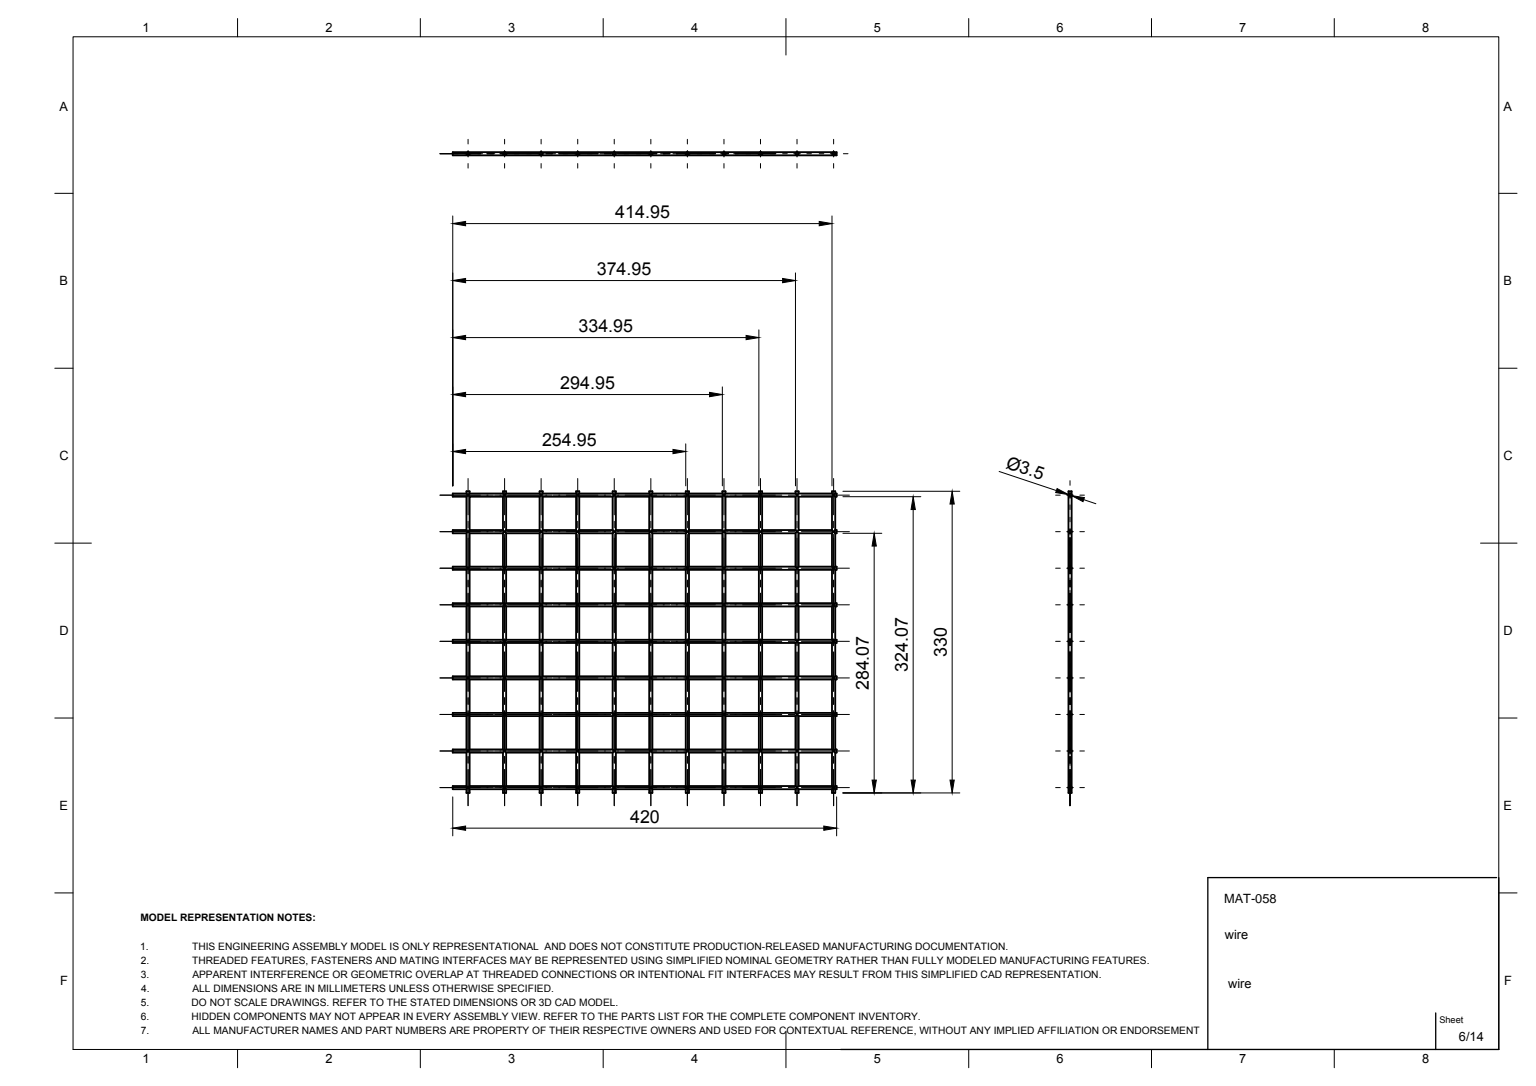
ISO-10303-21;
HEADER;
FILE_DESCRIPTION (('STEP AP214'),
    '1' );
FILE_NAME ('wire.step',
    '2026-10-21T17:54:40',
    ( '' ),
    ( '' ),
    'SwSTEP 2.0',
    'SolidWorks 2026',
    '' );
FILE_SCHEMA (( 'AUTOMOTIVE_DESIGN' ));
ENDSEC;

DATA;
#4=FACE_OUTER_BOUND ( 'NONE', #5138, .T. ) ;
#5=ORIENTED_EDGE ( 'NONE', *, *, #50322, .T. ) ;
#7=ORIENTED_EDGE ( 'NONE', *, *, #34701, .F. ) ;
#9=DIRECTION ( 'NONE',  ( -1.000000000000000000, -0.000000000000000000, -0.000000000000000000 ) ) ;
#11=ORIENTED_EDGE ( 'NONE', *, *, #36636, .F. ) ;
#12=EDGE_CURVE ( 'NONE', #49361, #27194, #1364, .T. ) ;
#14=ORIENTED_EDGE ( 'NONE', *, *, #5906, .T. ) ;
#15=CARTESIAN_POINT ( 'NONE',  ( 71.55402655318505367, 1.025126265847089657, 79.06828755692797017 ) ) ;
#16=DIRECTION ( 'NONE',  ( -1.000000000000000000, -0.000000000000000000, -0.000000000000000000 ) ) ;
#17=ORIENTED_EDGE ( 'NONE', *, *, #15192, .T. ) ;
#21=CARTESIAN_POINT ( 'NONE',  ( 191.5540265531851105, 0.000000000000000000, 162.5682875569279702 ) ) ;
#29=CARTESIAN_POINT ( 'NONE',  ( 155.0540265531850537, 2.143131898507880377E-16, -37.43171244307205825 ) ) ;
#39=CARTESIAN_POINT ( 'NONE',  ( -48.44597344681495343, 0.000000000000000000, 159.0682875569279702 ) ) ;
#41=DIRECTION ( 'NONE',  ( -1.000000000000000000, -0.000000000000000000, -0.000000000000000000 ) ) ;
#47=ADVANCED_FACE ( 'NONE', ( #25459 ), #1863, .T. ) ;
#50=CARTESIAN_POINT ( 'NONE',  ( 112.2789002873379758, -1.749999999999996891, -80.20683870891909351 ) ) ;
#54=CARTESIAN_POINT ( 'NONE',  ( -85.67084718096784002, 1.750000000000010214, -118.1565861772249519 ) ) ;
#60=AXIS2_PLACEMENT_3D ( 'NONE', #7908, #4040, #30745 ) ;
#63=ORIENTED_EDGE ( 'NONE', *, *, #25801, .F. ) ;
#64=CYLINDRICAL_SURFACE ( 'NONE', #8155, 1.750000000000001554 ) ;
#66=ORIENTED_EDGE ( 'NONE', *, *, #13113, .F. ) ;
#78=DIRECTION ( 'NONE',  ( -0.000000000000000000, -0.000000000000000000, -1.000000000000000000 ) ) ;
#81=EDGE_CURVE ( 'NONE', #16655, #7516, #13481, .T. ) ;
#82=ORIENTED_EDGE ( 'NONE', *, *, #7839, .T. ) ;
#85=ORIENTED_EDGE ( 'NONE', *, *, #19964, .F. ) ;
#86=CARTESIAN_POINT ( 'NONE',  ( 71.55402655318505367, 0.000000000000000000, 165.0000000000000000 ) ) ;
#90=CARTESIAN_POINT ( 'NONE',  ( 193.3040265531851105, 1.750000000000010658, 80.81828755692798438 ) ) ;
#95=CARTESIAN_POINT ( 'NONE',  ( 111.5540265531850679, 0.000000000000000000, -77.43171244307204404 ) ) ;
#104=CARTESIAN_POINT ( 'NONE',  ( -164.9459734468149463, 1.025126265847089435, -40.93171244307204404 ) ) ;
#112=ORIENTED_EDGE ( 'NONE', *, *, #36233, .F. ) ;
#113=EDGE_CURVE ( 'NONE', #40036, #44970, #10285, .T. ) ;
#122=( BOUNDED_CURVE ( )  B_SPLINE_CURVE ( 3, ( #11119, #46228, #4929, #44170 ),
 .UNSPECIFIED., .F., .F. ) 
 B_SPLINE_CURVE_WITH_KNOTS ( ( 4, 4 ),
 ( 0.000000000000000000, 1.570796326794896558 ),
 .UNSPECIFIED. ) 
 CURVE ( )  GEOMETRIC_REPRESENTATION_ITEM ( )  RATIONAL_B_SPLINE_CURVE ( ( 1.000000000000000000, 0.8047378541243649375, 0.8047378541243649375, 1.000000000000000000 ) ) 
 REPRESENTATION_ITEM ( '' )  );
#124=DIRECTION ( 'NONE',  ( -0.000000000000000000, -0.000000000000000000, -1.000000000000000000 ) ) ;
#136=CARTESIAN_POINT ( 'NONE',  ( -127.7210997126620242, -1.749999999999996891, 119.7931612910809065 ) ) ;
#139=ORIENTED_EDGE ( 'NONE', *, *, #39135, .F. ) ;
#143=ADVANCED_FACE ( 'NONE', ( #18750 ), #30578, .T. ) ;
#144=FACE_OUTER_BOUND ( 'NONE', #19501, .T. ) ;
#145=ORIENTED_EDGE ( 'NONE', *, *, #17426, .F. ) ;
#147=CARTESIAN_POINT ( 'NONE',  ( -44.94597344681493922, 2.143131898507880377E-16, -37.43171244307200141 ) ) ;
#155=DIRECTION ( 'NONE',  ( 0.000000000000000000, 0.000000000000000000, 1.000000000000000000 ) ) ;
#159=CARTESIAN_POINT ( 'NONE',  ( 73.30402655318508209, 1.750000000000010658, -119.1817124430720440 ) ) ;
#160=ORIENTED_EDGE ( 'NONE', *, *, #20171, .T. ) ;
#161=ORIENTED_EDGE ( 'NONE', *, *, #26521, .T. ) ;
#163=CARTESIAN_POINT ( 'NONE',  ( -124.9459734468149463, 2.143131898507847836E-16, -120.9317124430720156 ) ) ;
#172=EDGE_CURVE ( 'NONE', #7661, #23271, #44918, .T. ) ;
#173=CARTESIAN_POINT ( 'NONE',  ( 113.3040265531850537, 1.749999999999997113, 40.81828755692798438 ) ) ;
#179=ORIENTED_EDGE ( 'NONE', *, *, #14430, .F. ) ;
#182=ADVANCED_FACE ( 'NONE', ( #17198 ), #5386, .T. ) ;
#183=DIRECTION ( 'NONE',  ( -1.000000000000000000, -0.000000000000000000, -0.000000000000000000 ) ) ;
#184=CARTESIAN_POINT ( 'NONE',  ( 115.0540265531850395, 2.143131898507847836E-16, 42.56828755692795596 ) ) ;
#190=CARTESIAN_POINT ( 'NONE',  ( 151.5540265531850537, 1.025126265847089435, 39.06828755692797728 ) ) ;
#191=ORIENTED_EDGE ( 'NONE', *, *, #24035, .F. ) ;
#192=CARTESIAN_POINT ( 'NONE',  ( -88.44597344681497475, 0.000000000000000000, 122.5682875569279986 ) ) ;
#194=ADVANCED_FACE ( 'NONE', ( #21045 ), #12090, .T. ) ;
#199=CYLINDRICAL_SURFACE ( 'NONE', #44476, 1.750000000000015543 ) ;
#201=AXIS2_PLACEMENT_3D ( 'NONE', #39874, #40365, #36024 ) ;
#202=ORIENTED_EDGE ( 'NONE', *, *, #48337, .T. ) ;
#205=ORIENTED_EDGE ( 'NONE', *, *, #34328, .T. ) ;
#206=CARTESIAN_POINT ( 'NONE',  ( -46.69597344681494633, -1.750000000000010214, -39.18171244307202983 ) ) ;
#214=VERTEX_POINT ( 'NONE', #5134 ) ;
#217=DIRECTION ( 'NONE',  ( -1.000000000000000000, -0.000000000000000000, -0.000000000000000000 ) ) ;
#222=EDGE_CURVE ( 'NONE', #31646, #38096, #39265, .T. ) ;
#226=VECTOR ( 'NONE', #47044, 1000.000000000000000 ) ;
#228=ORIENTED_EDGE ( 'NONE', *, *, #24802, .T. ) ;
#229=CARTESIAN_POINT ( 'NONE',  ( -166.6959734468149463, -1.750000000000010658, -79.18171244307201562 ) ) ;
#232=ADVANCED_FACE ( 'NONE', ( #4388 ), #35956, .T. ) ;
#237=AXIS2_PLACEMENT_3D ( 'NONE', #8518, #24169, #12111 ) ;
#242=EDGE_CURVE ( 'NONE', #42713, #16089, #36464, .T. ) ;
#247=EDGE_CURVE ( 'NONE', #43286, #47057, #22018, .T. ) ;
#248=LINE ( 'NONE', #3822, #36404 ) ;
#249=CARTESIAN_POINT ( 'NONE',  ( -128.4459734468149179, 0.000000000000000000, -117.4317124430720725 ) ) ;
#252=CARTESIAN_POINT ( 'NONE',  ( -86.69597344681494633, -1.750000000000009992, 0.8182875569279768335 ) ) ;
#258=CARTESIAN_POINT ( 'NONE',  ( 155.0540265531850537, 2.143131898507880377E-16, 165.0000000000000000 ) ) ;
#259=( BOUNDED_CURVE ( )  B_SPLINE_CURVE ( 3, ( #2249, #37429, #6606, #3247 ),
 .UNSPECIFIED., .F., .F. ) 
 B_SPLINE_CURVE_WITH_KNOTS ( ( 4, 4 ),
 ( 1.570796326794896558, 3.141592653589793116 ),
 .UNSPECIFIED. ) 
 CURVE ( )  GEOMETRIC_REPRESENTATION_ITEM ( )  RATIONAL_B_SPLINE_CURVE ( ( 1.000000000000000000, 0.8047378541243649375, 0.8047378541243649375, 1.000000000000000000 ) ) 
 REPRESENTATION_ITEM ( '' )  );
#266=DIRECTION ( 'NONE',  ( 0.000000000000000000, 0.000000000000000000, 1.000000000000000000 ) ) ;
#267=( BOUNDED_CURVE ( )  B_SPLINE_CURVE ( 3, ( #50247, #49055, #13937, #13448 ),
 .UNSPECIFIED., .F., .F. ) 
 B_SPLINE_CURVE_WITH_KNOTS ( ( 4, 4 ),
 ( 4.712388980384689674, 6.283185307179586232 ),
 .UNSPECIFIED. ) 
 CURVE ( )  GEOMETRIC_REPRESENTATION_ITEM ( )  RATIONAL_B_SPLINE_CURVE ( ( 1.000000000000000000, 0.8047378541243649375, 0.8047378541243649375, 1.000000000000000000 ) ) 
 REPRESENTATION_ITEM ( '' )  );
#268=ORIENTED_EDGE ( 'NONE', *, *, #3344, .T. ) ;
#271=CARTESIAN_POINT ( 'NONE',  ( 71.55402655318506788, 0.000000000000000000, 162.5682875569279702 ) ) ;
#273=VECTOR ( 'NONE', #4541, 1000.000000000000000 ) ;
#275=CARTESIAN_POINT ( 'NONE',  ( -84.94597344681493212, 1.025126265847089879, 122.5682875569280128 ) ) ;
#283=ORIENTED_EDGE ( 'NONE', *, *, #247, .F. ) ;
#288=CARTESIAN_POINT ( 'NONE',  ( -168.4459734468149463, 0.000000000000000000, 2.568287556927978166 ) ) ;
#293=LINE ( 'NONE', #43877, #10669 ) ;
#294=CARTESIAN_POINT ( 'NONE',  ( 74.32915281903215998, -1.750000000000009548, -78.15658617722490931 ) ) ;
#307=CARTESIAN_POINT ( 'NONE',  ( 113.3040265531850537, -1.749999999999997335, -79.18171244307201562 ) ) ;
#309=CARTESIAN_POINT ( 'NONE',  ( 192.2789002873380184, 1.750000000000009548, 39.79316129108089228 ) ) ;
#314=EDGE_CURVE ( 'NONE', #4361, #2042, #6678, .T. ) ;
#317=DIRECTION ( 'NONE',  ( -0.000000000000000000, -0.000000000000000000, -1.000000000000000000 ) ) ;
#320=CYLINDRICAL_SURFACE ( 'NONE', #46063, 1.750000000000015543 ) ;
#322=CARTESIAN_POINT ( 'NONE',  ( -128.4459734468149179, 0.000000000000000000, 165.0000000000000000 ) ) ;
#326=FACE_OUTER_BOUND ( 'NONE', #20541, .T. ) ;
#329=CARTESIAN_POINT ( 'NONE',  ( 191.5540265531850537, -1.025126265847089435, -157.4317124430720582 ) ) ;
#349=EDGE_LOOP ( 'NONE', ( #28250, #8227, #4948, #139, #25034, #3385 ) ) ;
#358=ORIENTED_EDGE ( 'NONE', *, *, #25263, .T. ) ;
#360=DIRECTION ( 'NONE',  ( 0.000000000000000000, 0.000000000000000000, 1.000000000000000000 ) ) ;
#361=CARTESIAN_POINT ( 'NONE',  ( -84.94597344681493212, -1.025126265847088991, 159.0682875569279418 ) ) ;
#367=ORIENTED_EDGE ( 'NONE', *, *, #18075, .F. ) ;
#368=CARTESIAN_POINT ( 'NONE',  ( -126.6959734468149321, -1.749999999999997335, 80.81828755692798438 ) ) ;
#371=VECTOR ( 'NONE', #12956, 1000.000000000000000 ) ;
#374=EDGE_LOOP ( 'NONE', ( #37007, #35684, #23876, #49067, #24411 ) ) ;
#379=FACE_OUTER_BOUND ( 'NONE', #33356, .T. ) ;
#381=AXIS2_PLACEMENT_3D ( 'NONE', #4181, #15227, #23679 ) ;
#382=CARTESIAN_POINT ( 'NONE',  ( 195.0540265531851105, 2.143131898507880377E-16, 79.06828755692797017 ) ) ;
#383=ORIENTED_EDGE ( 'NONE', *, *, #37796, .F. ) ;
#387=VERTEX_POINT ( 'NONE', #1801 ) ;
#394=CARTESIAN_POINT ( 'NONE',  ( 153.3040265531850537, 1.750000000000010658, 80.81828755692798438 ) ) ;
#406=ORIENTED_EDGE ( 'NONE', *, *, #20191, .F. ) ;
#407=DIRECTION ( 'NONE',  ( -0.000000000000000000, -0.000000000000000000, -1.000000000000000000 ) ) ;
#411=ORIENTED_EDGE ( 'NONE', *, *, #49299, .F. ) ;
#413=CARTESIAN_POINT ( 'NONE',  ( -126.6959734468149321, -1.749999999999997113, -39.18171244307202983 ) ) ;
#415=( BOUNDED_CURVE ( )  B_SPLINE_CURVE ( 3, ( #5683, #44416, #25963, #48241 ),
 .UNSPECIFIED., .F., .F. ) 
 B_SPLINE_CURVE_WITH_KNOTS ( ( 4, 4 ),
 ( 4.712388980384689674, 6.283185307179586232 ),
 .UNSPECIFIED. ) 
 CURVE ( )  GEOMETRIC_REPRESENTATION_ITEM ( )  RATIONAL_B_SPLINE_CURVE ( ( 1.000000000000000000, 0.8047378541243649375, 0.8047378541243649375, 1.000000000000000000 ) ) 
 REPRESENTATION_ITEM ( '' )  );
#421=ORIENTED_EDGE ( 'NONE', *, *, #38475, .T. ) ;
#423=CARTESIAN_POINT ( 'NONE',  ( -47.72109971266203132, 1.750000000000010436, 119.7931612910808781 ) ) ;
#425=CYLINDRICAL_SURFACE ( 'NONE', #22465, 1.750000000000001554 ) ;
#429=DIRECTION ( 'NONE',  ( -1.000000000000000000, 0.000000000000000000, 0.000000000000000000 ) ) ;
#431=EDGE_CURVE ( 'NONE', #16089, #12079, #28992, .T. ) ;
#436=AXIS2_PLACEMENT_3D ( 'NONE', #25349, #45321, #26098 ) ;
#440=EDGE_CURVE ( 'NONE', #43432, #19548, #26025, .T. ) ;
#443=VECTOR ( 'NONE', #3485, 1000.000000000000000 ) ;
#447=CARTESIAN_POINT ( 'NONE',  ( 35.05402655318504657, 2.143131898507880377E-16, 42.56828755692798438 ) ) ;
#448=DIRECTION ( 'NONE',  ( 0.000000000000000000, 0.000000000000000000, 1.000000000000000000 ) ) ;
#452=ADVANCED_FACE ( 'NONE', ( #16069 ), #23519, .T. ) ;
#454=ORIENTED_EDGE ( 'NONE', *, *, #15929, .F. ) ;
#458=EDGE_CURVE ( 'NONE', #40596, #15960, #31982, .T. ) ;
#459=EDGE_CURVE ( 'NONE', #16448, #40222, #8626, .T. ) ;
#464=EDGE_CURVE ( 'NONE', #48470, #25557, #25629, .T. ) ;
#466=DIRECTION ( 'NONE',  ( 0.000000000000000000, 0.000000000000000000, 1.000000000000000000 ) ) ;
#467=ORIENTED_EDGE ( 'NONE', *, *, #8643, .T. ) ;
#470=AXIS2_PLACEMENT_3D ( 'NONE', #3136, #22152, #46465 ) ;
#472=CYLINDRICAL_SURFACE ( 'NONE', #11197, 1.750000000000008438 ) ;
#482=EDGE_CURVE ( 'NONE', #50669, #27161, #35845, .T. ) ;
#485=DIRECTION ( 'NONE',  ( -0.000000000000000000, -0.000000000000000000, -1.000000000000000000 ) ) ;
#488=CARTESIAN_POINT ( 'NONE',  ( -87.72109971266203843, -1.750000000000009548, 159.7931612910809065 ) ) ;
#491=AXIS2_PLACEMENT_3D ( 'NONE', #861, #24715, #16507 ) ;
#502=( BOUNDED_CURVE ( )  B_SPLINE_CURVE ( 3, ( #2955, #14255, #29915, #26067 ),
 .UNSPECIFIED., .F., .F. ) 
 B_SPLINE_CURVE_WITH_KNOTS ( ( 4, 4 ),
 ( 1.570796326794896558, 3.141592653589793116 ),
 .UNSPECIFIED. ) 
 CURVE ( )  GEOMETRIC_REPRESENTATION_ITEM ( )  RATIONAL_B_SPLINE_CURVE ( ( 1.000000000000000000, 0.8047378541243649375, 0.8047378541243649375, 1.000000000000000000 ) ) 
 REPRESENTATION_ITEM ( '' )  );
#506=CARTESIAN_POINT ( 'NONE',  ( 193.3040265531851105, 1.750000000000010658, -119.1817124430720440 ) ) ;
#507=CARTESIAN_POINT ( 'NONE',  ( 113.3040265531850537, -1.749999999999996891, 160.8182875569279702 ) ) ;
#510=ORIENTED_EDGE ( 'NONE', *, *, #27958, .F. ) ;
#511=FACE_OUTER_BOUND ( 'NONE', #39266, .T. ) ;
#519=CARTESIAN_POINT ( 'NONE',  ( 191.5540265531851105, 0.000000000000000000, -77.43171244307204404 ) ) ;
#520=CARTESIAN_POINT ( 'NONE',  ( 111.5540265531850537, 1.025126265847081886, -120.9317124430720440 ) ) ;
#523=ORIENTED_EDGE ( 'NONE', *, *, #44396, .T. ) ;
#526=ADVANCED_FACE ( 'NONE', ( #38927 ), #19406, .T. ) ;
#527=ORIENTED_EDGE ( 'NONE', *, *, #43614, .T. ) ;
#531=ORIENTED_EDGE ( 'NONE', *, *, #41855, .T. ) ;
#532=CARTESIAN_POINT ( 'NONE',  ( -126.6959734468149321, 1.749999999999996891, -159.1817124430720298 ) ) ;
#534=EDGE_CURVE ( 'NONE', #28470, #12513, #27359, .T. ) ;
#538=AXIS2_PLACEMENT_3D ( 'NONE', #2831, #26198, #14128 ) ;
#543=CARTESIAN_POINT ( 'NONE',  ( -127.7210997126620242, -1.749999999999996891, -80.20683870891909351 ) ) ;
#544=EDGE_LOOP ( 'NONE', ( #3336, #43444, #1050, #33795, #29407 ) ) ;
#546=FACE_OUTER_BOUND ( 'NONE', #42414, .T. ) ;
#547=ORIENTED_EDGE ( 'NONE', *, *, #1230, .F. ) ;
#548=LINE ( 'NONE', #16187, #556 ) ;
#555=CARTESIAN_POINT ( 'NONE',  ( -206.6959734468149463, 0.000000000000000000, 165.0000000000000000 ) ) ;
#556=VECTOR ( 'NONE', #4868, 1000.000000000000000 ) ;
#559=VERTEX_POINT ( 'NONE', #44993 ) ;
#560=ORIENTED_EDGE ( 'NONE', *, *, #34963, .T. ) ;
#563=( BOUNDED_CURVE ( )  B_SPLINE_CURVE ( 3, ( #5786, #21426, #38810, #49593 ),
 .UNSPECIFIED., .F., .F. ) 
 B_SPLINE_CURVE_WITH_KNOTS ( ( 4, 4 ),
 ( 1.570796326794896558, 3.141592653589793116 ),
 .UNSPECIFIED. ) 
 CURVE ( )  GEOMETRIC_REPRESENTATION_ITEM ( )  RATIONAL_B_SPLINE_CURVE ( ( 1.000000000000000000, 0.8047378541243649375, 0.8047378541243649375, 1.000000000000000000 ) ) 
 REPRESENTATION_ITEM ( '' )  );
#567=DIRECTION ( 'NONE',  ( -1.000000000000000000, -0.000000000000000000, -0.000000000000000000 ) ) ;
#568=( BOUNDED_CURVE ( )  B_SPLINE_CURVE ( 3, ( #26623, #27136, #28083, #11235 ),
 .UNSPECIFIED., .F., .F. ) 
 B_SPLINE_CURVE_WITH_KNOTS ( ( 4, 4 ),
 ( 1.570796326794896558, 3.141592653589793116 ),
 .UNSPECIFIED. ) 
 CURVE ( )  GEOMETRIC_REPRESENTATION_ITEM ( )  RATIONAL_B_SPLINE_CURVE ( ( 1.000000000000000000, 0.8047378541243649375, 0.8047378541243649375, 1.000000000000000000 ) ) 
 REPRESENTATION_ITEM ( '' )  );
#569=CARTESIAN_POINT ( 'NONE',  ( -47.72109971266203132, -1.750000000000009548, 41.84341382277508359 ) ) ;
#571=DIRECTION ( 'NONE',  ( 0.000000000000000000, 0.000000000000000000, 1.000000000000000000 ) ) ;
#573=DIRECTION ( 'NONE',  ( -1.000000000000000000, -0.000000000000000000, -0.000000000000000000 ) ) ;
#575=FACE_OUTER_BOUND ( 'NONE', #37918, .T. ) ;
#577=CARTESIAN_POINT ( 'NONE',  ( -4.945973446814917018, 1.025126265847097429, 42.56828755692800570 ) ) ;
#578=CARTESIAN_POINT ( 'NONE',  ( -4.945973446814903696, 2.143131898507912917E-16, 2.568287556928034121 ) ) ;
#580=ORIENTED_EDGE ( 'NONE', *, *, #21589, .T. ) ;
#581=ADVANCED_FACE ( 'NONE', ( #9872 ), #36344, .T. ) ;
#583=EDGE_CURVE ( 'NONE', #42490, #24640, #48326, .T. ) ;
#585=DIRECTION ( 'NONE',  ( -1.000000000000000000, 0.000000000000000000, 0.000000000000000000 ) ) ;
#587=CARTESIAN_POINT ( 'NONE',  ( -206.6959734468149463, 1.750000000000010214, -39.18171244307202983 ) ) ;
#588=CARTESIAN_POINT ( 'NONE',  ( 32.27890028733795447, -1.750000000000009548, 41.84341382277508359 ) ) ;
#591=ORIENTED_EDGE ( 'NONE', *, *, #21037, .F. ) ;
#595=EDGE_CURVE ( 'NONE', #49549, #4874, #20923, .T. ) ;
#600=FACE_OUTER_BOUND ( 'NONE', #36261, .T. ) ;
#601=ORIENTED_EDGE ( 'NONE', *, *, #3400, .F. ) ;
#602=CARTESIAN_POINT ( 'NONE',  ( 195.0540265531851105, 2.143131898507880377E-16, 79.06828755692797017 ) ) ;
#604=ADVANCED_FACE ( 'NONE', ( #36090 ), #930, .T. ) ;
#610=DIRECTION ( 'NONE',  ( -1.000000000000000000, -0.000000000000000000, -0.000000000000000000 ) ) ;
#611=CARTESIAN_POINT ( 'NONE',  ( -5.670847180967843570, -1.750000000000023315, 121.8434138227750623 ) ) ;
#620=CARTESIAN_POINT ( 'NONE',  ( 34.32915281903212446, 1.750000000000009326, 161.8434138227750907 ) ) ;
#630=FACE_OUTER_BOUND ( 'NONE', #38256, .T. ) ;
#635=ORIENTED_EDGE ( 'NONE', *, *, #15818, .F. ) ;
#638=DIRECTION ( 'NONE',  ( 0.000000000000000000, 0.000000000000000000, -1.000000000000000000 ) ) ;
#641=DIRECTION ( 'NONE',  ( -0.000000000000000000, -0.000000000000000000, -1.000000000000000000 ) ) ;
#645=ORIENTED_EDGE ( 'NONE', *, *, #18172, .T. ) ;
#646=CARTESIAN_POINT ( 'NONE',  ( -124.9459734468149463, 2.143131898507847836E-16, -120.9317124430720156 ) ) ;
#649=DIRECTION ( 'NONE',  ( -0.000000000000000000, -0.000000000000000000, -1.000000000000000000 ) ) ;
#652=ORIENTED_EDGE ( 'NONE', *, *, #762, .F. ) ;
#653=ADVANCED_FACE ( 'NONE', ( #40684 ), #36606, .T. ) ;
#658=ORIENTED_EDGE ( 'NONE', *, *, #1230, .T. ) ;
#662=CIRCLE ( 'NONE', #47316, 1.750000000000001554 ) ;
#663=CARTESIAN_POINT ( 'NONE',  ( -204.9459734468149463, 2.143131898507880377E-16, 2.568287556927978166 ) ) ;
#667=CARTESIAN_POINT ( 'NONE',  ( -126.6959734468149321, 1.749999999999997335, 80.81828755692798438 ) ) ;
#676=CARTESIAN_POINT ( 'NONE',  ( 155.0540265531850537, 1.025126265847089879, 122.5682875569280128 ) ) ;
#683=( BOUNDED_CURVE ( )  B_SPLINE_CURVE ( 3, ( #1713, #9405, #36121, #5040 ),
 .UNSPECIFIED., .F., .F. ) 
 B_SPLINE_CURVE_WITH_KNOTS ( ( 4, 4 ),
 ( 1.570796326794896558, 3.141592653589793116 ),
 .UNSPECIFIED. ) 
 CURVE ( )  GEOMETRIC_REPRESENTATION_ITEM ( )  RATIONAL_B_SPLINE_CURVE ( ( 1.000000000000000000, 0.8047378541243649375, 0.8047378541243649375, 1.000000000000000000 ) ) 
 REPRESENTATION_ITEM ( '' )  );
#687=ORIENTED_EDGE ( 'NONE', *, *, #36269, .F. ) ;
#689=CARTESIAN_POINT ( 'NONE',  ( 154.3291528190321458, -1.750000000000009548, -40.20683870891912193 ) ) ;
#691=CYLINDRICAL_SURFACE ( 'NONE', #41373, 1.750000000000015543 ) ;
#698=CARTESIAN_POINT ( 'NONE',  ( -210.0000000000000568, 0.000000000000000000, -119.1817124430720440 ) ) ;
#700=DIRECTION ( 'NONE',  ( 1.000000000000000000, 0.000000000000000000, 0.000000000000000000 ) ) ;
#703=ADVANCED_FACE ( 'NONE', ( #24523 ), #36856, .T. ) ;
#704=( BOUNDED_CURVE ( )  B_SPLINE_CURVE ( 3, ( #40799, #48942, #14089, #33120 ),
 .UNSPECIFIED., .F., .F. ) 
 B_SPLINE_CURVE_WITH_KNOTS ( ( 4, 4 ),
 ( 0.000000000000000000, 1.570796326794896558 ),
 .UNSPECIFIED. ) 
 CURVE ( )  GEOMETRIC_REPRESENTATION_ITEM ( )  RATIONAL_B_SPLINE_CURVE ( ( 1.000000000000000000, 0.8047378541243649375, 0.8047378541243649375, 1.000000000000000000 ) ) 
 REPRESENTATION_ITEM ( '' )  );
#705=CARTESIAN_POINT ( 'NONE',  ( 75.05402655318509630, 1.025126265847089879, 82.56828755692798438 ) ) ;
#713=CARTESIAN_POINT ( 'NONE',  ( 75.05402655318509630, 1.025126265847089879, 122.5682875569280128 ) ) ;
#714=ORIENTED_EDGE ( 'NONE', *, *, #39946, .T. ) ;
#719=EDGE_CURVE ( 'NONE', #32283, #25110, #43691, .T. ) ;
#725=CARTESIAN_POINT ( 'NONE',  ( 113.3040265531850537, 0.000000000000000000, 165.0000000000000000 ) ) ;
#729=CYLINDRICAL_SURFACE ( 'NONE', #31264, 1.750000000000015543 ) ;
#730=CARTESIAN_POINT ( 'NONE',  ( 152.2789002873379900, 1.750000000000009548, 159.7931612910809065 ) ) ;
#731=CARTESIAN_POINT ( 'NONE',  ( -204.9459734468149463, 2.143131898507880377E-16, -80.93171244307201562 ) ) ;
#734=PLANE ( 'NONE',  #17438 ) ;
#735=EDGE_CURVE ( 'NONE', #23031, #24640, #41747, .T. ) ;
#738=DIRECTION ( 'NONE',  ( -1.000000000000000000, -0.000000000000000000, -0.000000000000000000 ) ) ;
#741=CARTESIAN_POINT ( 'NONE',  ( -204.9459734468149463, 2.143131898507880377E-16, 39.06828755692798438 ) ) ;
#743=ORIENTED_EDGE ( 'NONE', *, *, #50525, .T. ) ;
#746=DIRECTION ( 'NONE',  ( -0.000000000000000000, -0.000000000000000000, -1.000000000000000000 ) ) ;
#748=CARTESIAN_POINT ( 'NONE',  ( 153.3040265531850537, -1.750000000000009992, 160.8182875569279702 ) ) ;
#749=VECTOR ( 'NONE', #19138, 1000.000000000000000 ) ;
#757=CARTESIAN_POINT ( 'NONE',  ( -124.9459734468149463, 2.143131898507847836E-16, -77.43171244307204404 ) ) ;
#758=VECTOR ( 'NONE', #16905, 1000.000000000000000 ) ;
#760=ORIENTED_EDGE ( 'NONE', *, *, #40276, .T. ) ;
#762=EDGE_CURVE ( 'NONE', #38466, #44684, #48892, .T. ) ;
#765=AXIS2_PLACEMENT_3D ( 'NONE', #29029, #12869, #12609 ) ;
#778=EDGE_CURVE ( 'NONE', #19154, #19994, #662, .T. ) ;
#784=DIRECTION ( 'NONE',  ( 1.000000000000000000, 0.000000000000000000, 0.000000000000000000 ) ) ;
#787=AXIS2_PLACEMENT_3D ( 'NONE', #7371, #10699, #11720 ) ;
#793=( BOUNDED_CURVE ( )  B_SPLINE_CURVE ( 3, ( #39098, #35003, #3405, #39345 ),
 .UNSPECIFIED., .F., .F. ) 
 B_SPLINE_CURVE_WITH_KNOTS ( ( 4, 4 ),
 ( 0.000000000000000000, 1.570796326794896558 ),
 .UNSPECIFIED. ) 
 CURVE ( )  GEOMETRIC_REPRESENTATION_ITEM ( )  RATIONAL_B_SPLINE_CURVE ( ( 1.000000000000000000, 0.8047378541243649375, 0.8047378541243649375, 1.000000000000000000 ) ) 
 REPRESENTATION_ITEM ( '' )  );
#796=VECTOR ( 'NONE', #5565, 1000.000000000000000 ) ;
#800=ORIENTED_EDGE ( 'NONE', *, *, #21171, .T. ) ;
#801=ADVANCED_FACE ( 'NONE', ( #14216 ), #41679, .T. ) ;
#807=EDGE_CURVE ( 'NONE', #14566, #8176, #18570, .T. ) ;
#809=DIRECTION ( 'NONE',  ( -1.000000000000000000, 0.000000000000000000, 0.000000000000000000 ) ) ;
#810=CARTESIAN_POINT ( 'NONE',  ( -85.67084718096784002, -1.750000000000010436, -80.20683870891910772 ) ) ;
#815=ADVANCED_FACE ( 'NONE', ( #7814 ), #26795, .T. ) ;
#824=CARTESIAN_POINT ( 'NONE',  ( 195.0540265531851105, 2.143131898507880377E-16, -80.93171244307201562 ) ) ;
#829=VERTEX_POINT ( 'NONE', #368 ) ;
#830=AXIS2_PLACEMENT_3D ( 'NONE', #22262, #22003, #42013 ) ;
#833=EDGE_CURVE ( 'NONE', #38070, #15143, #32836, .T. ) ;
#836=CARTESIAN_POINT ( 'NONE',  ( -208.4459734468148611, 1.025126265847089213, -37.43171244307202272 ) ) ;
#837=CARTESIAN_POINT ( 'NONE',  ( -44.94597344681493922, 2.143131898507880377E-16, 165.0000000000000000 ) ) ;
#840=AXIS2_PLACEMENT_3D ( 'NONE', #7728, #46676, #34680 ) ;
#841=ORIENTED_EDGE ( 'NONE', *, *, #33518, .T. ) ;
#851=LINE ( 'NONE', #19823, #3024 ) ;
#852=EDGE_CURVE ( 'NONE', #6557, #6202, #30915, .T. ) ;
#854=( BOUNDED_CURVE ( )  B_SPLINE_CURVE ( 3, ( #12564, #12315, #543, #19499 ),
 .UNSPECIFIED., .F., .F. ) 
 B_SPLINE_CURVE_WITH_KNOTS ( ( 4, 4 ),
 ( 0.000000000000000000, 1.570796326794896558 ),
 .UNSPECIFIED. ) 
 CURVE ( )  GEOMETRIC_REPRESENTATION_ITEM ( )  RATIONAL_B_SPLINE_CURVE ( ( 1.000000000000000000, 0.8047378541243649375, 0.8047378541243649375, 1.000000000000000000 ) ) 
 REPRESENTATION_ITEM ( '' )  );
#855=CARTESIAN_POINT ( 'NONE',  ( -204.9459734468148895, -1.025126265847089657, 119.0682875569279560 ) ) ;
#858=EDGE_CURVE ( 'NONE', #47433, #8314, #11391, .T. ) ;
#861=CARTESIAN_POINT ( 'NONE',  ( 153.3040265531850537, 0.000000000000000000, 165.0000000000000000 ) ) ;
#862=( BOUNDED_CURVE ( )  B_SPLINE_CURVE ( 3, ( #46764, #38884, #31695, #35808 ),
 .UNSPECIFIED., .F., .F. ) 
 B_SPLINE_CURVE_WITH_KNOTS ( ( 4, 4 ),
 ( 0.000000000000000000, 1.570796326794896780 ),
 .UNSPECIFIED. ) 
 CURVE ( )  GEOMETRIC_REPRESENTATION_ITEM ( )  RATIONAL_B_SPLINE_CURVE ( ( 1.000000000000000000, 0.8047378541243649375, 0.8047378541243649375, 1.000000000000000000 ) ) 
 REPRESENTATION_ITEM ( '' )  );
#864=ORIENTED_EDGE ( 'NONE', *, *, #18638, .T. ) ;
#868=ORIENTED_EDGE ( 'NONE', *, *, #35811, .F. ) ;
#872=CARTESIAN_POINT ( 'NONE',  ( 155.0540265531850537, -1.025126265847088991, -157.4317124430720582 ) ) ;
#886=DIRECTION ( 'NONE',  ( 1.000000000000000000, 0.000000000000000000, -0.000000000000000000 ) ) ;
#903=CARTESIAN_POINT ( 'NONE',  ( 153.3040265531850537, -1.750000000000010658, -119.1817124430720440 ) ) ;
#906=AXIS2_PLACEMENT_3D ( 'NONE', #14046, #29713, #45328 ) ;
#909=CARTESIAN_POINT ( 'NONE',  ( -44.94597344681493922, 2.143131898507880377E-16, 159.0682875569279702 ) ) ;
#910=CARTESIAN_POINT ( 'NONE',  ( 35.05402655318504657, 2.143131898507880377E-16, 42.56828755692798438 ) ) ;
#911=CARTESIAN_POINT ( 'NONE',  ( -204.9459734468148895, 1.025126265847089213, -0.9317124430720324924 ) ) ;
#915=ORIENTED_EDGE ( 'NONE', *, *, #35068, .T. ) ;
#918=CARTESIAN_POINT ( 'NONE',  ( -84.94597344681494633, 2.143131898507880377E-16, -77.43171244307204404 ) ) ;
#920=VERTEX_POINT ( 'NONE', #34765 ) ;
#923=FACE_OUTER_BOUND ( 'NONE', #18696, .T. ) ;
#924=CARTESIAN_POINT ( 'NONE',  ( -204.9459734468149463, 2.143131898507880377E-16, -117.4317124430720725 ) ) ;
#925=ORIENTED_EDGE ( 'NONE', *, *, #735, .T. ) ;
#926=ORIENTED_EDGE ( 'NONE', *, *, #50038, .F. ) ;
#928=CARTESIAN_POINT ( 'NONE',  ( -164.9459734468149463, 1.025126265847089657, -80.93171244307201562 ) ) ;
#930=CYLINDRICAL_SURFACE ( 'NONE', #24074, 1.750000000000015543 ) ;
#931=CARTESIAN_POINT ( 'NONE',  ( -207.7210997126620384, 1.750000000000009548, 121.8434138227750623 ) ) ;
#935=CARTESIAN_POINT ( 'NONE',  ( -84.94597344681494633, 2.143131898507873721E-16, 165.0000000000000000 ) ) ;
#936=VERTEX_POINT ( 'NONE', #12401 ) ;
#939=CARTESIAN_POINT ( 'NONE',  ( 210.0000000000000568, 0.000000000000000000, -79.18171244307201562 ) ) ;
#942=DIRECTION ( 'NONE',  ( -0.000000000000000000, -0.000000000000000000, -1.000000000000000000 ) ) ;
#944=ADVANCED_FACE ( 'NONE', ( #47762 ), #9567, .T. ) ;
#947=LINE ( 'NONE', #16587, #9432 ) ;
#956=CARTESIAN_POINT ( 'NONE',  ( -204.9459734468149463, 2.143131898507880377E-16, -77.43171244307204404 ) ) ;
#960=VERTEX_POINT ( 'NONE', #8817 ) ;
#962=CYLINDRICAL_SURFACE ( 'NONE', #6597, 1.750000000000008438 ) ;
#963=ORIENTED_EDGE ( 'NONE', *, *, #1726, .F. ) ;
#965=CYLINDRICAL_SURFACE ( 'NONE', #36426, 1.750000000000001554 ) ;
#969=CARTESIAN_POINT ( 'NONE',  ( 210.0000000000000568, 2.143131898507881856E-16, 119.0682875569279560 ) ) ;
#972=CARTESIAN_POINT ( 'NONE',  ( -8.445973446814962315, -1.025126265847097207, -157.4317124430720014 ) ) ;
#979=ORIENTED_EDGE ( 'NONE', *, *, #1420, .T. ) ;
#982=CARTESIAN_POINT ( 'NONE',  ( 191.5540265531850537, 1.025126265847089657, -80.93171244307201562 ) ) ;
#985=LINE ( 'NONE', #10188, #43833 ) ;
#986=CYLINDRICAL_SURFACE ( 'NONE', #23136, 1.750000000000008438 ) ;
#991=PLANE ( 'NONE',  #47135 ) ;
#992=FACE_OUTER_BOUND ( 'NONE', #20572, .T. ) ;
#995=( BOUNDED_CURVE ( )  B_SPLINE_CURVE ( 3, ( #20608, #1379, #32169, #1875 ),
 .UNSPECIFIED., .F., .F. ) 
 B_SPLINE_CURVE_WITH_KNOTS ( ( 4, 4 ),
 ( 0.000000000000000000, 1.570796326794896558 ),
 .UNSPECIFIED. ) 
 CURVE ( )  GEOMETRIC_REPRESENTATION_ITEM ( )  RATIONAL_B_SPLINE_CURVE ( ( 1.000000000000000000, 0.8047378541243649375, 0.8047378541243649375, 1.000000000000000000 ) ) 
 REPRESENTATION_ITEM ( '' )  );
#1000=FACE_OUTER_BOUND ( 'NONE', #32780, .T. ) ;
#1001=( BOUNDED_CURVE ( )  B_SPLINE_CURVE ( 3, ( #47575, #25032, #24518, #44247 ),
 .UNSPECIFIED., .F., .F. ) 
 B_SPLINE_CURVE_WITH_KNOTS ( ( 4, 4 ),
 ( 4.712388980384689674, 6.283185307179586232 ),
 .UNSPECIFIED. ) 
 CURVE ( )  GEOMETRIC_REPRESENTATION_ITEM ( )  RATIONAL_B_SPLINE_CURVE ( ( 1.000000000000000000, 0.8047378541243649375, 0.8047378541243649375, 1.000000000000000000 ) ) 
 REPRESENTATION_ITEM ( '' )  );
#1004=CARTESIAN_POINT ( 'NONE',  ( 210.0000000000000568, 0.000000000000000000, 0.8182875569279768335 ) ) ;
#1010=CARTESIAN_POINT ( 'NONE',  ( -210.0000000000000568, 0.000000000000000000, 80.81828755692798438 ) ) ;
#1015=( BOUNDED_CURVE ( )  B_SPLINE_CURVE ( 3, ( #7919, #15095, #7653, #30753 ),
 .UNSPECIFIED., .F., .F. ) 
 B_SPLINE_CURVE_WITH_KNOTS ( ( 4, 4 ),
 ( 4.712388980384689674, 6.283185307179586232 ),
 .UNSPECIFIED. ) 
 CURVE ( )  GEOMETRIC_REPRESENTATION_ITEM ( )  RATIONAL_B_SPLINE_CURVE ( ( 1.000000000000000000, 0.8047378541243649375, 0.8047378541243649375, 1.000000000000000000 ) ) 
 REPRESENTATION_ITEM ( '' )  );
#1017=ORIENTED_EDGE ( 'NONE', *, *, #10506, .T. ) ;
#1021=CARTESIAN_POINT ( 'NONE',  ( 210.0000000000000568, 0.000000000000000000, -79.18171244307201562 ) ) ;
#1022=VERTEX_POINT ( 'NONE', #16761 ) ;
#1023=FACE_OUTER_BOUND ( 'NONE', #10966, .T. ) ;
#1028=ORIENTED_EDGE ( 'NONE', *, *, #35334, .F. ) ;
#1030=ORIENTED_EDGE ( 'NONE', *, *, #46824, .F. ) ;
#1032=CARTESIAN_POINT ( 'NONE',  ( -86.69597344681496054, 0.000000000000000000, 165.0000000000000000 ) ) ;
#1040=CARTESIAN_POINT ( 'NONE',  ( -44.94597344681493922, 1.025126265847089657, 79.06828755692797017 ) ) ;
#1049=VERTEX_POINT ( 'NONE', #48515 ) ;
#1050=ORIENTED_EDGE ( 'NONE', *, *, #34971, .T. ) ;
#1052=CARTESIAN_POINT ( 'NONE',  ( -168.4459734468149747, 0.000000000000000000, 162.5682875569279702 ) ) ;
#1055=CARTESIAN_POINT ( 'NONE',  ( 191.5540265531850537, 1.025126265847089435, 39.06828755692797728 ) ) ;
#1059=CARTESIAN_POINT ( 'NONE',  ( 210.0000000000000568, 2.143131898507881856E-16, 119.0682875569279560 ) ) ;
#1061=VECTOR ( 'NONE', #15986, 1000.000000000000000 ) ;
#1062=CARTESIAN_POINT ( 'NONE',  ( -206.6959734468149463, -1.750000000000009992, 160.8182875569279702 ) ) ;
#1068=CARTESIAN_POINT ( 'NONE',  ( 193.3040265531851105, -1.750000000000010658, 120.8182875569279702 ) ) ;
#1072=DIRECTION ( 'NONE',  ( -0.000000000000000000, -0.000000000000000000, -1.000000000000000000 ) ) ;
#1075=CARTESIAN_POINT ( 'NONE',  ( -205.6708471809678827, 1.750000000000009548, -158.1565861772249377 ) ) ;
#1077=ORIENTED_EDGE ( 'NONE', *, *, #44672, .T. ) ;
#1081=ORIENTED_EDGE ( 'NONE', *, *, #27876, .T. ) ;
#1083=CARTESIAN_POINT ( 'NONE',  ( -5.670847180967843570, 1.750000000000022871, -160.2068387089191219 ) ) ;
#1085=DIRECTION ( 'NONE',  ( -0.000000000000000000, -0.000000000000000000, -1.000000000000000000 ) ) ;
#1086=ORIENTED_EDGE ( 'NONE', *, *, #37198, .T. ) ;
#1092=EDGE_CURVE ( 'NONE', #21408, #45663, #19109, .T. ) ;
#1093=EDGE_CURVE ( 'NONE', #47298, #26902, #31284, .T. ) ;
#1094=EDGE_LOOP ( 'NONE', ( #46101, #20220, #8122, #7542, #28111, #7098 ) ) ;
#1095=CARTESIAN_POINT ( 'NONE',  ( 33.30402655318503946, 0.000000000000000000, 165.0000000000000000 ) ) ;
#1098=( BOUNDED_CURVE ( )  B_SPLINE_CURVE ( 3, ( #43625, #11841, #40298, #12329 ),
 .UNSPECIFIED., .F., .F. ) 
 B_SPLINE_CURVE_WITH_KNOTS ( ( 4, 4 ),
 ( 0.000000000000000000, 1.570796326794896558 ),
 .UNSPECIFIED. ) 
 CURVE ( )  GEOMETRIC_REPRESENTATION_ITEM ( )  RATIONAL_B_SPLINE_CURVE ( ( 1.000000000000000000, 0.8047378541243649375, 0.8047378541243649375, 1.000000000000000000 ) ) 
 REPRESENTATION_ITEM ( '' )  );
#1099=ORIENTED_EDGE ( 'NONE', *, *, #42448, .F. ) ;
#1103=CARTESIAN_POINT ( 'NONE',  ( 111.5540265531850679, 0.000000000000000000, 79.06828755692798438 ) ) ;
#1110=EDGE_LOOP ( 'NONE', ( #43754, #46043, #30091, #454, #22015, #22407 ) ) ;
#1112=CIRCLE ( 'NONE', #1913, 1.749999999999987566 ) ;
#1113=CARTESIAN_POINT ( 'NONE',  ( -6.695973446814940111, -1.750000000000024203, 80.81828755692798438 ) ) ;
#1114=CARTESIAN_POINT ( 'NONE',  ( -6.695973446814940111, -1.750000000000023315, 0.8182875569279768335 ) ) ;
#1120=EDGE_LOOP ( 'NONE', ( #7077, #35444, #31188, #7911, #45465, #8066 ) ) ;
#1125=ADVANCED_FACE ( 'NONE', ( #2606 ), #42111, .T. ) ;
#1126=EDGE_CURVE ( 'NONE', #11740, #19783, #18760, .T. ) ;
#1129=CARTESIAN_POINT ( 'NONE',  ( -168.4459734468149747, 2.143131898507880377E-16, -160.9317124430720298 ) ) ;
#1135=DIRECTION ( 'NONE',  ( -1.000000000000000000, 0.000000000000000000, 0.000000000000000000 ) ) ;
#1139=CARTESIAN_POINT ( 'NONE',  ( 195.0540265531851105, 2.143131898507880377E-16, -40.93171244307202983 ) ) ;
#1141=EDGE_CURVE ( 'NONE', #23855, #44104, #48772, .T. ) ;
#1142=CARTESIAN_POINT ( 'NONE',  ( 210.0000000000000568, 2.143131898507881856E-16, 79.06828755692797017 ) ) ;
#1145=CARTESIAN_POINT ( 'NONE',  ( 111.5540265531850537, -1.025126265847082108, 82.56828755692798438 ) ) ;
#1149=CARTESIAN_POINT ( 'NONE',  ( -88.44597344681497475, 0.000000000000000000, -37.43171244307200141 ) ) ;
#1150=DIRECTION ( 'NONE',  ( 0.000000000000000000, 0.000000000000000000, 1.000000000000000000 ) ) ;
#1157=( BOUNDED_CURVE ( )  B_SPLINE_CURVE ( 3, ( #28676, #45302, #25091, #40741 ),
 .UNSPECIFIED., .F., .F. ) 
 B_SPLINE_CURVE_WITH_KNOTS ( ( 4, 4 ),
 ( 3.141592653589793116, 4.712388980384689674 ),
 .UNSPECIFIED. ) 
 CURVE ( )  GEOMETRIC_REPRESENTATION_ITEM ( )  RATIONAL_B_SPLINE_CURVE ( ( 1.000000000000000000, 0.8047378541243649375, 0.8047378541243649375, 1.000000000000000000 ) ) 
 REPRESENTATION_ITEM ( '' )  );
#1159=EDGE_CURVE ( 'NONE', #9081, #16392, #13856, .T. ) ;
#1160=ORIENTED_EDGE ( 'NONE', *, *, #3882, .F. ) ;
#1165=CARTESIAN_POINT ( 'NONE',  ( -124.9459734468149321, 1.025126265847081442, -160.9317124430720014 ) ) ;
#1167=ORIENTED_EDGE ( 'NONE', *, *, #38891, .F. ) ;
#1168=EDGE_LOOP ( 'NONE', ( #24157, #47816, #45794, #1614, #31460, #48514 ) ) ;
#1169=( BOUNDED_CURVE ( )  B_SPLINE_CURVE ( 3, ( #25913, #29750, #33611, #45623 ),
 .UNSPECIFIED., .F., .F. ) 
 B_SPLINE_CURVE_WITH_KNOTS ( ( 4, 4 ),
 ( 3.141592653589793116, 4.712388980384689674 ),
 .UNSPECIFIED. ) 
 CURVE ( )  GEOMETRIC_REPRESENTATION_ITEM ( )  RATIONAL_B_SPLINE_CURVE ( ( 1.000000000000000000, 0.8047378541243649375, 0.8047378541243649375, 1.000000000000000000 ) ) 
 REPRESENTATION_ITEM ( '' )  );
#1170=EDGE_CURVE ( 'NONE', #15638, #28163, #46956, .T. ) ;
#1173=EDGE_CURVE ( 'NONE', #7223, #5437, #15181, .T. ) ;
#1176=ORIENTED_EDGE ( 'NONE', *, *, #32433, .T. ) ;
#1178=EDGE_CURVE ( 'NONE', #36229, #829, #36440, .T. ) ;
#1179=CARTESIAN_POINT ( 'NONE',  ( 210.0000000000000568, 0.000000000000000000, -39.18171244307202983 ) ) ;
#1184=EDGE_LOOP ( 'NONE', ( #33562, #16368, #48239, #12425, #6053, #20848 ) ) ;
#1188=EDGE_CURVE ( 'NONE', #25957, #49918, #41661, .T. ) ;
#1189=VECTOR ( 'NONE', #4370, 1000.000000000000000 ) ;
#1192=AXIS2_PLACEMENT_3D ( 'NONE', #40576, #16973, #37010 ) ;
#1199=CARTESIAN_POINT ( 'NONE',  ( 193.3040265531851105, -1.750000000000009992, 0.8182875569279768335 ) ) ;
#1208=CARTESIAN_POINT ( 'NONE',  ( 153.3040265531850537, 0.000000000000000000, 165.0000000000000000 ) ) ;
#1212=CYLINDRICAL_SURFACE ( 'NONE', #9348, 1.750000000000001554 ) ;
#1217=EDGE_CURVE ( 'NONE', #29584, #33010, #8647, .T. ) ;
#1219=ORIENTED_EDGE ( 'NONE', *, *, #14868, .T. ) ;
#1221=CARTESIAN_POINT ( 'NONE',  ( -126.6959734468149321, 0.000000000000000000, 165.0000000000000000 ) ) ;
#1222=AXIS2_PLACEMENT_3D ( 'NONE', #1095, #37459, #12621 ) ;
#1224=ORIENTED_EDGE ( 'NONE', *, *, #47145, .F. ) ;
#1228=AXIS2_PLACEMENT_3D ( 'NONE', #19135, #50138, #31468 ) ;
#1230=EDGE_CURVE ( 'NONE', #27492, #45408, #11849, .T. ) ;
#1241=EDGE_CURVE ( 'NONE', #44363, #9118, #17083, .T. ) ;
#1243=EDGE_LOOP ( 'NONE', ( #50125, #24001, #26640, #3951, #38835, #44398 ) ) ;
#1244=FACE_OUTER_BOUND ( 'NONE', #11101, .T. ) ;
#1246=DIRECTION ( 'NONE',  ( -1.000000000000000000, -0.000000000000000000, -0.000000000000000000 ) ) ;
#1253=DIRECTION ( 'NONE',  ( -0.000000000000000000, -0.000000000000000000, -1.000000000000000000 ) ) ;
#1257=CARTESIAN_POINT ( 'NONE',  ( 193.3040265531851105, -1.750000000000009992, 160.8182875569279702 ) ) ;
#1258=ORIENTED_EDGE ( 'NONE', *, *, #41775, .T. ) ;
#1263=VECTOR ( 'NONE', #19839, 1000.000000000000000 ) ;
#1265=EDGE_CURVE ( 'NONE', #1473, #46979, #43333, .T. ) ;
#1267=CARTESIAN_POINT ( 'NONE',  ( -126.6959734468149321, 1.749999999999997335, -79.18171244307201562 ) ) ;
#1269=ORIENTED_EDGE ( 'NONE', *, *, #4630, .T. ) ;
#1276=VECTOR ( 'NONE', #31120, 1000.000000000000000 ) ;
#1279=CARTESIAN_POINT ( 'NONE',  ( 73.30402655318508209, 1.750000000000010658, -79.18171244307201562 ) ) ;
#1286=ORIENTED_EDGE ( 'NONE', *, *, #1126, .T. ) ;
#1291=VECTOR ( 'NONE', #33544, 1000.000000000000000 ) ;
#1295=EDGE_CURVE ( 'NONE', #17662, #44875, #38456, .T. ) ;
#1296=CYLINDRICAL_SURFACE ( 'NONE', #33237, 1.750000000000015543 ) ;
#1298=VECTOR ( 'NONE', #22249, 1000.000000000000000 ) ;
#1299=CARTESIAN_POINT ( 'NONE',  ( 210.0000000000000568, 0.000000000000000000, 80.81828755692798438 ) ) ;
#1302=( BOUNDED_CURVE ( )  B_SPLINE_CURVE ( 3, ( #10478, #2526, #13567, #6129 ),
 .UNSPECIFIED., .F., .F. ) 
 B_SPLINE_CURVE_WITH_KNOTS ( ( 4, 4 ),
 ( 3.141592653589793116, 4.712388980384689674 ),
 .UNSPECIFIED. ) 
 CURVE ( )  GEOMETRIC_REPRESENTATION_ITEM ( )  RATIONAL_B_SPLINE_CURVE ( ( 1.000000000000000000, 0.8047378541243649375, 0.8047378541243649375, 1.000000000000000000 ) ) 
 REPRESENTATION_ITEM ( '' )  );
#1307=( BOUNDED_CURVE ( )  B_SPLINE_CURVE ( 3, ( #25709, #38540, #45167, #41355 ),
 .UNSPECIFIED., .F., .F. ) 
 B_SPLINE_CURVE_WITH_KNOTS ( ( 4, 4 ),
 ( 1.570796326794896558, 3.141592653589793116 ),
 .UNSPECIFIED. ) 
 CURVE ( )  GEOMETRIC_REPRESENTATION_ITEM ( )  RATIONAL_B_SPLINE_CURVE ( ( 1.000000000000000000, 0.8047378541243649375, 0.8047378541243649375, 1.000000000000000000 ) ) 
 REPRESENTATION_ITEM ( '' )  );
#1313=CARTESIAN_POINT ( 'NONE',  ( 114.3291528190321173, -1.749999999999996669, -78.15658617722492352 ) ) ;
#1321=( BOUNDED_CURVE ( )  B_SPLINE_CURVE ( 3, ( #15247, #104, #47003, #15738 ),
 .UNSPECIFIED., .F., .F. ) 
 B_SPLINE_CURVE_WITH_KNOTS ( ( 4, 4 ),
 ( 0.000000000000000000, 1.570796326794896558 ),
 .UNSPECIFIED. ) 
 CURVE ( )  GEOMETRIC_REPRESENTATION_ITEM ( )  RATIONAL_B_SPLINE_CURVE ( ( 1.000000000000000000, 0.8047378541243649375, 0.8047378541243649375, 1.000000000000000000 ) ) 
 REPRESENTATION_ITEM ( '' )  );
#1324=CARTESIAN_POINT ( 'NONE',  ( 192.2789002873380184, 1.750000000000009548, -40.20683870891912193 ) ) ;
#1327=CARTESIAN_POINT ( 'NONE',  ( -44.94597344681493922, -1.025126265847089213, -0.9317124430720324924 ) ) ;
#1328=EDGE_LOOP ( 'NONE', ( #49208, #8539, #2407, #30372, #15839 ) ) ;
#1330=ORIENTED_EDGE ( 'NONE', *, *, #36328, .F. ) ;
#1335=AXIS2_PLACEMENT_3D ( 'NONE', #7844, #641, #27597 ) ;
#1339=CARTESIAN_POINT ( 'NONE',  ( -125.6708471809678542, -1.749999999999996669, -0.2068387089191042749 ) ) ;
#1340=DIRECTION ( 'NONE',  ( -1.000000000000000000, 0.000000000000000000, 0.000000000000000000 ) ) ;
#1343=ORIENTED_EDGE ( 'NONE', *, *, #6034, .T. ) ;
#1350=DIRECTION ( 'NONE',  ( -1.000000000000000000, 0.000000000000000000, 0.000000000000000000 ) ) ;
#1352=ORIENTED_EDGE ( 'NONE', *, *, #24699, .T. ) ;
#1355=CARTESIAN_POINT ( 'NONE',  ( 71.55402655318505367, 1.025126265847089213, -160.9317124430720014 ) ) ;
#1364=( BOUNDED_CURVE ( )  B_SPLINE_CURVE ( 3, ( #17997, #5699, #49762, #14661 ),
 .UNSPECIFIED., .F., .F. ) 
 B_SPLINE_CURVE_WITH_KNOTS ( ( 4, 4 ),
 ( 1.570796326794896558, 3.141592653589793116 ),
 .UNSPECIFIED. ) 
 CURVE ( )  GEOMETRIC_REPRESENTATION_ITEM ( )  RATIONAL_B_SPLINE_CURVE ( ( 1.000000000000000000, 0.8047378541243649375, 0.8047378541243649375, 1.000000000000000000 ) ) 
 REPRESENTATION_ITEM ( '' )  );
#1365=AXIS2_PLACEMENT_3D ( 'NONE', #3048, #30262, #37722 ) ;
#1369=EDGE_CURVE ( 'NONE', #19789, #23031, #22321, .T. ) ;
#1372=FACE_OUTER_BOUND ( 'NONE', #38774, .T. ) ;
#1373=ORIENTED_EDGE ( 'NONE', *, *, #32808, .T. ) ;
#1379=CARTESIAN_POINT ( 'NONE',  ( 151.5540265531850537, -1.025126265847089435, 39.06828755692797728 ) ) ;
#1380=DIRECTION ( 'NONE',  ( -0.000000000000000000, -0.000000000000000000, -1.000000000000000000 ) ) ;
#1383=CARTESIAN_POINT ( 'NONE',  ( -48.44597344681495343, 0.000000000000000000, 79.06828755692797017 ) ) ;
#1385=EDGE_CURVE ( 'NONE', #16019, #47057, #49932, .T. ) ;
#1388=EDGE_CURVE ( 'NONE', #559, #40360, #45760, .T. ) ;
#1392=CARTESIAN_POINT ( 'NONE',  ( 71.55402655318505367, 1.025126265847089657, -80.93171244307201562 ) ) ;
#1393=ORIENTED_EDGE ( 'NONE', *, *, #33518, .F. ) ;
#1395=CARTESIAN_POINT ( 'NONE',  ( 210.0000000000000568, 2.143131898507880377E-16, 159.0682875569279702 ) ) ;
#1396=EDGE_CURVE ( 'NONE', #41719, #15554, #13342, .T. ) ;
#1401=( BOUNDED_CURVE ( )  B_SPLINE_CURVE ( 3, ( #35197, #47685, #294, #11834 ),
 .UNSPECIFIED., .F., .F. ) 
 B_SPLINE_CURVE_WITH_KNOTS ( ( 4, 4 ),
 ( 3.141592653589793116, 4.712388980384689674 ),
 .UNSPECIFIED. ) 
 CURVE ( )  GEOMETRIC_REPRESENTATION_ITEM ( )  RATIONAL_B_SPLINE_CURVE ( ( 1.000000000000000000, 0.8047378541243649375, 0.8047378541243649375, 1.000000000000000000 ) ) 
 REPRESENTATION_ITEM ( '' )  );
#1402=DIRECTION ( 'NONE',  ( 1.000000000000000000, 0.000000000000000000, -0.000000000000000000 ) ) ;
#1403=DIRECTION ( 'NONE',  ( -1.000000000000000000, -0.000000000000000000, -0.000000000000000000 ) ) ;
#1410=EDGE_CURVE ( 'NONE', #28349, #13625, #22863, .T. ) ;
#1416=CARTESIAN_POINT ( 'NONE',  ( -126.6959734468149321, 0.000000000000000000, 165.0000000000000000 ) ) ;
#1418=EDGE_LOOP ( 'NONE', ( #24828, #1884, #25493, #14264, #8599, #47070 ) ) ;
#1419=ORIENTED_EDGE ( 'NONE', *, *, #15155, .F. ) ;
#1420=EDGE_CURVE ( 'NONE', #29366, #26020, #29016, .T. ) ;
#1423=DIRECTION ( 'NONE',  ( -1.000000000000000000, 0.000000000000000000, 0.000000000000000000 ) ) ;
#1427=ORIENTED_EDGE ( 'NONE', *, *, #38703, .F. ) ;
#1430=ORIENTED_EDGE ( 'NONE', *, *, #1388, .F. ) ;
#1431=ORIENTED_EDGE ( 'NONE', *, *, #5538, .T. ) ;
#1434=VERTEX_POINT ( 'NONE', #1052 ) ;
#1436=CARTESIAN_POINT ( 'NONE',  ( -86.69597344681494633, -1.750000000000009992, -159.1817124430720298 ) ) ;
#1437=CARTESIAN_POINT ( 'NONE',  ( 155.0540265531850537, 1.025126265847089435, -157.4317124430720582 ) ) ;
#1439=CARTESIAN_POINT ( 'NONE',  ( -44.94597344681493922, 2.143131898507880377E-16, -120.9317124430720725 ) ) ;
#1444=FACE_OUTER_BOUND ( 'NONE', #28602, .T. ) ;
#1446=EDGE_CURVE ( 'NONE', #7572, #36969, #31859, .T. ) ;
#1448=EDGE_CURVE ( 'NONE', #3971, #2131, #35928, .T. ) ;
#1452=CARTESIAN_POINT ( 'NONE',  ( -165.6708471809677974, 1.750000000000009326, 161.8434138227750907 ) ) ;
#1453=DIRECTION ( 'NONE',  ( -0.000000000000000000, -0.000000000000000000, -1.000000000000000000 ) ) ;
#1455=EDGE_LOOP ( 'NONE', ( #11191, #5724, #8614, #8801, #38223, #46999 ) ) ;
#1458=CYLINDRICAL_SURFACE ( 'NONE', #11513, 1.750000000000001554 ) ;
#1459=ORIENTED_EDGE ( 'NONE', *, *, #28494, .T. ) ;
#1460=DIRECTION ( 'NONE',  ( -0.000000000000000000, -0.000000000000000000, -1.000000000000000000 ) ) ;
#1463=( BOUNDED_CURVE ( )  B_SPLINE_CURVE ( 3, ( #9577, #49023, #10340, #2376 ),
 .UNSPECIFIED., .F., .F. ) 
 B_SPLINE_CURVE_WITH_KNOTS ( ( 4, 4 ),
 ( 3.141592653589793116, 4.712388980384689674 ),
 .UNSPECIFIED. ) 
 CURVE ( )  GEOMETRIC_REPRESENTATION_ITEM ( )  RATIONAL_B_SPLINE_CURVE ( ( 1.000000000000000000, 0.8047378541243649375, 0.8047378541243649375, 1.000000000000000000 ) ) 
 REPRESENTATION_ITEM ( '' )  );
#1464=ORIENTED_EDGE ( 'NONE', *, *, #17426, .T. ) ;
#1466=ORIENTED_EDGE ( 'NONE', *, *, #22101, .T. ) ;
#1468=CARTESIAN_POINT ( 'NONE',  ( -166.6959734468149463, -1.750000000000010658, -79.18171244307201562 ) ) ;
#1470=EDGE_CURVE ( 'NONE', #13625, #28349, #28185, .T. ) ;
#1473=VERTEX_POINT ( 'NONE', #36989 ) ;
#1475=AXIS2_PLACEMENT_3D ( 'NONE', #39373, #4210, #35524 ) ;
#1479=CARTESIAN_POINT ( 'NONE',  ( 154.3291528190321458, 1.750000000000009326, 161.8434138227750907 ) ) ;
#1480=FACE_OUTER_BOUND ( 'NONE', #35023, .T. ) ;
#1482=DIRECTION ( 'NONE',  ( -1.000000000000000000, -0.000000000000000000, -0.000000000000000000 ) ) ;
#1485=ORIENTED_EDGE ( 'NONE', *, *, #21891, .T. ) ;
#1486=CARTESIAN_POINT ( 'NONE',  ( -204.9459734468149463, 2.143131898507880377E-16, 122.5682875569279702 ) ) ;
#1487=EDGE_CURVE ( 'NONE', #11190, #14077, #2552, .T. ) ;
#1495=VECTOR ( 'NONE', #17389, 1000.000000000000000 ) ;
#1498=CARTESIAN_POINT ( 'NONE',  ( 31.55402655318503236, 1.025126265847089213, 42.56828755692799149 ) ) ;
#1499=DIRECTION ( 'NONE',  ( -1.000000000000000000, -0.000000000000000000, -0.000000000000000000 ) ) ;
#1500=CARTESIAN_POINT ( 'NONE',  ( -125.6708471809678542, -1.749999999999997113, 119.7931612910809065 ) ) ;
#1501=CARTESIAN_POINT ( 'NONE',  ( -6.695973446814940111, 0.000000000000000000, 165.0000000000000000 ) ) ;
#1502=EDGE_CURVE ( 'NONE', #35123, #48877, #11637, .T. ) ;
#1512=EDGE_CURVE ( 'NONE', #49857, #7014, #14095, .T. ) ;
#1517=CARTESIAN_POINT ( 'NONE',  ( 152.2789002873379900, 1.750000000000009548, -118.1565861772249519 ) ) ;
#1519=EDGE_CURVE ( 'NONE', #25904, #17310, #3074, .T. ) ;
#1521=CARTESIAN_POINT ( 'NONE',  ( -208.4459734468148611, -1.025126265847089879, 122.5682875569280128 ) ) ;
#1523=ORIENTED_EDGE ( 'NONE', *, *, #41886, .T. ) ;
#1527=CARTESIAN_POINT ( 'NONE',  ( -5.670847180967843570, -1.750000000000023981, -80.20683870891910772 ) ) ;
#1529=DIRECTION ( 'NONE',  ( 0.000000000000000000, 0.000000000000000000, -1.000000000000000000 ) ) ;
#1533=CARTESIAN_POINT ( 'NONE',  ( -166.6959734468149463, -1.750000000000009992, 0.8182875569279768335 ) ) ;
#1536=CARTESIAN_POINT ( 'NONE',  ( -210.0000000000000568, 0.000000000000000000, -79.18171244307201562 ) ) ;
#1537=ORIENTED_EDGE ( 'NONE', *, *, #15885, .T. ) ;
#1542=ORIENTED_EDGE ( 'NONE', *, *, #23285, .F. ) ;
#1546=ORIENTED_EDGE ( 'NONE', *, *, #35417, .T. ) ;
#1547=EDGE_CURVE ( 'NONE', #25771, #44889, #44722, .T. ) ;
#1548=CARTESIAN_POINT ( 'NONE',  ( -128.4459734468149179, 0.000000000000000000, 119.0682875569279986 ) ) ;
#1550=CARTESIAN_POINT ( 'NONE',  ( 193.3040265531851105, 0.000000000000000000, 165.0000000000000000 ) ) ;
#1553=DIRECTION ( 'NONE',  ( -0.000000000000000000, -0.000000000000000000, -1.000000000000000000 ) ) ;
#1558=CARTESIAN_POINT ( 'NONE',  ( 113.3040265531850537, -1.749999999999997335, 120.8182875569279702 ) ) ;
#1565=VECTOR ( 'NONE', #13665, 1000.000000000000000 ) ;
#1566=CARTESIAN_POINT ( 'NONE',  ( 195.0540265531851105, 2.143131898507880377E-16, 42.56828755692798438 ) ) ;
#1570=LINE ( 'NONE', #25167, #3304 ) ;
#1572=EDGE_CURVE ( 'NONE', #24608, #2518, #38179, .T. ) ;
#1574=ORIENTED_EDGE ( 'NONE', *, *, #47710, .F. ) ;
#1576=ORIENTED_EDGE ( 'NONE', *, *, #48562, .F. ) ;
#1581=DIRECTION ( 'NONE',  ( -0.000000000000000000, -0.000000000000000000, -1.000000000000000000 ) ) ;
#1582=CARTESIAN_POINT ( 'NONE',  ( 34.32915281903212446, 1.750000000000010214, 79.79316129108087807 ) ) ;
#1584=CARTESIAN_POINT ( 'NONE',  ( -8.445973446814976526, 0.000000000000000000, -77.43171244307198720 ) ) ;
#1586=CYLINDRICAL_SURFACE ( 'NONE', #35227, 1.750000000000015543 ) ;
#1588=FACE_OUTER_BOUND ( 'NONE', #19756, .T. ) ;
#1590=DIRECTION ( 'NONE',  ( -1.000000000000000000, -0.000000000000000000, -0.000000000000000000 ) ) ;
#1591=EDGE_LOOP ( 'NONE', ( #7982, #46133, #48902, #23547, #10690, #1872 ) ) ;
#1592=ORIENTED_EDGE ( 'NONE', *, *, #5961, .F. ) ;
#1594=( BOUNDED_CURVE ( )  B_SPLINE_CURVE ( 3, ( #48627, #41480, #48878, #13516 ),
 .UNSPECIFIED., .F., .F. ) 
 B_SPLINE_CURVE_WITH_KNOTS ( ( 4, 4 ),
 ( 3.141592653589793116, 4.712388980384689674 ),
 .UNSPECIFIED. ) 
 CURVE ( )  GEOMETRIC_REPRESENTATION_ITEM ( )  RATIONAL_B_SPLINE_CURVE ( ( 1.000000000000000000, 0.8047378541243649375, 0.8047378541243649375, 1.000000000000000000 ) ) 
 REPRESENTATION_ITEM ( '' )  );
#1595=AXIS2_PLACEMENT_3D ( 'NONE', #29390, #45260, #29643 ) ;
#1596=ORIENTED_EDGE ( 'NONE', *, *, #17680, .T. ) ;
#1603=( BOUNDED_CURVE ( )  B_SPLINE_CURVE ( 3, ( #5591, #14040, #45324, #13543 ),
 .UNSPECIFIED., .F., .F. ) 
 B_SPLINE_CURVE_WITH_KNOTS ( ( 4, 4 ),
 ( 4.712388980384689674, 6.283185307179586232 ),
 .UNSPECIFIED. ) 
 CURVE ( )  GEOMETRIC_REPRESENTATION_ITEM ( )  RATIONAL_B_SPLINE_CURVE ( ( 1.000000000000000000, 0.8047378541243649375, 0.8047378541243649375, 1.000000000000000000 ) ) 
 REPRESENTATION_ITEM ( '' )  );
#1607=EDGE_CURVE ( 'NONE', #31600, #29622, #248, .T. ) ;
#1610=AXIS2_PLACEMENT_3D ( 'NONE', #47849, #48853, #16594 ) ;
#1611=CYLINDRICAL_SURFACE ( 'NONE', #46841, 1.750000000000015543 ) ;
#1614=ORIENTED_EDGE ( 'NONE', *, *, #14576, .T. ) ;
#1618=( BOUNDED_CURVE ( )  B_SPLINE_CURVE ( 3, ( #30631, #42408, #38595, #3414 ),
 .UNSPECIFIED., .F., .F. ) 
 B_SPLINE_CURVE_WITH_KNOTS ( ( 4, 4 ),
 ( 3.141592653589793116, 4.712388980384689674 ),
 .UNSPECIFIED. ) 
 CURVE ( )  GEOMETRIC_REPRESENTATION_ITEM ( )  RATIONAL_B_SPLINE_CURVE ( ( 1.000000000000000000, 0.8047378541243649375, 0.8047378541243649375, 1.000000000000000000 ) ) 
 REPRESENTATION_ITEM ( '' )  );
#1620=ORIENTED_EDGE ( 'NONE', *, *, #34416, .F. ) ;
#1625=DIRECTION ( 'NONE',  ( 0.000000000000000000, 0.000000000000000000, 1.000000000000000000 ) ) ;
#1627=CARTESIAN_POINT ( 'NONE',  ( 210.0000000000000568, 0.000000000000000000, -77.43171244307200141 ) ) ;
#1629=ORIENTED_EDGE ( 'NONE', *, *, #19967, .T. ) ;
#1631=CARTESIAN_POINT ( 'NONE',  ( -44.94597344681493922, 2.143131898507880377E-16, 165.0000000000000000 ) ) ;
#1632=DIRECTION ( 'NONE',  ( -0.000000000000000000, -0.000000000000000000, -1.000000000000000000 ) ) ;
#1635=VECTOR ( 'NONE', #46203, 1000.000000000000000 ) ;
#1636=CARTESIAN_POINT ( 'NONE',  ( -46.69597344681494633, 0.000000000000000000, 165.0000000000000000 ) ) ;
#1637=ORIENTED_EDGE ( 'NONE', *, *, #40941, .F. ) ;
#1641=AXIS2_PLACEMENT_3D ( 'NONE', #31335, #27725, #27222 ) ;
#1650=DIRECTION ( 'NONE',  ( 0.000000000000000000, 0.000000000000000000, 1.000000000000000000 ) ) ;
#1651=ORIENTED_EDGE ( 'NONE', *, *, #23469, .T. ) ;
#1652=ORIENTED_EDGE ( 'NONE', *, *, #46034, .F. ) ;
#1656=ORIENTED_EDGE ( 'NONE', *, *, #833, .F. ) ;
#1657=CARTESIAN_POINT ( 'NONE',  ( -86.69597344681496054, 0.000000000000000000, 165.0000000000000000 ) ) ;
#1666=VECTOR ( 'NONE', #34213, 1000.000000000000000 ) ;
#1667=EDGE_CURVE ( 'NONE', #10095, #32209, #7435, .T. ) ;
#1672=CARTESIAN_POINT ( 'NONE',  ( 35.05402655318504657, -1.025126265847089213, -0.9317124430720324924 ) ) ;
#1674=CARTESIAN_POINT ( 'NONE',  ( 210.0000000000000568, 0.000000000000000000, 42.56828755692799149 ) ) ;
#1678=CARTESIAN_POINT ( 'NONE',  ( -128.4459734468149179, 0.000000000000000000, 82.56828755692795596 ) ) ;
#1679=ORIENTED_EDGE ( 'NONE', *, *, #13074, .F. ) ;
#1681=DIRECTION ( 'NONE',  ( -1.000000000000000000, 0.000000000000000000, 0.000000000000000000 ) ) ;
#1682=CARTESIAN_POINT ( 'NONE',  ( -206.6959734468149463, 1.750000000000010214, 40.81828755692798438 ) ) ;
#1684=CARTESIAN_POINT ( 'NONE',  ( 152.2789002873379900, -1.750000000000009548, 1.843413822775065825 ) ) ;
#1687=FACE_OUTER_BOUND ( 'NONE', #16486, .T. ) ;
#1693=CARTESIAN_POINT ( 'NONE',  ( 151.5540265531850537, 0.000000000000000000, 82.56828755692798438 ) ) ;
#1695=CYLINDRICAL_SURFACE ( 'NONE', #26203, 1.750000000000001554 ) ;
#1699=EDGE_LOOP ( 'NONE', ( #15444, #5119, #18178, #21063, #5514, #12297 ) ) ;
#1704=CYLINDRICAL_SURFACE ( 'NONE', #1610, 1.750000000000008438 ) ;
#1706=CARTESIAN_POINT ( 'NONE',  ( 31.55402655318503236, 1.025126265847089435, 39.06828755692797728 ) ) ;
#1713=CARTESIAN_POINT ( 'NONE',  ( -166.6959734468149463, -1.750000000000010658, 120.8182875569279702 ) ) ;
#1714=ORIENTED_EDGE ( 'NONE', *, *, #45469, .F. ) ;
#1715=CYLINDRICAL_SURFACE ( 'NONE', #30337, 1.750000000000001554 ) ;
#1720=EDGE_CURVE ( 'NONE', #12850, #13383, #4738, .T. ) ;
#1726=EDGE_CURVE ( 'NONE', #13717, #19110, #49961, .T. ) ;
#1727=CARTESIAN_POINT ( 'NONE',  ( 115.0540265531850395, 2.143131898507847836E-16, 79.06828755692798438 ) ) ;
#1735=DIRECTION ( 'NONE',  ( -1.000000000000000000, -0.000000000000000000, -0.000000000000000000 ) ) ;
#1736=ORIENTED_EDGE ( 'NONE', *, *, #9293, .T. ) ;
#1738=CARTESIAN_POINT ( 'NONE',  ( -88.44597344681494633, -1.025126265847089657, -120.9317124430720440 ) ) ;
#1739=LINE ( 'NONE', #41487, #7585 ) ;
#1741=CARTESIAN_POINT ( 'NONE',  ( -205.6708471809678827, -1.750000000000010436, -120.2068387089191219 ) ) ;
#1744=DIRECTION ( 'NONE',  ( 0.000000000000000000, 0.000000000000000000, 1.000000000000000000 ) ) ;
#1745=CYLINDRICAL_SURFACE ( 'NONE', #44480, 1.750000000000015543 ) ;
#1754=( BOUNDED_CURVE ( )  B_SPLINE_CURVE ( 3, ( #9067, #31680, #620, #16014 ),
 .UNSPECIFIED., .F., .F. ) 
 B_SPLINE_CURVE_WITH_KNOTS ( ( 4, 4 ),
 ( 3.141592653589793116, 4.712388980384689674 ),
 .UNSPECIFIED. ) 
 CURVE ( )  GEOMETRIC_REPRESENTATION_ITEM ( )  RATIONAL_B_SPLINE_CURVE ( ( 1.000000000000000000, 0.8047378541243649375, 0.8047378541243649375, 1.000000000000000000 ) ) 
 REPRESENTATION_ITEM ( '' )  );
#1763=DIRECTION ( 'NONE',  ( -1.000000000000000000, 0.000000000000000000, 0.000000000000000000 ) ) ;
#1764=EDGE_CURVE ( 'NONE', #43746, #42197, #37215, .T. ) ;
#1765=CARTESIAN_POINT ( 'NONE',  ( -45.67084718096785423, -1.750000000000009548, -40.20683870891912193 ) ) ;
#1767=ORIENTED_EDGE ( 'NONE', *, *, #19317, .F. ) ;
#1768=DIRECTION ( 'NONE',  ( 0.000000000000000000, 0.000000000000000000, 1.000000000000000000 ) ) ;
#1773=DIRECTION ( 'NONE',  ( 0.000000000000000000, 0.000000000000000000, 1.000000000000000000 ) ) ;
#1786=ADVANCED_FACE ( 'NONE', ( #24847 ), #20480, .T. ) ;
#1793=CARTESIAN_POINT ( 'NONE',  ( -46.69597344681494633, 1.750000000000010214, 40.81828755692798438 ) ) ;
#1798=ADVANCED_FACE ( 'NONE', ( #32050 ), #48395, .T. ) ;
#1801=CARTESIAN_POINT ( 'NONE',  ( -6.695973446814940111, -1.750000000000024203, -79.18171244307201562 ) ) ;
#1803=VECTOR ( 'NONE', #28805, 1000.000000000000000 ) ;
#1806=ORIENTED_EDGE ( 'NONE', *, *, #46982, .T. ) ;
#1810=CARTESIAN_POINT ( 'NONE',  ( 210.0000000000000568, 0.000000000000000000, -39.18171244307202983 ) ) ;
#1814=CYLINDRICAL_SURFACE ( 'NONE', #15023, 1.750000000000001554 ) ;
#1816=CARTESIAN_POINT ( 'NONE',  ( 111.5540265531850679, 0.000000000000000000, -80.93171244307201562 ) ) ;
#1819=CYLINDRICAL_SURFACE ( 'NONE', #30724, 1.750000000000015543 ) ;
#1821=ORIENTED_EDGE ( 'NONE', *, *, #4553, .F. ) ;
#1825=ORIENTED_EDGE ( 'NONE', *, *, #41293, .T. ) ;
#1827=PLANE ( 'NONE',  #9378 ) ;
#1835=FACE_OUTER_BOUND ( 'NONE', #10491, .T. ) ;
#1838=VECTOR ( 'NONE', #35519, 1000.000000000000000 ) ;
#1846=EDGE_CURVE ( 'NONE', #34157, #42077, #39752, .T. ) ;
#1849=CYLINDRICAL_SURFACE ( 'NONE', #5146, 1.750000000000001554 ) ;
#1850=EDGE_LOOP ( 'NONE', ( #41128, #43176, #714, #3952, #8728 ) ) ;
#1852=EDGE_CURVE ( 'NONE', #22517, #47093, #8348, .T. ) ;
#1854=ORIENTED_EDGE ( 'NONE', *, *, #32860, .T. ) ;
#1856=CARTESIAN_POINT ( 'NONE',  ( -168.4459734468149463, 0.000000000000000000, 42.56828755692798438 ) ) ;
#1857=EDGE_CURVE ( 'NONE', #12663, #29500, #44070, .T. ) ;
#1859=EDGE_CURVE ( 'NONE', #29900, #14767, #13571, .T. ) ;
#1860=CARTESIAN_POINT ( 'NONE',  ( 75.05402655318509630, 2.143131898507880377E-16, -157.4317124430720014 ) ) ;
#1862=EDGE_LOOP ( 'NONE', ( #10679, #24004, #17988, #47529, #29113, #6209 ) ) ;
#1863=PLANE ( 'NONE',  #11373 ) ;
#1865=EDGE_CURVE ( 'NONE', #12549, #9233, #37577, .T. ) ;
#1868=VECTOR ( 'NONE', #24949, 1000.000000000000000 ) ;
#1869=FACE_OUTER_BOUND ( 'NONE', #41521, .T. ) ;
#1870=ORIENTED_EDGE ( 'NONE', *, *, #39322, .T. ) ;
#1872=ORIENTED_EDGE ( 'NONE', *, *, #3267, .F. ) ;
#1873=CARTESIAN_POINT ( 'NONE',  ( 210.0000000000000568, 0.000000000000000000, 40.81828755692798438 ) ) ;
#1875=CARTESIAN_POINT ( 'NONE',  ( 153.3040265531850537, -1.750000000000010214, 40.81828755692798438 ) ) ;
#1877=CARTESIAN_POINT ( 'NONE',  ( -4.945973446814916130, -1.025126265847097207, -117.4317124430720014 ) ) ;
#1881=DIRECTION ( 'NONE',  ( -1.000000000000000000, -0.000000000000000000, -0.000000000000000000 ) ) ;
#1882=CARTESIAN_POINT ( 'NONE',  ( -44.94597344681493922, 2.143131898507880377E-16, 165.0000000000000000 ) ) ;
#1884=ORIENTED_EDGE ( 'NONE', *, *, #43377, .T. ) ;
#1886=CYLINDRICAL_SURFACE ( 'NONE', #26163, 1.750000000000008438 ) ;
#1890=CARTESIAN_POINT ( 'NONE',  ( 113.3040265531850537, 1.749999999999997335, 120.8182875569279702 ) ) ;
#1893=ORIENTED_EDGE ( 'NONE', *, *, #9050, .T. ) ;
#1894=( BOUNDED_CURVE ( )  B_SPLINE_CURVE ( 3, ( #41568, #34150, #37741, #30036 ),
 .UNSPECIFIED., .F., .F. ) 
 B_SPLINE_CURVE_WITH_KNOTS ( ( 4, 4 ),
 ( 3.141592653589793116, 4.712388980384689674 ),
 .UNSPECIFIED. ) 
 CURVE ( )  GEOMETRIC_REPRESENTATION_ITEM ( )  RATIONAL_B_SPLINE_CURVE ( ( 1.000000000000000000, 0.8047378541243649375, 0.8047378541243649375, 1.000000000000000000 ) ) 
 REPRESENTATION_ITEM ( '' )  );
#1896=DIRECTION ( 'NONE',  ( -1.000000000000000000, -0.000000000000000000, -0.000000000000000000 ) ) ;
#1897=CARTESIAN_POINT ( 'NONE',  ( 191.5540265531851105, 0.000000000000000000, 122.5682875569279702 ) ) ;
#1898=CYLINDRICAL_SURFACE ( 'NONE', #47107, 1.750000000000015543 ) ;
#1899=( BOUNDED_CURVE ( )  B_SPLINE_CURVE ( 3, ( #48724, #49230, #21568, #2085 ),
 .UNSPECIFIED., .F., .F. ) 
 B_SPLINE_CURVE_WITH_KNOTS ( ( 4, 4 ),
 ( 1.570796326794896558, 3.141592653589793116 ),
 .UNSPECIFIED. ) 
 CURVE ( )  GEOMETRIC_REPRESENTATION_ITEM ( )  RATIONAL_B_SPLINE_CURVE ( ( 1.000000000000000000, 0.8047378541243649375, 0.8047378541243649375, 1.000000000000000000 ) ) 
 REPRESENTATION_ITEM ( '' )  );
#1901=ORIENTED_EDGE ( 'NONE', *, *, #25875, .F. ) ;
#1904=VERTEX_POINT ( 'NONE', #5846 ) ;
#1909=AXIS2_PLACEMENT_3D ( 'NONE', #12057, #9, #266 ) ;
#1910=CARTESIAN_POINT ( 'NONE',  ( 195.0540265531851105, 2.143131898507880377E-16, 165.0000000000000000 ) ) ;
#1911=ORIENTED_EDGE ( 'NONE', *, *, #42272, .T. ) ;
#1913=AXIS2_PLACEMENT_3D ( 'NONE', #28622, #40183, #13223 ) ;
#1914=VERTEX_POINT ( 'NONE', #29443 ) ;
#1915=( BOUNDED_CURVE ( )  B_SPLINE_CURVE ( 3, ( #26416, #22314, #37990, #2808 ),
 .UNSPECIFIED., .F., .F. ) 
 B_SPLINE_CURVE_WITH_KNOTS ( ( 4, 4 ),
 ( 4.712388980384689674, 6.283185307179586232 ),
 .UNSPECIFIED. ) 
 CURVE ( )  GEOMETRIC_REPRESENTATION_ITEM ( )  RATIONAL_B_SPLINE_CURVE ( ( 1.000000000000000000, 0.8047378541243649375, 0.8047378541243649375, 1.000000000000000000 ) ) 
 REPRESENTATION_ITEM ( '' )  );
#1919=AXIS2_PLACEMENT_3D ( 'NONE', #37490, #44623, #28758 ) ;
#1921=ORIENTED_EDGE ( 'NONE', *, *, #20459, .T. ) ;
#1924=CARTESIAN_POINT ( 'NONE',  ( 191.5540265531850537, -1.025126265847089213, -0.9317124430720324924 ) ) ;
#1926=ORIENTED_EDGE ( 'NONE', *, *, #34329, .T. ) ;
#1931=DIRECTION ( 'NONE',  ( -1.000000000000000000, 0.000000000000000000, 0.000000000000000000 ) ) ;
#1943=VECTOR ( 'NONE', #24188, 1000.000000000000000 ) ;
#1946=FACE_OUTER_BOUND ( 'NONE', #38863, .T. ) ;
#1947=DIRECTION ( 'NONE',  ( -1.000000000000000000, 0.000000000000000000, 0.000000000000000000 ) ) ;
#1948=AXIS2_PLACEMENT_3D ( 'NONE', #12120, #40325, #32122 ) ;
#1950=ORIENTED_EDGE ( 'NONE', *, *, #18975, .T. ) ;
#1951=CYLINDRICAL_SURFACE ( 'NONE', #46917, 1.750000000000001554 ) ;
#1955=DIRECTION ( 'NONE',  ( -0.000000000000000000, -0.000000000000000000, -1.000000000000000000 ) ) ;
#1962=ORIENTED_EDGE ( 'NONE', *, *, #5488, .T. ) ;
#1967=CARTESIAN_POINT ( 'NONE',  ( 210.0000000000000568, 2.143131898507881116E-16, -40.93171244307203693 ) ) ;
#1973=CARTESIAN_POINT ( 'NONE',  ( 33.30402655318503946, 1.750000000000010658, 120.8182875569279702 ) ) ;
#1977=ORIENTED_EDGE ( 'NONE', *, *, #7701, .T. ) ;
#1980=VECTOR ( 'NONE', #46135, 1000.000000000000000 ) ;
#1984=CARTESIAN_POINT ( 'NONE',  ( 210.0000000000000568, 2.143131898507881856E-16, 79.06828755692797017 ) ) ;
#1992=DIRECTION ( 'NONE',  ( -0.000000000000000000, -0.000000000000000000, -1.000000000000000000 ) ) ;
#1993=FACE_OUTER_BOUND ( 'NONE', #14346, .T. ) ;
#1994=ADVANCED_FACE ( 'NONE', ( #23255 ), #26608, .T. ) ;
#1996=ADVANCED_FACE ( 'NONE', ( #30458 ), #10695, .T. ) ;
#1997=CARTESIAN_POINT ( 'NONE',  ( 112.2789002873379758, 1.749999999999996225, -158.1565861772249377 ) ) ;
#2001=DIRECTION ( 'NONE',  ( -1.000000000000000000, -0.000000000000000000, -0.000000000000000000 ) ) ;
#2002=EDGE_CURVE ( 'NONE', #37195, #28486, #15058, .T. ) ;
#2003=ADVANCED_FACE ( 'NONE', ( #30721 ), #22499, .T. ) ;
#2006=ORIENTED_EDGE ( 'NONE', *, *, #12062, .T. ) ;
#2007=CARTESIAN_POINT ( 'NONE',  ( -86.69597344681494633, 1.750000000000010658, -119.1817124430720440 ) ) ;
#2008=EDGE_CURVE ( 'NONE', #36250, #23942, #18637, .T. ) ;
#2012=CYLINDRICAL_SURFACE ( 'NONE', #25510, 1.750000000000001554 ) ;
#2013=ADVANCED_FACE ( 'NONE', ( #42003 ), #22754, .T. ) ;
#2016=CARTESIAN_POINT ( 'NONE',  ( 151.5540265531850537, 0.000000000000000000, -117.4317124430720725 ) ) ;
#2020=CARTESIAN_POINT ( 'NONE',  ( 75.05402655318509630, 2.143131898507880377E-16, -117.4317124430720156 ) ) ;
#2022=VERTEX_POINT ( 'NONE', #50418 ) ;
#2024=ORIENTED_EDGE ( 'NONE', *, *, #18436, .T. ) ;
#2028=CYLINDRICAL_SURFACE ( 'NONE', #21636, 1.749999999999987566 ) ;
#2030=EDGE_CURVE ( 'NONE', #19110, #1049, #17178, .T. ) ;
#2036=EDGE_CURVE ( 'NONE', #34157, #44875, #35350, .T. ) ;
#2039=VERTEX_POINT ( 'NONE', #35599 ) ;
#2042=VERTEX_POINT ( 'NONE', #31993 ) ;
#2050=FACE_OUTER_BOUND ( 'NONE', #45912, .T. ) ;
#2052=AXIS2_PLACEMENT_3D ( 'NONE', #21375, #33699, #25745 ) ;
#2054=FACE_OUTER_BOUND ( 'NONE', #36715, .T. ) ;
#2055=( BOUNDED_CURVE ( )  B_SPLINE_CURVE ( 3, ( #37071, #21383, #17037, #25753 ),
 .UNSPECIFIED., .F., .F. ) 
 B_SPLINE_CURVE_WITH_KNOTS ( ( 4, 4 ),
 ( 3.141592653589793116, 4.712388980384689674 ),
 .UNSPECIFIED. ) 
 CURVE ( )  GEOMETRIC_REPRESENTATION_ITEM ( )  RATIONAL_B_SPLINE_CURVE ( ( 1.000000000000000000, 0.8047378541243649375, 0.8047378541243649375, 1.000000000000000000 ) ) 
 REPRESENTATION_ITEM ( '' )  );
#2060=CARTESIAN_POINT ( 'NONE',  ( 72.27890028733797578, 1.750000000000009548, -78.15658617722490931 ) ) ;
#2064=FACE_OUTER_BOUND ( 'NONE', #10931, .T. ) ;
#2066=CARTESIAN_POINT ( 'NONE',  ( -8.445973446814964092, 1.025126265847097207, 122.5682875569280128 ) ) ;
#2071=EDGE_CURVE ( 'NONE', #43863, #40138, #23778, .T. ) ;
#2072=ORIENTED_EDGE ( 'NONE', *, *, #5771, .T. ) ;
#2077=CYLINDRICAL_SURFACE ( 'NONE', #20479, 1.750000000000010214 ) ;
#2082=CARTESIAN_POINT ( 'NONE',  ( 210.0000000000000568, 2.143131898507881856E-16, -80.93171244307202983 ) ) ;
#2083=EDGE_CURVE ( 'NONE', #11343, #22517, #18803, .T. ) ;
#2085=CARTESIAN_POINT ( 'NONE',  ( -164.9459734468149747, 0.000000000000000000, 162.5682875569279702 ) ) ;
#2089=ORIENTED_EDGE ( 'NONE', *, *, #43773, .T. ) ;
#2093=CARTESIAN_POINT ( 'NONE',  ( 115.0540265531850395, 1.025126265847081664, -157.4317124430720582 ) ) ;
#2095=CARTESIAN_POINT ( 'NONE',  ( -46.69597344681494633, 0.000000000000000000, 165.0000000000000000 ) ) ;
#2098=CARTESIAN_POINT ( 'NONE',  ( 191.5540265531850537, 1.025126265847089213, 159.0682875569279418 ) ) ;
#2100=ORIENTED_EDGE ( 'NONE', *, *, #4279, .T. ) ;
#2101=EDGE_CURVE ( 'NONE', #9119, #32429, #27886, .T. ) ;
#2102=DIRECTION ( 'NONE',  ( -0.000000000000000000, -0.000000000000000000, -1.000000000000000000 ) ) ;
#2104=ORIENTED_EDGE ( 'NONE', *, *, #2924, .F. ) ;
#2113=ORIENTED_EDGE ( 'NONE', *, *, #11138, .T. ) ;
#2119=DIRECTION ( 'NONE',  ( -1.000000000000000000, 0.000000000000000000, 0.000000000000000000 ) ) ;
#2121=CARTESIAN_POINT ( 'NONE',  ( -46.69597344681494633, 1.750000000000010658, -79.18171244307201562 ) ) ;
#2126=FACE_OUTER_BOUND ( 'NONE', #28340, .T. ) ;
#2129=CARTESIAN_POINT ( 'NONE',  ( -4.945973446814903696, 2.143131898507912917E-16, -117.4317124430720156 ) ) ;
#2130=CARTESIAN_POINT ( 'NONE',  ( -45.67084718096785423, 1.750000000000010214, -120.2068387089191219 ) ) ;
#2131=VERTEX_POINT ( 'NONE', #8637 ) ;
#2140=( BOUNDED_CURVE ( )  B_SPLINE_CURVE ( 3, ( #33015, #47850, #44517, #12741 ),
 .UNSPECIFIED., .F., .F. ) 
 B_SPLINE_CURVE_WITH_KNOTS ( ( 4, 4 ),
 ( 1.570796326794896558, 3.141592653589793116 ),
 .UNSPECIFIED. ) 
 CURVE ( )  GEOMETRIC_REPRESENTATION_ITEM ( )  RATIONAL_B_SPLINE_CURVE ( ( 1.000000000000000000, 0.8047378541243649375, 0.8047378541243649375, 1.000000000000000000 ) ) 
 REPRESENTATION_ITEM ( '' )  );
#2143=CARTESIAN_POINT ( 'NONE',  ( 72.27890028733797578, -1.750000000000010214, -78.15658617722490931 ) ) ;
#2148=ADVANCED_FACE ( 'NONE', ( #22919 ), #46235, .T. ) ;
#2153=AXIS2_PLACEMENT_3D ( 'NONE', #23373, #24400, #27731 ) ;
#2155=CARTESIAN_POINT ( 'NONE',  ( -6.695973446814940111, -1.750000000000023315, 0.8182875569279768335 ) ) ;
#2164=CARTESIAN_POINT ( 'NONE',  ( 155.0540265531850537, 2.143131898507880377E-16, -77.43171244307204404 ) ) ;
#2166=CARTESIAN_POINT ( 'NONE',  ( 34.32915281903212446, -1.750000000000009548, -78.15658617722490931 ) ) ;
#2169=ORIENTED_EDGE ( 'NONE', *, *, #17078, .F. ) ;
#2170=ORIENTED_EDGE ( 'NONE', *, *, #41182, .T. ) ;
#2171=CIRCLE ( 'NONE', #12823, 1.750000000000015543 ) ;
#2174=ORIENTED_EDGE ( 'NONE', *, *, #25665, .F. ) ;
#2177=LINE ( 'NONE', #10380, #18316 ) ;
#2182=DIRECTION ( 'NONE',  ( -1.000000000000000000, -0.000000000000000000, -0.000000000000000000 ) ) ;
#2184=CARTESIAN_POINT ( 'NONE',  ( -48.44597344681496054, -1.025126265847089879, -77.43171244307200141 ) ) ;
#2191=CARTESIAN_POINT ( 'NONE',  ( -204.9459734468149463, 2.143131898507880377E-16, 165.0000000000000000 ) ) ;
#2193=FACE_OUTER_BOUND ( 'NONE', #40521, .T. ) ;
#2195=( BOUNDED_CURVE ( )  B_SPLINE_CURVE ( 3, ( #16084, #47336, #19672, #35358 ),
 .UNSPECIFIED., .F., .F. ) 
 B_SPLINE_CURVE_WITH_KNOTS ( ( 4, 4 ),
 ( 0.000000000000000000, 1.570796326794896558 ),
 .UNSPECIFIED. ) 
 CURVE ( )  GEOMETRIC_REPRESENTATION_ITEM ( )  RATIONAL_B_SPLINE_CURVE ( ( 1.000000000000000000, 0.8047378541243649375, 0.8047378541243649375, 1.000000000000000000 ) ) 
 REPRESENTATION_ITEM ( '' )  );
#2197=CARTESIAN_POINT ( 'NONE',  ( 72.27890028733797578, -1.750000000000010214, 121.8434138227750623 ) ) ;
#2200=( BOUNDED_CURVE ( )  B_SPLINE_CURVE ( 3, ( #18719, #41836, #11041, #45146 ),
 .UNSPECIFIED., .F., .F. ) 
 B_SPLINE_CURVE_WITH_KNOTS ( ( 4, 4 ),
 ( 1.570796326794896558, 3.141592653589793116 ),
 .UNSPECIFIED. ) 
 CURVE ( )  GEOMETRIC_REPRESENTATION_ITEM ( )  RATIONAL_B_SPLINE_CURVE ( ( 1.000000000000000000, 0.8047378541243649375, 0.8047378541243649375, 1.000000000000000000 ) ) 
 REPRESENTATION_ITEM ( '' )  );
#2207=CARTESIAN_POINT ( 'NONE',  ( 210.0000000000000568, 0.000000000000000000, 122.5682875569279844 ) ) ;
#2215=AXIS2_PLACEMENT_3D ( 'NONE', #38167, #22491, #25842 ) ;
#2218=DIRECTION ( 'NONE',  ( 0.000000000000000000, 0.000000000000000000, 1.000000000000000000 ) ) ;
#2222=CARTESIAN_POINT ( 'NONE',  ( 193.3040265531851105, -1.750000000000010658, 120.8182875569279702 ) ) ;
#2230=CARTESIAN_POINT ( 'NONE',  ( 112.2789002873379758, -1.749999999999996669, 159.7931612910809065 ) ) ;
#2232=CARTESIAN_POINT ( 'NONE',  ( -204.9459734468149463, 2.143131898507880377E-16, -160.9317124430720014 ) ) ;
#2235=CARTESIAN_POINT ( 'NONE',  ( 111.5540265531850537, -1.025126265847082108, 42.56828755692797017 ) ) ;
#2242=CARTESIAN_POINT ( 'NONE',  ( -166.6959734468149463, -1.750000000000009992, -159.1817124430720298 ) ) ;
#2246=ORIENTED_EDGE ( 'NONE', *, *, #40382, .T. ) ;
#2247=DIRECTION ( 'NONE',  ( -0.000000000000000000, -0.000000000000000000, -1.000000000000000000 ) ) ;
#2249=CARTESIAN_POINT ( 'NONE',  ( -86.69597344681494633, 1.750000000000009992, -159.1817124430720298 ) ) ;
#2254=DIRECTION ( 'NONE',  ( -1.000000000000000000, -0.000000000000000000, -0.000000000000000000 ) ) ;
#2255=DIRECTION ( 'NONE',  ( -0.000000000000000000, -0.000000000000000000, -1.000000000000000000 ) ) ;
#2258=DIRECTION ( 'NONE',  ( -1.000000000000000000, -0.000000000000000000, -0.000000000000000000 ) ) ;
#2259=VERTEX_POINT ( 'NONE', #19062 ) ;
#2260=FACE_OUTER_BOUND ( 'NONE', #4386, .T. ) ;
#2262=ORIENTED_EDGE ( 'NONE', *, *, #42212, .T. ) ;
#2263=ORIENTED_EDGE ( 'NONE', *, *, #26257, .F. ) ;
#2265=ORIENTED_EDGE ( 'NONE', *, *, #48091, .T. ) ;
#2266=CARTESIAN_POINT ( 'NONE',  ( -128.4459734468149179, 0.000000000000000000, 39.06828755692801280 ) ) ;
#2267=CYLINDRICAL_SURFACE ( 'NONE', #3574, 1.750000000000001554 ) ;
#2271=CARTESIAN_POINT ( 'NONE',  ( -166.6959734468149463, 1.750000000000010658, 80.81828755692798438 ) ) ;
#2273=ORIENTED_EDGE ( 'NONE', *, *, #32773, .F. ) ;
#2280=LINE ( 'NONE', #48431, #50475 ) ;
#2290=CARTESIAN_POINT ( 'NONE',  ( -166.6959734468149463, 0.000000000000000000, 165.0000000000000000 ) ) ;
#2291=CYLINDRICAL_SURFACE ( 'NONE', #32009, 1.750000000000036193 ) ;
#2293=ADVANCED_FACE ( 'NONE', ( #48232 ), #25439, .T. ) ;
#2294=EDGE_CURVE ( 'NONE', #19943, #37516, #21076, .T. ) ;
#2296=DIRECTION ( 'NONE',  ( -1.000000000000000000, -0.000000000000000000, -0.000000000000000000 ) ) ;
#2297=CARTESIAN_POINT ( 'NONE',  ( -164.9459734468149463, 2.143131898507880377E-16, 165.0000000000000000 ) ) ;
#2305=ORIENTED_EDGE ( 'NONE', *, *, #1512, .F. ) ;
#2310=EDGE_CURVE ( 'NONE', #49578, #37522, #40337, .T. ) ;
#2314=LINE ( 'NONE', #17954, #23145 ) ;
#2317=ADVANCED_FACE ( 'NONE', ( #37271 ), #33159, .T. ) ;
#2318=CARTESIAN_POINT ( 'NONE',  ( 210.0000000000000568, 0.000000000000000000, 0.8182875569279768335 ) ) ;
#2320=DIRECTION ( 'NONE',  ( 1.000000000000000000, 0.000000000000000000, 0.000000000000000000 ) ) ;
#2321=EDGE_CURVE ( 'NONE', #13085, #5639, #43096, .T. ) ;
#2326=( BOUNDED_CURVE ( )  B_SPLINE_CURVE ( 3, ( #7322, #10911, #26567, #34798 ),
 .UNSPECIFIED., .F., .F. ) 
 B_SPLINE_CURVE_WITH_KNOTS ( ( 4, 4 ),
 ( 0.000000000000000000, 1.570796326794896558 ),
 .UNSPECIFIED. ) 
 CURVE ( )  GEOMETRIC_REPRESENTATION_ITEM ( )  RATIONAL_B_SPLINE_CURVE ( ( 1.000000000000000000, 0.8047378541243649375, 0.8047378541243649375, 1.000000000000000000 ) ) 
 REPRESENTATION_ITEM ( '' )  );
#2331=CARTESIAN_POINT ( 'NONE',  ( 113.3040265531850537, 1.749999999999996891, -159.1817124430720298 ) ) ;
#2338=ORIENTED_EDGE ( 'NONE', *, *, #25664, .F. ) ;
#2343=( BOUNDED_CURVE ( )  B_SPLINE_CURVE ( 3, ( #23743, #20137, #35827, #12436 ),
 .UNSPECIFIED., .F., .F. ) 
 B_SPLINE_CURVE_WITH_KNOTS ( ( 4, 4 ),
 ( 3.141592653589793116, 4.712388980384689674 ),
 .UNSPECIFIED. ) 
 CURVE ( )  GEOMETRIC_REPRESENTATION_ITEM ( )  RATIONAL_B_SPLINE_CURVE ( ( 1.000000000000000000, 0.8047378541243649375, 0.8047378541243649375, 1.000000000000000000 ) ) 
 REPRESENTATION_ITEM ( '' )  );
#2349=CARTESIAN_POINT ( 'NONE',  ( 155.0540265531850537, 2.143131898507880377E-16, -117.4317124430720725 ) ) ;
#2350=CARTESIAN_POINT ( 'NONE',  ( -127.7210997126620242, -1.749999999999996669, 159.7931612910809065 ) ) ;
#2351=CARTESIAN_POINT ( 'NONE',  ( 73.30402655318508209, -1.750000000000009992, -159.1817124430720298 ) ) ;
#2352=EDGE_CURVE ( 'NONE', #28177, #387, #24089, .T. ) ;
#2353=ADVANCED_FACE ( 'NONE', ( #7465 ), #38275, .T. ) ;
#2354=ORIENTED_EDGE ( 'NONE', *, *, #33928, .T. ) ;
#2358=EDGE_CURVE ( 'NONE', #7036, #16858, #9980, .T. ) ;
#2364=VERTEX_POINT ( 'NONE', #14898 ) ;
#2366=ORIENTED_EDGE ( 'NONE', *, *, #34383, .T. ) ;
#2370=DIRECTION ( 'NONE',  ( -0.000000000000000000, -0.000000000000000000, -1.000000000000000000 ) ) ;
#2376=CARTESIAN_POINT ( 'NONE',  ( 73.30402655318508209, 1.750000000000009992, -159.1817124430720298 ) ) ;
#2382=ORIENTED_EDGE ( 'NONE', *, *, #42487, .T. ) ;
#2391=CARTESIAN_POINT ( 'NONE',  ( 33.30402655318503946, 0.000000000000000000, 165.0000000000000000 ) ) ;
#2394=CARTESIAN_POINT ( 'NONE',  ( -208.4459734468148611, -1.025126265847089435, -40.93171244307204404 ) ) ;
#2398=ORIENTED_EDGE ( 'NONE', *, *, #9205, .F. ) ;
#2402=ORIENTED_EDGE ( 'NONE', *, *, #20620, .T. ) ;
#2406=EDGE_CURVE ( 'NONE', #45654, #13485, #8049, .T. ) ;
#2407=ORIENTED_EDGE ( 'NONE', *, *, #26303, .T. ) ;
#2409=ORIENTED_EDGE ( 'NONE', *, *, #22387, .F. ) ;
#2410=CARTESIAN_POINT ( 'NONE',  ( -46.69597344681494633, 0.000000000000000000, 165.0000000000000000 ) ) ;
#2413=ADVANCED_FACE ( 'NONE', ( #42342 ), #49994, .T. ) ;
#2426=AXIS2_PLACEMENT_3D ( 'NONE', #37433, #21497, #6610 ) ;
#2427=ORIENTED_EDGE ( 'NONE', *, *, #18054, .F. ) ;
#2430=CARTESIAN_POINT ( 'NONE',  ( -166.6959734468149463, -1.750000000000010214, -39.18171244307202983 ) ) ;
#2432=DIRECTION ( 'NONE',  ( -0.000000000000000000, -0.000000000000000000, -1.000000000000000000 ) ) ;
#2433=AXIS2_PLACEMENT_3D ( 'NONE', #14749, #5587, #48149 ) ;
#2434=( BOUNDED_CURVE ( )  B_SPLINE_CURVE ( 3, ( #20078, #46227, #27017, #43177 ),
 .UNSPECIFIED., .F., .F. ) 
 B_SPLINE_CURVE_WITH_KNOTS ( ( 4, 4 ),
 ( 1.570796326794896558, 3.141592653589793116 ),
 .UNSPECIFIED. ) 
 CURVE ( )  GEOMETRIC_REPRESENTATION_ITEM ( )  RATIONAL_B_SPLINE_CURVE ( ( 1.000000000000000000, 0.8047378541243649375, 0.8047378541243649375, 1.000000000000000000 ) ) 
 REPRESENTATION_ITEM ( '' )  );
#2435=DIRECTION ( 'NONE',  ( -1.000000000000000000, -0.000000000000000000, -0.000000000000000000 ) ) ;
#2436=VERTEX_POINT ( 'NONE', #34168 ) ;
#2440=ADVANCED_FACE ( 'NONE', ( #14391 ), #6685, .T. ) ;
#2441=CARTESIAN_POINT ( 'NONE',  ( 72.27890028733797578, 1.750000000000009548, -118.1565861772249519 ) ) ;
#2445=DIRECTION ( 'NONE',  ( -1.000000000000000000, 0.000000000000000000, 0.000000000000000000 ) ) ;
#2446=CARTESIAN_POINT ( 'NONE',  ( 112.2789002873379758, 1.749999999999997113, 119.7931612910809065 ) ) ;
#2454=ORIENTED_EDGE ( 'NONE', *, *, #37265, .T. ) ;
#2456=CARTESIAN_POINT ( 'NONE',  ( 115.0540265531850395, 2.143131898507847836E-16, 165.0000000000000000 ) ) ;
#2459=VECTOR ( 'NONE', #48852, 1000.000000000000000 ) ;
#2465=VECTOR ( 'NONE', #10680, 1000.000000000000000 ) ;
#2466=ORIENTED_EDGE ( 'NONE', *, *, #39946, .F. ) ;
#2471=AXIS2_PLACEMENT_3D ( 'NONE', #7256, #39587, #3909 ) ;
#2474=CARTESIAN_POINT ( 'NONE',  ( 210.0000000000000568, 0.000000000000000000, 0.8182875569279768335 ) ) ;
#2476=CARTESIAN_POINT ( 'NONE',  ( 75.05402655318509630, 2.143131898507880377E-16, 82.56828755692799859 ) ) ;
#2479=ORIENTED_EDGE ( 'NONE', *, *, #42053, .F. ) ;
#2480=CARTESIAN_POINT ( 'NONE',  ( 111.5540265531850679, 0.000000000000000000, -40.93171244307202983 ) ) ;
#2487=( BOUNDED_CURVE ( )  B_SPLINE_CURVE ( 3, ( #46976, #11618, #23920, #38581 ),
 .UNSPECIFIED., .F., .F. ) 
 B_SPLINE_CURVE_WITH_KNOTS ( ( 4, 4 ),
 ( 1.570796326794896558, 3.141592653589793116 ),
 .UNSPECIFIED. ) 
 CURVE ( )  GEOMETRIC_REPRESENTATION_ITEM ( )  RATIONAL_B_SPLINE_CURVE ( ( 1.000000000000000000, 0.8047378541243649375, 0.8047378541243649375, 1.000000000000000000 ) ) 
 REPRESENTATION_ITEM ( '' )  );
#2499=DIRECTION ( 'NONE',  ( -0.000000000000000000, -0.000000000000000000, -1.000000000000000000 ) ) ;
#2505=AXIS2_PLACEMENT_3D ( 'NONE', #5657, #21558, #20802 ) ;
#2508=FACE_OUTER_BOUND ( 'NONE', #19419, .T. ) ;
#2511=CARTESIAN_POINT ( 'NONE',  ( -44.94597344681493922, 2.143131898507880377E-16, -40.93171244307205825 ) ) ;
#2518=VERTEX_POINT ( 'NONE', #8734 ) ;
#2520=CARTESIAN_POINT ( 'NONE',  ( -5.670847180967843570, -1.750000000000023981, -120.2068387089191219 ) ) ;
#2523=FACE_OUTER_BOUND ( 'NONE', #1862, .T. ) ;
#2525=CARTESIAN_POINT ( 'NONE',  ( 73.30402655318508209, -1.750000000000009992, 0.8182875569279768335 ) ) ;
#2526=CARTESIAN_POINT ( 'NONE',  ( 31.55402655318503236, 1.025126265847088991, 2.568287556927986159 ) ) ;
#2530=DIRECTION ( 'NONE',  ( -0.000000000000000000, -0.000000000000000000, -1.000000000000000000 ) ) ;
#2534=CARTESIAN_POINT ( 'NONE',  ( 153.3040265531850537, 1.750000000000010658, -119.1817124430720440 ) ) ;
#2535=EDGE_LOOP ( 'NONE', ( #31786, #44451, #48293, #20274, #5994, #14410 ) ) ;
#2538=CARTESIAN_POINT ( 'NONE',  ( 191.5540265531851105, 0.000000000000000000, 165.0000000000000000 ) ) ;
#2539=CARTESIAN_POINT ( 'NONE',  ( 33.30402655318503946, 0.000000000000000000, 165.0000000000000000 ) ) ;
#2542=DIRECTION ( 'NONE',  ( -0.000000000000000000, -0.000000000000000000, -1.000000000000000000 ) ) ;
#2543=CARTESIAN_POINT ( 'NONE',  ( -86.69597344681494633, -1.750000000000010658, 80.81828755692798438 ) ) ;
#2549=CARTESIAN_POINT ( 'NONE',  ( 210.0000000000000568, 0.000000000000000000, 42.56828755692799149 ) ) ;
#2552=LINE ( 'NONE', #14358, #38851 ) ;
#2556=ORIENTED_EDGE ( 'NONE', *, *, #807, .F. ) ;
#2558=DIRECTION ( 'NONE',  ( 0.000000000000000000, 0.000000000000000000, 1.000000000000000000 ) ) ;
#2559=CARTESIAN_POINT ( 'NONE',  ( -44.94597344681493922, 1.025126265847089435, -157.4317124430720582 ) ) ;
#2563=CARTESIAN_POINT ( 'NONE',  ( -48.44597344681496054, -1.025126265847089879, 122.5682875569280128 ) ) ;
#2564=ORIENTED_EDGE ( 'NONE', *, *, #49638, .F. ) ;
#2569=DIRECTION ( 'NONE',  ( -1.000000000000000000, -0.000000000000000000, -0.000000000000000000 ) ) ;
#2570=AXIS2_PLACEMENT_3D ( 'NONE', #20119, #8583, #24239 ) ;
#2571=EDGE_LOOP ( 'NONE', ( #46749, #13467, #29657, #17898, #34645, #15068 ) ) ;
#2591=CARTESIAN_POINT ( 'NONE',  ( 31.55402655318503236, 0.000000000000000000, -165.0000000000000000 ) ) ;
#2593=CARTESIAN_POINT ( 'NONE',  ( 155.0540265531850537, 2.143131898507880377E-16, 79.06828755692797017 ) ) ;
#2602=EDGE_CURVE ( 'NONE', #3325, #48435, #48297, .T. ) ;
#2606=FACE_OUTER_BOUND ( 'NONE', #42301, .T. ) ;
#2609=DIRECTION ( 'NONE',  ( 0.000000000000000000, 0.000000000000000000, 1.000000000000000000 ) ) ;
#2614=EDGE_CURVE ( 'NONE', #34400, #46777, #40033, .T. ) ;
#2617=( BOUNDED_CURVE ( )  B_SPLINE_CURVE ( 3, ( #23273, #18914, #15346, #27653 ),
 .UNSPECIFIED., .F., .F. ) 
 B_SPLINE_CURVE_WITH_KNOTS ( ( 4, 4 ),
 ( 0.000000000000000000, 1.570796326794896558 ),
 .UNSPECIFIED. ) 
 CURVE ( )  GEOMETRIC_REPRESENTATION_ITEM ( )  RATIONAL_B_SPLINE_CURVE ( ( 1.000000000000000000, 0.8047378541243649375, 0.8047378541243649375, 1.000000000000000000 ) ) 
 REPRESENTATION_ITEM ( '' )  );
#2620=DIRECTION ( 'NONE',  ( 1.000000000000000000, 0.000000000000000000, -0.000000000000000000 ) ) ;
#2622=FACE_OUTER_BOUND ( 'NONE', #44189, .T. ) ;
#2623=( BOUNDED_CURVE ( )  B_SPLINE_CURVE ( 3, ( #29682, #44808, #40985, #26348 ),
 .UNSPECIFIED., .F., .F. ) 
 B_SPLINE_CURVE_WITH_KNOTS ( ( 4, 4 ),
 ( 1.570796326794896558, 3.141592653589793116 ),
 .UNSPECIFIED. ) 
 CURVE ( )  GEOMETRIC_REPRESENTATION_ITEM ( )  RATIONAL_B_SPLINE_CURVE ( ( 1.000000000000000000, 0.8047378541243649375, 0.8047378541243649375, 1.000000000000000000 ) ) 
 REPRESENTATION_ITEM ( '' )  );
#2626=EDGE_CURVE ( 'NONE', #41151, #33474, #47825, .T. ) ;
#2627=DIRECTION ( 'NONE',  ( 0.000000000000000000, 0.000000000000000000, -1.000000000000000000 ) ) ;
#2632=EDGE_CURVE ( 'NONE', #14525, #387, #13267, .T. ) ;
#2641=( BOUNDED_CURVE ( )  B_SPLINE_CURVE ( 3, ( #33806, #3231, #33554, #22245 ),
 .UNSPECIFIED., .F., .F. ) 
 B_SPLINE_CURVE_WITH_KNOTS ( ( 4, 4 ),
 ( 3.141592653589793116, 4.712388980384689674 ),
 .UNSPECIFIED. ) 
 CURVE ( )  GEOMETRIC_REPRESENTATION_ITEM ( )  RATIONAL_B_SPLINE_CURVE ( ( 1.000000000000000000, 0.8047378541243649375, 0.8047378541243649375, 1.000000000000000000 ) ) 
 REPRESENTATION_ITEM ( '' )  );
#2642=ORIENTED_EDGE ( 'NONE', *, *, #28141, .F. ) ;
#2643=ORIENTED_EDGE ( 'NONE', *, *, #15632, .F. ) ;
#2647=EDGE_LOOP ( 'NONE', ( #8365, #19298, #46418, #20713, #36956, #22631 ) ) ;
#2652=FACE_OUTER_BOUND ( 'NONE', #21506, .T. ) ;
#2656=CARTESIAN_POINT ( 'NONE',  ( -166.6959734468149463, 1.750000000000010658, -79.18171244307201562 ) ) ;
#2657=CYLINDRICAL_SURFACE ( 'NONE', #42104, 1.750000000000010214 ) ;
#2659=EDGE_CURVE ( 'NONE', #9213, #50130, #13564, .T. ) ;
#2660=ORIENTED_EDGE ( 'NONE', *, *, #18732, .T. ) ;
#2665=CARTESIAN_POINT ( 'NONE',  ( -46.69597344681494633, -1.750000000000010214, 40.81828755692798438 ) ) ;
#2668=ORIENTED_EDGE ( 'NONE', *, *, #23201, .T. ) ;
#2671=DIRECTION ( 'NONE',  ( -0.000000000000000000, -0.000000000000000000, -1.000000000000000000 ) ) ;
#2673=ORIENTED_EDGE ( 'NONE', *, *, #6086, .T. ) ;
#2676=CARTESIAN_POINT ( 'NONE',  ( -168.4459734468149463, 0.000000000000000000, 165.0000000000000000 ) ) ;
#2678=CARTESIAN_POINT ( 'NONE',  ( -164.9459734468149463, -1.025126265847089657, 79.06828755692797017 ) ) ;
#2679=ORIENTED_EDGE ( 'NONE', *, *, #28748, .T. ) ;
#2686=CYLINDRICAL_SURFACE ( 'NONE', #23111, 1.750000000000008438 ) ;
#2687=CARTESIAN_POINT ( 'NONE',  ( 71.55402655318505367, 0.000000000000000000, 122.5682875569279844 ) ) ;
#2688=ADVANCED_FACE ( 'NONE', ( #5872 ), #6127, .T. ) ;
#2699=ADVANCED_FACE ( 'NONE', ( #44347 ), #2028, .T. ) ;
#2704=EDGE_CURVE ( 'NONE', #4734, #34716, #37453, .T. ) ;
#2708=AXIS2_PLACEMENT_3D ( 'NONE', #11786, #7946, #23582 ) ;
#2712=ORIENTED_EDGE ( 'NONE', *, *, #6473, .F. ) ;
#2715=CARTESIAN_POINT ( 'NONE',  ( -125.6708471809678542, -1.749999999999996669, -160.2068387089191219 ) ) ;
#2716=CARTESIAN_POINT ( 'NONE',  ( 210.0000000000000568, 0.000000000000000000, -159.1817124430720298 ) ) ;
#2722=ORIENTED_EDGE ( 'NONE', *, *, #2924, .T. ) ;
#2724=ORIENTED_EDGE ( 'NONE', *, *, #34275, .F. ) ;
#2725=CARTESIAN_POINT ( 'NONE',  ( 210.0000000000000568, 0.000000000000000000, 122.5682875569279844 ) ) ;
#2726=DIRECTION ( 'NONE',  ( -1.000000000000000000, 0.000000000000000000, 0.000000000000000000 ) ) ;
#2727=LINE ( 'NONE', #2974, #10291 ) ;
#2729=CARTESIAN_POINT ( 'NONE',  ( -208.4459734468149463, 0.000000000000000000, -0.9317124430720247208 ) ) ;
#2732=CYLINDRICAL_SURFACE ( 'NONE', #43327, 1.750000000000001554 ) ;
#2737=AXIS2_PLACEMENT_3D ( 'NONE', #21421, #29632, #11155 ) ;
#2738=CARTESIAN_POINT ( 'NONE',  ( -210.0000000000000568, 0.000000000000000000, 80.81828755692798438 ) ) ;
#2744=CARTESIAN_POINT ( 'NONE',  ( 151.5540265531850537, 0.000000000000000000, 165.0000000000000000 ) ) ;
#2745=DIRECTION ( 'NONE',  ( 0.000000000000000000, 0.000000000000000000, 1.000000000000000000 ) ) ;
#2754=CARTESIAN_POINT ( 'NONE',  ( 32.27890028733795447, 1.750000000000009548, -38.15658617722494483 ) ) ;
#2757=ORIENTED_EDGE ( 'NONE', *, *, #36900, .F. ) ;
#2771=EDGE_CURVE ( 'NONE', #35393, #42459, #37875, .T. ) ;
#2776=AXIS2_PLACEMENT_3D ( 'NONE', #47639, #12527, #28690 ) ;
#2777=DIRECTION ( 'NONE',  ( -1.000000000000000000, -0.000000000000000000, -0.000000000000000000 ) ) ;
#2778=( BOUNDED_CURVE ( )  B_SPLINE_CURVE ( 3, ( #2525, #18166, #49434, #14321 ),
 .UNSPECIFIED., .F., .F. ) 
 B_SPLINE_CURVE_WITH_KNOTS ( ( 4, 4 ),
 ( 4.712388980384689674, 6.283185307179586232 ),
 .UNSPECIFIED. ) 
 CURVE ( )  GEOMETRIC_REPRESENTATION_ITEM ( )  RATIONAL_B_SPLINE_CURVE ( ( 1.000000000000000000, 0.8047378541243649375, 0.8047378541243649375, 1.000000000000000000 ) ) 
 REPRESENTATION_ITEM ( '' )  );
#2781=VERTEX_POINT ( 'NONE', #10722 ) ;
#2782=ORIENTED_EDGE ( 'NONE', *, *, #37767, .T. ) ;
#2786=( BOUNDED_CURVE ( )  B_SPLINE_CURVE ( 3, ( #26945, #47166, #35176, #15144 ),
 .UNSPECIFIED., .F., .F. ) 
 B_SPLINE_CURVE_WITH_KNOTS ( ( 4, 4 ),
 ( 3.141592653589793116, 4.712388980384689674 ),
 .UNSPECIFIED. ) 
 CURVE ( )  GEOMETRIC_REPRESENTATION_ITEM ( )  RATIONAL_B_SPLINE_CURVE ( ( 1.000000000000000000, 0.8047378541243649375, 0.8047378541243649375, 1.000000000000000000 ) ) 
 REPRESENTATION_ITEM ( '' )  );
#2789=ORIENTED_EDGE ( 'NONE', *, *, #5538, .F. ) ;
#2790=CARTESIAN_POINT ( 'NONE',  ( -206.6959734468149463, 1.750000000000009992, 0.8182875569279768335 ) ) ;
#2794=CARTESIAN_POINT ( 'NONE',  ( 151.5540265531850537, -1.025126265847089879, -77.43171244307200141 ) ) ;
#2801=AXIS2_PLACEMENT_3D ( 'NONE', #27850, #12435, #39410 ) ;
#2803=CARTESIAN_POINT ( 'NONE',  ( -44.94597344681493922, 2.143131898507880377E-16, 39.06828755692798438 ) ) ;
#2804=ORIENTED_EDGE ( 'NONE', *, *, #38669, .F. ) ;
#2805=CARTESIAN_POINT ( 'NONE',  ( 210.0000000000000568, 2.143131898507881856E-16, -120.9317124430720582 ) ) ;
#2808=CARTESIAN_POINT ( 'NONE',  ( 71.55402655318506788, 0.000000000000000000, 162.5682875569279702 ) ) ;
#2809=AXIS2_PLACEMENT_3D ( 'NONE', #38403, #11199, #46799 ) ;
#2812=VERTEX_POINT ( 'NONE', #23497 ) ;
#2813=DIRECTION ( 'NONE',  ( -1.000000000000000000, -0.000000000000000000, -0.000000000000000000 ) ) ;
#2815=CARTESIAN_POINT ( 'NONE',  ( -6.695973446814940111, -1.750000000000023759, 40.81828755692798438 ) ) ;
#2816=DIRECTION ( 'NONE',  ( -1.000000000000000000, 0.000000000000000000, 0.000000000000000000 ) ) ;
#2820=VECTOR ( 'NONE', #30331, 1000.000000000000000 ) ;
#2821=CARTESIAN_POINT ( 'NONE',  ( -85.67084718096784002, -1.750000000000009548, -0.2068387089191121020 ) ) ;
#2826=CARTESIAN_POINT ( 'NONE',  ( -88.44597344681497475, 0.000000000000000000, -117.4317124430720156 ) ) ;
#2829=ORIENTED_EDGE ( 'NONE', *, *, #26161, .F. ) ;
#2831=CARTESIAN_POINT ( 'NONE',  ( 210.0000000000000568, 0.000000000000000000, -79.18171244307201562 ) ) ;
#2837=CARTESIAN_POINT ( 'NONE',  ( -44.94597344681493922, -1.025126265847088991, -157.4317124430720582 ) ) ;
#2838=CARTESIAN_POINT ( 'NONE',  ( 155.0540265531850537, 2.143131898507880377E-16, -80.93171244307201562 ) ) ;
#2844=ORIENTED_EDGE ( 'NONE', *, *, #35570, .T. ) ;
#2846=CARTESIAN_POINT ( 'NONE',  ( 115.0540265531850395, 1.025126265847081664, 2.568287556927973281 ) ) ;
#2854=CARTESIAN_POINT ( 'NONE',  ( 114.3291528190321173, 1.749999999999996891, 79.79316129108087807 ) ) ;
#2858=CARTESIAN_POINT ( 'NONE',  ( 210.0000000000000568, 0.000000000000000000, -37.43171244307202272 ) ) ;
#2863=VECTOR ( 'NONE', #30453, 1000.000000000000000 ) ;
#2867=CARTESIAN_POINT ( 'NONE',  ( 115.0540265531850395, 1.025126265847082108, 82.56828755692798438 ) ) ;
#2869=CARTESIAN_POINT ( 'NONE',  ( -166.6959734468149463, 0.000000000000000000, 165.0000000000000000 ) ) ;
#2878=EDGE_CURVE ( 'NONE', #5639, #25771, #10477, .T. ) ;
#2883=ORIENTED_EDGE ( 'NONE', *, *, #47411, .F. ) ;
#2885=CARTESIAN_POINT ( 'NONE',  ( -204.9459734468149463, 2.143131898507880377E-16, 79.06828755692797017 ) ) ;
#2892=ADVANCED_FACE ( 'NONE', ( #33590 ), #6373, .T. ) ;
#2893=AXIS2_PLACEMENT_3D ( 'NONE', #43630, #40305, #24161 ) ;
#2894=EDGE_CURVE ( 'NONE', #47489, #48612, #14926, .T. ) ;
#2896=EDGE_CURVE ( 'NONE', #936, #48865, #18420, .T. ) ;
#2899=EDGE_LOOP ( 'NONE', ( #926, #6392, #23218, #19533, #19849, #34241 ) ) ;
#2902=ORIENTED_EDGE ( 'NONE', *, *, #25498, .T. ) ;
#2904=CARTESIAN_POINT ( 'NONE',  ( -210.0000000000000568, 2.143131898507876926E-16, -80.93171244307202983 ) ) ;
#2905=EDGE_LOOP ( 'NONE', ( #43290, #29468, #50497, #15454, #205 ) ) ;
#2907=EDGE_CURVE ( 'NONE', #36589, #33796, #2778, .T. ) ;
#2915=( BOUNDED_CURVE ( )  B_SPLINE_CURVE ( 3, ( #10716, #2520, #18415, #29980 ),
 .UNSPECIFIED., .F., .F. ) 
 B_SPLINE_CURVE_WITH_KNOTS ( ( 4, 4 ),
 ( 4.712388980384689674, 6.283185307179586232 ),
 .UNSPECIFIED. ) 
 CURVE ( )  GEOMETRIC_REPRESENTATION_ITEM ( )  RATIONAL_B_SPLINE_CURVE ( ( 1.000000000000000000, 0.8047378541243649375, 0.8047378541243649375, 1.000000000000000000 ) ) 
 REPRESENTATION_ITEM ( '' )  );
#2916=EDGE_CURVE ( 'NONE', #31511, #25305, #21824, .T. ) ;
#2917=CARTESIAN_POINT ( 'NONE',  ( 115.0540265531850395, 2.143131898507847836E-16, -37.43171244307205825 ) ) ;
#2918=CARTESIAN_POINT ( 'NONE',  ( 75.05402655318509630, -1.025126265847089435, -117.4317124430720156 ) ) ;
#2920=EDGE_CURVE ( 'NONE', #44875, #17662, #36277, .T. ) ;
#2921=CARTESIAN_POINT ( 'NONE',  ( -166.6959734468149463, -1.750000000000010658, -119.1817124430720440 ) ) ;
#2922=ORIENTED_EDGE ( 'NONE', *, *, #5675, .F. ) ;
#2923=( BOUNDED_CURVE ( )  B_SPLINE_CURVE ( 3, ( #6080, #21726, #2235, #42481 ),
 .UNSPECIFIED., .F., .F. ) 
 B_SPLINE_CURVE_WITH_KNOTS ( ( 4, 4 ),
 ( 1.570796326794896558, 3.141592653589793116 ),
 .UNSPECIFIED. ) 
 CURVE ( )  GEOMETRIC_REPRESENTATION_ITEM ( )  RATIONAL_B_SPLINE_CURVE ( ( 1.000000000000000000, 0.8047378541243649375, 0.8047378541243649375, 1.000000000000000000 ) ) 
 REPRESENTATION_ITEM ( '' )  );
#2924=EDGE_CURVE ( 'NONE', #42077, #42464, #39827, .T. ) ;
#2927=CARTESIAN_POINT ( 'NONE',  ( 72.27890028733797578, 1.750000000000009548, -38.15658617722494483 ) ) ;
#2936=ORIENTED_EDGE ( 'NONE', *, *, #20797, .T. ) ;
#2939=ADVANCED_FACE ( 'NONE', ( #36322 ), #4745, .T. ) ;
#2940=ADVANCED_FACE ( 'NONE', ( #24505 ), #43982, .T. ) ;
#2947=ORIENTED_EDGE ( 'NONE', *, *, #9831, .T. ) ;
#2950=EDGE_CURVE ( 'NONE', #40469, #36951, #13197, .T. ) ;
#2955=CARTESIAN_POINT ( 'NONE',  ( 193.3040265531851105, 1.750000000000010214, -39.18171244307202983 ) ) ;
#2957=EDGE_LOOP ( 'NONE', ( #35682, #1523, #14776, #47922, #39971, #20751 ) ) ;
#2958=ORIENTED_EDGE ( 'NONE', *, *, #2310, .T. ) ;
#2965=VECTOR ( 'NONE', #33104, 1000.000000000000000 ) ;
#2971=ORIENTED_EDGE ( 'NONE', *, *, #30880, .T. ) ;
#2972=CARTESIAN_POINT ( 'NONE',  ( 111.5540265531850537, -1.025126265847081442, 159.0682875569279418 ) ) ;
#2974=CARTESIAN_POINT ( 'NONE',  ( 210.0000000000000568, 2.143131898507881116E-16, 39.06828755692797728 ) ) ;
#2980=EDGE_CURVE ( 'NONE', #2364, #49857, #50235, .T. ) ;
#2982=CARTESIAN_POINT ( 'NONE',  ( -86.69597344681494633, 1.750000000000009992, -159.1817124430720298 ) ) ;
#2983=ADVANCED_FACE ( 'NONE', ( #27852 ), #43485, .T. ) ;
#2985=CARTESIAN_POINT ( 'NONE',  ( 210.0000000000000568, 2.143131898507881856E-16, 119.0682875569279560 ) ) ;
#2991=LINE ( 'NONE', #31482, #32243 ) ;
#2997=VERTEX_POINT ( 'NONE', #10368 ) ;
#3001=ORIENTED_EDGE ( 'NONE', *, *, #9563, .F. ) ;
#3006=ORIENTED_EDGE ( 'NONE', *, *, #34345, .F. ) ;
#3012=VERTEX_POINT ( 'NONE', #13698 ) ;
#3013=ORIENTED_EDGE ( 'NONE', *, *, #1265, .T. ) ;
#3015=ORIENTED_EDGE ( 'NONE', *, *, #25363, .T. ) ;
#3016=CARTESIAN_POINT ( 'NONE',  ( 111.5540265531850679, 0.000000000000000000, -40.93171244307202983 ) ) ;
#3018=( BOUNDED_CURVE ( )  B_SPLINE_CURVE ( 3, ( #36533, #47755, #4204, #4708 ),
 .UNSPECIFIED., .F., .F. ) 
 B_SPLINE_CURVE_WITH_KNOTS ( ( 4, 4 ),
 ( 4.712388980384689674, 6.283185307179586232 ),
 .UNSPECIFIED. ) 
 CURVE ( )  GEOMETRIC_REPRESENTATION_ITEM ( )  RATIONAL_B_SPLINE_CURVE ( ( 1.000000000000000000, 0.8047378541243649375, 0.8047378541243649375, 1.000000000000000000 ) ) 
 REPRESENTATION_ITEM ( '' )  );
#3022=CARTESIAN_POINT ( 'NONE',  ( 195.0540265531851105, 2.143131898507880377E-16, 165.0000000000000000 ) ) ;
#3024=VECTOR ( 'NONE', #43424, 1000.000000000000000 ) ;
#3025=DIRECTION ( 'NONE',  ( 0.000000000000000000, 0.000000000000000000, 1.000000000000000000 ) ) ;
#3035=ORIENTED_EDGE ( 'NONE', *, *, #8382, .F. ) ;
#3036=DIRECTION ( 'NONE',  ( -0.000000000000000000, -0.000000000000000000, -1.000000000000000000 ) ) ;
#3037=FACE_OUTER_BOUND ( 'NONE', #21079, .T. ) ;
#3039=LINE ( 'NONE', #17694, #20841 ) ;
#3045=EDGE_CURVE ( 'NONE', #23318, #42480, #30981, .T. ) ;
#3048=CARTESIAN_POINT ( 'NONE',  ( 73.30402655318508209, 0.000000000000000000, 165.0000000000000000 ) ) ;
#3054=DIRECTION ( 'NONE',  ( -1.000000000000000000, -0.000000000000000000, -0.000000000000000000 ) ) ;
#3058=ORIENTED_EDGE ( 'NONE', *, *, #5388, .F. ) ;
#3059=CARTESIAN_POINT ( 'NONE',  ( -165.6708471809677974, 1.750000000000010214, 119.7931612910808781 ) ) ;
#3061=EDGE_CURVE ( 'NONE', #9299, #5041, #18513, .T. ) ;
#3070=DIRECTION ( 'NONE',  ( -0.000000000000000000, -0.000000000000000000, -1.000000000000000000 ) ) ;
#3071=ORIENTED_EDGE ( 'NONE', *, *, #26122, .T. ) ;
#3072=DIRECTION ( 'NONE',  ( -1.000000000000000000, -0.000000000000000000, -0.000000000000000000 ) ) ;
#3074=( BOUNDED_CURVE ( )  B_SPLINE_CURVE ( 3, ( #13599, #45631, #9744, #34135 ),
 .UNSPECIFIED., .F., .F. ) 
 B_SPLINE_CURVE_WITH_KNOTS ( ( 4, 4 ),
 ( 4.712388980384689674, 6.283185307179586232 ),
 .UNSPECIFIED. ) 
 CURVE ( )  GEOMETRIC_REPRESENTATION_ITEM ( )  RATIONAL_B_SPLINE_CURVE ( ( 1.000000000000000000, 0.8047378541243649375, 0.8047378541243649375, 1.000000000000000000 ) ) 
 REPRESENTATION_ITEM ( '' )  );
#3080=ORIENTED_EDGE ( 'NONE', *, *, #47279, .F. ) ;
#3082=FACE_OUTER_BOUND ( 'NONE', #32907, .T. ) ;
#3084=( BOUNDED_CURVE ( )  B_SPLINE_CURVE ( 3, ( #19137, #27112, #19659, #11455 ),
 .UNSPECIFIED., .F., .F. ) 
 B_SPLINE_CURVE_WITH_KNOTS ( ( 4, 4 ),
 ( 1.570796326794896558, 3.141592653589793116 ),
 .UNSPECIFIED. ) 
 CURVE ( )  GEOMETRIC_REPRESENTATION_ITEM ( )  RATIONAL_B_SPLINE_CURVE ( ( 1.000000000000000000, 0.8047378541243649375, 0.8047378541243649375, 1.000000000000000000 ) ) 
 REPRESENTATION_ITEM ( '' )  );
#3085=EDGE_LOOP ( 'NONE', ( #2922, #23541, #10418, #18159, #25180, #45487 ) ) ;
#3094=CARTESIAN_POINT ( 'NONE',  ( -168.4459734468149463, 0.000000000000000000, 82.56828755692798438 ) ) ;
#3108=ORIENTED_EDGE ( 'NONE', *, *, #35912, .F. ) ;
#3110=EDGE_CURVE ( 'NONE', #15554, #9081, #37082, .T. ) ;
#3111=EDGE_CURVE ( 'NONE', #20412, #42459, #33229, .T. ) ;
#3112=DIRECTION ( 'NONE',  ( -1.000000000000000000, 0.000000000000000000, 0.000000000000000000 ) ) ;
#3114=CARTESIAN_POINT ( 'NONE',  ( 115.0540265531850395, 2.143131898507847836E-16, 79.06828755692798438 ) ) ;
#3120=EDGE_CURVE ( 'NONE', #18505, #50033, #41449, .T. ) ;
#3126=DIRECTION ( 'NONE',  ( -1.000000000000000000, -0.000000000000000000, -0.000000000000000000 ) ) ;
#3132=CARTESIAN_POINT ( 'NONE',  ( -210.0000000000000568, 0.000000000000000000, -39.18171244307202983 ) ) ;
#3135=DIRECTION ( 'NONE',  ( 0.000000000000000000, 0.000000000000000000, 1.000000000000000000 ) ) ;
#3136=CARTESIAN_POINT ( 'NONE',  ( 210.0000000000000568, 0.000000000000000000, 160.8182875569279702 ) ) ;
#3139=CARTESIAN_POINT ( 'NONE',  ( -208.4459734468148611, -1.025126265847089435, 162.5682875569279133 ) ) ;
#3143=EDGE_LOOP ( 'NONE', ( #11241, #17569, #15727, #15784, #45336, #25581 ) ) ;
#3147=LINE ( 'NONE', #46728, #12000 ) ;
#3151=ORIENTED_EDGE ( 'NONE', *, *, #8795, .F. ) ;
#3155=ORIENTED_EDGE ( 'NONE', *, *, #27453, .F. ) ;
#3160=CARTESIAN_POINT ( 'NONE',  ( -167.7210997126620384, 1.750000000000010436, -120.2068387089191219 ) ) ;
#3163=ORIENTED_EDGE ( 'NONE', *, *, #23730, .F. ) ;
#3167=CARTESIAN_POINT ( 'NONE',  ( -208.4459734468149463, 0.000000000000000000, 2.568287556927978166 ) ) ;
#3169=CARTESIAN_POINT ( 'NONE',  ( -88.44597344681494633, 1.025126265847089213, -37.43171244307202272 ) ) ;
#3170=CARTESIAN_POINT ( 'NONE',  ( 71.55402655318505367, 0.000000000000000000, -0.9317124430720524764 ) ) ;
#3178=CIRCLE ( 'NONE', #31046, 1.750000000000001554 ) ;
#3195=ORIENTED_EDGE ( 'NONE', *, *, #14454, .F. ) ;
#3203=ORIENTED_EDGE ( 'NONE', *, *, #39529, .T. ) ;
#3205=ORIENTED_EDGE ( 'NONE', *, *, #50496, .T. ) ;
#3210=( BOUNDED_CURVE ( )  B_SPLINE_CURVE ( 3, ( #8952, #28706, #47906, #40510 ),
 .UNSPECIFIED., .F., .F. ) 
 B_SPLINE_CURVE_WITH_KNOTS ( ( 4, 4 ),
 ( 4.712388980384689674, 6.283185307179586232 ),
 .UNSPECIFIED. ) 
 CURVE ( )  GEOMETRIC_REPRESENTATION_ITEM ( )  RATIONAL_B_SPLINE_CURVE ( ( 1.000000000000000000, 0.8047378541243649375, 0.8047378541243649375, 1.000000000000000000 ) ) 
 REPRESENTATION_ITEM ( '' )  );
#3212=CIRCLE ( 'NONE', #2433, 1.750000000000001554 ) ;
#3214=CARTESIAN_POINT ( 'NONE',  ( 75.05402655318509630, 2.143131898507880377E-16, -40.93171244307205825 ) ) ;
#3215=VERTEX_POINT ( 'NONE', #15470 ) ;
#3217=DIRECTION ( 'NONE',  ( 0.000000000000000000, 0.000000000000000000, -1.000000000000000000 ) ) ;
#3220=( BOUNDED_CURVE ( )  B_SPLINE_CURVE ( 3, ( #11599, #27249, #42874, #7238 ),
 .UNSPECIFIED., .F., .F. ) 
 B_SPLINE_CURVE_WITH_KNOTS ( ( 4, 4 ),
 ( 4.712388980384689674, 6.283185307179586232 ),
 .UNSPECIFIED. ) 
 CURVE ( )  GEOMETRIC_REPRESENTATION_ITEM ( )  RATIONAL_B_SPLINE_CURVE ( ( 1.000000000000000000, 0.8047378541243649375, 0.8047378541243649375, 1.000000000000000000 ) ) 
 REPRESENTATION_ITEM ( '' )  );
#3222=CARTESIAN_POINT ( 'NONE',  ( 115.0540265531850395, 1.025126265847082108, -37.43171244307203693 ) ) ;
#3223=ORIENTED_EDGE ( 'NONE', *, *, #41886, .F. ) ;
#3224=ORIENTED_EDGE ( 'NONE', *, *, #3704, .F. ) ;
#3225=CARTESIAN_POINT ( 'NONE',  ( 191.5540265531850537, 1.025126265847089657, 119.0682875569279560 ) ) ;
#3226=FACE_OUTER_BOUND ( 'NONE', #27179, .T. ) ;
#3228=CYLINDRICAL_SURFACE ( 'NONE', #4739, 1.750000000000015543 ) ;
#3231=CARTESIAN_POINT ( 'NONE',  ( -44.94597344681493922, -1.025126265847088991, 159.0682875569279418 ) ) ;
#3237=( BOUNDED_CURVE ( )  B_SPLINE_CURVE ( 3, ( #23946, #43940, #39608, #32410 ),
 .UNSPECIFIED., .F., .F. ) 
 B_SPLINE_CURVE_WITH_KNOTS ( ( 4, 4 ),
 ( 3.141592653589793116, 4.712388980384689674 ),
 .UNSPECIFIED. ) 
 CURVE ( )  GEOMETRIC_REPRESENTATION_ITEM ( )  RATIONAL_B_SPLINE_CURVE ( ( 1.000000000000000000, 0.8047378541243649375, 0.8047378541243649375, 1.000000000000000000 ) ) 
 REPRESENTATION_ITEM ( '' )  );
#3245=DIRECTION ( 'NONE',  ( -1.000000000000000000, 0.000000000000000000, 0.000000000000000000 ) ) ;
#3247=CARTESIAN_POINT ( 'NONE',  ( -84.94597344681494633, 2.143131898507880377E-16, -157.4317124430720582 ) ) ;
#3249=CARTESIAN_POINT ( 'NONE',  ( -206.6959734468149463, 0.000000000000000000, 165.0000000000000000 ) ) ;
#3260=ADVANCED_FACE ( 'NONE', ( #18549 ), #7267, .T. ) ;
#3264=DIRECTION ( 'NONE',  ( -0.000000000000000000, -0.000000000000000000, -1.000000000000000000 ) ) ;
#3266=EDGE_CURVE ( 'NONE', #14624, #46895, #27063, .T. ) ;
#3267=EDGE_CURVE ( 'NONE', #12079, #14709, #30671, .T. ) ;
#3273=ADVANCED_FACE ( 'NONE', ( #27019 ), #3666, .T. ) ;
#3274=CARTESIAN_POINT ( 'NONE',  ( 73.30402655318508209, -1.750000000000010658, 80.81828755692798438 ) ) ;
#3276=CARTESIAN_POINT ( 'NONE',  ( 74.32915281903215998, 1.750000000000009548, 159.7931612910809065 ) ) ;
#3277=FACE_OUTER_BOUND ( 'NONE', #48315, .T. ) ;
#3278=CARTESIAN_POINT ( 'NONE',  ( -8.445973446814964092, 1.025126265847097429, 119.0682875569279133 ) ) ;
#3288=AXIS2_PLACEMENT_3D ( 'NONE', #19939, #8158, #39211 ) ;
#3289=ADVANCED_FACE ( 'NONE', ( #50573 ), #16493, .T. ) ;
#3293=VECTOR ( 'NONE', #13618, 1000.000000000000000 ) ;
#3294=ADVANCED_FACE ( 'NONE', ( #4692 ), #32393, .T. ) ;
#3295=CARTESIAN_POINT ( 'NONE',  ( 32.27890028733795447, -1.750000000000010214, -80.20683870891910772 ) ) ;
#3296=CARTESIAN_POINT ( 'NONE',  ( -86.69597344681494633, -1.750000000000010658, 80.81828755692798438 ) ) ;
#3299=CYLINDRICAL_SURFACE ( 'NONE', #39700, 1.750000000000001554 ) ;
#3300=CARTESIAN_POINT ( 'NONE',  ( -124.9459734468149463, 2.143131898507847836E-16, 79.06828755692798438 ) ) ;
#3303=CARTESIAN_POINT ( 'NONE',  ( -126.6959734468149321, 0.000000000000000000, 165.0000000000000000 ) ) ;
#3304=VECTOR ( 'NONE', #28764, 1000.000000000000000 ) ;
#3305=ORIENTED_EDGE ( 'NONE', *, *, #13985, .T. ) ;
#3310=ORIENTED_EDGE ( 'NONE', *, *, #28398, .T. ) ;
#3311=CARTESIAN_POINT ( 'NONE',  ( -7.721099712662037540, 1.750000000000023315, 121.8434138227750623 ) ) ;
#3313=DIRECTION ( 'NONE',  ( 1.000000000000000000, 0.000000000000000000, 0.000000000000000000 ) ) ;
#3321=ORIENTED_EDGE ( 'NONE', *, *, #10741, .F. ) ;
#3324=ORIENTED_EDGE ( 'NONE', *, *, #40374, .F. ) ;
#3325=VERTEX_POINT ( 'NONE', #28541 ) ;
#3328=ADVANCED_FACE ( 'NONE', ( #600 ), #8042, .F. ) ;
#3335=CARTESIAN_POINT ( 'NONE',  ( -45.67084718096785423, 1.750000000000009548, 1.843413822775065825 ) ) ;
#3336=ORIENTED_EDGE ( 'NONE', *, *, #17142, .F. ) ;
#3340=ORIENTED_EDGE ( 'NONE', *, *, #13714, .F. ) ;
#3341=CARTESIAN_POINT ( 'NONE',  ( -87.72109971266203843, -1.750000000000009548, 161.8434138227750907 ) ) ;
#3344=EDGE_CURVE ( 'NONE', #34855, #45594, #22413, .T. ) ;
#3347=CARTESIAN_POINT ( 'NONE',  ( 73.30402655318508209, 0.000000000000000000, 165.0000000000000000 ) ) ;
#3352=EDGE_LOOP ( 'NONE', ( #11966, #12871, #41989, #33452, #15521, #7643 ) ) ;
#3354=CARTESIAN_POINT ( 'NONE',  ( 153.3040265531850537, 0.000000000000000000, 165.0000000000000000 ) ) ;
#3365=CARTESIAN_POINT ( 'NONE',  ( 115.0540265531850395, 2.143131898507847836E-16, 122.5682875569279560 ) ) ;
#3371=CARTESIAN_POINT ( 'NONE',  ( -46.69597344681494633, 1.750000000000010658, -79.18171244307201562 ) ) ;
#3382=LINE ( 'NONE', #11348, #13475 ) ;
#3383=( BOUNDED_CURVE ( )  B_SPLINE_CURVE ( 3, ( #12038, #22625, #6717, #49769 ),
 .UNSPECIFIED., .F., .F. ) 
 B_SPLINE_CURVE_WITH_KNOTS ( ( 4, 4 ),
 ( 1.570796326794896558, 3.141592653589793116 ),
 .UNSPECIFIED. ) 
 CURVE ( )  GEOMETRIC_REPRESENTATION_ITEM ( )  RATIONAL_B_SPLINE_CURVE ( ( 1.000000000000000000, 0.8047378541243649375, 0.8047378541243649375, 1.000000000000000000 ) ) 
 REPRESENTATION_ITEM ( '' )  );
#3384=CARTESIAN_POINT ( 'NONE',  ( -46.69597344681494633, 1.750000000000009992, 160.8182875569279702 ) ) ;
#3385=ORIENTED_EDGE ( 'NONE', *, *, #3061, .T. ) ;
#3386=EDGE_CURVE ( 'NONE', #37650, #42224, #20834, .T. ) ;
#3387=FACE_OUTER_BOUND ( 'NONE', #9694, .T. ) ;
#3390=ORIENTED_EDGE ( 'NONE', *, *, #43963, .F. ) ;
#3391=CARTESIAN_POINT ( 'NONE',  ( 194.3291528190321742, -1.750000000000009326, 159.7931612910809065 ) ) ;
#3393=FACE_OUTER_BOUND ( 'NONE', #43556, .T. ) ;
#3397=ORIENTED_EDGE ( 'NONE', *, *, #26556, .F. ) ;
#3400=EDGE_CURVE ( 'NONE', #12850, #18090, #27783, .T. ) ;
#3401=ADVANCED_FACE ( 'NONE', ( #31656 ), #47243, .T. ) ;
#3403=ORIENTED_EDGE ( 'NONE', *, *, #36200, .T. ) ;
#3405=CARTESIAN_POINT ( 'NONE',  ( 194.3291528190321742, 1.750000000000010214, -120.2068387089191219 ) ) ;
#3406=CARTESIAN_POINT ( 'NONE',  ( -84.94597344681493212, 1.025126265847089657, -120.9317124430720440 ) ) ;
#3407=CARTESIAN_POINT ( 'NONE',  ( 35.05402655318504657, 1.025126265847089435, 39.06828755692797728 ) ) ;
#3410=EDGE_CURVE ( 'NONE', #47482, #16170, #16889, .T. ) ;
#3411=ORIENTED_EDGE ( 'NONE', *, *, #1446, .F. ) ;
#3414=CARTESIAN_POINT ( 'NONE',  ( 193.3040265531851105, -1.750000000000010658, 80.81828755692798438 ) ) ;
#3417=ORIENTED_EDGE ( 'NONE', *, *, #44305, .F. ) ;
#3423=CARTESIAN_POINT ( 'NONE',  ( 195.0540265531851105, 1.025126265847089435, 39.06828755692797728 ) ) ;
#3425=CARTESIAN_POINT ( 'NONE',  ( -6.695973446814940111, 1.750000000000023315, -159.1817124430720298 ) ) ;
#3430=FACE_OUTER_BOUND ( 'NONE', #20895, .T. ) ;
#3434=EDGE_CURVE ( 'NONE', #27788, #18915, #36228, .T. ) ;
#3436=CARTESIAN_POINT ( 'NONE',  ( 72.27890028733797578, -1.750000000000010214, -118.1565861772249519 ) ) ;
#3437=FACE_OUTER_BOUND ( 'NONE', #5296, .T. ) ;
#3443=ORIENTED_EDGE ( 'NONE', *, *, #1572, .T. ) ;
#3447=DIRECTION ( 'NONE',  ( -0.000000000000000000, -0.000000000000000000, -1.000000000000000000 ) ) ;
#3450=AXIS2_PLACEMENT_3D ( 'NONE', #20387, #43735, #48303 ) ;
#3455=ORIENTED_EDGE ( 'NONE', *, *, #583, .F. ) ;
#3456=EDGE_LOOP ( 'NONE', ( #18971, #34663, #41921, #30952, #6831 ) ) ;
#3458=CARTESIAN_POINT ( 'NONE',  ( -125.6708471809678542, -1.749999999999996225, -158.1565861772249377 ) ) ;
#3459=LINE ( 'NONE', #30426, #41439 ) ;
#3460=AXIS2_PLACEMENT_3D ( 'NONE', #21411, #21668, #25271 ) ;
#3461=ORIENTED_EDGE ( 'NONE', *, *, #26682, .F. ) ;
#3466=AXIS2_PLACEMENT_3D ( 'NONE', #31875, #4666, #47967 ) ;
#3469=ORIENTED_EDGE ( 'NONE', *, *, #35637, .F. ) ;
#3471=VECTOR ( 'NONE', #22284, 1000.000000000000000 ) ;
#3472=CARTESIAN_POINT ( 'NONE',  ( 155.0540265531850537, 2.143131898507880377E-16, 42.56828755692798438 ) ) ;
#3476=ORIENTED_EDGE ( 'NONE', *, *, #18614, .T. ) ;
#3477=ORIENTED_EDGE ( 'NONE', *, *, #34297, .F. ) ;
#3483=CYLINDRICAL_SURFACE ( 'NONE', #20815, 1.750000000000015543 ) ;
#3485=DIRECTION ( 'NONE',  ( -1.000000000000000000, -0.000000000000000000, -0.000000000000000000 ) ) ;
#3486=CARTESIAN_POINT ( 'NONE',  ( 191.5540265531850537, -1.025126265847089213, -160.9317124430720014 ) ) ;
#3488=CYLINDRICAL_SURFACE ( 'NONE', #46067, 1.750000000000010214 ) ;
#3489=CARTESIAN_POINT ( 'NONE',  ( 151.5540265531850537, -1.025126265847089657, -37.43171244307202272 ) ) ;
#3492=CARTESIAN_POINT ( 'NONE',  ( -124.9459734468149321, 1.025126265847081886, -120.9317124430720440 ) ) ;
#3493=ORIENTED_EDGE ( 'NONE', *, *, #41058, .F. ) ;
#3503=ORIENTED_EDGE ( 'NONE', *, *, #39131, .T. ) ;
#3513=ORIENTED_EDGE ( 'NONE', *, *, #2083, .F. ) ;
#3514=CARTESIAN_POINT ( 'NONE',  ( 210.0000000000000568, 0.000000000000000000, -117.4317124430720298 ) ) ;
#3515=( BOUNDED_CURVE ( )  B_SPLINE_CURVE ( 3, ( #39533, #4371, #3341, #35694 ),
 .UNSPECIFIED., .F., .F. ) 
 B_SPLINE_CURVE_WITH_KNOTS ( ( 4, 4 ),
 ( 0.000000000000000000, 1.570796326794896558 ),
 .UNSPECIFIED. ) 
 CURVE ( )  GEOMETRIC_REPRESENTATION_ITEM ( )  RATIONAL_B_SPLINE_CURVE ( ( 1.000000000000000000, 0.8047378541243649375, 0.8047378541243649375, 1.000000000000000000 ) ) 
 REPRESENTATION_ITEM ( '' )  );
#3518=FACE_OUTER_BOUND ( 'NONE', #45969, .T. ) ;
#3521=( BOUNDED_CURVE ( )  B_SPLINE_CURVE ( 3, ( #42759, #49673, #26109, #26627 ),
 .UNSPECIFIED., .F., .F. ) 
 B_SPLINE_CURVE_WITH_KNOTS ( ( 4, 4 ),
 ( 3.141592653589793116, 4.712388980384689674 ),
 .UNSPECIFIED. ) 
 CURVE ( )  GEOMETRIC_REPRESENTATION_ITEM ( )  RATIONAL_B_SPLINE_CURVE ( ( 1.000000000000000000, 0.8047378541243649375, 0.8047378541243649375, 1.000000000000000000 ) ) 
 REPRESENTATION_ITEM ( '' )  );
#3524=CARTESIAN_POINT ( 'NONE',  ( 193.3040265531851105, -1.750000000000010658, -79.18171244307201562 ) ) ;
#3530=DIRECTION ( 'NONE',  ( -1.000000000000000000, -0.000000000000000000, -0.000000000000000000 ) ) ;
#3533=ORIENTED_EDGE ( 'NONE', *, *, #48129, .F. ) ;
#3535=VECTOR ( 'NONE', #183, 1000.000000000000000 ) ;
#3538=( BOUNDED_CURVE ( )  B_SPLINE_CURVE ( 3, ( #19582, #31148, #31407, #7805 ),
 .UNSPECIFIED., .F., .F. ) 
 B_SPLINE_CURVE_WITH_KNOTS ( ( 4, 4 ),
 ( 0.000000000000000000, 1.570796326794896558 ),
 .UNSPECIFIED. ) 
 CURVE ( )  GEOMETRIC_REPRESENTATION_ITEM ( )  RATIONAL_B_SPLINE_CURVE ( ( 1.000000000000000000, 0.8047378541243649375, 0.8047378541243649375, 1.000000000000000000 ) ) 
 REPRESENTATION_ITEM ( '' )  );
#3539=CARTESIAN_POINT ( 'NONE',  ( 155.0540265531850537, 2.143131898507880377E-16, 2.568287556927978166 ) ) ;
#3540=ORIENTED_EDGE ( 'NONE', *, *, #31994, .T. ) ;
#3546=CARTESIAN_POINT ( 'NONE',  ( -48.44597344681495343, 0.000000000000000000, 42.56828755692798438 ) ) ;
#3548=CARTESIAN_POINT ( 'NONE',  ( 115.0540265531850395, 2.143131898507847836E-16, 165.0000000000000000 ) ) ;
#3549=CARTESIAN_POINT ( 'NONE',  ( -6.695973446814940111, 0.000000000000000000, 165.0000000000000000 ) ) ;
#3552=LINE ( 'NONE', #2549, #4333 ) ;
#3555=ORIENTED_EDGE ( 'NONE', *, *, #23846, .F. ) ;
#3557=CARTESIAN_POINT ( 'NONE',  ( -124.9459734468149321, 1.025126265847082108, 42.56828755692797017 ) ) ;
#3558=EDGE_CURVE ( 'NONE', #9513, #48877, #13873, .T. ) ;
#3560=AXIS2_PLACEMENT_3D ( 'NONE', #19131, #50398, #50133 ) ;
#3564=ADVANCED_FACE ( 'NONE', ( #32910 ), #1849, .T. ) ;
#3566=CARTESIAN_POINT ( 'NONE',  ( -6.695973446814940111, 0.000000000000000000, 165.0000000000000000 ) ) ;
#3571=ORIENTED_EDGE ( 'NONE', *, *, #46563, .T. ) ;
#3574=AXIS2_PLACEMENT_3D ( 'NONE', #44094, #9714, #41025 ) ;
#3575=ORIENTED_EDGE ( 'NONE', *, *, #33987, .T. ) ;
#3579=VERTEX_POINT ( 'NONE', #19246 ) ;
#3580=CARTESIAN_POINT ( 'NONE',  ( 195.0540265531851105, 2.143131898507880377E-16, 165.0000000000000000 ) ) ;
#3583=VECTOR ( 'NONE', #39264, 1000.000000000000000 ) ;
#3584=VECTOR ( 'NONE', #7170, 1000.000000000000000 ) ;
#3589=CYLINDRICAL_SURFACE ( 'NONE', #14230, 1.750000000000008438 ) ;
#3593=ADVANCED_FACE ( 'NONE', ( #38284 ), #14649, .T. ) ;
#3594=CARTESIAN_POINT ( 'NONE',  ( 210.0000000000000568, 0.000000000000000000, -119.1817124430720440 ) ) ;
#3596=ORIENTED_EDGE ( 'NONE', *, *, #40000, .F. ) ;
#3600=AXIS2_PLACEMENT_3D ( 'NONE', #9631, #36347, #24788 ) ;
#3601=ORIENTED_EDGE ( 'NONE', *, *, #19583, .F. ) ;
#3602=CARTESIAN_POINT ( 'NONE',  ( -165.6708471809677974, 1.750000000000009548, -38.15658617722494483 ) ) ;
#3604=ORIENTED_EDGE ( 'NONE', *, *, #46511, .T. ) ;
#3618=CARTESIAN_POINT ( 'NONE',  ( 113.3040265531850537, -1.749999999999996891, 0.8182875569279768335 ) ) ;
#3625=CARTESIAN_POINT ( 'NONE',  ( 33.30402655318503946, -1.750000000000010214, 40.81828755692798438 ) ) ;
#3631=CARTESIAN_POINT ( 'NONE',  ( 33.30402655318503946, 1.750000000000010214, -39.18171244307202983 ) ) ;
#3632=ORIENTED_EDGE ( 'NONE', *, *, #6372, .T. ) ;
#3635=EDGE_CURVE ( 'NONE', #21418, #28177, #4441, .T. ) ;
#3637=DIRECTION ( 'NONE',  ( -0.000000000000000000, -0.000000000000000000, -1.000000000000000000 ) ) ;
#3638=DIRECTION ( 'NONE',  ( -0.000000000000000000, -0.000000000000000000, -1.000000000000000000 ) ) ;
#3643=VERTEX_POINT ( 'NONE', #11055 ) ;
#3647=DIRECTION ( 'NONE',  ( -1.000000000000000000, 0.000000000000000000, 0.000000000000000000 ) ) ;
#3649=CARTESIAN_POINT ( 'NONE',  ( 114.3291528190321173, 1.749999999999996669, -0.2068387089191042749 ) ) ;
#3651=DIRECTION ( 'NONE',  ( -1.000000000000000000, -0.000000000000000000, -0.000000000000000000 ) ) ;
#3656=VECTOR ( 'NONE', #11629, 1000.000000000000000 ) ;
#3657=LINE ( 'NONE', #27273, #9833 ) ;
#3661=VECTOR ( 'NONE', #29191, 1000.000000000000000 ) ;
#3665=CARTESIAN_POINT ( 'NONE',  ( -85.67084718096784002, 1.750000000000010214, -120.2068387089191219 ) ) ;
#3666=CYLINDRICAL_SURFACE ( 'NONE', #23948, 1.750000000000010214 ) ;
#3667=ORIENTED_EDGE ( 'NONE', *, *, #20668, .T. ) ;
#3670=EDGE_CURVE ( 'NONE', #47848, #29172, #854, .T. ) ;
#3671=DIRECTION ( 'NONE',  ( 0.000000000000000000, 0.000000000000000000, 1.000000000000000000 ) ) ;
#3672=CARTESIAN_POINT ( 'NONE',  ( -84.94597344681494633, 2.143131898507880377E-16, 79.06828755692797017 ) ) ;
#3678=FACE_OUTER_BOUND ( 'NONE', #38951, .T. ) ;
#3682=ORIENTED_EDGE ( 'NONE', *, *, #40758, .T. ) ;
#3685=CARTESIAN_POINT ( 'NONE',  ( -164.9459734468149463, 2.143131898507880377E-16, 42.56828755692798438 ) ) ;
#3686=EDGE_LOOP ( 'NONE', ( #31338, #48065, #22159, #18658, #11705, #26828 ) ) ;
#3689=CARTESIAN_POINT ( 'NONE',  ( -84.94597344681493212, -1.025126265847089657, 119.0682875569279560 ) ) ;
#3697=CARTESIAN_POINT ( 'NONE',  ( 153.3040265531850537, 1.750000000000009992, -159.1817124430720298 ) ) ;
#3698=CARTESIAN_POINT ( 'NONE',  ( -86.69597344681494633, -1.750000000000010658, -79.18171244307201562 ) ) ;
#3699=( BOUNDED_CURVE ( )  B_SPLINE_CURVE ( 3, ( #37582, #49057, #40664, #36831 ),
 .UNSPECIFIED., .F., .F. ) 
 B_SPLINE_CURVE_WITH_KNOTS ( ( 4, 4 ),
 ( 4.712388980384689674, 6.283185307179586232 ),
 .UNSPECIFIED. ) 
 CURVE ( )  GEOMETRIC_REPRESENTATION_ITEM ( )  RATIONAL_B_SPLINE_CURVE ( ( 1.000000000000000000, 0.8047378541243649375, 0.8047378541243649375, 1.000000000000000000 ) ) 
 REPRESENTATION_ITEM ( '' )  );
#3701=DIRECTION ( 'NONE',  ( 1.000000000000000000, 0.000000000000000000, -0.000000000000000000 ) ) ;
#3704=EDGE_CURVE ( 'NONE', #40138, #34589, #22121, .T. ) ;
#3710=ADVANCED_FACE ( 'NONE', ( #31593 ), #47674, .T. ) ;
#3724=ORIENTED_EDGE ( 'NONE', *, *, #40212, .F. ) ;
#3726=DIRECTION ( 'NONE',  ( -1.000000000000000000, -0.000000000000000000, -0.000000000000000000 ) ) ;
#3727=DIRECTION ( 'NONE',  ( -0.000000000000000000, -0.000000000000000000, -1.000000000000000000 ) ) ;
#3736=LINE ( 'NONE', #46036, #47958 ) ;
#3744=FACE_OUTER_BOUND ( 'NONE', #19132, .T. ) ;
#3747=ORIENTED_EDGE ( 'NONE', *, *, #48586, .F. ) ;
#3748=ORIENTED_EDGE ( 'NONE', *, *, #9507, .F. ) ;
#3752=AXIS2_PLACEMENT_3D ( 'NONE', #18603, #34279, #3981 ) ;
#3755=CARTESIAN_POINT ( 'NONE',  ( -210.0000000000000568, 0.000000000000000000, -159.1817124430720298 ) ) ;
#3756=CARTESIAN_POINT ( 'NONE',  ( -167.7210997126620384, -1.750000000000010214, 81.84341382277507648 ) ) ;
#3759=LINE ( 'NONE', #47071, #12747 ) ;
#3764=DIRECTION ( 'NONE',  ( -1.000000000000000000, 0.000000000000000000, 0.000000000000000000 ) ) ;
#3765=EDGE_CURVE ( 'NONE', #9029, #24426, #18751, .T. ) ;
#3769=EDGE_CURVE ( 'NONE', #34589, #47864, #20467, .T. ) ;
#3775=CARTESIAN_POINT ( 'NONE',  ( -4.945973446814917018, -1.025126265847096763, 159.0682875569279418 ) ) ;
#3777=( BOUNDED_CURVE ( )  B_SPLINE_CURVE ( 3, ( #10523, #6424, #34159, #6670 ),
 .UNSPECIFIED., .F., .F. ) 
 B_SPLINE_CURVE_WITH_KNOTS ( ( 4, 4 ),
 ( 0.000000000000000000, 1.570796326794896558 ),
 .UNSPECIFIED. ) 
 CURVE ( )  GEOMETRIC_REPRESENTATION_ITEM ( )  RATIONAL_B_SPLINE_CURVE ( ( 1.000000000000000000, 0.8047378541243649375, 0.8047378541243649375, 1.000000000000000000 ) ) 
 REPRESENTATION_ITEM ( '' )  );
#3779=CARTESIAN_POINT ( 'NONE',  ( -44.94597344681493922, 2.143131898507880377E-16, 119.0682875569279702 ) ) ;
#3782=LINE ( 'NONE', #15587, #43815 ) ;
#3787=CARTESIAN_POINT ( 'NONE',  ( 195.0540265531851105, 2.143131898507880377E-16, 122.5682875569279702 ) ) ;
#3793=CARTESIAN_POINT ( 'NONE',  ( -8.445973446814914354, 2.143131898507880377E-16, -160.9317124430720298 ) ) ;
#3794=VERTEX_POINT ( 'NONE', #47429 ) ;
#3797=CARTESIAN_POINT ( 'NONE',  ( -6.695973446814940111, 1.750000000000024203, 120.8182875569279702 ) ) ;
#3799=AXIS2_PLACEMENT_3D ( 'NONE', #2716, #49862, #33290 ) ;
#3810=AXIS2_PLACEMENT_3D ( 'NONE', #5177, #32388, #4924 ) ;
#3814=CYLINDRICAL_SURFACE ( 'NONE', #23539, 1.749999999999973799 ) ;
#3815=CARTESIAN_POINT ( 'NONE',  ( 151.5540265531850537, 0.000000000000000000, -77.43171244307204404 ) ) ;
#3822=CARTESIAN_POINT ( 'NONE',  ( 210.0000000000000568, 2.143131898507881856E-16, 119.0682875569279560 ) ) ;
#3824=AXIS2_PLACEMENT_3D ( 'NONE', #35385, #15605, #19446 ) ;
#3825=CARTESIAN_POINT ( 'NONE',  ( 113.3040265531850537, 1.749999999999996891, 0.8182875569279768335 ) ) ;
#3826=CARTESIAN_POINT ( 'NONE',  ( -87.72109971266203843, -1.750000000000009548, -0.2068387089191121020 ) ) ;
#3831=CARTESIAN_POINT ( 'NONE',  ( -124.9459734468149605, 0.000000000000000000, 162.5682875569279702 ) ) ;
#3833=( BOUNDED_CURVE ( )  B_SPLINE_CURVE ( 3, ( #14959, #23667, #23425, #34732 ),
 .UNSPECIFIED., .F., .F. ) 
 B_SPLINE_CURVE_WITH_KNOTS ( ( 4, 4 ),
 ( 0.000000000000000000, 1.570796326794896780 ),
 .UNSPECIFIED. ) 
 CURVE ( )  GEOMETRIC_REPRESENTATION_ITEM ( )  RATIONAL_B_SPLINE_CURVE ( ( 1.000000000000000000, 0.8047378541243649375, 0.8047378541243649375, 1.000000000000000000 ) ) 
 REPRESENTATION_ITEM ( '' )  );
#3836=ORIENTED_EDGE ( 'NONE', *, *, #42791, .F. ) ;
#3842=( BOUNDED_CURVE ( )  B_SPLINE_CURVE ( 3, ( #18011, #29571, #2130, #29829 ),
 .UNSPECIFIED., .F., .F. ) 
 B_SPLINE_CURVE_WITH_KNOTS ( ( 4, 4 ),
 ( 0.000000000000000000, 1.570796326794896558 ),
 .UNSPECIFIED. ) 
 CURVE ( )  GEOMETRIC_REPRESENTATION_ITEM ( )  RATIONAL_B_SPLINE_CURVE ( ( 1.000000000000000000, 0.8047378541243649375, 0.8047378541243649375, 1.000000000000000000 ) ) 
 REPRESENTATION_ITEM ( '' )  );
#3843=ORIENTED_EDGE ( 'NONE', *, *, #5961, .T. ) ;
#3844=DIRECTION ( 'NONE',  ( -1.000000000000000000, 0.000000000000000000, 0.000000000000000000 ) ) ;
#3845=ORIENTED_EDGE ( 'NONE', *, *, #39163, .T. ) ;
#3848=ORIENTED_EDGE ( 'NONE', *, *, #25155, .F. ) ;
#3849=FACE_OUTER_BOUND ( 'NONE', #16334, .T. ) ;
#3862=LINE ( 'NONE', #7980, #39047 ) ;
#3864=ORIENTED_EDGE ( 'NONE', *, *, #28961, .F. ) ;
#3866=CARTESIAN_POINT ( 'NONE',  ( 210.0000000000000568, 2.143131898507881856E-16, 79.06828755692797017 ) ) ;
#3876=EDGE_LOOP ( 'NONE', ( #20562, #30762, #43189, #31382, #33457, #22011 ) ) ;
#3878=VERTEX_POINT ( 'NONE', #37218 ) ;
#3882=EDGE_CURVE ( 'NONE', #34400, #47251, #17126, .T. ) ;
#3885=CARTESIAN_POINT ( 'NONE',  ( 155.0540265531850537, 2.143131898507880377E-16, -120.9317124430720156 ) ) ;
#3887=CARTESIAN_POINT ( 'NONE',  ( -166.6959734468149463, 1.750000000000009992, 0.8182875569279768335 ) ) ;
#3890=CARTESIAN_POINT ( 'NONE',  ( -164.9459734468149463, 1.025126265847089435, 159.0682875569279418 ) ) ;
#3896=ORIENTED_EDGE ( 'NONE', *, *, #28398, .F. ) ;
#3899=ORIENTED_EDGE ( 'NONE', *, *, #28728, .F. ) ;
#3906=ORIENTED_EDGE ( 'NONE', *, *, #35697, .F. ) ;
#3909=DIRECTION ( 'NONE',  ( 0.000000000000000000, 0.000000000000000000, 1.000000000000000000 ) ) ;
#3912=ORIENTED_EDGE ( 'NONE', *, *, #48957, .T. ) ;
#3915=CARTESIAN_POINT ( 'NONE',  ( 210.0000000000000568, 0.000000000000000000, -79.18171244307201562 ) ) ;
#3922=CARTESIAN_POINT ( 'NONE',  ( 151.5540265531850537, 0.000000000000000000, 165.0000000000000000 ) ) ;
#3923=CARTESIAN_POINT ( 'NONE',  ( 34.32915281903212446, 1.750000000000009548, 39.79316129108089228 ) ) ;
#3924=ORIENTED_EDGE ( 'NONE', *, *, #37456, .T. ) ;
#3925=DIRECTION ( 'NONE',  ( -0.000000000000000000, -0.000000000000000000, -1.000000000000000000 ) ) ;
#3930=CARTESIAN_POINT ( 'NONE',  ( -126.6959734468149321, 0.000000000000000000, 165.0000000000000000 ) ) ;
#3933=AXIS2_PLACEMENT_3D ( 'NONE', #38935, #27118, #7620 ) ;
#3935=ORIENTED_EDGE ( 'NONE', *, *, #16714, .T. ) ;
#3937=CARTESIAN_POINT ( 'NONE',  ( -48.44597344681495343, 0.000000000000000000, 165.0000000000000000 ) ) ;
#3945=CARTESIAN_POINT ( 'NONE',  ( 75.05402655318509630, 2.143131898507880377E-16, 165.0000000000000000 ) ) ;
#3948=ADVANCED_FACE ( 'NONE', ( #28979 ), #44594, .T. ) ;
#3950=CYLINDRICAL_SURFACE ( 'NONE', #50286, 1.750000000000008438 ) ;
#3951=ORIENTED_EDGE ( 'NONE', *, *, #17445, .F. ) ;
#3952=ORIENTED_EDGE ( 'NONE', *, *, #48838, .T. ) ;
#3956=DIRECTION ( 'NONE',  ( 0.000000000000000000, 0.000000000000000000, 1.000000000000000000 ) ) ;
#3966=EDGE_CURVE ( 'NONE', #46337, #15022, #22288, .T. ) ;
#3971=VERTEX_POINT ( 'NONE', #34604 ) ;
#3974=( BOUNDED_CURVE ( )  B_SPLINE_CURVE ( 3, ( #31860, #30848, #39059, #23638 ),
 .UNSPECIFIED., .F., .F. ) 
 B_SPLINE_CURVE_WITH_KNOTS ( ( 4, 4 ),
 ( 4.712388980384689674, 6.283185307179586232 ),
 .UNSPECIFIED. ) 
 CURVE ( )  GEOMETRIC_REPRESENTATION_ITEM ( )  RATIONAL_B_SPLINE_CURVE ( ( 1.000000000000000000, 0.8047378541243649375, 0.8047378541243649375, 1.000000000000000000 ) ) 
 REPRESENTATION_ITEM ( '' )  );
#3977=ORIENTED_EDGE ( 'NONE', *, *, #44635, .T. ) ;
#3978=ORIENTED_EDGE ( 'NONE', *, *, #29078, .F. ) ;
#3981=DIRECTION ( 'NONE',  ( -1.000000000000000000, 0.000000000000000000, 0.000000000000000000 ) ) ;
#3983=ORIENTED_EDGE ( 'NONE', *, *, #21589, .F. ) ;
#3985=VERTEX_POINT ( 'NONE', #30000 ) ;
#3993=CARTESIAN_POINT ( 'NONE',  ( 33.30402655318503946, -1.750000000000010658, 80.81828755692798438 ) ) ;
#3997=DIRECTION ( 'NONE',  ( 0.000000000000000000, 0.000000000000000000, 1.000000000000000000 ) ) ;
#3999=EDGE_CURVE ( 'NONE', #45654, #40426, #19184, .T. ) ;
#4000=( BOUNDED_CURVE ( )  B_SPLINE_CURVE ( 3, ( #39859, #12622, #36258, #24450 ),
 .UNSPECIFIED., .F., .F. ) 
 B_SPLINE_CURVE_WITH_KNOTS ( ( 4, 4 ),
 ( 1.570796326794896558, 3.141592653589793116 ),
 .UNSPECIFIED. ) 
 CURVE ( )  GEOMETRIC_REPRESENTATION_ITEM ( )  RATIONAL_B_SPLINE_CURVE ( ( 1.000000000000000000, 0.8047378541243649375, 0.8047378541243649375, 1.000000000000000000 ) ) 
 REPRESENTATION_ITEM ( '' )  );
#4001=CARTESIAN_POINT ( 'NONE',  ( 112.2789002873379758, -1.749999999999996669, -0.2068387089191042749 ) ) ;
#4008=CARTESIAN_POINT ( 'NONE',  ( 210.0000000000000568, 2.143131898507881116E-16, -40.93171244307203693 ) ) ;
#4011=VECTOR ( 'NONE', #27751, 1000.000000000000000 ) ;
#4012=CARTESIAN_POINT ( 'NONE',  ( -86.69597344681496054, 0.000000000000000000, 165.0000000000000000 ) ) ;
#4017=LINE ( 'NONE', #19413, #46952 ) ;
#4031=ORIENTED_EDGE ( 'NONE', *, *, #39464, .F. ) ;
#4036=CARTESIAN_POINT ( 'NONE',  ( 195.0540265531851105, 1.025126265847089879, -117.4317124430720156 ) ) ;
#4038=ORIENTED_EDGE ( 'NONE', *, *, #49620, .T. ) ;
#4040=DIRECTION ( 'NONE',  ( -1.000000000000000000, -0.000000000000000000, -0.000000000000000000 ) ) ;
#4049=VECTOR ( 'NONE', #32562, 1000.000000000000000 ) ;
#4052=CARTESIAN_POINT ( 'NONE',  ( 73.30402655318508209, 1.750000000000010658, 120.8182875569279702 ) ) ;
#4058=VERTEX_POINT ( 'NONE', #2534 ) ;
#4059=DIRECTION ( 'NONE',  ( -1.000000000000000000, 0.000000000000000000, 0.000000000000000000 ) ) ;
#4068=ORIENTED_EDGE ( 'NONE', *, *, #9441, .T. ) ;
#4076=FACE_OUTER_BOUND ( 'NONE', #31892, .T. ) ;
#4079=CARTESIAN_POINT ( 'NONE',  ( 35.05402655318504657, 2.143131898507880377E-16, 119.0682875569279702 ) ) ;
#4083=VECTOR ( 'NONE', #46518, 1000.000000000000000 ) ;
#4084=( BOUNDED_CURVE ( )  B_SPLINE_CURVE ( 3, ( #29993, #38216, #10989, #45608 ),
 .UNSPECIFIED., .F., .F. ) 
 B_SPLINE_CURVE_WITH_KNOTS ( ( 4, 4 ),
 ( 3.141592653589793116, 4.712388980384689674 ),
 .UNSPECIFIED. ) 
 CURVE ( )  GEOMETRIC_REPRESENTATION_ITEM ( )  RATIONAL_B_SPLINE_CURVE ( ( 1.000000000000000000, 0.8047378541243649375, 0.8047378541243649375, 1.000000000000000000 ) ) 
 REPRESENTATION_ITEM ( '' )  );
#4087=ORIENTED_EDGE ( 'NONE', *, *, #15514, .T. ) ;
#4097=DIRECTION ( 'NONE',  ( 1.000000000000000000, 0.000000000000000000, 0.000000000000000000 ) ) ;
#4102=CARTESIAN_POINT ( 'NONE',  ( -48.44597344681495343, 0.000000000000000000, 165.0000000000000000 ) ) ;
#4108=DIRECTION ( 'NONE',  ( -0.000000000000000000, -0.000000000000000000, -1.000000000000000000 ) ) ;
#4111=CARTESIAN_POINT ( 'NONE',  ( -4.945973446814917018, 1.025126265847097429, -37.43171244307200851 ) ) ;
#4117=CARTESIAN_POINT ( 'NONE',  ( -210.0000000000000568, 0.000000000000000000, 162.5682875569279702 ) ) ;
#4119=VECTOR ( 'NONE', #6423, 1000.000000000000000 ) ;
#4122=AXIS2_PLACEMENT_3D ( 'NONE', #13723, #20925, #48072 ) ;
#4125=ORIENTED_EDGE ( 'NONE', *, *, #14574, .F. ) ;
#4126=CARTESIAN_POINT ( 'NONE',  ( -88.44597344681494633, 1.025126265847089213, -0.9317124430720324924 ) ) ;
#4131=ORIENTED_EDGE ( 'NONE', *, *, #9276, .F. ) ;
#4134=DIRECTION ( 'NONE',  ( 1.000000000000000000, 0.000000000000000000, 0.000000000000000000 ) ) ;
#4138=CARTESIAN_POINT ( 'NONE',  ( -85.67084718096784002, 1.750000000000009548, -160.2068387089191219 ) ) ;
#4144=( BOUNDED_CURVE ( )  B_SPLINE_CURVE ( 3, ( #21576, #10292, #37269, #41335 ),
 .UNSPECIFIED., .F., .F. ) 
 B_SPLINE_CURVE_WITH_KNOTS ( ( 4, 4 ),
 ( 1.570796326794896558, 3.141592653589793116 ),
 .UNSPECIFIED. ) 
 CURVE ( )  GEOMETRIC_REPRESENTATION_ITEM ( )  RATIONAL_B_SPLINE_CURVE ( ( 1.000000000000000000, 0.8047378541243649375, 0.8047378541243649375, 1.000000000000000000 ) ) 
 REPRESENTATION_ITEM ( '' )  );
#4148=CARTESIAN_POINT ( 'NONE',  ( -86.69597344681494633, 1.750000000000010658, -119.1817124430720440 ) ) ;
#4149=ORIENTED_EDGE ( 'NONE', *, *, #50255, .T. ) ;
#4151=( BOUNDED_CURVE ( )  B_SPLINE_CURVE ( 3, ( #39901, #7638, #15584, #46583 ),
 .UNSPECIFIED., .F., .F. ) 
 B_SPLINE_CURVE_WITH_KNOTS ( ( 4, 4 ),
 ( 4.712388980384689674, 6.283185307179586232 ),
 .UNSPECIFIED. ) 
 CURVE ( )  GEOMETRIC_REPRESENTATION_ITEM ( )  RATIONAL_B_SPLINE_CURVE ( ( 1.000000000000000000, 0.8047378541243649375, 0.8047378541243649375, 1.000000000000000000 ) ) 
 REPRESENTATION_ITEM ( '' )  );
#4155=AXIS2_PLACEMENT_3D ( 'NONE', #17900, #17664, #48915 ) ;
#4156=ORIENTED_EDGE ( 'NONE', *, *, #13284, .F. ) ;
#4157=VECTOR ( 'NONE', #45461, 1000.000000000000000 ) ;
#4158=CARTESIAN_POINT ( 'NONE',  ( 155.0540265531850537, 2.143131898507880377E-16, 159.0682875569279702 ) ) ;
#4162=CARTESIAN_POINT ( 'NONE',  ( -44.94597344681493922, 2.143131898507880377E-16, 165.0000000000000000 ) ) ;
#4166=CARTESIAN_POINT ( 'NONE',  ( 75.05402655318509630, 2.143131898507880377E-16, 42.56828755692799859 ) ) ;
#4175=CYLINDRICAL_SURFACE ( 'NONE', #39814, 1.750000000000001554 ) ;
#4176=EDGE_LOOP ( 'NONE', ( #8785, #33695, #17889, #30160, #42386, #35308 ) ) ;
#4177=ORIENTED_EDGE ( 'NONE', *, *, #34369, .F. ) ;
#4178=CARTESIAN_POINT ( 'NONE',  ( 111.5540265531850537, -1.025126265847082108, -117.4317124430720440 ) ) ;
#4181=CARTESIAN_POINT ( 'NONE',  ( -86.69597344681496054, 0.000000000000000000, 165.0000000000000000 ) ) ;
#4185=CARTESIAN_POINT ( 'NONE',  ( 195.0540265531851105, 1.025126265847089657, 79.06828755692797017 ) ) ;
#4195=ORIENTED_EDGE ( 'NONE', *, *, #29985, .F. ) ;
#4200=LINE ( 'NONE', #3937, #14220 ) ;
#4204=CARTESIAN_POINT ( 'NONE',  ( 191.5540265531850537, 1.025126265847089213, -0.9317124430720324924 ) ) ;
#4210=DIRECTION ( 'NONE',  ( -0.000000000000000000, -0.000000000000000000, -1.000000000000000000 ) ) ;
#4212=CARTESIAN_POINT ( 'NONE',  ( -168.4459734468149463, 0.000000000000000000, -117.4317124430720725 ) ) ;
#4215=ORIENTED_EDGE ( 'NONE', *, *, #39352, .T. ) ;
#4219=FACE_OUTER_BOUND ( 'NONE', #26773, .T. ) ;
#4220=EDGE_CURVE ( 'NONE', #2364, #50479, #6082, .T. ) ;
#4221=ADVANCED_FACE ( 'NONE', ( #27663 ), #23292, .T. ) ;
#4230=CARTESIAN_POINT ( 'NONE',  ( -165.6708471809677974, 1.750000000000009548, -158.1565861772249377 ) ) ;
#4238=EDGE_LOOP ( 'NONE', ( #17859, #49257, #27859, #523, #20517, #8561 ) ) ;
#4240=CARTESIAN_POINT ( 'NONE',  ( 153.3040265531850537, 0.000000000000000000, 165.0000000000000000 ) ) ;
#4248=DIRECTION ( 'NONE',  ( 0.000000000000000000, 0.000000000000000000, 1.000000000000000000 ) ) ;
#4249=ORIENTED_EDGE ( 'NONE', *, *, #27985, .F. ) ;
#4250=ORIENTED_EDGE ( 'NONE', *, *, #13132, .F. ) ;
#4251=ORIENTED_EDGE ( 'NONE', *, *, #40268, .F. ) ;
#4252=EDGE_CURVE ( 'NONE', #34485, #38451, #34569, .T. ) ;
#4253=ORIENTED_EDGE ( 'NONE', *, *, #26768, .T. ) ;
#4258=LINE ( 'NONE', #31728, #46709 ) ;
#4261=FACE_OUTER_BOUND ( 'NONE', #9905, .T. ) ;
#4267=ORIENTED_EDGE ( 'NONE', *, *, #38433, .T. ) ;
#4271=VECTOR ( 'NONE', #567, 1000.000000000000000 ) ;
#4272=EDGE_CURVE ( 'NONE', #27650, #39465, #17370, .T. ) ;
#4279=EDGE_CURVE ( 'NONE', #17107, #19110, #46657, .T. ) ;
#4280=EDGE_CURVE ( 'NONE', #23932, #38451, #17620, .T. ) ;
#4286=ADVANCED_FACE ( 'NONE', ( #45046 ), #48875, .T. ) ;
#4287=( BOUNDED_CURVE ( )  B_SPLINE_CURVE ( 3, ( #46835, #31496, #30991, #11729 ),
 .UNSPECIFIED., .F., .F. ) 
 B_SPLINE_CURVE_WITH_KNOTS ( ( 4, 4 ),
 ( 0.000000000000000000, 1.570796326794896780 ),
 .UNSPECIFIED. ) 
 CURVE ( )  GEOMETRIC_REPRESENTATION_ITEM ( )  RATIONAL_B_SPLINE_CURVE ( ( 1.000000000000000000, 0.8047378541243649375, 0.8047378541243649375, 1.000000000000000000 ) ) 
 REPRESENTATION_ITEM ( '' )  );
#4288=ORIENTED_EDGE ( 'NONE', *, *, #778, .F. ) ;
#4289=CARTESIAN_POINT ( 'NONE',  ( 153.3040265531850537, 0.000000000000000000, 165.0000000000000000 ) ) ;
#4291=ORIENTED_EDGE ( 'NONE', *, *, #40242, .T. ) ;
#4293=CARTESIAN_POINT ( 'NONE',  ( 210.0000000000000568, 0.000000000000000000, -157.4317124430720298 ) ) ;
#4294=( BOUNDED_CURVE ( )  B_SPLINE_CURVE ( 3, ( #13777, #40240, #48391, #28937 ),
 .UNSPECIFIED., .F., .F. ) 
 B_SPLINE_CURVE_WITH_KNOTS ( ( 4, 4 ),
 ( 1.570796326794896558, 3.141592653589793116 ),
 .UNSPECIFIED. ) 
 CURVE ( )  GEOMETRIC_REPRESENTATION_ITEM ( )  RATIONAL_B_SPLINE_CURVE ( ( 1.000000000000000000, 0.8047378541243649375, 0.8047378541243649375, 1.000000000000000000 ) ) 
 REPRESENTATION_ITEM ( '' )  );
#4295=AXIS2_PLACEMENT_3D ( 'NONE', #31411, #34496, #46745 ) ;
#4296=ORIENTED_EDGE ( 'NONE', *, *, #23738, .F. ) ;
#4297=CARTESIAN_POINT ( 'NONE',  ( -164.9459734468149463, -1.025126265847089435, -40.93171244307204404 ) ) ;
#4299=ORIENTED_EDGE ( 'NONE', *, *, #6752, .F. ) ;
#4302=CARTESIAN_POINT ( 'NONE',  ( 113.3040265531850537, 0.000000000000000000, 165.0000000000000000 ) ) ;
#4308=( BOUNDED_CURVE ( )  B_SPLINE_CURVE ( 3, ( #44547, #5577, #21232, #17383 ),
 .UNSPECIFIED., .F., .F. ) 
 B_SPLINE_CURVE_WITH_KNOTS ( ( 4, 4 ),
 ( 1.570796326794896558, 3.141592653589793116 ),
 .UNSPECIFIED. ) 
 CURVE ( )  GEOMETRIC_REPRESENTATION_ITEM ( )  RATIONAL_B_SPLINE_CURVE ( ( 1.000000000000000000, 0.8047378541243649375, 0.8047378541243649375, 1.000000000000000000 ) ) 
 REPRESENTATION_ITEM ( '' )  );
#4316=CARTESIAN_POINT ( 'NONE',  ( 210.0000000000000568, 2.143131898507881116E-16, 39.06828755692797728 ) ) ;
#4318=ORIENTED_EDGE ( 'NONE', *, *, #1857, .T. ) ;
#4321=LINE ( 'NONE', #7154, #18025 ) ;
#4322=VECTOR ( 'NONE', #22280, 1000.000000000000000 ) ;
#4324=ORIENTED_EDGE ( 'NONE', *, *, #13583, .F. ) ;
#4327=FACE_OUTER_BOUND ( 'NONE', #11889, .T. ) ;
#4333=VECTOR ( 'NONE', #6399, 1000.000000000000000 ) ;
#4334=CARTESIAN_POINT ( 'NONE',  ( -4.945973446814917018, 1.025126265847096985, -0.9317124430720461481 ) ) ;
#4339=CARTESIAN_POINT ( 'NONE',  ( -124.9459734468149463, 2.143131898507847836E-16, 42.56828755692795596 ) ) ;
#4342=CARTESIAN_POINT ( 'NONE',  ( -205.6708471809678827, -1.750000000000009548, 39.79316129108089228 ) ) ;
#4343=CARTESIAN_POINT ( 'NONE',  ( 153.3040265531850537, 1.750000000000010658, 120.8182875569279702 ) ) ;
#4358=CARTESIAN_POINT ( 'NONE',  ( 75.05402655318509630, 2.143131898507880377E-16, -40.93171244307205825 ) ) ;
#4360=EDGE_CURVE ( 'NONE', #36853, #40426, #11940, .T. ) ;
#4361=VERTEX_POINT ( 'NONE', #26338 ) ;
#4365=CYLINDRICAL_SURFACE ( 'NONE', #11434, 1.750000000000008438 ) ;
#4366=CARTESIAN_POINT ( 'NONE',  ( -84.94597344681494633, 2.143131898507880377E-16, 122.5682875569279702 ) ) ;
#4367=ORIENTED_EDGE ( 'NONE', *, *, #12538, .F. ) ;
#4368=DIRECTION ( 'NONE',  ( 0.000000000000000000, 0.000000000000000000, 1.000000000000000000 ) ) ;
#4369=CARTESIAN_POINT ( 'NONE',  ( -5.670847180967843570, 1.750000000000023315, -38.15658617722493062 ) ) ;
#4370=DIRECTION ( 'NONE',  ( -1.000000000000000000, -0.000000000000000000, -0.000000000000000000 ) ) ;
#4371=CARTESIAN_POINT ( 'NONE',  ( -88.44597344681494633, -1.025126265847089213, 162.5682875569279133 ) ) ;
#4386=EDGE_LOOP ( 'NONE', ( #15931, #16609, #44113, #2724, #14117 ) ) ;
#4387=( BOUNDED_CURVE ( )  B_SPLINE_CURVE ( 3, ( #45771, #6555, #25809, #21695 ),
 .UNSPECIFIED., .F., .F. ) 
 B_SPLINE_CURVE_WITH_KNOTS ( ( 4, 4 ),
 ( 4.712388980384689674, 6.283185307179586232 ),
 .UNSPECIFIED. ) 
 CURVE ( )  GEOMETRIC_REPRESENTATION_ITEM ( )  RATIONAL_B_SPLINE_CURVE ( ( 1.000000000000000000, 0.8047378541243649375, 0.8047378541243649375, 1.000000000000000000 ) ) 
 REPRESENTATION_ITEM ( '' )  );
#4388=FACE_OUTER_BOUND ( 'NONE', #1120, .T. ) ;
#4401=AXIS2_PLACEMENT_3D ( 'NONE', #11536, #38995, #14870 ) ;
#4403=CARTESIAN_POINT ( 'NONE',  ( -166.6959734468149463, 1.750000000000009992, 160.8182875569279702 ) ) ;
#4408=CARTESIAN_POINT ( 'NONE',  ( 191.5540265531851105, 0.000000000000000000, 119.0682875569279702 ) ) ;
#4411=ORIENTED_EDGE ( 'NONE', *, *, #29292, .T. ) ;
#4415=CARTESIAN_POINT ( 'NONE',  ( 31.55402655318503236, 0.000000000000000000, 165.0000000000000000 ) ) ;
#4416=CARTESIAN_POINT ( 'NONE',  ( -4.945973446814917018, -1.025126265847096763, -157.4317124430720014 ) ) ;
#4419=LINE ( 'NONE', #43404, #4847 ) ;
#4423=CARTESIAN_POINT ( 'NONE',  ( -4.945973446814903696, 2.143131898507912917E-16, -160.9317124430720582 ) ) ;
#4424=CARTESIAN_POINT ( 'NONE',  ( 210.0000000000000568, 0.000000000000000000, -117.4317124430720298 ) ) ;
#4428=CARTESIAN_POINT ( 'NONE',  ( 155.0540265531850537, 1.025126265847089435, -40.93171244307204404 ) ) ;
#4429=ORIENTED_EDGE ( 'NONE', *, *, #28643, .T. ) ;
#4430=CARTESIAN_POINT ( 'NONE',  ( 193.3040265531851105, 1.750000000000010658, -79.18171244307201562 ) ) ;
#4432=AXIS2_PLACEMENT_3D ( 'NONE', #2095, #16985, #13124 ) ;
#4441=( BOUNDED_CURVE ( )  B_SPLINE_CURVE ( 3, ( #14906, #38777, #45917, #33911 ),
 .UNSPECIFIED., .F., .F. ) 
 B_SPLINE_CURVE_WITH_KNOTS ( ( 4, 4 ),
 ( 4.712388980384689674, 6.283185307179586232 ),
 .UNSPECIFIED. ) 
 CURVE ( )  GEOMETRIC_REPRESENTATION_ITEM ( )  RATIONAL_B_SPLINE_CURVE ( ( 1.000000000000000000, 0.8047378541243649375, 0.8047378541243649375, 1.000000000000000000 ) ) 
 REPRESENTATION_ITEM ( '' )  );
#4446=VERTEX_POINT ( 'NONE', #10929 ) ;
#4449=( BOUNDED_CURVE ( )  B_SPLINE_CURVE ( 3, ( #49921, #38208, #6880, #2266 ),
 .UNSPECIFIED., .F., .F. ) 
 B_SPLINE_CURVE_WITH_KNOTS ( ( 4, 4 ),
 ( 4.712388980384689674, 6.283185307179586232 ),
 .UNSPECIFIED. ) 
 CURVE ( )  GEOMETRIC_REPRESENTATION_ITEM ( )  RATIONAL_B_SPLINE_CURVE ( ( 1.000000000000000000, 0.8047378541243649375, 0.8047378541243649375, 1.000000000000000000 ) ) 
 REPRESENTATION_ITEM ( '' )  );
#4456=CARTESIAN_POINT ( 'NONE',  ( -8.445973446814964092, 1.025126265847097207, -117.4317124430720014 ) ) ;
#4462=VERTEX_POINT ( 'NONE', #30698 ) ;
#4464=CARTESIAN_POINT ( 'NONE',  ( 153.3040265531850537, 0.000000000000000000, 165.0000000000000000 ) ) ;
#4467=CARTESIAN_POINT ( 'NONE',  ( -84.94597344681494633, 2.143131898507880377E-16, -117.4317124430720725 ) ) ;
#4468=ORIENTED_EDGE ( 'NONE', *, *, #31539, .T. ) ;
#4471=CARTESIAN_POINT ( 'NONE',  ( -168.4459734468149463, 0.000000000000000000, 119.0682875569279702 ) ) ;
#4480=ORIENTED_EDGE ( 'NONE', *, *, #45948, .F. ) ;
#4486=VERTEX_POINT ( 'NONE', #8611 ) ;
#4492=CARTESIAN_POINT ( 'NONE',  ( 111.5540265531850537, -1.025126265847081886, -120.9317124430720440 ) ) ;
#4496=ORIENTED_EDGE ( 'NONE', *, *, #7218, .F. ) ;
#4498=EDGE_CURVE ( 'NONE', #4914, #35123, #27673, .T. ) ;
#4501=ORIENTED_EDGE ( 'NONE', *, *, #7966, .F. ) ;
#4502=EDGE_CURVE ( 'NONE', #26902, #39708, #9681, .T. ) ;
#4504=VECTOR ( 'NONE', #50122, 1000.000000000000000 ) ;
#4505=ORIENTED_EDGE ( 'NONE', *, *, #18934, .T. ) ;
#4510=CARTESIAN_POINT ( 'NONE',  ( -210.0000000000000568, 0.000000000000000000, 42.56828755692799149 ) ) ;
#4512=ORIENTED_EDGE ( 'NONE', *, *, #15506, .T. ) ;
#4522=CARTESIAN_POINT ( 'NONE',  ( 191.5540265531851105, 0.000000000000000000, -120.9317124430720156 ) ) ;
#4531=ADVANCED_FACE ( 'NONE', ( #39165 ), #15798, .T. ) ;
#4537=CARTESIAN_POINT ( 'NONE',  ( 195.0540265531851105, -1.025126265847089435, 162.5682875569279133 ) ) ;
#4540=CARTESIAN_POINT ( 'NONE',  ( 155.0540265531850537, -1.025126265847089435, -40.93171244307204404 ) ) ;
#4541=DIRECTION ( 'NONE',  ( -0.000000000000000000, -0.000000000000000000, -1.000000000000000000 ) ) ;
#4546=ORIENTED_EDGE ( 'NONE', *, *, #21898, .T. ) ;
#4547=AXIS2_PLACEMENT_3D ( 'NONE', #42677, #42422, #34242 ) ;
#4549=CARTESIAN_POINT ( 'NONE',  ( -7.721099712662037540, 1.750000000000023981, 79.79316129108087807 ) ) ;
#4553=EDGE_CURVE ( 'NONE', #9206, #40841, #39922, .T. ) ;
#4557=ORIENTED_EDGE ( 'NONE', *, *, #39805, .T. ) ;
#4558=CYLINDRICAL_SURFACE ( 'NONE', #31592, 1.750000000000015543 ) ;
#4562=ORIENTED_EDGE ( 'NONE', *, *, #29967, .T. ) ;
#4574=CARTESIAN_POINT ( 'NONE',  ( 35.05402655318504657, 2.143131898507880377E-16, 119.0682875569279702 ) ) ;
#4575=ORIENTED_EDGE ( 'NONE', *, *, #34002, .T. ) ;
#4576=CARTESIAN_POINT ( 'NONE',  ( -45.67084718096785423, -1.750000000000009548, 121.8434138227750623 ) ) ;
#4584=CARTESIAN_POINT ( 'NONE',  ( -84.94597344681493212, -1.025126265847089435, 39.06828755692797728 ) ) ;
#4592=( BOUNDED_CURVE ( )  B_SPLINE_CURVE ( 3, ( #3296, #44920, #11007, #7163 ),
 .UNSPECIFIED., .F., .F. ) 
 B_SPLINE_CURVE_WITH_KNOTS ( ( 4, 4 ),
 ( 1.570796326794896558, 3.141592653589793116 ),
 .UNSPECIFIED. ) 
 CURVE ( )  GEOMETRIC_REPRESENTATION_ITEM ( )  RATIONAL_B_SPLINE_CURVE ( ( 1.000000000000000000, 0.8047378541243649375, 0.8047378541243649375, 1.000000000000000000 ) ) 
 REPRESENTATION_ITEM ( '' )  );
#4595=CARTESIAN_POINT ( 'NONE',  ( 151.5540265531850537, 0.000000000000000000, 119.0682875569279702 ) ) ;
#4598=( BOUNDED_CURVE ( )  B_SPLINE_CURVE ( 3, ( #5970, #18013, #37310, #29077 ),
 .UNSPECIFIED., .F., .F. ) 
 B_SPLINE_CURVE_WITH_KNOTS ( ( 4, 4 ),
 ( 4.712388980384689674, 6.283185307179586232 ),
 .UNSPECIFIED. ) 
 CURVE ( )  GEOMETRIC_REPRESENTATION_ITEM ( )  RATIONAL_B_SPLINE_CURVE ( ( 1.000000000000000000, 0.8047378541243649375, 0.8047378541243649375, 1.000000000000000000 ) ) 
 REPRESENTATION_ITEM ( '' )  );
#4607=AXIS2_PLACEMENT_3D ( 'NONE', #14913, #45676, #34685 ) ;
#4611=EDGE_CURVE ( 'NONE', #11124, #41652, #20908, .T. ) ;
#4613=( BOUNDED_CURVE ( )  B_SPLINE_CURVE ( 3, ( #48134, #37168, #47888, #32552 ),
 .UNSPECIFIED., .F., .F. ) 
 B_SPLINE_CURVE_WITH_KNOTS ( ( 4, 4 ),
 ( 1.570796326794896558, 3.141592653589793116 ),
 .UNSPECIFIED. ) 
 CURVE ( )  GEOMETRIC_REPRESENTATION_ITEM ( )  RATIONAL_B_SPLINE_CURVE ( ( 1.000000000000000000, 0.8047378541243649375, 0.8047378541243649375, 1.000000000000000000 ) ) 
 REPRESENTATION_ITEM ( '' )  );
#4615=FACE_OUTER_BOUND ( 'NONE', #17247, .T. ) ;
#4616=EDGE_LOOP ( 'NONE', ( #23040, #33537, #3836, #29847, #40588, #31326 ) ) ;
#4618=CARTESIAN_POINT ( 'NONE',  ( -206.6959734468149463, 1.750000000000010658, 120.8182875569279702 ) ) ;
#4625=ORIENTED_EDGE ( 'NONE', *, *, #39462, .T. ) ;
#4627=CARTESIAN_POINT ( 'NONE',  ( -84.94597344681494633, 2.143131898507880377E-16, -117.4317124430720725 ) ) ;
#4628=EDGE_CURVE ( 'NONE', #6245, #49119, #32621, .T. ) ;
#4629=VERTEX_POINT ( 'NONE', #44485 ) ;
#4630=EDGE_CURVE ( 'NONE', #45663, #44427, #43389, .T. ) ;
#4637=VERTEX_POINT ( 'NONE', #6213 ) ;
#4638=CARTESIAN_POINT ( 'NONE',  ( -45.67084718096785423, 1.750000000000010214, 79.79316129108087807 ) ) ;
#4640=CARTESIAN_POINT ( 'NONE',  ( 71.55402655318505367, 1.025126265847089213, 159.0682875569279418 ) ) ;
#4646=CARTESIAN_POINT ( 'NONE',  ( -45.67084718096785423, 1.750000000000010214, 119.7931612910808781 ) ) ;
#4652=ORIENTED_EDGE ( 'NONE', *, *, #34626, .F. ) ;
#4658=CARTESIAN_POINT ( 'NONE',  ( 210.0000000000000568, 0.000000000000000000, -119.1817124430720440 ) ) ;
#4659=ORIENTED_EDGE ( 'NONE', *, *, #4896, .F. ) ;
#4665=ORIENTED_EDGE ( 'NONE', *, *, #2071, .F. ) ;
#4666=DIRECTION ( 'NONE',  ( -0.000000000000000000, -0.000000000000000000, -1.000000000000000000 ) ) ;
#4669=ORIENTED_EDGE ( 'NONE', *, *, #3120, .T. ) ;
#4677=AXIS2_PLACEMENT_3D ( 'NONE', #39477, #43554, #27409 ) ;
#4678=CARTESIAN_POINT ( 'NONE',  ( 210.0000000000000568, 0.000000000000000000, 162.5682875569279702 ) ) ;
#4681=FACE_OUTER_BOUND ( 'NONE', #374, .T. ) ;
#4683=FACE_OUTER_BOUND ( 'NONE', #36084, .T. ) ;
#4688=EDGE_LOOP ( 'NONE', ( #31087, #510, #30808, #41552, #18648 ) ) ;
#4690=LINE ( 'NONE', #20581, #6917 ) ;
#4692=FACE_OUTER_BOUND ( 'NONE', #35270, .T. ) ;
#4693=( BOUNDED_CURVE ( )  B_SPLINE_CURVE ( 3, ( #49650, #49400, #34067, #14541 ),
 .UNSPECIFIED., .F., .F. ) 
 B_SPLINE_CURVE_WITH_KNOTS ( ( 4, 4 ),
 ( 0.000000000000000000, 1.570796326794896558 ),
 .UNSPECIFIED. ) 
 CURVE ( )  GEOMETRIC_REPRESENTATION_ITEM ( )  RATIONAL_B_SPLINE_CURVE ( ( 1.000000000000000000, 0.8047378541243649375, 0.8047378541243649375, 1.000000000000000000 ) ) 
 REPRESENTATION_ITEM ( '' )  );
#4696=FACE_OUTER_BOUND ( 'NONE', #34839, .T. ) ;
#4698=EDGE_CURVE ( 'NONE', #22032, #7355, #20172, .T. ) ;
#4701=ORIENTED_EDGE ( 'NONE', *, *, #19984, .T. ) ;
#4706=CARTESIAN_POINT ( 'NONE',  ( -8.445973446814976526, 0.000000000000000000, 82.56828755692801280 ) ) ;
#4707=ORIENTED_EDGE ( 'NONE', *, *, #3110, .F. ) ;
#4708=CARTESIAN_POINT ( 'NONE',  ( 191.5540265531851105, 0.000000000000000000, -0.9317124430720247208 ) ) ;
#4714=CARTESIAN_POINT ( 'NONE',  ( -8.445973446814976526, 0.000000000000000000, -117.4317124430720156 ) ) ;
#4715=DIRECTION ( 'NONE',  ( -0.000000000000000000, -0.000000000000000000, -1.000000000000000000 ) ) ;
#4716=AXIS2_PLACEMENT_3D ( 'NONE', #19387, #50389, #27611 ) ;
#4727=CARTESIAN_POINT ( 'NONE',  ( -208.4459734468149463, 0.000000000000000000, -117.4317124430720725 ) ) ;
#4734=VERTEX_POINT ( 'NONE', #39 ) ;
#4738=( BOUNDED_CURVE ( )  B_SPLINE_CURVE ( 3, ( #19204, #23319, #43070, #6915 ),
 .UNSPECIFIED., .F., .F. ) 
 B_SPLINE_CURVE_WITH_KNOTS ( ( 4, 4 ),
 ( 3.141592653589793116, 4.712388980384689674 ),
 .UNSPECIFIED. ) 
 CURVE ( )  GEOMETRIC_REPRESENTATION_ITEM ( )  RATIONAL_B_SPLINE_CURVE ( ( 1.000000000000000000, 0.8047378541243649375, 0.8047378541243649375, 1.000000000000000000 ) ) 
 REPRESENTATION_ITEM ( '' )  );
#4739=AXIS2_PLACEMENT_3D ( 'NONE', #47067, #15047, #11972 ) ;
#4744=CARTESIAN_POINT ( 'NONE',  ( 192.2789002873380184, -1.750000000000010214, -78.15658617722490931 ) ) ;
#4745=CYLINDRICAL_SURFACE ( 'NONE', #3450, 1.750000000000001554 ) ;
#4747=ORIENTED_EDGE ( 'NONE', *, *, #2101, .F. ) ;
#4749=( BOUNDED_CURVE ( )  B_SPLINE_CURVE ( 3, ( #9787, #33173, #25707, #48753 ),
 .UNSPECIFIED., .F., .F. ) 
 B_SPLINE_CURVE_WITH_KNOTS ( ( 4, 4 ),
 ( 4.712388980384689674, 6.283185307179586232 ),
 .UNSPECIFIED. ) 
 CURVE ( )  GEOMETRIC_REPRESENTATION_ITEM ( )  RATIONAL_B_SPLINE_CURVE ( ( 1.000000000000000000, 0.8047378541243649375, 0.8047378541243649375, 1.000000000000000000 ) ) 
 REPRESENTATION_ITEM ( '' )  );
#4753=ORIENTED_EDGE ( 'NONE', *, *, #43004, .T. ) ;
#4756=DIRECTION ( 'NONE',  ( 0.000000000000000000, 0.000000000000000000, 1.000000000000000000 ) ) ;
#4761=CARTESIAN_POINT ( 'NONE',  ( -124.9459734468149321, 1.025126265847081886, 79.06828755692797017 ) ) ;
#4764=CARTESIAN_POINT ( 'NONE',  ( -84.94597344681493212, -1.025126265847089213, -160.9317124430720014 ) ) ;
#4771=VECTOR ( 'NONE', #14422, 1000.000000000000000 ) ;
#4777=CARTESIAN_POINT ( 'NONE',  ( 155.0540265531850537, 2.143131898507880377E-16, 42.56828755692798438 ) ) ;
#4778=VERTEX_POINT ( 'NONE', #15671 ) ;
#4781=ORIENTED_EDGE ( 'NONE', *, *, #20610, .T. ) ;
#4790=VERTEX_POINT ( 'NONE', #31079 ) ;
#4797=CIRCLE ( 'NONE', #38417, 1.750000000000015543 ) ;
#4800=CARTESIAN_POINT ( 'NONE',  ( 75.05402655318509630, 2.143131898507880377E-16, 122.5682875569279844 ) ) ;
#4802=VERTEX_POINT ( 'NONE', #42603 ) ;
#4803=VERTEX_POINT ( 'NONE', #7484 ) ;
#4804=CARTESIAN_POINT ( 'NONE',  ( -86.69597344681494633, 1.750000000000010658, 80.81828755692798438 ) ) ;
#4805=EDGE_CURVE ( 'NONE', #46904, #16166, #23114, .T. ) ;
#4807=ORIENTED_EDGE ( 'NONE', *, *, #8704, .T. ) ;
#4809=DIRECTION ( 'NONE',  ( 1.000000000000000000, 0.000000000000000000, 0.000000000000000000 ) ) ;
#4812=CARTESIAN_POINT ( 'NONE',  ( -124.9459734468149463, 2.143131898507847836E-16, 82.56828755692797017 ) ) ;
#4813=CARTESIAN_POINT ( 'NONE',  ( 34.32915281903212446, 1.750000000000009548, -160.2068387089191219 ) ) ;
#4815=DIRECTION ( 'NONE',  ( -0.000000000000000000, -0.000000000000000000, -1.000000000000000000 ) ) ;
#4817=CARTESIAN_POINT ( 'NONE',  ( 33.30402655318503946, -1.750000000000010658, 80.81828755692798438 ) ) ;
#4822=DIRECTION ( 'NONE',  ( -1.000000000000000000, -0.000000000000000000, -0.000000000000000000 ) ) ;
#4825=EDGE_CURVE ( 'NONE', #15344, #37516, #44243, .T. ) ;
#4834=DIRECTION ( 'NONE',  ( 1.000000000000000000, 0.000000000000000000, 0.000000000000000000 ) ) ;
#4836=ORIENTED_EDGE ( 'NONE', *, *, #41224, .T. ) ;
#4837=EDGE_CURVE ( 'NONE', #30887, #12850, #27733, .T. ) ;
#4845=VERTEX_POINT ( 'NONE', #15935 ) ;
#4847=VECTOR ( 'NONE', #50043, 1000.000000000000000 ) ;
#4855=CARTESIAN_POINT ( 'NONE',  ( 111.5540265531850679, 0.000000000000000000, -37.43171244307205825 ) ) ;
#4862=FACE_OUTER_BOUND ( 'NONE', #30834, .T. ) ;
#4863=ORIENTED_EDGE ( 'NONE', *, *, #49340, .F. ) ;
#4864=CARTESIAN_POINT ( 'NONE',  ( 210.0000000000000568, 0.000000000000000000, -77.43171244307200141 ) ) ;
#4868=DIRECTION ( 'NONE',  ( -0.000000000000000000, -0.000000000000000000, -1.000000000000000000 ) ) ;
#4872=( BOUNDED_CURVE ( )  B_SPLINE_CURVE ( 3, ( #602, #4185, #43667, #90 ),
 .UNSPECIFIED., .F., .F. ) 
 B_SPLINE_CURVE_WITH_KNOTS ( ( 4, 4 ),
 ( 0.000000000000000000, 1.570796326794896558 ),
 .UNSPECIFIED. ) 
 CURVE ( )  GEOMETRIC_REPRESENTATION_ITEM ( )  RATIONAL_B_SPLINE_CURVE ( ( 1.000000000000000000, 0.8047378541243649375, 0.8047378541243649375, 1.000000000000000000 ) ) 
 REPRESENTATION_ITEM ( '' )  );
#4874=VERTEX_POINT ( 'NONE', #43619 ) ;
#4875=DIRECTION ( 'NONE',  ( 1.000000000000000000, 0.000000000000000000, 0.000000000000000000 ) ) ;
#4877=EDGE_CURVE ( 'NONE', #47806, #36821, #293, .T. ) ;
#4889=DIRECTION ( 'NONE',  ( 1.000000000000000000, 0.000000000000000000, 0.000000000000000000 ) ) ;
#4892=( BOUNDED_CURVE ( )  B_SPLINE_CURVE ( 3, ( #12322, #1040, #4638, #20281 ),
 .UNSPECIFIED., .F., .F. ) 
 B_SPLINE_CURVE_WITH_KNOTS ( ( 4, 4 ),
 ( 0.000000000000000000, 1.570796326794896558 ),
 .UNSPECIFIED. ) 
 CURVE ( )  GEOMETRIC_REPRESENTATION_ITEM ( )  RATIONAL_B_SPLINE_CURVE ( ( 1.000000000000000000, 0.8047378541243649375, 0.8047378541243649375, 1.000000000000000000 ) ) 
 REPRESENTATION_ITEM ( '' )  );
#4893=CARTESIAN_POINT ( 'NONE',  ( -204.9459734468148895, -1.025126265847088991, 162.5682875569279133 ) ) ;
#4895=CARTESIAN_POINT ( 'NONE',  ( 155.0540265531850537, 2.143131898507880377E-16, -80.93171244307201562 ) ) ;
#4896=EDGE_CURVE ( 'NONE', #49775, #46959, #16678, .T. ) ;
#4897=VERTEX_POINT ( 'NONE', #31604 ) ;
#4899=ORIENTED_EDGE ( 'NONE', *, *, #42974, .T. ) ;
#4902=CARTESIAN_POINT ( 'NONE',  ( 155.0540265531850537, 1.025126265847089657, 119.0682875569279560 ) ) ;
#4904=EDGE_CURVE ( 'NONE', #13485, #19656, #34263, .T. ) ;
#4905=CARTESIAN_POINT ( 'NONE',  ( -84.94597344681493212, 1.025126265847089657, -80.93171244307201562 ) ) ;
#4908=EDGE_LOOP ( 'NONE', ( #17498, #20340, #44801, #29110, #43346 ) ) ;
#4909=EDGE_CURVE ( 'NONE', #17018, #42553, #6381, .T. ) ;
#4914=VERTEX_POINT ( 'NONE', #7990 ) ;
#4915=CARTESIAN_POINT ( 'NONE',  ( -164.9459734468149463, 2.143131898507880377E-16, 39.06828755692798438 ) ) ;
#4918=CARTESIAN_POINT ( 'NONE',  ( -205.6708471809678827, -1.750000000000009548, -0.2068387089191121020 ) ) ;
#4924=DIRECTION ( 'NONE',  ( 0.000000000000000000, 0.000000000000000000, 1.000000000000000000 ) ) ;
#4925=VECTOR ( 'NONE', #26702, 1000.000000000000000 ) ;
#4929=CARTESIAN_POINT ( 'NONE',  ( 192.2789002873380184, -1.750000000000009548, 39.79316129108089228 ) ) ;
#4933=CARTESIAN_POINT ( 'NONE',  ( -48.44597344681492501, 2.143131898507880377E-16, -160.9317124430720298 ) ) ;
#4934=LINE ( 'NONE', #31908, #11163 ) ;
#4937=ORIENTED_EDGE ( 'NONE', *, *, #13729, .F. ) ;
#4940=LINE ( 'NONE', #47751, #16498 ) ;
#4944=CARTESIAN_POINT ( 'NONE',  ( -8.445973446814976526, 0.000000000000000000, -0.9317124430720524764 ) ) ;
#4945=ORIENTED_EDGE ( 'NONE', *, *, #1846, .T. ) ;
#4946=CARTESIAN_POINT ( 'NONE',  ( 210.0000000000000568, 2.143131898507881856E-16, -80.93171244307202983 ) ) ;
#4948=ORIENTED_EDGE ( 'NONE', *, *, #44613, .F. ) ;
#4949=( NAMED_UNIT ( * ) PLANE_ANGLE_UNIT ( ) SI_UNIT ( $, .RADIAN. ) );
#4951=PLANE ( 'NONE',  #21111 ) ;
#4952=CARTESIAN_POINT ( 'NONE',  ( -46.69597344681494633, 1.750000000000010658, -119.1817124430720440 ) ) ;
#4967=ADVANCED_FACE ( 'NONE', ( #9486 ), #25396, .T. ) ;
#4975=ADVANCED_FACE ( 'NONE', ( #21536 ), #2291, .T. ) ;
#4977=CARTESIAN_POINT ( 'NONE',  ( 33.30402655318503946, -1.750000000000010658, -119.1817124430720440 ) ) ;
#4981=EDGE_CURVE ( 'NONE', #38568, #20319, #25728, .T. ) ;
#4982=ORIENTED_EDGE ( 'NONE', *, *, #1720, .T. ) ;
#4985=FACE_OUTER_BOUND ( 'NONE', #42044, .T. ) ;
#4988=EDGE_LOOP ( 'NONE', ( #48397, #20655, #17417, #2673, #10655 ) ) ;
#4990=CARTESIAN_POINT ( 'NONE',  ( -48.44597344681495343, 0.000000000000000000, -37.43171244307200141 ) ) ;
#4991=DIRECTION ( 'NONE',  ( 0.000000000000000000, 0.000000000000000000, 1.000000000000000000 ) ) ;
#4993=DIRECTION ( 'NONE',  ( -0.000000000000000000, -0.000000000000000000, -1.000000000000000000 ) ) ;
#4995=ORIENTED_EDGE ( 'NONE', *, *, #34184, .F. ) ;
#4999=CARTESIAN_POINT ( 'NONE',  ( 71.55402655318505367, -1.025126265847089657, 42.56828755692799149 ) ) ;
#5001=ORIENTED_EDGE ( 'NONE', *, *, #4502, .T. ) ;
#5009=CYLINDRICAL_SURFACE ( 'NONE', #29890, 1.750000000000015543 ) ;
#5012=DIRECTION ( 'NONE',  ( -0.000000000000000000, -0.000000000000000000, -1.000000000000000000 ) ) ;
#5015=CARTESIAN_POINT ( 'NONE',  ( -206.6959734468149463, 1.750000000000010214, -39.18171244307202983 ) ) ;
#5016=ORIENTED_EDGE ( 'NONE', *, *, #42212, .F. ) ;
#5017=LINE ( 'NONE', #17077, #20143 ) ;
#5020=CARTESIAN_POINT ( 'NONE',  ( 155.0540265531850537, 2.143131898507880377E-16, 165.0000000000000000 ) ) ;
#5023=CARTESIAN_POINT ( 'NONE',  ( -207.7210997126620384, -1.750000000000010214, 119.7931612910808781 ) ) ;
#5030=CARTESIAN_POINT ( 'NONE',  ( -84.94597344681494633, 2.143131898507880377E-16, -120.9317124430720156 ) ) ;
#5033=CARTESIAN_POINT ( 'NONE',  ( -205.6708471809678827, -1.750000000000009548, -78.15658617722490931 ) ) ;
#5034=( BOUNDED_CURVE ( )  B_SPLINE_CURVE ( 3, ( #31983, #43756, #931, #12714 ),
 .UNSPECIFIED., .F., .F. ) 
 B_SPLINE_CURVE_WITH_KNOTS ( ( 4, 4 ),
 ( 3.141592653589793116, 4.712388980384689674 ),
 .UNSPECIFIED. ) 
 CURVE ( )  GEOMETRIC_REPRESENTATION_ITEM ( )  RATIONAL_B_SPLINE_CURVE ( ( 1.000000000000000000, 0.8047378541243649375, 0.8047378541243649375, 1.000000000000000000 ) ) 
 REPRESENTATION_ITEM ( '' )  );
#5040=CARTESIAN_POINT ( 'NONE',  ( -168.4459734468149463, 0.000000000000000000, 122.5682875569279702 ) ) ;
#5041=VERTEX_POINT ( 'NONE', #14340 ) ;
#5043=CARTESIAN_POINT ( 'NONE',  ( 210.0000000000000568, 2.143131898507881116E-16, -40.93171244307203693 ) ) ;
#5047=CARTESIAN_POINT ( 'NONE',  ( 210.0000000000000568, 0.000000000000000000, 160.8182875569279702 ) ) ;
#5063=CARTESIAN_POINT ( 'NONE',  ( 35.05402655318504657, 1.025126265847089879, -77.43171244307200141 ) ) ;
#5067=CARTESIAN_POINT ( 'NONE',  ( -206.6959734468149463, -1.750000000000010658, -119.1817124430720440 ) ) ;
#5076=CARTESIAN_POINT ( 'NONE',  ( 210.0000000000000568, 0.000000000000000000, -37.43171244307202272 ) ) ;
#5079=FACE_OUTER_BOUND ( 'NONE', #46048, .T. ) ;
#5081=CARTESIAN_POINT ( 'NONE',  ( 194.3291528190321742, 1.750000000000009548, -0.2068387089191121020 ) ) ;
#5088=CARTESIAN_POINT ( 'NONE',  ( -44.94597344681493922, 2.143131898507880377E-16, -117.4317124430720156 ) ) ;
#5092=ORIENTED_EDGE ( 'NONE', *, *, #50468, .F. ) ;
#5097=EDGE_CURVE ( 'NONE', #39980, #23318, #32938, .T. ) ;
#5101=FACE_OUTER_BOUND ( 'NONE', #6898, .T. ) ;
#5106=EDGE_CURVE ( 'NONE', #32944, #4897, #39522, .T. ) ;
#5114=VERTEX_POINT ( 'NONE', #24581 ) ;
#5115=CARTESIAN_POINT ( 'NONE',  ( 210.0000000000000568, 0.000000000000000000, 162.5682875569279702 ) ) ;
#5119=ORIENTED_EDGE ( 'NONE', *, *, #5771, .F. ) ;
#5124=ORIENTED_EDGE ( 'NONE', *, *, #1720, .F. ) ;
#5129=CARTESIAN_POINT ( 'NONE',  ( 195.0540265531851105, 2.143131898507880377E-16, 159.0682875569279702 ) ) ;
#5134=CARTESIAN_POINT ( 'NONE',  ( -206.6959734468149463, -1.750000000000009992, -159.1817124430720298 ) ) ;
#5138=EDGE_LOOP ( 'NONE', ( #9903, #6864 ) ) ;
#5139=ORIENTED_EDGE ( 'NONE', *, *, #11088, .T. ) ;
#5143=CARTESIAN_POINT ( 'NONE',  ( -168.4459734468149463, 0.000000000000000000, -80.93171244307201562 ) ) ;
#5146=AXIS2_PLACEMENT_3D ( 'NONE', #33166, #13637, #6696 ) ;
#5147=CARTESIAN_POINT ( 'NONE',  ( -48.44597344681495343, 0.000000000000000000, 42.56828755692798438 ) ) ;
#5157=CYLINDRICAL_SURFACE ( 'NONE', #35274, 1.750000000000001554 ) ;
#5158=EDGE_CURVE ( 'NONE', #30382, #48120, #37725, .T. ) ;
#5160=FACE_OUTER_BOUND ( 'NONE', #46527, .T. ) ;
#5163=DIRECTION ( 'NONE',  ( -1.000000000000000000, -0.000000000000000000, -0.000000000000000000 ) ) ;
#5164=ORIENTED_EDGE ( 'NONE', *, *, #36112, .T. ) ;
#5173=CARTESIAN_POINT ( 'NONE',  ( -128.4459734468149463, 1.025126265847081664, -117.4317124430720440 ) ) ;
#5174=DIRECTION ( 'NONE',  ( -1.000000000000000000, 0.000000000000000000, 0.000000000000000000 ) ) ;
#5176=EDGE_LOOP ( 'NONE', ( #23301, #12458, #37630, #48825, #24406, #11538 ) ) ;
#5177=CARTESIAN_POINT ( 'NONE',  ( 210.0000000000000568, 0.000000000000000000, -39.18171244307202983 ) ) ;
#5178=ADVANCED_FACE ( 'NONE', ( #35652 ), #39232, .T. ) ;
#5180=VERTEX_POINT ( 'NONE', #43307 ) ;
#5187=( BOUNDED_CURVE ( )  B_SPLINE_CURVE ( 3, ( #11474, #3775, #7633, #19424 ),
 .UNSPECIFIED., .F., .F. ) 
 B_SPLINE_CURVE_WITH_KNOTS ( ( 4, 4 ),
 ( 3.141592653589793116, 4.712388980384689674 ),
 .UNSPECIFIED. ) 
 CURVE ( )  GEOMETRIC_REPRESENTATION_ITEM ( )  RATIONAL_B_SPLINE_CURVE ( ( 1.000000000000000000, 0.8047378541243649375, 0.8047378541243649375, 1.000000000000000000 ) ) 
 REPRESENTATION_ITEM ( '' )  );
#5191=CARTESIAN_POINT ( 'NONE',  ( 210.0000000000000568, 0.000000000000000000, 0.8182875569279768335 ) ) ;
#5194=EDGE_CURVE ( 'NONE', #15554, #17436, #25419, .T. ) ;
#5200=CARTESIAN_POINT ( 'NONE',  ( 191.5540265531851105, 0.000000000000000000, 165.0000000000000000 ) ) ;
#5201=ADVANCED_FACE ( 'NONE', ( #20464 ), #986, .T. ) ;
#5205=( BOUNDED_CURVE ( )  B_SPLINE_CURVE ( 3, ( #30857, #12342, #24168, #7756 ),
 .UNSPECIFIED., .F., .T. ) 
 B_SPLINE_CURVE_WITH_KNOTS ( ( 4, 4 ),
 ( 0.000000000000000000, 1.570796326794896558 ),
 .UNSPECIFIED. ) 
 CURVE ( )  GEOMETRIC_REPRESENTATION_ITEM ( )  RATIONAL_B_SPLINE_CURVE ( ( 1.000000000000000000, 0.8047378541243649375, 0.8047378541243649375, 1.000000000000000000 ) ) 
 REPRESENTATION_ITEM ( '' )  );
#5207=ORIENTED_EDGE ( 'NONE', *, *, #46093, .T. ) ;
#5209=CARTESIAN_POINT ( 'NONE',  ( -8.445973446814976526, 0.000000000000000000, 165.0000000000000000 ) ) ;
#5223=ORIENTED_EDGE ( 'NONE', *, *, #18836, .F. ) ;
#5224=EDGE_CURVE ( 'NONE', #43947, #44210, #1157, .T. ) ;
#5226=ORIENTED_EDGE ( 'NONE', *, *, #41644, .T. ) ;
#5230=ORIENTED_EDGE ( 'NONE', *, *, #2406, .T. ) ;
#5231=ORIENTED_EDGE ( 'NONE', *, *, #20245, .F. ) ;
#5238=ORIENTED_EDGE ( 'NONE', *, *, #40359, .F. ) ;
#5243=EDGE_LOOP ( 'NONE', ( #4659, #1921, #31577, #49527, #10802, #20257 ) ) ;
#5244=ORIENTED_EDGE ( 'NONE', *, *, #13930, .T. ) ;
#5247=CARTESIAN_POINT ( 'NONE',  ( 191.5540265531851105, 0.000000000000000000, -77.43171244307204404 ) ) ;
#5253=EDGE_CURVE ( 'NONE', #9269, #16197, #41143, .T. ) ;
#5264=EDGE_CURVE ( 'NONE', #39465, #8778, #21489, .T. ) ;
#5266=CARTESIAN_POINT ( 'NONE',  ( -127.7210997126620242, 1.749999999999996669, 81.84341382277506227 ) ) ;
#5267=EDGE_LOOP ( 'NONE', ( #16213, #13340, #29410, #39219, #28843, #6897 ) ) ;
#5271=CARTESIAN_POINT ( 'NONE',  ( 210.0000000000000568, 2.143131898507881116E-16, 39.06828755692797728 ) ) ;
#5273=CARTESIAN_POINT ( 'NONE',  ( 210.0000000000000568, 0.000000000000000000, -159.1817124430720298 ) ) ;
#5274=ORIENTED_EDGE ( 'NONE', *, *, #32620, .F. ) ;
#5279=CARTESIAN_POINT ( 'NONE',  ( 153.3040265531850537, 1.750000000000010658, 120.8182875569279702 ) ) ;
#5283=DIRECTION ( 'NONE',  ( 1.000000000000000000, 0.000000000000000000, 0.000000000000000000 ) ) ;
#5284=CARTESIAN_POINT ( 'NONE',  ( -8.445973446814976526, 0.000000000000000000, -117.4317124430720156 ) ) ;
#5285=CARTESIAN_POINT ( 'NONE',  ( -46.69597344681494633, -1.750000000000010658, 80.81828755692798438 ) ) ;
#5296=EDGE_LOOP ( 'NONE', ( #35875, #32658, #39711, #202, #25420, #36700 ) ) ;
#5298=EDGE_CURVE ( 'NONE', #32944, #4845, #46364, .T. ) ;
#5299=CARTESIAN_POINT ( 'NONE',  ( 32.27890028733795447, -1.750000000000010214, -120.2068387089191219 ) ) ;
#5306=CARTESIAN_POINT ( 'NONE',  ( 74.32915281903215998, 1.750000000000010214, 81.84341382277507648 ) ) ;
#5312=EDGE_LOOP ( 'NONE', ( #20604, #5207, #2100, #13380, #30065, #50084 ) ) ;
#5313=CARTESIAN_POINT ( 'NONE',  ( -124.9459734468149463, 2.143131898507847836E-16, -157.4317124430720582 ) ) ;
#5314=EDGE_CURVE ( 'NONE', #17018, #6332, #1739, .T. ) ;
#5318=ORIENTED_EDGE ( 'NONE', *, *, #14260, .T. ) ;
#5322=EDGE_CURVE ( 'NONE', #22009, #36281, #11331, .T. ) ;
#5323=DIRECTION ( 'NONE',  ( 0.000000000000000000, 0.000000000000000000, 1.000000000000000000 ) ) ;
#5328=CARTESIAN_POINT ( 'NONE',  ( -124.9459734468149321, 1.025126265847082108, 82.56828755692798438 ) ) ;
#5335=FACE_OUTER_BOUND ( 'NONE', #9411, .T. ) ;
#5341=LINE ( 'NONE', #5076, #50699 ) ;
#5342=( BOUNDED_CURVE ( )  B_SPLINE_CURVE ( 3, ( #2921, #30140, #45503, #34505 ),
 .UNSPECIFIED., .F., .F. ) 
 B_SPLINE_CURVE_WITH_KNOTS ( ( 4, 4 ),
 ( 4.712388980384689674, 6.283185307179586232 ),
 .UNSPECIFIED. ) 
 CURVE ( )  GEOMETRIC_REPRESENTATION_ITEM ( )  RATIONAL_B_SPLINE_CURVE ( ( 1.000000000000000000, 0.8047378541243649375, 0.8047378541243649375, 1.000000000000000000 ) ) 
 REPRESENTATION_ITEM ( '' )  );
#5344=CARTESIAN_POINT ( 'NONE',  ( -128.4459734468149179, 0.000000000000000000, 165.0000000000000000 ) ) ;
#5355=ORIENTED_EDGE ( 'NONE', *, *, #10249, .T. ) ;
#5356=ORIENTED_EDGE ( 'NONE', *, *, #1852, .T. ) ;
#5358=AXIS2_PLACEMENT_3D ( 'NONE', #34993, #19305, #23154 ) ;
#5360=CARTESIAN_POINT ( 'NONE',  ( -167.7210997126620384, -1.750000000000009548, 39.79316129108089228 ) ) ;
#5362=ORIENTED_EDGE ( 'NONE', *, *, #34367, .F. ) ;
#5365=CARTESIAN_POINT ( 'NONE',  ( -48.44597344681495343, 0.000000000000000000, 165.0000000000000000 ) ) ;
#5369=CARTESIAN_POINT ( 'NONE',  ( -206.6959734468149463, 0.000000000000000000, 165.0000000000000000 ) ) ;
#5371=ORIENTED_EDGE ( 'NONE', *, *, #16278, .F. ) ;
#5380=EDGE_LOOP ( 'NONE', ( #10022, #34348, #22990, #49445, #2829 ) ) ;
#5383=CARTESIAN_POINT ( 'NONE',  ( -164.9459734468149463, 2.143131898507880377E-16, 165.0000000000000000 ) ) ;
#5384=CARTESIAN_POINT ( 'NONE',  ( -208.4459734468148611, -1.025126265847089435, -157.4317124430720582 ) ) ;
#5386=CYLINDRICAL_SURFACE ( 'NONE', #16329, 1.750000000000008438 ) ;
#5387=CARTESIAN_POINT ( 'NONE',  ( 210.0000000000000568, 2.143131898507881856E-16, -120.9317124430720582 ) ) ;
#5388=EDGE_CURVE ( 'NONE', #4058, #47505, #16583, .T. ) ;
#5393=CARTESIAN_POINT ( 'NONE',  ( -6.695973446814940111, 1.750000000000023759, -39.18171244307202983 ) ) ;
#5397=AXIS2_PLACEMENT_3D ( 'NONE', #34541, #50123, #30691 ) ;
#5399=VERTEX_POINT ( 'NONE', #42482 ) ;
#5402=CARTESIAN_POINT ( 'NONE',  ( 210.0000000000000568, 0.000000000000000000, 120.8182875569279702 ) ) ;
#5404=AXIS2_PLACEMENT_3D ( 'NONE', #17365, #48617, #32777 ) ;
#5411=DIRECTION ( 'NONE',  ( -1.000000000000000000, -0.000000000000000000, -0.000000000000000000 ) ) ;
#5412=FACE_OUTER_BOUND ( 'NONE', #25586, .T. ) ;
#5415=ORIENTED_EDGE ( 'NONE', *, *, #10741, .T. ) ;
#5420=LINE ( 'NONE', #9770, #30303 ) ;
#5422=( BOUNDED_CURVE ( )  B_SPLINE_CURVE ( 3, ( #30650, #49079, #41429, #45742 ),
 .UNSPECIFIED., .F., .F. ) 
 B_SPLINE_CURVE_WITH_KNOTS ( ( 4, 4 ),
 ( 4.712388980384689674, 6.283185307179586232 ),
 .UNSPECIFIED. ) 
 CURVE ( )  GEOMETRIC_REPRESENTATION_ITEM ( )  RATIONAL_B_SPLINE_CURVE ( ( 1.000000000000000000, 0.8047378541243649375, 0.8047378541243649375, 1.000000000000000000 ) ) 
 REPRESENTATION_ITEM ( '' )  );
#5423=DIRECTION ( 'NONE',  ( -0.000000000000000000, -0.000000000000000000, -1.000000000000000000 ) ) ;
#5427=ORIENTED_EDGE ( 'NONE', *, *, #7999, .F. ) ;
#5437=VERTEX_POINT ( 'NONE', #21985 ) ;
#5439=DIRECTION ( 'NONE',  ( -0.000000000000000000, -0.000000000000000000, -1.000000000000000000 ) ) ;
#5440=CIRCLE ( 'NONE', #12012, 1.750000000000001554 ) ;
#5446=ORIENTED_EDGE ( 'NONE', *, *, #18323, .T. ) ;
#5447=CARTESIAN_POINT ( 'NONE',  ( -167.7210997126620384, -1.750000000000010214, -118.1565861772249519 ) ) ;
#5458=( NAMED_UNIT ( * ) SI_UNIT ( $, .STERADIAN. ) SOLID_ANGLE_UNIT ( ) );
#5462=FACE_OUTER_BOUND ( 'NONE', #38966, .T. ) ;
#5463=CARTESIAN_POINT ( 'NONE',  ( -46.69597344681494633, -1.750000000000010658, 120.8182875569279702 ) ) ;
#5472=ORIENTED_EDGE ( 'NONE', *, *, #46969, .F. ) ;
#5473=CARTESIAN_POINT ( 'NONE',  ( 193.3040265531851105, 1.750000000000009992, 0.8182875569279768335 ) ) ;
#5475=ADVANCED_FACE ( 'NONE', ( #3226 ), #34556, .T. ) ;
#5478=ORIENTED_EDGE ( 'NONE', *, *, #458, .F. ) ;
#5479=( BOUNDED_CURVE ( )  B_SPLINE_CURVE ( 3, ( #21753, #10208, #25860, #14550 ),
 .UNSPECIFIED., .F., .F. ) 
 B_SPLINE_CURVE_WITH_KNOTS ( ( 4, 4 ),
 ( 0.000000000000000000, 1.570796326794896558 ),
 .UNSPECIFIED. ) 
 CURVE ( )  GEOMETRIC_REPRESENTATION_ITEM ( )  RATIONAL_B_SPLINE_CURVE ( ( 1.000000000000000000, 0.8047378541243649375, 0.8047378541243649375, 1.000000000000000000 ) ) 
 REPRESENTATION_ITEM ( '' )  );
#5484=FACE_OUTER_BOUND ( 'NONE', #40392, .T. ) ;
#5487=( BOUNDED_CURVE ( )  B_SPLINE_CURVE ( 3, ( #19024, #26989, #15198, #46450 ),
 .UNSPECIFIED., .F., .F. ) 
 B_SPLINE_CURVE_WITH_KNOTS ( ( 4, 4 ),
 ( 3.141592653589793116, 4.712388980384689674 ),
 .UNSPECIFIED. ) 
 CURVE ( )  GEOMETRIC_REPRESENTATION_ITEM ( )  RATIONAL_B_SPLINE_CURVE ( ( 1.000000000000000000, 0.8047378541243649375, 0.8047378541243649375, 1.000000000000000000 ) ) 
 REPRESENTATION_ITEM ( '' )  );
#5488=EDGE_CURVE ( 'NONE', #12229, #25250, #9088, .T. ) ;
#5497=FACE_OUTER_BOUND ( 'NONE', #47328, .T. ) ;
#5498=CARTESIAN_POINT ( 'NONE',  ( -168.4459734468149747, 1.025126265847089213, 159.0682875569279418 ) ) ;
#5499=CARTESIAN_POINT ( 'NONE',  ( 33.30402655318503946, 1.750000000000009992, 160.8182875569279702 ) ) ;
#5500=ORIENTED_EDGE ( 'NONE', *, *, #25818, .F. ) ;
#5503=( BOUNDED_CURVE ( )  B_SPLINE_CURVE ( 3, ( #29115, #37087, #41154, #14199 ),
 .UNSPECIFIED., .F., .F. ) 
 B_SPLINE_CURVE_WITH_KNOTS ( ( 4, 4 ),
 ( 0.000000000000000000, 1.570796326794896558 ),
 .UNSPECIFIED. ) 
 CURVE ( )  GEOMETRIC_REPRESENTATION_ITEM ( )  RATIONAL_B_SPLINE_CURVE ( ( 1.000000000000000000, 0.8047378541243649375, 0.8047378541243649375, 1.000000000000000000 ) ) 
 REPRESENTATION_ITEM ( '' )  );
#5504=EDGE_CURVE ( 'NONE', #960, #14675, #33665, .T. ) ;
#5510=ORIENTED_EDGE ( 'NONE', *, *, #12538, .T. ) ;
#5511=VERTEX_POINT ( 'NONE', #19901 ) ;
#5513=CYLINDRICAL_SURFACE ( 'NONE', #28990, 1.750000000000015543 ) ;
#5514=ORIENTED_EDGE ( 'NONE', *, *, #10198, .F. ) ;
#5517=CARTESIAN_POINT ( 'NONE',  ( 210.0000000000000568, 0.000000000000000000, -37.43171244307202272 ) ) ;
#5518=ORIENTED_EDGE ( 'NONE', *, *, #49972, .T. ) ;
#5519=CARTESIAN_POINT ( 'NONE',  ( 152.2789002873379900, -1.750000000000010214, 121.8434138227750623 ) ) ;
#5521=CARTESIAN_POINT ( 'NONE',  ( -86.69597344681494633, -1.750000000000009992, -159.1817124430720298 ) ) ;
#5523=CARTESIAN_POINT ( 'NONE',  ( -206.6959734468149463, 0.000000000000000000, 165.0000000000000000 ) ) ;
#5525=EDGE_CURVE ( 'NONE', #33474, #21965, #27625, .T. ) ;
#5535=CYLINDRICAL_SURFACE ( 'NONE', #1595, 1.750000000000015543 ) ;
#5536=ORIENTED_EDGE ( 'NONE', *, *, #35030, .T. ) ;
#5538=EDGE_CURVE ( 'NONE', #16170, #28550, #19862, .T. ) ;
#5542=FACE_OUTER_BOUND ( 'NONE', #18492, .T. ) ;
#5544=CARTESIAN_POINT ( 'NONE',  ( -44.94597344681493922, 2.143131898507880377E-16, -37.43171244307200141 ) ) ;
#5548=EDGE_LOOP ( 'NONE', ( #25671, #32865, #14516, #34864, #2466 ) ) ;
#5551=CARTESIAN_POINT ( 'NONE',  ( -168.4459734468149747, -1.025126265847089657, -80.93171244307201562 ) ) ;
#5552=EDGE_CURVE ( 'NONE', #40604, #15344, #41165, .T. ) ;
#5554=CARTESIAN_POINT ( 'NONE',  ( -164.9459734468149463, 2.143131898507880377E-16, -160.9317124430720014 ) ) ;
#5560=CYLINDRICAL_SURFACE ( 'NONE', #36501, 1.750000000000010214 ) ;
#5563=ORIENTED_EDGE ( 'NONE', *, *, #43099, .T. ) ;
#5565=DIRECTION ( 'NONE',  ( -0.000000000000000000, -0.000000000000000000, -1.000000000000000000 ) ) ;
#5566=ORIENTED_EDGE ( 'NONE', *, *, #5552, .F. ) ;
#5570=CARTESIAN_POINT ( 'NONE',  ( 192.2789002873380184, 1.750000000000010436, -80.20683870891910772 ) ) ;
#5572=CARTESIAN_POINT ( 'NONE',  ( 34.32915281903212446, 1.750000000000010214, -78.15658617722490931 ) ) ;
#5577=CARTESIAN_POINT ( 'NONE',  ( -205.6708471809678827, 1.750000000000009548, 41.84341382277508359 ) ) ;
#5578=CARTESIAN_POINT ( 'NONE',  ( -47.72109971266203132, -1.750000000000009548, 161.8434138227750907 ) ) ;
#5579=CARTESIAN_POINT ( 'NONE',  ( -88.44597344681497475, 0.000000000000000000, -117.4317124430720156 ) ) ;
#5582=EDGE_CURVE ( 'NONE', #20412, #14675, #30074, .T. ) ;
#5587=DIRECTION ( 'NONE',  ( 1.000000000000000000, 0.000000000000000000, 0.000000000000000000 ) ) ;
#5589=CARTESIAN_POINT ( 'NONE',  ( 155.0540265531850537, 2.143131898507880377E-16, -80.93171244307201562 ) ) ;
#5591=CARTESIAN_POINT ( 'NONE',  ( 33.30402655318503946, 1.750000000000010658, -79.18171244307201562 ) ) ;
#5592=ADVANCED_FACE ( 'NONE', ( #13466 ), #37099, .T. ) ;
#5593=ADVANCED_FACE ( 'NONE', ( #36603 ), #9623, .T. ) ;
#5597=CYLINDRICAL_SURFACE ( 'NONE', #11020, 1.749999999999973799 ) ;
#5598=DIRECTION ( 'NONE',  ( 0.000000000000000000, 0.000000000000000000, 1.000000000000000000 ) ) ;
#5607=AXIS2_PLACEMENT_3D ( 'NONE', #5782, #45751, #6539 ) ;
#5608=ORIENTED_EDGE ( 'NONE', *, *, #18881, .F. ) ;
#5615=DIRECTION ( 'NONE',  ( -1.000000000000000000, 0.000000000000000000, 0.000000000000000000 ) ) ;
#5620=ORIENTED_EDGE ( 'NONE', *, *, #45836, .F. ) ;
#5625=ORIENTED_EDGE ( 'NONE', *, *, #24370, .T. ) ;
#5626=LINE ( 'NONE', #4864, #13876 ) ;
#5627=CARTESIAN_POINT ( 'NONE',  ( -48.44597344681495343, 0.000000000000000000, 39.06828755692798438 ) ) ;
#5630=DIRECTION ( 'NONE',  ( -0.000000000000000000, -0.000000000000000000, -1.000000000000000000 ) ) ;
#5631=CARTESIAN_POINT ( 'NONE',  ( -84.94597344681493212, -1.025126265847089657, 79.06828755692797017 ) ) ;
#5632=CARTESIAN_POINT ( 'NONE',  ( -207.7210997126620384, -1.750000000000009548, -158.1565861772249377 ) ) ;
#5633=ORIENTED_EDGE ( 'NONE', *, *, #24333, .T. ) ;
#5637=( BOUNDED_CURVE ( )  B_SPLINE_CURVE ( 3, ( #10303, #29296, #16991, #48986 ),
 .UNSPECIFIED., .F., .F. ) 
 B_SPLINE_CURVE_WITH_KNOTS ( ( 4, 4 ),
 ( 3.141592653589793116, 4.712388980384689674 ),
 .UNSPECIFIED. ) 
 CURVE ( )  GEOMETRIC_REPRESENTATION_ITEM ( )  RATIONAL_B_SPLINE_CURVE ( ( 1.000000000000000000, 0.8047378541243649375, 0.8047378541243649375, 1.000000000000000000 ) ) 
 REPRESENTATION_ITEM ( '' )  );
#5639=VERTEX_POINT ( 'NONE', #33743 ) ;
#5644=DIRECTION ( 'NONE',  ( 0.000000000000000000, 0.000000000000000000, -1.000000000000000000 ) ) ;
#5646=VECTOR ( 'NONE', #746, 1000.000000000000000 ) ;
#5649=ORIENTED_EDGE ( 'NONE', *, *, #41016, .T. ) ;
#5652=FACE_OUTER_BOUND ( 'NONE', #23410, .T. ) ;
#5656=VECTOR ( 'NONE', #47947, 1000.000000000000000 ) ;
#5657=CARTESIAN_POINT ( 'NONE',  ( 210.0000000000000568, 0.000000000000000000, -119.1817124430720440 ) ) ;
#5661=ORIENTED_EDGE ( 'NONE', *, *, #2704, .T. ) ;
#5664=EDGE_LOOP ( 'NONE', ( #283, #37998, #29739, #28090, #37122, #49497 ) ) ;
#5665=LINE ( 'NONE', #36752, #3293 ) ;
#5666=CARTESIAN_POINT ( 'NONE',  ( -207.7210997126620384, -1.750000000000009548, -160.2068387089191219 ) ) ;
#5668=ORIENTED_EDGE ( 'NONE', *, *, #31852, .F. ) ;
#5675=EDGE_CURVE ( 'NONE', #37518, #33796, #18310, .T. ) ;
#5683=CARTESIAN_POINT ( 'NONE',  ( -126.6959734468149321, -1.749999999999997335, -79.18171244307201562 ) ) ;
#5684=CARTESIAN_POINT ( 'NONE',  ( 32.27890028733795447, 1.750000000000009326, -158.1565861772249377 ) ) ;
#5685=EDGE_LOOP ( 'NONE', ( #1427, #28695, #32580, #5124, #31405, #18798 ) ) ;
#5686=DIRECTION ( 'NONE',  ( -1.000000000000000000, -0.000000000000000000, -0.000000000000000000 ) ) ;
#5689=DIRECTION ( 'NONE',  ( 0.000000000000000000, 0.000000000000000000, 1.000000000000000000 ) ) ;
#5694=AXIS2_PLACEMENT_3D ( 'NONE', #42204, #6045, #30413 ) ;
#5696=ORIENTED_EDGE ( 'NONE', *, *, #25363, .F. ) ;
#5699=CARTESIAN_POINT ( 'NONE',  ( -85.67084718096784002, 1.750000000000010214, 81.84341382277507648 ) ) ;
#5706=VERTEX_POINT ( 'NONE', #14212 ) ;
#5711=CARTESIAN_POINT ( 'NONE',  ( 210.0000000000000568, 0.000000000000000000, 120.8182875569279702 ) ) ;
#5712=DIRECTION ( 'NONE',  ( -1.000000000000000000, -0.000000000000000000, -0.000000000000000000 ) ) ;
#5722=( BOUNDED_CURVE ( )  B_SPLINE_CURVE ( 3, ( #27703, #46902, #7704, #19746 ),
 .UNSPECIFIED., .F., .F. ) 
 B_SPLINE_CURVE_WITH_KNOTS ( ( 4, 4 ),
 ( 1.570796326794896558, 3.141592653589793116 ),
 .UNSPECIFIED. ) 
 CURVE ( )  GEOMETRIC_REPRESENTATION_ITEM ( )  RATIONAL_B_SPLINE_CURVE ( ( 1.000000000000000000, 0.8047378541243649375, 0.8047378541243649375, 1.000000000000000000 ) ) 
 REPRESENTATION_ITEM ( '' )  );
#5724=ORIENTED_EDGE ( 'NONE', *, *, #28511, .T. ) ;
#5726=LINE ( 'NONE', #44455, #7380 ) ;
#5727=CARTESIAN_POINT ( 'NONE',  ( 115.0540265531850395, 2.143131898507847836E-16, 122.5682875569279560 ) ) ;
#5730=AXIS2_PLACEMENT_3D ( 'NONE', #36247, #24940, #9282 ) ;
#5733=DIRECTION ( 'NONE',  ( -1.000000000000000000, -0.000000000000000000, -0.000000000000000000 ) ) ;
#5735=ADVANCED_FACE ( 'NONE', ( #45497 ), #10385, .T. ) ;
#5736=EDGE_LOOP ( 'NONE', ( #48782, #6809, #5608, #21655, #28005, #8658 ) ) ;
#5739=ADVANCED_FACE ( 'NONE', ( #43387 ), #320, .T. ) ;
#5742=ORIENTED_EDGE ( 'NONE', *, *, #2036, .T. ) ;
#5743=VERTEX_POINT ( 'NONE', #8774 ) ;
#5745=DIRECTION ( 'NONE',  ( -0.000000000000000000, -0.000000000000000000, -1.000000000000000000 ) ) ;
#5748=ORIENTED_EDGE ( 'NONE', *, *, #35417, .F. ) ;
#5749=ORIENTED_EDGE ( 'NONE', *, *, #16083, .F. ) ;
#5756=AXIS2_PLACEMENT_3D ( 'NONE', #23139, #20060, #27260 ) ;
#5758=ORIENTED_EDGE ( 'NONE', *, *, #26959, .T. ) ;
#5761=AXIS2_PLACEMENT_3D ( 'NONE', #39042, #4134, #8494 ) ;
#5763=VERTEX_POINT ( 'NONE', #43638 ) ;
#5764=ADVANCED_FACE ( 'NONE', ( #31873 ), #20303, .T. ) ;
#5768=DIRECTION ( 'NONE',  ( -1.000000000000000000, 0.000000000000000000, 0.000000000000000000 ) ) ;
#5769=VERTEX_POINT ( 'NONE', #31100 ) ;
#5770=CARTESIAN_POINT ( 'NONE',  ( 153.3040265531850537, 1.750000000000009992, 160.8182875569279702 ) ) ;
#5771=EDGE_CURVE ( 'NONE', #16293, #6202, #9386, .T. ) ;
#5777=VERTEX_POINT ( 'NONE', #28264 ) ;
#5779=CYLINDRICAL_SURFACE ( 'NONE', #43067, 1.750000000000001554 ) ;
#5780=ADVANCED_FACE ( 'NONE', ( #20052 ), #19794, .T. ) ;
#5782=CARTESIAN_POINT ( 'NONE',  ( 210.0000000000000568, 0.000000000000000000, 40.81828755692798438 ) ) ;
#5783=CARTESIAN_POINT ( 'NONE',  ( -6.695973446814940111, -1.750000000000023315, 0.8182875569279768335 ) ) ;
#5784=( BOUNDED_CURVE ( )  B_SPLINE_CURVE ( 3, ( #35862, #16337, #32005, #47598 ),
 .UNSPECIFIED., .F., .F. ) 
 B_SPLINE_CURVE_WITH_KNOTS ( ( 4, 4 ),
 ( 0.000000000000000000, 1.570796326794896558 ),
 .UNSPECIFIED. ) 
 CURVE ( )  GEOMETRIC_REPRESENTATION_ITEM ( )  RATIONAL_B_SPLINE_CURVE ( ( 1.000000000000000000, 0.8047378541243649375, 0.8047378541243649375, 1.000000000000000000 ) ) 
 REPRESENTATION_ITEM ( '' )  );
#5786=CARTESIAN_POINT ( 'NONE',  ( 193.3040265531851105, -1.750000000000010658, -119.1817124430720440 ) ) ;
#5787=MANIFOLD_SOLID_BREP ( 'Boss-Extrude2', #44141 ) ;
#5789=DIRECTION ( 'NONE',  ( 0.000000000000000000, 0.000000000000000000, 1.000000000000000000 ) ) ;
#5790=( BOUNDED_CURVE ( )  B_SPLINE_CURVE ( 3, ( #31643, #836, #31383, #587 ),
 .UNSPECIFIED., .F., .F. ) 
 B_SPLINE_CURVE_WITH_KNOTS ( ( 4, 4 ),
 ( 3.141592653589793116, 4.712388980384689674 ),
 .UNSPECIFIED. ) 
 CURVE ( )  GEOMETRIC_REPRESENTATION_ITEM ( )  RATIONAL_B_SPLINE_CURVE ( ( 1.000000000000000000, 0.8047378541243649375, 0.8047378541243649375, 1.000000000000000000 ) ) 
 REPRESENTATION_ITEM ( '' )  );
#5800=CARTESIAN_POINT ( 'NONE',  ( 75.05402655318509630, 2.143131898507880377E-16, -80.93171244307204404 ) ) ;
#5804=CARTESIAN_POINT ( 'NONE',  ( -207.7210997126620384, -1.750000000000009548, 1.843413822775065825 ) ) ;
#5810=DIRECTION ( 'NONE',  ( -1.000000000000000000, -0.000000000000000000, -0.000000000000000000 ) ) ;
#5818=ORIENTED_EDGE ( 'NONE', *, *, #7121, .F. ) ;
#5819=CARTESIAN_POINT ( 'NONE',  ( -86.69597344681496054, 0.000000000000000000, 165.0000000000000000 ) ) ;
#5821=CARTESIAN_POINT ( 'NONE',  ( -86.69597344681494633, -1.750000000000010658, -79.18171244307201562 ) ) ;
#5823=EDGE_CURVE ( 'NONE', #47489, #24452, #41065, .T. ) ;
#5825=ORIENTED_EDGE ( 'NONE', *, *, #25519, .T. ) ;
#5826=FACE_OUTER_BOUND ( 'NONE', #30998, .T. ) ;
#5827=CARTESIAN_POINT ( 'NONE',  ( 191.5540265531851105, 0.000000000000000000, -80.93171244307201562 ) ) ;
#5828=ORIENTED_EDGE ( 'NONE', *, *, #45645, .T. ) ;
#5831=CARTESIAN_POINT ( 'NONE',  ( -6.695973446814940111, 1.750000000000024203, -119.1817124430720440 ) ) ;
#5833=CARTESIAN_POINT ( 'NONE',  ( 210.0000000000000568, 0.000000000000000000, 0.8182875569279768335 ) ) ;
#5834=CARTESIAN_POINT ( 'NONE',  ( 73.30402655318508209, 1.750000000000010214, 40.81828755692798438 ) ) ;
#5835=EDGE_CURVE ( 'NONE', #48110, #16730, #32858, .T. ) ;
#5838=EDGE_CURVE ( 'NONE', #19943, #41219, #1570, .T. ) ;
#5846=CARTESIAN_POINT ( 'NONE',  ( -208.4459734468149463, 0.000000000000000000, 122.5682875569279702 ) ) ;
#5849=CARTESIAN_POINT ( 'NONE',  ( -128.4459734468149179, 0.000000000000000000, -37.43171244307205825 ) ) ;
#5851=CARTESIAN_POINT ( 'NONE',  ( 210.0000000000000568, 0.000000000000000000, -159.1817124430720298 ) ) ;
#5853=FACE_OUTER_BOUND ( 'NONE', #32483, .T. ) ;
#5858=CARTESIAN_POINT ( 'NONE',  ( -48.44597344681495343, 0.000000000000000000, 119.0682875569279702 ) ) ;
#5859=CARTESIAN_POINT ( 'NONE',  ( 192.2789002873380184, 1.750000000000009548, 121.8434138227750623 ) ) ;
#5863=ORIENTED_EDGE ( 'NONE', *, *, #16654, .T. ) ;
#5864=ORIENTED_EDGE ( 'NONE', *, *, #24684, .T. ) ;
#5866=ORIENTED_EDGE ( 'NONE', *, *, #26236, .T. ) ;
#5867=DIRECTION ( 'NONE',  ( -1.000000000000000000, -0.000000000000000000, -0.000000000000000000 ) ) ;
#5869=VERTEX_POINT ( 'NONE', #33384 ) ;
#5872=FACE_OUTER_BOUND ( 'NONE', #3456, .T. ) ;
#5873=AXIS2_PLACEMENT_3D ( 'NONE', #44458, #28577, #9338 ) ;
#5875=ORIENTED_EDGE ( 'NONE', *, *, #33151, .F. ) ;
#5877=ORIENTED_EDGE ( 'NONE', *, *, #39352, .F. ) ;
#5878=CARTESIAN_POINT ( 'NONE',  ( -8.445973446814962315, -1.025126265847097207, 2.568287556927999926 ) ) ;
#5880=ORIENTED_EDGE ( 'NONE', *, *, #18054, .T. ) ;
#5881=ORIENTED_EDGE ( 'NONE', *, *, #29143, .F. ) ;
#5882=ORIENTED_EDGE ( 'NONE', *, *, #30777, .T. ) ;
#5884=CARTESIAN_POINT ( 'NONE',  ( -47.72109971266203132, 1.750000000000009548, 39.79316129108089228 ) ) ;
#5890=CARTESIAN_POINT ( 'NONE',  ( -4.945973446814916130, 1.025126265847097651, 82.56828755692798438 ) ) ;
#5891=EDGE_CURVE ( 'NONE', #4629, #3971, #17901, .T. ) ;
#5895=EDGE_CURVE ( 'NONE', #21583, #13512, #28423, .T. ) ;
#5906=EDGE_CURVE ( 'NONE', #4790, #28808, #40554, .T. ) ;
#5909=CARTESIAN_POINT ( 'NONE',  ( 191.5540265531851105, 0.000000000000000000, -40.93171244307202983 ) ) ;
#5910=VERTEX_POINT ( 'NONE', #33884 ) ;
#5911=CARTESIAN_POINT ( 'NONE',  ( -166.6959734468149463, 1.750000000000009992, 0.8182875569279768335 ) ) ;
#5919=( BOUNDED_CURVE ( )  B_SPLINE_CURVE ( 3, ( #12475, #19926, #4537, #16088 ),
 .UNSPECIFIED., .F., .F. ) 
 B_SPLINE_CURVE_WITH_KNOTS ( ( 4, 4 ),
 ( 1.570796326794896558, 3.141592653589793116 ),
 .UNSPECIFIED. ) 
 CURVE ( )  GEOMETRIC_REPRESENTATION_ITEM ( )  RATIONAL_B_SPLINE_CURVE ( ( 1.000000000000000000, 0.8047378541243649375, 0.8047378541243649375, 1.000000000000000000 ) ) 
 REPRESENTATION_ITEM ( '' )  );
#5920=CARTESIAN_POINT ( 'NONE',  ( 35.05402655318504657, 2.143131898507880377E-16, 39.06828755692798438 ) ) ;
#5923=CYLINDRICAL_SURFACE ( 'NONE', #18290, 1.750000000000008438 ) ;
#5925=CARTESIAN_POINT ( 'NONE',  ( 115.0540265531850395, 2.143131898507847836E-16, 42.56828755692795596 ) ) ;
#5928=CARTESIAN_POINT ( 'NONE',  ( 113.3040265531850537, 0.000000000000000000, 165.0000000000000000 ) ) ;
#5929=ORIENTED_EDGE ( 'NONE', *, *, #40910, .F. ) ;
#5930=ORIENTED_EDGE ( 'NONE', *, *, #28345, .T. ) ;
#5932=VECTOR ( 'NONE', #41070, 1000.000000000000000 ) ;
#5933=EDGE_CURVE ( 'NONE', #11195, #4845, #41817, .T. ) ;
#5934=ORIENTED_EDGE ( 'NONE', *, *, #8795, .T. ) ;
#5941=( BOUNDED_CURVE ( )  B_SPLINE_CURVE ( 3, ( #663, #32719, #44743, #36845 ),
 .UNSPECIFIED., .F., .F. ) 
 B_SPLINE_CURVE_WITH_KNOTS ( ( 4, 4 ),
 ( 3.141592653589793116, 4.712388980384689674 ),
 .UNSPECIFIED. ) 
 CURVE ( )  GEOMETRIC_REPRESENTATION_ITEM ( )  RATIONAL_B_SPLINE_CURVE ( ( 1.000000000000000000, 0.8047378541243649375, 0.8047378541243649375, 1.000000000000000000 ) ) 
 REPRESENTATION_ITEM ( '' )  );
#5944=CARTESIAN_POINT ( 'NONE',  ( 194.3291528190321742, 1.750000000000010214, -78.15658617722490931 ) ) ;
#5945=CARTESIAN_POINT ( 'NONE',  ( -126.6959734468149321, 1.749999999999997113, -39.18171244307202983 ) ) ;
#5947=CARTESIAN_POINT ( 'NONE',  ( 115.0540265531850395, 2.143131898507847836E-16, 39.06828755692798438 ) ) ;
#5955=AXIS2_PLACEMENT_3D ( 'NONE', #12138, #21083, #14132 ) ;
#5956=DIRECTION ( 'NONE',  ( -1.000000000000000000, -0.000000000000000000, -0.000000000000000000 ) ) ;
#5957=ORIENTED_EDGE ( 'NONE', *, *, #37256, .T. ) ;
#5961=EDGE_CURVE ( 'NONE', #18600, #42641, #7446, .T. ) ;
#5962=DIRECTION ( 'NONE',  ( 0.000000000000000000, 0.000000000000000000, 1.000000000000000000 ) ) ;
#5964=CYLINDRICAL_SURFACE ( 'NONE', #46278, 1.750000000000008438 ) ;
#5970=CARTESIAN_POINT ( 'NONE',  ( 193.3040265531851105, -1.750000000000010214, -39.18171244307202983 ) ) ;
#5971=AXIS2_PLACEMENT_3D ( 'NONE', #41236, #13024, #20732 ) ;
#5983=CARTESIAN_POINT ( 'NONE',  ( 111.5540265531850679, 0.000000000000000000, 165.0000000000000000 ) ) ;
#5987=CARTESIAN_POINT ( 'NONE',  ( 75.05402655318509630, 2.143131898507880377E-16, -77.43171244307198720 ) ) ;
#5989=ORIENTED_EDGE ( 'NONE', *, *, #41771, .T. ) ;
#5991=DIRECTION ( 'NONE',  ( -1.000000000000000000, 0.000000000000000000, 0.000000000000000000 ) ) ;
#5992=CARTESIAN_POINT ( 'NONE',  ( -124.9459734468149463, 2.143131898507847836E-16, -37.43171244307205825 ) ) ;
#5994=ORIENTED_EDGE ( 'NONE', *, *, #31272, .F. ) ;
#5995=ORIENTED_EDGE ( 'NONE', *, *, #18018, .T. ) ;
#5996=CARTESIAN_POINT ( 'NONE',  ( 154.3291528190321458, 1.750000000000010214, -78.15658617722490931 ) ) ;
#5997=CARTESIAN_POINT ( 'NONE',  ( -85.67084718096784002, 1.750000000000010214, -78.15658617722490931 ) ) ;
#5998=CARTESIAN_POINT ( 'NONE',  ( -206.6959734468149463, 1.750000000000010658, 80.81828755692798438 ) ) ;
#5999=CARTESIAN_POINT ( 'NONE',  ( -84.94597344681493212, -1.025126265847089213, 42.56828755692799149 ) ) ;
#6001=VECTOR ( 'NONE', #46006, 1000.000000000000000 ) ;
#6009=DIRECTION ( 'NONE',  ( 0.000000000000000000, 0.000000000000000000, 1.000000000000000000 ) ) ;
#6010=CARTESIAN_POINT ( 'NONE',  ( -207.7210997126620384, 1.750000000000009326, -158.1565861772249377 ) ) ;
#6012=ORIENTED_EDGE ( 'NONE', *, *, #8932, .T. ) ;
#6013=CARTESIAN_POINT ( 'NONE',  ( -126.6959734468149321, 1.749999999999997113, 40.81828755692798438 ) ) ;
#6017=CARTESIAN_POINT ( 'NONE',  ( 193.3040265531851105, 0.000000000000000000, 165.0000000000000000 ) ) ;
#6021=( BOUNDED_CURVE ( )  B_SPLINE_CURVE ( 3, ( #14558, #22513, #2754, #21763 ),
 .UNSPECIFIED., .F., .F. ) 
 B_SPLINE_CURVE_WITH_KNOTS ( ( 4, 4 ),
 ( 3.141592653589793116, 4.712388980384689674 ),
 .UNSPECIFIED. ) 
 CURVE ( )  GEOMETRIC_REPRESENTATION_ITEM ( )  RATIONAL_B_SPLINE_CURVE ( ( 1.000000000000000000, 0.8047378541243649375, 0.8047378541243649375, 1.000000000000000000 ) ) 
 REPRESENTATION_ITEM ( '' )  );
#6033=CIRCLE ( 'NONE', #11801, 1.750000000000009992 ) ;
#6034=EDGE_CURVE ( 'NONE', #28309, #39980, #1894, .T. ) ;
#6036=EDGE_CURVE ( 'NONE', #10604, #36951, #45755, .T. ) ;
#6040=EDGE_CURVE ( 'NONE', #26888, #1022, #38745, .T. ) ;
#6043=CARTESIAN_POINT ( 'NONE',  ( 33.30402655318503946, 1.750000000000010658, 120.8182875569279702 ) ) ;
#6045=DIRECTION ( 'NONE',  ( -0.000000000000000000, -0.000000000000000000, -1.000000000000000000 ) ) ;
#6052=EDGE_CURVE ( 'NONE', #22572, #46647, #23849, .T. ) ;
#6053=ORIENTED_EDGE ( 'NONE', *, *, #39805, .F. ) ;
#6057=EDGE_CURVE ( 'NONE', #13717, #40787, #8453, .T. ) ;
#6060=ORIENTED_EDGE ( 'NONE', *, *, #4498, .F. ) ;
#6061=DIRECTION ( 'NONE',  ( -1.000000000000000000, -0.000000000000000000, -0.000000000000000000 ) ) ;
#6063=ORIENTED_EDGE ( 'NONE', *, *, #14408, .F. ) ;
#6064=VERTEX_POINT ( 'NONE', #12050 ) ;
#6066=CARTESIAN_POINT ( 'NONE',  ( -124.9459734468149463, 2.143131898507847836E-16, -160.9317124430720014 ) ) ;
#6067=FACE_OUTER_BOUND ( 'NONE', #28869, .T. ) ;
#6072=ORIENTED_EDGE ( 'NONE', *, *, #47432, .F. ) ;
#6074=VECTOR ( 'NONE', #18713, 1000.000000000000000 ) ;
#6080=CARTESIAN_POINT ( 'NONE',  ( 113.3040265531850537, -1.749999999999997113, 40.81828755692798438 ) ) ;
#6082=( BOUNDED_CURVE ( )  B_SPLINE_CURVE ( 3, ( #16615, #31527, #713, #4800 ),
 .UNSPECIFIED., .F., .F. ) 
 B_SPLINE_CURVE_WITH_KNOTS ( ( 4, 4 ),
 ( 1.570796326794896558, 3.141592653589793116 ),
 .UNSPECIFIED. ) 
 CURVE ( )  GEOMETRIC_REPRESENTATION_ITEM ( )  RATIONAL_B_SPLINE_CURVE ( ( 1.000000000000000000, 0.8047378541243649375, 0.8047378541243649375, 1.000000000000000000 ) ) 
 REPRESENTATION_ITEM ( '' )  );
#6086=EDGE_CURVE ( 'NONE', #4778, #37949, #47697, .T. ) ;
#6087=CARTESIAN_POINT ( 'NONE',  ( -204.9459734468148895, -1.025126265847089657, -120.9317124430720440 ) ) ;
#6091=( BOUNDED_CURVE ( )  B_SPLINE_CURVE ( 3, ( #26181, #41825, #18712, #6669 ),
 .UNSPECIFIED., .F., .F. ) 
 B_SPLINE_CURVE_WITH_KNOTS ( ( 4, 4 ),
 ( 3.141592653589793116, 4.712388980384689674 ),
 .UNSPECIFIED. ) 
 CURVE ( )  GEOMETRIC_REPRESENTATION_ITEM ( )  RATIONAL_B_SPLINE_CURVE ( ( 1.000000000000000000, 0.8047378541243649375, 0.8047378541243649375, 1.000000000000000000 ) ) 
 REPRESENTATION_ITEM ( '' )  );
#6094=EDGE_CURVE ( 'NONE', #28572, #33964, #35338, .T. ) ;
#6095=CARTESIAN_POINT ( 'NONE',  ( 210.0000000000000568, 0.000000000000000000, -157.4317124430720298 ) ) ;
#6099=EDGE_LOOP ( 'NONE', ( #43587, #31846, #9985, #46890, #4156, #9861 ) ) ;
#6103=CARTESIAN_POINT ( 'NONE',  ( 155.0540265531850537, 2.143131898507880377E-16, -40.93171244307202983 ) ) ;
#6106=EDGE_CURVE ( 'NONE', #17197, #14015, #20743, .T. ) ;
#6107=ORIENTED_EDGE ( 'NONE', *, *, #222, .F. ) ;
#6108=CARTESIAN_POINT ( 'NONE',  ( -5.670847180967843570, -1.750000000000022427, -158.1565861772249093 ) ) ;
#6109=CYLINDRICAL_SURFACE ( 'NONE', #906, 1.749999999999987566 ) ;
#6110=CARTESIAN_POINT ( 'NONE',  ( -206.6959734468149463, 1.750000000000009992, -159.1817124430720298 ) ) ;
#6111=CARTESIAN_POINT ( 'NONE',  ( 191.5540265531851105, 0.000000000000000000, 122.5682875569279702 ) ) ;
#6117=VECTOR ( 'NONE', #24580, 1000.000000000000000 ) ;
#6123=CARTESIAN_POINT ( 'NONE',  ( 75.05402655318509630, 2.143131898507880377E-16, -80.93171244307204404 ) ) ;
#6125=CARTESIAN_POINT ( 'NONE',  ( 155.0540265531850537, 2.143131898507880377E-16, 79.06828755692797017 ) ) ;
#6127=CYLINDRICAL_SURFACE ( 'NONE', #8544, 1.750000000000008438 ) ;
#6129=CARTESIAN_POINT ( 'NONE',  ( 33.30402655318503946, 1.750000000000009992, 0.8182875569279768335 ) ) ;
#6131=CARTESIAN_POINT ( 'NONE',  ( 210.0000000000000568, 2.143131898507880377E-16, 159.0682875569279702 ) ) ;
#6134=VECTOR ( 'NONE', #42620, 1000.000000000000000 ) ;
#6136=DIRECTION ( 'NONE',  ( -1.000000000000000000, -0.000000000000000000, -0.000000000000000000 ) ) ;
#6137=DIRECTION ( 'NONE',  ( 0.000000000000000000, 0.000000000000000000, -1.000000000000000000 ) ) ;
#6139=VECTOR ( 'NONE', #37000, 1000.000000000000000 ) ;
#6141=ORIENTED_EDGE ( 'NONE', *, *, #21807, .T. ) ;
#6142=CARTESIAN_POINT ( 'NONE',  ( -4.945973446814903696, 2.143131898507912917E-16, -157.4317124430720014 ) ) ;
#6144=VERTEX_POINT ( 'NONE', #32568 ) ;
#6145=CARTESIAN_POINT ( 'NONE',  ( -208.4459734468149463, 0.000000000000000000, 165.0000000000000000 ) ) ;
#6148=CARTESIAN_POINT ( 'NONE',  ( 210.0000000000000568, 0.000000000000000000, -119.1817124430720440 ) ) ;
#6150=ORIENTED_EDGE ( 'NONE', *, *, #28338, .T. ) ;
#6159=CARTESIAN_POINT ( 'NONE',  ( 193.3040265531851105, -1.750000000000010214, -39.18171244307202983 ) ) ;
#6165=ADVANCED_FACE ( 'NONE', ( #21246 ), #13036, .T. ) ;
#6168=CARTESIAN_POINT ( 'NONE',  ( -128.4459734468149179, 0.000000000000000000, 122.5682875569279418 ) ) ;
#6170=ORIENTED_EDGE ( 'NONE', *, *, #1388, .T. ) ;
#6177=ORIENTED_EDGE ( 'NONE', *, *, #14200, .T. ) ;
#6188=CARTESIAN_POINT ( 'NONE',  ( 195.0540265531851105, 2.143131898507880377E-16, 162.5682875569279702 ) ) ;
#6189=DIRECTION ( 'NONE',  ( -0.000000000000000000, -0.000000000000000000, -1.000000000000000000 ) ) ;
#6192=CARTESIAN_POINT ( 'NONE',  ( -126.6959734468149321, 1.749999999999997335, -119.1817124430720440 ) ) ;
#6198=CARTESIAN_POINT ( 'NONE',  ( 193.3040265531851105, 1.750000000000009992, 160.8182875569279702 ) ) ;
#6200=EDGE_CURVE ( 'NONE', #48473, #20980, #14617, .T. ) ;
#6202=VERTEX_POINT ( 'NONE', #5589 ) ;
#6208=CARTESIAN_POINT ( 'NONE',  ( 72.27890028733797578, 1.750000000000009548, -160.2068387089191219 ) ) ;
#6209=ORIENTED_EDGE ( 'NONE', *, *, #24456, .T. ) ;
#6212=FACE_OUTER_BOUND ( 'NONE', #36170, .T. ) ;
#6213=CARTESIAN_POINT ( 'NONE',  ( 195.0540265531851105, 2.143131898507880377E-16, 119.0682875569279702 ) ) ;
#6214=CARTESIAN_POINT ( 'NONE',  ( 113.3040265531850537, 0.000000000000000000, 165.0000000000000000 ) ) ;
#6220=CARTESIAN_POINT ( 'NONE',  ( -46.69597344681494633, -1.750000000000010214, 40.81828755692798438 ) ) ;
#6221=CARTESIAN_POINT ( 'NONE',  ( 113.3040265531850537, 0.000000000000000000, 165.0000000000000000 ) ) ;
#6224=ORIENTED_EDGE ( 'NONE', *, *, #40094, .T. ) ;
#6229=LINE ( 'NONE', #44438, #23600 ) ;
#6231=CARTESIAN_POINT ( 'NONE',  ( 210.0000000000000568, 0.000000000000000000, -39.18171244307202983 ) ) ;
#6234=CARTESIAN_POINT ( 'NONE',  ( -84.94597344681494633, 2.143131898507880377E-16, -157.4317124430720582 ) ) ;
#6235=ORIENTED_EDGE ( 'NONE', *, *, #45914, .F. ) ;
#6240=AXIS2_PLACEMENT_3D ( 'NONE', #44222, #29351, #5991 ) ;
#6241=( BOUNDED_CURVE ( )  B_SPLINE_CURVE ( 3, ( #29321, #25218, #44933, #40865 ),
 .UNSPECIFIED., .F., .F. ) 
 B_SPLINE_CURVE_WITH_KNOTS ( ( 4, 4 ),
 ( 4.712388980384689674, 6.283185307179586232 ),
 .UNSPECIFIED. ) 
 CURVE ( )  GEOMETRIC_REPRESENTATION_ITEM ( )  RATIONAL_B_SPLINE_CURVE ( ( 1.000000000000000000, 0.8047378541243649375, 0.8047378541243649375, 1.000000000000000000 ) ) 
 REPRESENTATION_ITEM ( '' )  );
#6242=CARTESIAN_POINT ( 'NONE',  ( -126.6959734468149321, -1.749999999999996891, 0.8182875569279768335 ) ) ;
#6245=VERTEX_POINT ( 'NONE', #30728 ) ;
#6247=( BOUNDED_CURVE ( )  B_SPLINE_CURVE ( 3, ( #32417, #48013, #12898, #34624 ),
 .UNSPECIFIED., .F., .F. ) 
 B_SPLINE_CURVE_WITH_KNOTS ( ( 4, 4 ),
 ( 4.712388980384689674, 6.283185307179586232 ),
 .UNSPECIFIED. ) 
 CURVE ( )  GEOMETRIC_REPRESENTATION_ITEM ( )  RATIONAL_B_SPLINE_CURVE ( ( 1.000000000000000000, 0.8047378541243649375, 0.8047378541243649375, 1.000000000000000000 ) ) 
 REPRESENTATION_ITEM ( '' )  );
#6252=EDGE_CURVE ( 'NONE', #14684, #45429, #21210, .T. ) ;
#6256=CARTESIAN_POINT ( 'NONE',  ( -207.7210997126620384, -1.750000000000009548, 41.84341382277508359 ) ) ;
#6259=( BOUNDED_CURVE ( )  B_SPLINE_CURVE ( 3, ( #21479, #24587, #41233, #13022 ),
 .UNSPECIFIED., .F., .F. ) 
 B_SPLINE_CURVE_WITH_KNOTS ( ( 4, 4 ),
 ( 0.000000000000000000, 1.570796326794896780 ),
 .UNSPECIFIED. ) 
 CURVE ( )  GEOMETRIC_REPRESENTATION_ITEM ( )  RATIONAL_B_SPLINE_CURVE ( ( 1.000000000000000000, 0.8047378541243649375, 0.8047378541243649375, 1.000000000000000000 ) ) 
 REPRESENTATION_ITEM ( '' )  );
#6266=AXIS2_PLACEMENT_3D ( 'NONE', #36389, #28170, #43800 ) ;
#6272=CARTESIAN_POINT ( 'NONE',  ( -86.69597344681494633, -1.750000000000010214, 40.81828755692798438 ) ) ;
#6279=DIRECTION ( 'NONE',  ( -0.000000000000000000, -0.000000000000000000, -1.000000000000000000 ) ) ;
#6282=ORIENTED_EDGE ( 'NONE', *, *, #41178, .T. ) ;
#6287=ORIENTED_EDGE ( 'NONE', *, *, #9924, .F. ) ;
#6288=LINE ( 'NONE', #41164, #8621 ) ;
#6293=LINE ( 'NONE', #40927, #15373 ) ;
#6297=CARTESIAN_POINT ( 'NONE',  ( -207.7210997126620384, -1.750000000000010214, -80.20683870891910772 ) ) ;
#6298=CARTESIAN_POINT ( 'NONE',  ( 153.3040265531850537, -1.750000000000009992, 160.8182875569279702 ) ) ;
#6303=CARTESIAN_POINT ( 'NONE',  ( 193.3040265531851105, 0.000000000000000000, 165.0000000000000000 ) ) ;
#6319=VECTOR ( 'NONE', #44811, 1000.000000000000000 ) ;
#6322=CYLINDRICAL_SURFACE ( 'NONE', #20833, 1.750000000000001554 ) ;
#6324=EDGE_LOOP ( 'NONE', ( #40781, #39962, #3977, #41126, #30715 ) ) ;
#6326=ORIENTED_EDGE ( 'NONE', *, *, #41178, .F. ) ;
#6328=CARTESIAN_POINT ( 'NONE',  ( -126.6959734468149321, -1.749999999999996891, -159.1817124430720298 ) ) ;
#6329=DIRECTION ( 'NONE',  ( -0.000000000000000000, -0.000000000000000000, -1.000000000000000000 ) ) ;
#6331=CARTESIAN_POINT ( 'NONE',  ( -6.695973446814940111, 1.750000000000023315, -159.1817124430720298 ) ) ;
#6332=VERTEX_POINT ( 'NONE', #30206 ) ;
#6333=( BOUNDED_CURVE ( )  B_SPLINE_CURVE ( 3, ( #23324, #49964, #46120, #38494 ),
 .UNSPECIFIED., .F., .F. ) 
 B_SPLINE_CURVE_WITH_KNOTS ( ( 4, 4 ),
 ( 0.000000000000000000, 1.570796326794896558 ),
 .UNSPECIFIED. ) 
 CURVE ( )  GEOMETRIC_REPRESENTATION_ITEM ( )  RATIONAL_B_SPLINE_CURVE ( ( 1.000000000000000000, 0.8047378541243649375, 0.8047378541243649375, 1.000000000000000000 ) ) 
 REPRESENTATION_ITEM ( '' )  );
#6338=ORIENTED_EDGE ( 'NONE', *, *, #3266, .T. ) ;
#6341=CARTESIAN_POINT ( 'NONE',  ( 210.0000000000000568, 0.000000000000000000, 40.81828755692798438 ) ) ;
#6342=CARTESIAN_POINT ( 'NONE',  ( -87.72109971266203843, 1.750000000000009326, -158.1565861772249377 ) ) ;
#6343=DIRECTION ( 'NONE',  ( -1.000000000000000000, -0.000000000000000000, -0.000000000000000000 ) ) ;
#6344=CARTESIAN_POINT ( 'NONE',  ( 111.5540265531850679, 0.000000000000000000, -165.0000000000000000 ) ) ;
#6345=CARTESIAN_POINT ( 'NONE',  ( -166.6959734468149463, -1.750000000000010214, -39.18171244307202983 ) ) ;
#6348=CARTESIAN_POINT ( 'NONE',  ( -5.670847180967843570, 1.750000000000022871, 1.843413822775074040 ) ) ;
#6350=CARTESIAN_POINT ( 'NONE',  ( 113.3040265531850537, -1.749999999999996891, 160.8182875569279702 ) ) ;
#6355=EDGE_LOOP ( 'NONE', ( #39831, #22422, #27160, #1592, #50379, #22645 ) ) ;
#6358=CARTESIAN_POINT ( 'NONE',  ( 112.2789002873379758, 1.749999999999996669, 161.8434138227750907 ) ) ;
#6361=CARTESIAN_POINT ( 'NONE',  ( 191.5540265531850537, 1.025126265847089435, 122.5682875569280128 ) ) ;
#6367=EDGE_CURVE ( 'NONE', #44970, #37221, #259, .T. ) ;
#6372=EDGE_CURVE ( 'NONE', #42683, #19177, #49157, .T. ) ;
#6373=CYLINDRICAL_SURFACE ( 'NONE', #50106, 1.750000000000008438 ) ;
#6375=VERTEX_POINT ( 'NONE', #25608 ) ;
#6381=( BOUNDED_CURVE ( )  B_SPLINE_CURVE ( 3, ( #12085, #44117, #23883, #24649 ),
 .UNSPECIFIED., .F., .F. ) 
 B_SPLINE_CURVE_WITH_KNOTS ( ( 4, 4 ),
 ( 3.141592653589793116, 4.712388980384689674 ),
 .UNSPECIFIED. ) 
 CURVE ( )  GEOMETRIC_REPRESENTATION_ITEM ( )  RATIONAL_B_SPLINE_CURVE ( ( 1.000000000000000000, 0.8047378541243649375, 0.8047378541243649375, 1.000000000000000000 ) ) 
 REPRESENTATION_ITEM ( '' )  );
#6390=( BOUNDED_CURVE ( )  B_SPLINE_CURVE ( 3, ( #36694, #32828, #520, #43593 ),
 .UNSPECIFIED., .F., .F. ) 
 B_SPLINE_CURVE_WITH_KNOTS ( ( 4, 4 ),
 ( 4.712388980384689674, 6.283185307179586232 ),
 .UNSPECIFIED. ) 
 CURVE ( )  GEOMETRIC_REPRESENTATION_ITEM ( )  RATIONAL_B_SPLINE_CURVE ( ( 1.000000000000000000, 0.8047378541243649375, 0.8047378541243649375, 1.000000000000000000 ) ) 
 REPRESENTATION_ITEM ( '' )  );
#6391=DIRECTION ( 'NONE',  ( -0.000000000000000000, -0.000000000000000000, -1.000000000000000000 ) ) ;
#6392=ORIENTED_EDGE ( 'NONE', *, *, #762, .T. ) ;
#6393=CARTESIAN_POINT ( 'NONE',  ( 75.05402655318509630, 2.143131898507880377E-16, 122.5682875569279844 ) ) ;
#6396=ORIENTED_EDGE ( 'NONE', *, *, #41535, .T. ) ;
#6399=DIRECTION ( 'NONE',  ( -1.000000000000000000, -0.000000000000000000, -0.000000000000000000 ) ) ;
#6401=EDGE_CURVE ( 'NONE', #22572, #4058, #5479, .T. ) ;
#6410=EDGE_CURVE ( 'NONE', #26079, #14709, #31736, .T. ) ;
#6412=CARTESIAN_POINT ( 'NONE',  ( -205.6708471809678827, 1.750000000000010214, 81.84341382277507648 ) ) ;
#6414=CARTESIAN_POINT ( 'NONE',  ( 113.3040265531850537, 0.000000000000000000, 165.0000000000000000 ) ) ;
#6417=ORIENTED_EDGE ( 'NONE', *, *, #16790, .T. ) ;
#6421=DIRECTION ( 'NONE',  ( -0.000000000000000000, -0.000000000000000000, -1.000000000000000000 ) ) ;
#6423=DIRECTION ( 'NONE',  ( -1.000000000000000000, -0.000000000000000000, -0.000000000000000000 ) ) ;
#6424=CARTESIAN_POINT ( 'NONE',  ( 35.05402655318504657, 1.025126265847089657, -80.93171244307201562 ) ) ;
#6427=ORIENTED_EDGE ( 'NONE', *, *, #30634, .F. ) ;
#6434=CARTESIAN_POINT ( 'NONE',  ( -7.721099712662037540, 1.750000000000023315, 41.84341382277508359 ) ) ;
#6439=CARTESIAN_POINT ( 'NONE',  ( 192.2789002873380184, 1.750000000000009548, 159.7931612910809065 ) ) ;
#6441=ORIENTED_EDGE ( 'NONE', *, *, #47534, .F. ) ;
#6446=CARTESIAN_POINT ( 'NONE',  ( 210.0000000000000568, 0.000000000000000000, 82.56828755692799859 ) ) ;
#6450=DIRECTION ( 'NONE',  ( -1.000000000000000000, -0.000000000000000000, -0.000000000000000000 ) ) ;
#6459=ORIENTED_EDGE ( 'NONE', *, *, #46034, .T. ) ;
#6470=CARTESIAN_POINT ( 'NONE',  ( 73.30402655318508209, 0.000000000000000000, 165.0000000000000000 ) ) ;
#6472=CARTESIAN_POINT ( 'NONE',  ( -7.721099712662037540, -1.750000000000023315, 39.79316129108089228 ) ) ;
#6473=EDGE_CURVE ( 'NONE', #29314, #11997, #2195, .T. ) ;
#6475=CARTESIAN_POINT ( 'NONE',  ( -210.0000000000000568, 0.000000000000000000, 82.56828755692799859 ) ) ;
#6480=FACE_OUTER_BOUND ( 'NONE', #49849, .T. ) ;
#6483=CARTESIAN_POINT ( 'NONE',  ( 210.0000000000000568, 2.143131898507881116E-16, -40.93171244307203693 ) ) ;
#6485=DIRECTION ( 'NONE',  ( 1.000000000000000000, 0.000000000000000000, 0.000000000000000000 ) ) ;
#6490=DIRECTION ( 'NONE',  ( -1.000000000000000000, 0.000000000000000000, 0.000000000000000000 ) ) ;
#6492=CARTESIAN_POINT ( 'NONE',  ( -46.69597344681494633, 1.750000000000010214, 40.81828755692798438 ) ) ;
#6495=CYLINDRICAL_SURFACE ( 'NONE', #470, 1.750000000000001554 ) ;
#6500=CIRCLE ( 'NONE', #38504, 1.750000000000015543 ) ;
#6501=ORIENTED_EDGE ( 'NONE', *, *, #39050, .T. ) ;
#6526=( BOUNDED_CURVE ( )  B_SPLINE_CURVE ( 3, ( #24299, #12966, #31996, #40187 ),
 .UNSPECIFIED., .F., .F. ) 
 B_SPLINE_CURVE_WITH_KNOTS ( ( 4, 4 ),
 ( 4.712388980384689674, 6.283185307179586232 ),
 .UNSPECIFIED. ) 
 CURVE ( )  GEOMETRIC_REPRESENTATION_ITEM ( )  RATIONAL_B_SPLINE_CURVE ( ( 1.000000000000000000, 0.8047378541243649375, 0.8047378541243649375, 1.000000000000000000 ) ) 
 REPRESENTATION_ITEM ( '' )  );
#6529=EDGE_CURVE ( 'NONE', #6375, #36250, #12673, .T. ) ;
#6536=( BOUNDED_CURVE ( )  B_SPLINE_CURVE ( 3, ( #31078, #4640, #35953, #11319 ),
 .UNSPECIFIED., .F., .F. ) 
 B_SPLINE_CURVE_WITH_KNOTS ( ( 4, 4 ),
 ( 0.000000000000000000, 1.570796326794896558 ),
 .UNSPECIFIED. ) 
 CURVE ( )  GEOMETRIC_REPRESENTATION_ITEM ( )  RATIONAL_B_SPLINE_CURVE ( ( 1.000000000000000000, 0.8047378541243649375, 0.8047378541243649375, 1.000000000000000000 ) ) 
 REPRESENTATION_ITEM ( '' )  );
#6537=CARTESIAN_POINT ( 'NONE',  ( 75.05402655318509630, 2.143131898507880377E-16, 165.0000000000000000 ) ) ;
#6539=DIRECTION ( 'NONE',  ( 0.000000000000000000, 0.000000000000000000, 1.000000000000000000 ) ) ;
#6540=LINE ( 'NONE', #30925, #19199 ) ;
#6542=EDGE_CURVE ( 'NONE', #38070, #5777, #44130, .T. ) ;
#6549=( BOUNDED_CURVE ( )  B_SPLINE_CURVE ( 3, ( #45233, #1924, #10116, #41671 ),
 .UNSPECIFIED., .F., .F. ) 
 B_SPLINE_CURVE_WITH_KNOTS ( ( 4, 4 ),
 ( 0.000000000000000000, 1.570796326794896780 ),
 .UNSPECIFIED. ) 
 CURVE ( )  GEOMETRIC_REPRESENTATION_ITEM ( )  RATIONAL_B_SPLINE_CURVE ( ( 1.000000000000000000, 0.8047378541243649375, 0.8047378541243649375, 1.000000000000000000 ) ) 
 REPRESENTATION_ITEM ( '' )  );
#6555=CARTESIAN_POINT ( 'NONE',  ( -205.6708471809678827, -1.750000000000009548, -160.2068387089191219 ) ) ;
#6557=VERTEX_POINT ( 'NONE', #28892 ) ;
#6561=CARTESIAN_POINT ( 'NONE',  ( -44.94597344681493922, 2.143131898507880377E-16, 165.0000000000000000 ) ) ;
#6565=CARTESIAN_POINT ( 'NONE',  ( -44.94597344681497475, 0.000000000000000000, 162.5682875569279702 ) ) ;
#6566=CARTESIAN_POINT ( 'NONE',  ( -206.6959734468149463, 1.750000000000010658, -119.1817124430720440 ) ) ;
#6573=CARTESIAN_POINT ( 'NONE',  ( -205.6708471809678827, 1.750000000000009548, -38.15658617722494483 ) ) ;
#6574=CARTESIAN_POINT ( 'NONE',  ( -88.44597344681497475, 0.000000000000000000, 2.568287556928006143 ) ) ;
#6580=CARTESIAN_POINT ( 'NONE',  ( -48.44597344681496054, -1.025126265847089879, -117.4317124430720156 ) ) ;
#6587=DIRECTION ( 'NONE',  ( -0.000000000000000000, -0.000000000000000000, -1.000000000000000000 ) ) ;
#6597=AXIS2_PLACEMENT_3D ( 'NONE', #32525, #48106, #16346 ) ;
#6598=CARTESIAN_POINT ( 'NONE',  ( 111.5540265531850679, 0.000000000000000000, -157.4317124430720582 ) ) ;
#6599=AXIS2_PLACEMENT_3D ( 'NONE', #29273, #1072, #25424 ) ;
#6600=DIRECTION ( 'NONE',  ( -1.000000000000000000, 0.000000000000000000, 0.000000000000000000 ) ) ;
#6603=DIRECTION ( 'NONE',  ( -0.000000000000000000, -0.000000000000000000, -1.000000000000000000 ) ) ;
#6606=CARTESIAN_POINT ( 'NONE',  ( -84.94597344681493212, 1.025126265847089435, -157.4317124430720582 ) ) ;
#6608=CARTESIAN_POINT ( 'NONE',  ( 111.5540265531850679, 0.000000000000000000, -77.43171244307204404 ) ) ;
#6610=DIRECTION ( 'NONE',  ( -1.000000000000000000, 0.000000000000000000, 0.000000000000000000 ) ) ;
#6611=ORIENTED_EDGE ( 'NONE', *, *, #44325, .F. ) ;
#6612=CARTESIAN_POINT ( 'NONE',  ( 111.5540265531850537, 1.025126265847081442, 162.5682875569279133 ) ) ;
#6614=DIRECTION ( 'NONE',  ( -0.000000000000000000, -0.000000000000000000, -1.000000000000000000 ) ) ;
#6615=CARTESIAN_POINT ( 'NONE',  ( -44.94597344681493922, -1.025126265847089435, -40.93171244307204404 ) ) ;
#6617=DIRECTION ( 'NONE',  ( -0.000000000000000000, -0.000000000000000000, -1.000000000000000000 ) ) ;
#6624=( BOUNDED_CURVE ( )  B_SPLINE_CURVE ( 3, ( #23376, #16190, #19774, #35454 ),
 .UNSPECIFIED., .F., .F. ) 
 B_SPLINE_CURVE_WITH_KNOTS ( ( 4, 4 ),
 ( 0.000000000000000000, 1.570796326794896558 ),
 .UNSPECIFIED. ) 
 CURVE ( )  GEOMETRIC_REPRESENTATION_ITEM ( )  RATIONAL_B_SPLINE_CURVE ( ( 1.000000000000000000, 0.8047378541243649375, 0.8047378541243649375, 1.000000000000000000 ) ) 
 REPRESENTATION_ITEM ( '' )  );
#6628=CYLINDRICAL_SURFACE ( 'NONE', #13662, 1.750000000000008438 ) ;
#6630=CARTESIAN_POINT ( 'NONE',  ( -44.94597344681493922, 2.143131898507880377E-16, -37.43171244307200141 ) ) ;
#6637=CARTESIAN_POINT ( 'NONE',  ( 210.0000000000000568, 0.000000000000000000, -79.18171244307201562 ) ) ;
#6645=ORIENTED_EDGE ( 'NONE', *, *, #42734, .F. ) ;
#6655=DIRECTION ( 'NONE',  ( -0.000000000000000000, -0.000000000000000000, -1.000000000000000000 ) ) ;
#6658=EDGE_CURVE ( 'NONE', #21408, #36017, #8882, .T. ) ;
#6665=CARTESIAN_POINT ( 'NONE',  ( 33.30402655318503946, -1.750000000000010658, 80.81828755692798438 ) ) ;
#6669=CARTESIAN_POINT ( 'NONE',  ( -86.69597344681494633, -1.750000000000010214, -39.18171244307202983 ) ) ;
#6670=CARTESIAN_POINT ( 'NONE',  ( 33.30402655318503946, 1.750000000000010658, -79.18171244307201562 ) ) ;
#6671=ADVANCED_FACE ( 'NONE', ( #32747 ), #48340, .T. ) ;
#6672=EDGE_CURVE ( 'NONE', #37522, #42553, #32026, .T. ) ;
#6678=( BOUNDED_CURVE ( )  B_SPLINE_CURVE ( 3, ( #22047, #13827, #37721, #9738 ),
 .UNSPECIFIED., .F., .F. ) 
 B_SPLINE_CURVE_WITH_KNOTS ( ( 4, 4 ),
 ( 0.000000000000000000, 1.570796326794896780 ),
 .UNSPECIFIED. ) 
 CURVE ( )  GEOMETRIC_REPRESENTATION_ITEM ( )  RATIONAL_B_SPLINE_CURVE ( ( 1.000000000000000000, 0.8047378541243649375, 0.8047378541243649375, 1.000000000000000000 ) ) 
 REPRESENTATION_ITEM ( '' )  );
#6681=DIRECTION ( 'NONE',  ( -1.000000000000000000, -0.000000000000000000, -0.000000000000000000 ) ) ;
#6685=CYLINDRICAL_SURFACE ( 'NONE', #29004, 1.750000000000015543 ) ;
#6686=( BOUNDED_CURVE ( )  B_SPLINE_CURVE ( 3, ( #12270, #20988, #39741, #13268 ),
 .UNSPECIFIED., .F., .F. ) 
 B_SPLINE_CURVE_WITH_KNOTS ( ( 4, 4 ),
 ( 1.570796326794896558, 3.141592653589793116 ),
 .UNSPECIFIED. ) 
 CURVE ( )  GEOMETRIC_REPRESENTATION_ITEM ( )  RATIONAL_B_SPLINE_CURVE ( ( 1.000000000000000000, 0.8047378541243649375, 0.8047378541243649375, 1.000000000000000000 ) ) 
 REPRESENTATION_ITEM ( '' )  );
#6694=EDGE_LOOP ( 'NONE', ( #26065, #24713, #33988, #48027, #47760, #3493 ) ) ;
#6696=DIRECTION ( 'NONE',  ( -1.000000000000000000, 0.000000000000000000, 0.000000000000000000 ) ) ;
#6699=AXIS2_PLACEMENT_3D ( 'NONE', #1550, #8992, #21801 ) ;
#6706=CARTESIAN_POINT ( 'NONE',  ( -87.72109971266203843, 1.750000000000009548, 39.79316129108089228 ) ) ;
#6714=ORIENTED_EDGE ( 'NONE', *, *, #47843, .T. ) ;
#6716=CARTESIAN_POINT ( 'NONE',  ( 75.05402655318509630, 1.025126265847089657, -120.9317124430720440 ) ) ;
#6717=CARTESIAN_POINT ( 'NONE',  ( -44.94597344681493922, -1.025126265847089435, 162.5682875569279133 ) ) ;
#6721=DIRECTION ( 'NONE',  ( 0.000000000000000000, 0.000000000000000000, 1.000000000000000000 ) ) ;
#6723=LINE ( 'NONE', #2858, #14130 ) ;
#6727=LINE ( 'NONE', #49777, #20408 ) ;
#6734=EDGE_LOOP ( 'NONE', ( #635, #47451, #7310, #5661, #30992, #14840 ) ) ;
#6738=CARTESIAN_POINT ( 'NONE',  ( -207.7210997126620384, -1.750000000000010214, -78.15658617722490931 ) ) ;
#6739=VERTEX_POINT ( 'NONE', #10644 ) ;
#6741=AXIS2_PLACEMENT_3D ( 'NONE', #13315, #21274, #17177 ) ;
#6746=DIRECTION ( 'NONE',  ( -1.000000000000000000, -0.000000000000000000, -0.000000000000000000 ) ) ;
#6752=EDGE_CURVE ( 'NONE', #24640, #14882, #22699, .T. ) ;
#6753=EDGE_CURVE ( 'NONE', #5437, #36214, #23162, .T. ) ;
#6770=MECHANICAL_DESIGN_GEOMETRIC_PRESENTATION_REPRESENTATION('',(#28896),#45071);
#6771=VERTEX_POINT ( 'NONE', #14235 ) ;
#6773=AXIS2_PLACEMENT_3D ( 'NONE', #44817, #1499, #49146 ) ;
#6779=CARTESIAN_POINT ( 'NONE',  ( 35.05402655318504657, 2.143131898507880377E-16, 165.0000000000000000 ) ) ;
#6781=ORIENTED_EDGE ( 'NONE', *, *, #44542, .F. ) ;
#6783=DIRECTION ( 'NONE',  ( -1.000000000000000000, 0.000000000000000000, 0.000000000000000000 ) ) ;
#6787=CARTESIAN_POINT ( 'NONE',  ( 210.0000000000000568, 2.143131898507881856E-16, 79.06828755692797017 ) ) ;
#6794=DIRECTION ( 'NONE',  ( 1.000000000000000000, 0.000000000000000000, 0.000000000000000000 ) ) ;
#6795=FACE_OUTER_BOUND ( 'NONE', #16561, .T. ) ;
#6796=CYLINDRICAL_SURFACE ( 'NONE', #35174, 1.750000000000001554 ) ;
#6797=CARTESIAN_POINT ( 'NONE',  ( -86.69597344681494633, -1.750000000000009992, -159.1817124430720298 ) ) ;
#6807=CARTESIAN_POINT ( 'NONE',  ( -8.445973446814976526, 0.000000000000000000, -40.93171244307205825 ) ) ;
#6808=AXIS2_PLACEMENT_3D ( 'NONE', #38107, #41685, #30144 ) ;
#6809=ORIENTED_EDGE ( 'NONE', *, *, #40032, .T. ) ;
#6814=ADVANCED_FACE ( 'NONE', ( #15515 ), #34789, .T. ) ;
#6816=ORIENTED_EDGE ( 'NONE', *, *, #22360, .T. ) ;
#6820=LINE ( 'NONE', #18852, #7874 ) ;
#6823=ORIENTED_EDGE ( 'NONE', *, *, #31272, .T. ) ;
#6827=LINE ( 'NONE', #42977, #36570 ) ;
#6830=( BOUNDED_CURVE ( )  B_SPLINE_CURVE ( 3, ( #39925, #27865, #32221, #31973 ),
 .UNSPECIFIED., .F., .F. ) 
 B_SPLINE_CURVE_WITH_KNOTS ( ( 4, 4 ),
 ( 0.000000000000000000, 1.570796326794896558 ),
 .UNSPECIFIED. ) 
 CURVE ( )  GEOMETRIC_REPRESENTATION_ITEM ( )  RATIONAL_B_SPLINE_CURVE ( ( 1.000000000000000000, 0.8047378541243649375, 0.8047378541243649375, 1.000000000000000000 ) ) 
 REPRESENTATION_ITEM ( '' )  );
#6831=ORIENTED_EDGE ( 'NONE', *, *, #26303, .F. ) ;
#6832=CARTESIAN_POINT ( 'NONE',  ( -207.7210997126620384, -1.750000000000010214, 81.84341382277507648 ) ) ;
#6833=CARTESIAN_POINT ( 'NONE',  ( -204.9459734468148895, 1.025126265847089435, 2.568287556927986159 ) ) ;
#6834=CARTESIAN_POINT ( 'NONE',  ( -47.72109971266203132, -1.750000000000010214, -118.1565861772249519 ) ) ;
#6837=CARTESIAN_POINT ( 'NONE',  ( -8.445973446814976526, 0.000000000000000000, 39.06828755692792754 ) ) ;
#6838=( BOUNDED_CURVE ( )  B_SPLINE_CURVE ( 3, ( #4627, #47176, #8482, #27470 ),
 .UNSPECIFIED., .F., .F. ) 
 B_SPLINE_CURVE_WITH_KNOTS ( ( 4, 4 ),
 ( 3.141592653589793116, 4.712388980384689674 ),
 .UNSPECIFIED. ) 
 CURVE ( )  GEOMETRIC_REPRESENTATION_ITEM ( )  RATIONAL_B_SPLINE_CURVE ( ( 1.000000000000000000, 0.8047378541243649375, 0.8047378541243649375, 1.000000000000000000 ) ) 
 REPRESENTATION_ITEM ( '' )  );
#6841=CARTESIAN_POINT ( 'NONE',  ( -48.44597344681496054, 1.025126265847089435, -40.93171244307204404 ) ) ;
#6842=VERTEX_POINT ( 'NONE', #7570 ) ;
#6844=DIRECTION ( 'NONE',  ( -1.000000000000000000, -0.000000000000000000, -0.000000000000000000 ) ) ;
#6847=LINE ( 'NONE', #10943, #749 ) ;
#6848=AXIS2_PLACEMENT_3D ( 'NONE', #12713, #12953, #24784 ) ;
#6850=DIRECTION ( 'NONE',  ( -1.000000000000000000, -0.000000000000000000, -0.000000000000000000 ) ) ;
#6854=( BOUNDED_CURVE ( )  B_SPLINE_CURVE ( 3, ( #45923, #10804, #6962, #46430 ),
 .UNSPECIFIED., .F., .F. ) 
 B_SPLINE_CURVE_WITH_KNOTS ( ( 4, 4 ),
 ( 3.141592653589793116, 4.712388980384689674 ),
 .UNSPECIFIED. ) 
 CURVE ( )  GEOMETRIC_REPRESENTATION_ITEM ( )  RATIONAL_B_SPLINE_CURVE ( ( 1.000000000000000000, 0.8047378541243649375, 0.8047378541243649375, 1.000000000000000000 ) ) 
 REPRESENTATION_ITEM ( '' )  );
#6859=ORIENTED_EDGE ( 'NONE', *, *, #46926, .T. ) ;
#6864=ORIENTED_EDGE ( 'NONE', *, *, #14260, .F. ) ;
#6865=CARTESIAN_POINT ( 'NONE',  ( 195.0540265531851105, 2.143131898507880377E-16, 82.56828755692798438 ) ) ;
#6868=ORIENTED_EDGE ( 'NONE', *, *, #46653, .T. ) ;
#6869=CARTESIAN_POINT ( 'NONE',  ( -48.44597344681496054, -1.025126265847089435, 39.06828755692797728 ) ) ;
#6870=CARTESIAN_POINT ( 'NONE',  ( -164.9459734468149463, 2.143131898507880377E-16, 79.06828755692797017 ) ) ;
#6872=CARTESIAN_POINT ( 'NONE',  ( -87.72109971266203843, 1.750000000000009548, 41.84341382277508359 ) ) ;
#6874=DIRECTION ( 'NONE',  ( 0.000000000000000000, 0.000000000000000000, 1.000000000000000000 ) ) ;
#6880=CARTESIAN_POINT ( 'NONE',  ( -128.4459734468149463, 1.025126265847081886, 39.06828755692799149 ) ) ;
#6890=EDGE_CURVE ( 'NONE', #47659, #12079, #23481, .T. ) ;
#6891=ADVANCED_FACE ( 'NONE', ( #8083 ), #42444, .T. ) ;
#6896=ORIENTED_EDGE ( 'NONE', *, *, #24569, .F. ) ;
#6897=ORIENTED_EDGE ( 'NONE', *, *, #39672, .F. ) ;
#6898=EDGE_LOOP ( 'NONE', ( #33958, #7577, #23608, #21034, #41757 ) ) ;
#6904=CARTESIAN_POINT ( 'NONE',  ( 74.32915281903215998, -1.750000000000009548, 121.8434138227750623 ) ) ;
#6906=CARTESIAN_POINT ( 'NONE',  ( -88.44597344681497475, 0.000000000000000000, 119.0682875569279418 ) ) ;
#6910=CARTESIAN_POINT ( 'NONE',  ( 71.55402655318505367, -1.025126265847089879, 82.56828755692798438 ) ) ;
#6911=DIRECTION ( 'NONE',  ( -0.000000000000000000, -0.000000000000000000, -1.000000000000000000 ) ) ;
#6915=CARTESIAN_POINT ( 'NONE',  ( -6.695973446814940111, 1.750000000000024203, 80.81828755692798438 ) ) ;
#6917=VECTOR ( 'NONE', #25895, 1000.000000000000000 ) ;
#6919=DIRECTION ( 'NONE',  ( 0.000000000000000000, 0.000000000000000000, 1.000000000000000000 ) ) ;
#6920=EDGE_LOOP ( 'NONE', ( #13462, #46064, #40915, #35482, #37027, #868 ) ) ;
#6926=VECTOR ( 'NONE', #45420, 1000.000000000000000 ) ;
#6930=CARTESIAN_POINT ( 'NONE',  ( 153.3040265531850537, 0.000000000000000000, 165.0000000000000000 ) ) ;
#6935=CARTESIAN_POINT ( 'NONE',  ( -206.6959734468149463, 0.000000000000000000, 165.0000000000000000 ) ) ;
#6938=AXIS2_PLACEMENT_3D ( 'NONE', #5273, #47827, #21172 ) ;
#6943=VECTOR ( 'NONE', #26486, 1000.000000000000000 ) ;
#6947=CARTESIAN_POINT ( 'NONE',  ( -47.72109971266203132, -1.750000000000010214, -80.20683870891910772 ) ) ;
#6949=ORIENTED_EDGE ( 'NONE', *, *, #34297, .T. ) ;
#6959=FACE_OUTER_BOUND ( 'NONE', #21472, .T. ) ;
#6961=AXIS2_PLACEMENT_3D ( 'NONE', #14530, #6844, #17871 ) ;
#6962=CARTESIAN_POINT ( 'NONE',  ( 34.32915281903212446, -1.750000000000009326, -158.1565861772249377 ) ) ;
#6966=ORIENTED_EDGE ( 'NONE', *, *, #43237, .F. ) ;
#6983=CARTESIAN_POINT ( 'NONE',  ( -164.9459734468149463, 2.143131898507880377E-16, 2.568287556927978166 ) ) ;
#6992=VERTEX_POINT ( 'NONE', #28834 ) ;
#6993=DIRECTION ( 'NONE',  ( -1.000000000000000000, -0.000000000000000000, -0.000000000000000000 ) ) ;
#6995=( BOUNDED_CURVE ( )  B_SPLINE_CURVE ( 3, ( #36146, #32042, #5328, #4812 ),
 .UNSPECIFIED., .F., .F. ) 
 B_SPLINE_CURVE_WITH_KNOTS ( ( 4, 4 ),
 ( 1.570796326794896558, 3.141592653589793116 ),
 .UNSPECIFIED. ) 
 CURVE ( )  GEOMETRIC_REPRESENTATION_ITEM ( )  RATIONAL_B_SPLINE_CURVE ( ( 1.000000000000000000, 0.8047378541243649375, 0.8047378541243649375, 1.000000000000000000 ) ) 
 REPRESENTATION_ITEM ( '' )  );
#6997=CARTESIAN_POINT ( 'NONE',  ( 192.2789002873380184, -1.750000000000009548, -158.1565861772249377 ) ) ;
#7001=ORIENTED_EDGE ( 'NONE', *, *, #26488, .T. ) ;
#7004=CARTESIAN_POINT ( 'NONE',  ( -128.4459734468149463, -1.025126265847081664, 2.568287556927973281 ) ) ;
#7011=EDGE_CURVE ( 'NONE', #38516, #12576, #35810, .T. ) ;
#7012=VERTEX_POINT ( 'NONE', #40141 ) ;
#7013=EDGE_CURVE ( 'NONE', #10841, #48741, #23901, .T. ) ;
#7014=VERTEX_POINT ( 'NONE', #32957 ) ;
#7015=CARTESIAN_POINT ( 'NONE',  ( -4.945973446814903696, 2.143131898507912917E-16, -157.4317124430720014 ) ) ;
#7021=EDGE_CURVE ( 'NONE', #3215, #33964, #44425, .T. ) ;
#7033=ORIENTED_EDGE ( 'NONE', *, *, #8020, .T. ) ;
#7035=DIRECTION ( 'NONE',  ( -0.000000000000000000, -0.000000000000000000, -1.000000000000000000 ) ) ;
#7036=VERTEX_POINT ( 'NONE', #36047 ) ;
#7039=AXIS2_PLACEMENT_3D ( 'NONE', #2738, #38174, #34065 ) ;
#7041=CYLINDRICAL_SURFACE ( 'NONE', #48743, 1.750000000000015543 ) ;
#7045=CARTESIAN_POINT ( 'NONE',  ( 113.3040265531850537, -1.749999999999997113, -39.18171244307202983 ) ) ;
#7048=DIRECTION ( 'NONE',  ( -0.000000000000000000, -0.000000000000000000, -1.000000000000000000 ) ) ;
#7050=CARTESIAN_POINT ( 'NONE',  ( 155.0540265531850537, 2.143131898507880377E-16, 119.0682875569279702 ) ) ;
#7057=EDGE_CURVE ( 'NONE', #36214, #38997, #14314, .T. ) ;
#7064=ORIENTED_EDGE ( 'NONE', *, *, #11770, .T. ) ;
#7066=DIRECTION ( 'NONE',  ( 0.000000000000000000, 0.000000000000000000, 1.000000000000000000 ) ) ;
#7071=EDGE_LOOP ( 'NONE', ( #32883, #14586, #31441, #8056, #17554 ) ) ;
#7072=EDGE_CURVE ( 'NONE', #10836, #29314, #38926, .T. ) ;
#7074=CIRCLE ( 'NONE', #46377, 1.750000000000001554 ) ;
#7076=EDGE_CURVE ( 'NONE', #46979, #1473, #50064, .T. ) ;
#7077=ORIENTED_EDGE ( 'NONE', *, *, #18745, .F. ) ;
#7079=VERTEX_POINT ( 'NONE', #4727 ) ;
#7080=CARTESIAN_POINT ( 'NONE',  ( -84.94597344681497475, 0.000000000000000000, 162.5682875569279702 ) ) ;
#7081=FACE_OUTER_BOUND ( 'NONE', #49441, .T. ) ;
#7082=ORIENTED_EDGE ( 'NONE', *, *, #46969, .T. ) ;
#7086=CARTESIAN_POINT ( 'NONE',  ( -8.445973446814964092, -1.025126265847097651, 122.5682875569280128 ) ) ;
#7089=DIRECTION ( 'NONE',  ( -0.000000000000000000, -0.000000000000000000, -1.000000000000000000 ) ) ;
#7090=VECTOR ( 'NONE', #19056, 1000.000000000000000 ) ;
#7097=CARTESIAN_POINT ( 'NONE',  ( -46.69597344681494633, 1.750000000000010214, -39.18171244307202983 ) ) ;
#7098=ORIENTED_EDGE ( 'NONE', *, *, #45095, .F. ) ;
#7100=CARTESIAN_POINT ( 'NONE',  ( 74.32915281903215998, 1.750000000000009548, -160.2068387089191219 ) ) ;
#7101=CARTESIAN_POINT ( 'NONE',  ( 153.3040265531850537, 1.750000000000010658, -119.1817124430720440 ) ) ;
#7105=EDGE_CURVE ( 'NONE', #23986, #41219, #12962, .T. ) ;
#7106=LINE ( 'NONE', #2985, #15070 ) ;
#7107=VERTEX_POINT ( 'NONE', #33701 ) ;
#7110=CARTESIAN_POINT ( 'NONE',  ( -124.9459734468149463, 2.143131898507847836E-16, -37.43171244307205825 ) ) ;
#7118=CYLINDRICAL_SURFACE ( 'NONE', #25047, 1.750000000000001554 ) ;
#7120=ADVANCED_FACE ( 'NONE', ( #45456 ), #10350, .T. ) ;
#7121=EDGE_CURVE ( 'NONE', #4802, #24870, #29612, .T. ) ;
#7123=CARTESIAN_POINT ( 'NONE',  ( 210.0000000000000568, 0.000000000000000000, 120.8182875569279702 ) ) ;
#7125=CARTESIAN_POINT ( 'NONE',  ( -4.945973446814903696, 2.143131898507912917E-16, -77.43171244307198720 ) ) ;
#7127=CARTESIAN_POINT ( 'NONE',  ( 111.5540265531850537, 0.000000000000000000, 162.5682875569279702 ) ) ;
#7137=( BOUNDED_CURVE ( )  B_SPLINE_CURVE ( 3, ( #32252, #33014, #44271, #12978 ),
 .UNSPECIFIED., .F., .F. ) 
 B_SPLINE_CURVE_WITH_KNOTS ( ( 4, 4 ),
 ( 3.141592653589793116, 4.712388980384689674 ),
 .UNSPECIFIED. ) 
 CURVE ( )  GEOMETRIC_REPRESENTATION_ITEM ( )  RATIONAL_B_SPLINE_CURVE ( ( 1.000000000000000000, 0.8047378541243649375, 0.8047378541243649375, 1.000000000000000000 ) ) 
 REPRESENTATION_ITEM ( '' )  );
#7141=LINE ( 'NONE', #15087, #36015 ) ;
#7142=( BOUNDED_CURVE ( )  B_SPLINE_CURVE ( 3, ( #34653, #46655, #30804, #26184 ),
 .UNSPECIFIED., .F., .F. ) 
 B_SPLINE_CURVE_WITH_KNOTS ( ( 4, 4 ),
 ( 1.570796326794896558, 3.141592653589793116 ),
 .UNSPECIFIED. ) 
 CURVE ( )  GEOMETRIC_REPRESENTATION_ITEM ( )  RATIONAL_B_SPLINE_CURVE ( ( 1.000000000000000000, 0.8047378541243649375, 0.8047378541243649375, 1.000000000000000000 ) ) 
 REPRESENTATION_ITEM ( '' )  );
#7151=EDGE_LOOP ( 'NONE', ( #4995, #47656, #11427, #25624, #20511, #3983 ) ) ;
#7154=CARTESIAN_POINT ( 'NONE',  ( 210.0000000000000568, 2.143131898507880377E-16, 159.0682875569279702 ) ) ;
#7155=( BOUNDED_CURVE ( )  B_SPLINE_CURVE ( 3, ( #24230, #39891, #23200, #16269 ),
 .UNSPECIFIED., .F., .F. ) 
 B_SPLINE_CURVE_WITH_KNOTS ( ( 4, 4 ),
 ( 0.000000000000000000, 1.570796326794896558 ),
 .UNSPECIFIED. ) 
 CURVE ( )  GEOMETRIC_REPRESENTATION_ITEM ( )  RATIONAL_B_SPLINE_CURVE ( ( 1.000000000000000000, 0.8047378541243649375, 0.8047378541243649375, 1.000000000000000000 ) ) 
 REPRESENTATION_ITEM ( '' )  );
#7159=CYLINDRICAL_SURFACE ( 'NONE', #24996, 1.749999999999987566 ) ;
#7160=CARTESIAN_POINT ( 'NONE',  ( 113.3040265531850537, 1.749999999999997335, 80.81828755692798438 ) ) ;
#7162=CYLINDRICAL_SURFACE ( 'NONE', #26825, 1.749999999999987566 ) ;
#7163=CARTESIAN_POINT ( 'NONE',  ( -88.44597344681497475, 0.000000000000000000, 82.56828755692801280 ) ) ;
#7165=CARTESIAN_POINT ( 'NONE',  ( 33.30402655318503946, -1.750000000000010214, -39.18171244307202983 ) ) ;
#7166=CARTESIAN_POINT ( 'NONE',  ( -206.6959734468149463, 0.000000000000000000, 165.0000000000000000 ) ) ;
#7169=VERTEX_POINT ( 'NONE', #5983 ) ;
#7170=DIRECTION ( 'NONE',  ( -0.000000000000000000, -0.000000000000000000, -1.000000000000000000 ) ) ;
#7174=CARTESIAN_POINT ( 'NONE',  ( 112.2789002873379758, 1.749999999999996225, 1.843413822775058497 ) ) ;
#7177=DIRECTION ( 'NONE',  ( -1.000000000000000000, -0.000000000000000000, -0.000000000000000000 ) ) ;
#7181=CARTESIAN_POINT ( 'NONE',  ( -128.4459734468149463, 1.025126265847081664, 122.5682875569279702 ) ) ;
#7184=EDGE_CURVE ( 'NONE', #36250, #43432, #35481, .T. ) ;
#7185=ORIENTED_EDGE ( 'NONE', *, *, #31190, .T. ) ;
#7188=CARTESIAN_POINT ( 'NONE',  ( 71.55402655318505367, 0.000000000000000000, 42.56828755692799859 ) ) ;
#7189=ORIENTED_EDGE ( 'NONE', *, *, #13566, .T. ) ;
#7192=CARTESIAN_POINT ( 'NONE',  ( 210.0000000000000568, 0.000000000000000000, -119.1817124430720440 ) ) ;
#7193=ORIENTED_EDGE ( 'NONE', *, *, #49595, .F. ) ;
#7201=CARTESIAN_POINT ( 'NONE',  ( 210.0000000000000568, 2.143131898507881856E-16, 79.06828755692797017 ) ) ;
#7203=CARTESIAN_POINT ( 'NONE',  ( -46.69597344681494633, 1.750000000000009992, 0.8182875569279768335 ) ) ;
#7206=CYLINDRICAL_SURFACE ( 'NONE', #49611, 1.750000000000001554 ) ;
#7213=CARTESIAN_POINT ( 'NONE',  ( 210.0000000000000568, 0.000000000000000000, 120.8182875569279702 ) ) ;
#7214=EDGE_CURVE ( 'NONE', #47457, #48103, #7745, .T. ) ;
#7218=EDGE_CURVE ( 'NONE', #10836, #2436, #10717, .T. ) ;
#7220=CARTESIAN_POINT ( 'NONE',  ( -128.4459734468149179, 0.000000000000000000, -77.43171244307204404 ) ) ;
#7223=VERTEX_POINT ( 'NONE', #23415 ) ;
#7225=CARTESIAN_POINT ( 'NONE',  ( 113.3040265531850537, 1.749999999999996891, 0.8182875569279768335 ) ) ;
#7238=CARTESIAN_POINT ( 'NONE',  ( 195.0540265531851105, 2.143131898507880377E-16, 119.0682875569279702 ) ) ;
#7245=ORIENTED_EDGE ( 'NONE', *, *, #13949, .F. ) ;
#7246=ADVANCED_FACE ( 'NONE', ( #19296 ), #35226, .T. ) ;
#7247=LINE ( 'NONE', #14168, #1635 ) ;
#7252=DIRECTION ( 'NONE',  ( 0.000000000000000000, 0.000000000000000000, 1.000000000000000000 ) ) ;
#7255=CARTESIAN_POINT ( 'NONE',  ( 193.3040265531851105, -1.750000000000009992, 160.8182875569279702 ) ) ;
#7256=CARTESIAN_POINT ( 'NONE',  ( 210.0000000000000568, 0.000000000000000000, -39.18171244307202983 ) ) ;
#7261=CARTESIAN_POINT ( 'NONE',  ( 113.3040265531850537, -1.749999999999997335, -79.18171244307201562 ) ) ;
#7265=CARTESIAN_POINT ( 'NONE',  ( 75.05402655318509630, 1.025126265847089213, -0.9317124430720324924 ) ) ;
#7267=CYLINDRICAL_SURFACE ( 'NONE', #19020, 1.750000000000001554 ) ;
#7270=EDGE_LOOP ( 'NONE', ( #25862, #6224, #367, #44266, #66, #9102 ) ) ;
#7277=VERTEX_POINT ( 'NONE', #11612 ) ;
#7278=ORIENTED_EDGE ( 'NONE', *, *, #8105, .F. ) ;
#7281=DIRECTION ( 'NONE',  ( -0.000000000000000000, -0.000000000000000000, -1.000000000000000000 ) ) ;
#7287=CARTESIAN_POINT ( 'NONE',  ( -206.6959734468149463, 1.750000000000009992, 0.8182875569279768335 ) ) ;
#7290=CARTESIAN_POINT ( 'NONE',  ( 210.0000000000000568, 0.000000000000000000, 160.8182875569279702 ) ) ;
#7291=CARTESIAN_POINT ( 'NONE',  ( 210.0000000000000568, 2.143131898507881116E-16, -40.93171244307203693 ) ) ;
#7292=ORIENTED_EDGE ( 'NONE', *, *, #22439, .T. ) ;
#7295=( BOUNDED_CURVE ( )  B_SPLINE_CURVE ( 3, ( #6111, #6361, #5859, #44831 ),
 .UNSPECIFIED., .F., .F. ) 
 B_SPLINE_CURVE_WITH_KNOTS ( ( 4, 4 ),
 ( 3.141592653589793116, 4.712388980384689674 ),
 .UNSPECIFIED. ) 
 CURVE ( )  GEOMETRIC_REPRESENTATION_ITEM ( )  RATIONAL_B_SPLINE_CURVE ( ( 1.000000000000000000, 0.8047378541243649375, 0.8047378541243649375, 1.000000000000000000 ) ) 
 REPRESENTATION_ITEM ( '' )  );
#7299=AXIS2_PLACEMENT_3D ( 'NONE', #39823, #317, #20301 ) ;
#7304=ORIENTED_EDGE ( 'NONE', *, *, #23469, .F. ) ;
#7310=ORIENTED_EDGE ( 'NONE', *, *, #44305, .T. ) ;
#7312=FACE_OUTER_BOUND ( 'NONE', #1243, .T. ) ;
#7315=CARTESIAN_POINT ( 'NONE',  ( 73.30402655318508209, 1.750000000000010658, -119.1817124430720440 ) ) ;
#7317=ADVANCED_FACE ( 'NONE', ( #18777 ), #31376, .T. ) ;
#7318=VERTEX_POINT ( 'NONE', #46967 ) ;
#7322=CARTESIAN_POINT ( 'NONE',  ( 71.55402655318505367, 0.000000000000000000, 119.0682875569279560 ) ) ;
#7326=CARTESIAN_POINT ( 'NONE',  ( -46.69597344681494633, 1.750000000000010214, -39.18171244307202983 ) ) ;
#7331=ORIENTED_EDGE ( 'NONE', *, *, #22390, .F. ) ;
#7332=EDGE_CURVE ( 'NONE', #24760, #36401, #15981, .T. ) ;
#7337=CARTESIAN_POINT ( 'NONE',  ( -86.69597344681494633, 1.750000000000009992, 160.8182875569279702 ) ) ;
#7352=ADVANCED_FACE ( 'NONE', ( #8527 ), #48906, .T. ) ;
#7353=CARTESIAN_POINT ( 'NONE',  ( 210.0000000000000568, 0.000000000000000000, 160.8182875569279702 ) ) ;
#7355=VERTEX_POINT ( 'NONE', #13790 ) ;
#7357=FACE_OUTER_BOUND ( 'NONE', #24249, .T. ) ;
#7358=CARTESIAN_POINT ( 'NONE',  ( -44.94597344681493922, 2.143131898507880377E-16, 2.568287556927978166 ) ) ;
#7361=LINE ( 'NONE', #49885, #2863 ) ;
#7363=CARTESIAN_POINT ( 'NONE',  ( -48.44597344681495343, 0.000000000000000000, -117.4317124430720156 ) ) ;
#7364=CARTESIAN_POINT ( 'NONE',  ( 153.3040265531850537, -1.750000000000010214, -39.18171244307202983 ) ) ;
#7365=ADVANCED_FACE ( 'NONE', ( #12606 ), #20312, .T. ) ;
#7371=CARTESIAN_POINT ( 'NONE',  ( 210.0000000000000568, 0.000000000000000000, 80.81828755692798438 ) ) ;
#7377=EDGE_CURVE ( 'NONE', #49500, #8521, #47392, .T. ) ;
#7379=ORIENTED_EDGE ( 'NONE', *, *, #28643, .F. ) ;
#7380=VECTOR ( 'NONE', #9335, 1000.000000000000000 ) ;
#7382=( BOUNDED_CURVE ( )  B_SPLINE_CURVE ( 3, ( #11813, #20510, #8471, #28223 ),
 .UNSPECIFIED., .F., .F. ) 
 B_SPLINE_CURVE_WITH_KNOTS ( ( 4, 4 ),
 ( 1.570796326794896558, 3.141592653589793116 ),
 .UNSPECIFIED. ) 
 CURVE ( )  GEOMETRIC_REPRESENTATION_ITEM ( )  RATIONAL_B_SPLINE_CURVE ( ( 1.000000000000000000, 0.8047378541243649375, 0.8047378541243649375, 1.000000000000000000 ) ) 
 REPRESENTATION_ITEM ( '' )  );
#7383=ORIENTED_EDGE ( 'NONE', *, *, #7105, .F. ) ;
#7386=CARTESIAN_POINT ( 'NONE',  ( 75.05402655318509630, -1.025126265847089657, -80.93171244307201562 ) ) ;
#7390=VERTEX_POINT ( 'NONE', #28526 ) ;
#7393=ORIENTED_EDGE ( 'NONE', *, *, #81, .T. ) ;
#7394=ADVANCED_FACE ( 'NONE', ( #47224 ), #2012, .T. ) ;
#7398=DIRECTION ( 'NONE',  ( -1.000000000000000000, -0.000000000000000000, -0.000000000000000000 ) ) ;
#7399=CYLINDRICAL_SURFACE ( 'NONE', #40479, 1.750000000000015543 ) ;
#7404=CARTESIAN_POINT ( 'NONE',  ( -166.6959734468149463, 0.000000000000000000, -165.0000000000000000 ) ) ;
#7406=CARTESIAN_POINT ( 'NONE',  ( -208.4459734468148611, -1.025126265847089657, 79.06828755692797017 ) ) ;
#7408=ORIENTED_EDGE ( 'NONE', *, *, #20678, .F. ) ;
#7413=ORIENTED_EDGE ( 'NONE', *, *, #14574, .T. ) ;
#7415=CARTESIAN_POINT ( 'NONE',  ( 210.0000000000000568, 0.000000000000000000, 160.8182875569279702 ) ) ;
#7416=EDGE_CURVE ( 'NONE', #44023, #41284, #24823, .T. ) ;
#7420=EDGE_CURVE ( 'NONE', #11639, #29172, #17616, .T. ) ;
#7426=FACE_OUTER_BOUND ( 'NONE', #17430, .T. ) ;
#7427=CARTESIAN_POINT ( 'NONE',  ( 75.05402655318509630, 2.143131898507880377E-16, 122.5682875569279844 ) ) ;
#7433=VECTOR ( 'NONE', #47147, 1000.000000000000000 ) ;
#7435=LINE ( 'NONE', #11781, #10147 ) ;
#7444=CYLINDRICAL_SURFACE ( 'NONE', #35689, 1.750000000000015543 ) ;
#7446=( BOUNDED_CURVE ( )  B_SPLINE_CURVE ( 3, ( #17950, #23072, #26681, #46128 ),
 .UNSPECIFIED., .F., .F. ) 
 B_SPLINE_CURVE_WITH_KNOTS ( ( 4, 4 ),
 ( 3.141592653589793116, 4.712388980384689674 ),
 .UNSPECIFIED. ) 
 CURVE ( )  GEOMETRIC_REPRESENTATION_ITEM ( )  RATIONAL_B_SPLINE_CURVE ( ( 1.000000000000000000, 0.8047378541243649375, 0.8047378541243649375, 1.000000000000000000 ) ) 
 REPRESENTATION_ITEM ( '' )  );
#7448=CARTESIAN_POINT ( 'NONE',  ( 35.05402655318504657, 2.143131898507880377E-16, 82.56828755692798438 ) ) ;
#7449=EDGE_LOOP ( 'NONE', ( #34439, #14565, #48935, #2902, #28578, #41636 ) ) ;
#7454=EDGE_CURVE ( 'NONE', #40358, #34395, #42190, .T. ) ;
#7455=( BOUNDED_CURVE ( )  B_SPLINE_CURVE ( 3, ( #10515, #45888, #8951, #12291 ),
 .UNSPECIFIED., .F., .F. ) 
 B_SPLINE_CURVE_WITH_KNOTS ( ( 4, 4 ),
 ( 0.000000000000000000, 1.570796326794896558 ),
 .UNSPECIFIED. ) 
 CURVE ( )  GEOMETRIC_REPRESENTATION_ITEM ( )  RATIONAL_B_SPLINE_CURVE ( ( 1.000000000000000000, 0.8047378541243649375, 0.8047378541243649375, 1.000000000000000000 ) ) 
 REPRESENTATION_ITEM ( '' )  );
#7456=VERTEX_POINT ( 'NONE', #2511 ) ;
#7458=AXIS2_PLACEMENT_3D ( 'NONE', #2391, #34215, #18035 ) ;
#7460=CARTESIAN_POINT ( 'NONE',  ( -84.94597344681494633, 2.143131898507880377E-16, -37.43171244307205825 ) ) ;
#7465=FACE_OUTER_BOUND ( 'NONE', #29065, .T. ) ;
#7469=DIRECTION ( 'NONE',  ( 0.000000000000000000, 0.000000000000000000, 1.000000000000000000 ) ) ;
#7472=ORIENTED_EDGE ( 'NONE', *, *, #49872, .F. ) ;
#7476=ORIENTED_EDGE ( 'NONE', *, *, #45645, .F. ) ;
#7480=ORIENTED_EDGE ( 'NONE', *, *, #22248, .F. ) ;
#7484=CARTESIAN_POINT ( 'NONE',  ( 73.30402655318508209, 1.750000000000010214, 40.81828755692798438 ) ) ;
#7486=CARTESIAN_POINT ( 'NONE',  ( -88.44597344681497475, 0.000000000000000000, 39.06828755692795596 ) ) ;
#7487=ORIENTED_EDGE ( 'NONE', *, *, #42143, .F. ) ;
#7488=DIRECTION ( 'NONE',  ( -0.000000000000000000, -0.000000000000000000, -1.000000000000000000 ) ) ;
#7489=EDGE_CURVE ( 'NONE', #13763, #33331, #11602, .T. ) ;
#7495=CARTESIAN_POINT ( 'NONE',  ( -206.6959734468149463, 1.750000000000010658, -79.18171244307201562 ) ) ;
#7498=DIRECTION ( 'NONE',  ( -1.000000000000000000, 0.000000000000000000, 0.000000000000000000 ) ) ;
#7500=CARTESIAN_POINT ( 'NONE',  ( 153.3040265531850537, 1.750000000000010214, 40.81828755692798438 ) ) ;
#7510=DIRECTION ( 'NONE',  ( -1.000000000000000000, -0.000000000000000000, -0.000000000000000000 ) ) ;
#7513=EDGE_CURVE ( 'NONE', #26878, #24770, #26461, .T. ) ;
#7516=VERTEX_POINT ( 'NONE', #30734 ) ;
#7517=CARTESIAN_POINT ( 'NONE',  ( -7.721099712662037540, 1.750000000000023315, -0.2068387089191201234 ) ) ;
#7521=AXIS2_PLACEMENT_3D ( 'NONE', #25832, #18119, #49130 ) ;
#7522=VECTOR ( 'NONE', #23770, 1000.000000000000000 ) ;
#7530=CARTESIAN_POINT ( 'NONE',  ( 191.5540265531851105, 2.143131898507880377E-16, -160.9317124430720298 ) ) ;
#7531=CYLINDRICAL_SURFACE ( 'NONE', #14443, 1.750000000000010214 ) ;
#7533=ORIENTED_EDGE ( 'NONE', *, *, #7701, .F. ) ;
#7536=DIRECTION ( 'NONE',  ( -1.000000000000000000, -0.000000000000000000, -0.000000000000000000 ) ) ;
#7542=ORIENTED_EDGE ( 'NONE', *, *, #44762, .F. ) ;
#7548=CARTESIAN_POINT ( 'NONE',  ( -87.72109971266203843, -1.750000000000009548, 39.79316129108089228 ) ) ;
#7551=ORIENTED_EDGE ( 'NONE', *, *, #47222, .F. ) ;
#7555=DIRECTION ( 'NONE',  ( -1.000000000000000000, -0.000000000000000000, -0.000000000000000000 ) ) ;
#7568=ORIENTED_EDGE ( 'NONE', *, *, #242, .F. ) ;
#7570=CARTESIAN_POINT ( 'NONE',  ( 151.5540265531850537, 0.000000000000000000, 79.06828755692797017 ) ) ;
#7572=VERTEX_POINT ( 'NONE', #23010 ) ;
#7574=CARTESIAN_POINT ( 'NONE',  ( -168.4459734468149747, 1.025126265847089435, 39.06828755692797728 ) ) ;
#7576=ORIENTED_EDGE ( 'NONE', *, *, #23378, .F. ) ;
#7577=ORIENTED_EDGE ( 'NONE', *, *, #4272, .T. ) ;
#7578=DIRECTION ( 'NONE',  ( -0.000000000000000000, -0.000000000000000000, -1.000000000000000000 ) ) ;
#7580=( BOUNDED_CURVE ( )  B_SPLINE_CURVE ( 3, ( #48295, #20380, #12429, #27845 ),
 .UNSPECIFIED., .F., .F. ) 
 B_SPLINE_CURVE_WITH_KNOTS ( ( 4, 4 ),
 ( 3.141592653589793116, 4.712388980384689674 ),
 .UNSPECIFIED. ) 
 CURVE ( )  GEOMETRIC_REPRESENTATION_ITEM ( )  RATIONAL_B_SPLINE_CURVE ( ( 1.000000000000000000, 0.8047378541243649375, 0.8047378541243649375, 1.000000000000000000 ) ) 
 REPRESENTATION_ITEM ( '' )  );
#7583=DIRECTION ( 'NONE',  ( -1.000000000000000000, -0.000000000000000000, -0.000000000000000000 ) ) ;
#7584=CARTESIAN_POINT ( 'NONE',  ( 71.55402655318505367, 0.000000000000000000, 165.0000000000000000 ) ) ;
#7585=VECTOR ( 'NONE', #17378, 1000.000000000000000 ) ;
#7586=ORIENTED_EDGE ( 'NONE', *, *, #40930, .T. ) ;
#7589=EDGE_LOOP ( 'NONE', ( #35675, #43028, #12282, #4807, #19537, #17621 ) ) ;
#7591=CARTESIAN_POINT ( 'NONE',  ( 193.3040265531851105, -1.750000000000010214, -39.18171244307202983 ) ) ;
#7599=ORIENTED_EDGE ( 'NONE', *, *, #16419, .T. ) ;
#7600=DIRECTION ( 'NONE',  ( -1.000000000000000000, 0.000000000000000000, 0.000000000000000000 ) ) ;
#7603=( BOUNDED_CURVE ( )  B_SPLINE_CURVE ( 3, ( #13939, #25253, #40906, #21394 ),
 .UNSPECIFIED., .F., .F. ) 
 B_SPLINE_CURVE_WITH_KNOTS ( ( 4, 4 ),
 ( 1.570796326794896558, 3.141592653589793116 ),
 .UNSPECIFIED. ) 
 CURVE ( )  GEOMETRIC_REPRESENTATION_ITEM ( )  RATIONAL_B_SPLINE_CURVE ( ( 1.000000000000000000, 0.8047378541243649375, 0.8047378541243649375, 1.000000000000000000 ) ) 
 REPRESENTATION_ITEM ( '' )  );
#7604=CARTESIAN_POINT ( 'NONE',  ( 111.5540265531850679, 0.000000000000000000, -0.9317124430719969652 ) ) ;
#7606=EDGE_LOOP ( 'NONE', ( #21266, #28265, #39229, #26984, #16343, #32088 ) ) ;
#7607=ORIENTED_EDGE ( 'NONE', *, *, #2310, .F. ) ;
#7609=CARTESIAN_POINT ( 'NONE',  ( -125.6708471809678542, 1.749999999999996891, 79.79316129108087807 ) ) ;
#7615=EDGE_LOOP ( 'NONE', ( #45956, #38588, #4468, #14310, #14728, #16993 ) ) ;
#7617=LINE ( 'NONE', #30977, #31635 ) ;
#7620=DIRECTION ( 'NONE',  ( 0.000000000000000000, 0.000000000000000000, 1.000000000000000000 ) ) ;
#7621=EDGE_CURVE ( 'NONE', #20141, #17107, #42483, .T. ) ;
#7627=EDGE_CURVE ( 'NONE', #20559, #38882, #36990, .T. ) ;
#7633=CARTESIAN_POINT ( 'NONE',  ( -5.670847180967843570, -1.750000000000022427, 159.7931612910808781 ) ) ;
#7634=AXIS2_PLACEMENT_3D ( 'NONE', #36741, #48208, #6919 ) ;
#7635=CARTESIAN_POINT ( 'NONE',  ( 33.30402655318503946, 0.000000000000000000, -165.0000000000000000 ) ) ;
#7638=CARTESIAN_POINT ( 'NONE',  ( 72.27890028733797578, 1.750000000000009548, 39.79316129108089228 ) ) ;
#7640=FACE_OUTER_BOUND ( 'NONE', #24597, .T. ) ;
#7641=ORIENTED_EDGE ( 'NONE', *, *, #14848, .T. ) ;
#7643=ORIENTED_EDGE ( 'NONE', *, *, #29939, .T. ) ;
#7651=ORIENTED_EDGE ( 'NONE', *, *, #33145, .T. ) ;
#7653=CARTESIAN_POINT ( 'NONE',  ( 115.0540265531850395, -1.025126265847081886, -120.9317124430720440 ) ) ;
#7661=VERTEX_POINT ( 'NONE', #3779 ) ;
#7674=AXIS2_PLACEMENT_3D ( 'NONE', #1636, #18021, #33694 ) ;
#7675=LINE ( 'NONE', #26909, #44648 ) ;
#7680=ORIENTED_EDGE ( 'NONE', *, *, #1448, .F. ) ;
#7682=CARTESIAN_POINT ( 'NONE',  ( -125.6708471809678542, 1.749999999999996669, 41.84341382277508359 ) ) ;
#7684=( BOUNDED_CURVE ( )  B_SPLINE_CURVE ( 3, ( #32319, #12805, #16919, #32576 ),
 .UNSPECIFIED., .F., .F. ) 
 B_SPLINE_CURVE_WITH_KNOTS ( ( 4, 4 ),
 ( 4.712388980384689674, 6.283185307179586232 ),
 .UNSPECIFIED. ) 
 CURVE ( )  GEOMETRIC_REPRESENTATION_ITEM ( )  RATIONAL_B_SPLINE_CURVE ( ( 1.000000000000000000, 0.8047378541243649375, 0.8047378541243649375, 1.000000000000000000 ) ) 
 REPRESENTATION_ITEM ( '' )  );
#7686=DIRECTION ( 'NONE',  ( -1.000000000000000000, 0.000000000000000000, 0.000000000000000000 ) ) ;
#7688=DIRECTION ( 'NONE',  ( -1.000000000000000000, 0.000000000000000000, 0.000000000000000000 ) ) ;
#7691=EDGE_CURVE ( 'NONE', #28486, #33010, #18205, .T. ) ;
#7700=ORIENTED_EDGE ( 'NONE', *, *, #32054, .T. ) ;
#7701=EDGE_CURVE ( 'NONE', #4897, #43762, #5784, .T. ) ;
#7704=CARTESIAN_POINT ( 'NONE',  ( 195.0540265531851105, 1.025126265847089879, 122.5682875569280128 ) ) ;
#7714=ORIENTED_EDGE ( 'NONE', *, *, #13596, .T. ) ;
#7724=ADVANCED_FACE ( 'NONE', ( #5542 ), #32518, .T. ) ;
#7725=CARTESIAN_POINT ( 'NONE',  ( 210.0000000000000568, 0.000000000000000000, -159.1817124430720298 ) ) ;
#7728=CARTESIAN_POINT ( 'NONE',  ( -206.6959734468149463, 0.000000000000000000, -165.0000000000000000 ) ) ;
#7729=DIRECTION ( 'NONE',  ( -1.000000000000000000, 0.000000000000000000, 0.000000000000000000 ) ) ;
#7736=AXIS2_PLACEMENT_3D ( 'NONE', #34861, #31008, #11494 ) ;
#7739=VECTOR ( 'NONE', #22143, 1000.000000000000000 ) ;
#7744=CARTESIAN_POINT ( 'NONE',  ( 32.27890028733795447, 1.750000000000010436, -120.2068387089191219 ) ) ;
#7745=( BOUNDED_CURVE ( )  B_SPLINE_CURVE ( 3, ( #42640, #11098, #3649, #23142 ),
 .UNSPECIFIED., .F., .F. ) 
 B_SPLINE_CURVE_WITH_KNOTS ( ( 4, 4 ),
 ( 0.000000000000000000, 1.570796326794896780 ),
 .UNSPECIFIED. ) 
 CURVE ( )  GEOMETRIC_REPRESENTATION_ITEM ( )  RATIONAL_B_SPLINE_CURVE ( ( 1.000000000000000000, 0.8047378541243649375, 0.8047378541243649375, 1.000000000000000000 ) ) 
 REPRESENTATION_ITEM ( '' )  );
#7752=CARTESIAN_POINT ( 'NONE',  ( -47.72109971266203132, 1.750000000000009548, -78.15658617722490931 ) ) ;
#7753=( BOUNDED_CURVE ( )  B_SPLINE_CURVE ( 3, ( #19538, #35223, #577, #16216 ),
 .UNSPECIFIED., .F., .F. ) 
 B_SPLINE_CURVE_WITH_KNOTS ( ( 4, 4 ),
 ( 1.570796326794896558, 3.141592653589793116 ),
 .UNSPECIFIED. ) 
 CURVE ( )  GEOMETRIC_REPRESENTATION_ITEM ( )  RATIONAL_B_SPLINE_CURVE ( ( 1.000000000000000000, 0.8047378541243649375, 0.8047378541243649375, 1.000000000000000000 ) ) 
 REPRESENTATION_ITEM ( '' )  );
#7756=CARTESIAN_POINT ( 'NONE',  ( 113.3040265531850537, 1.749999999999997113, -39.18171244307202983 ) ) ;
#7757=( LENGTH_UNIT ( ) NAMED_UNIT ( * ) SI_UNIT ( .MILLI., .METRE. ) );
#7762=ADVANCED_FACE ( 'NONE', ( #36366 ), #29396, .T. ) ;
#7763=VERTEX_POINT ( 'NONE', #13234 ) ;
#7764=CARTESIAN_POINT ( 'NONE',  ( 73.30402655318508209, -1.750000000000009992, 160.8182875569279702 ) ) ;
#7767=ORIENTED_EDGE ( 'NONE', *, *, #47179, .T. ) ;
#7774=ADVANCED_FACE ( 'NONE', ( #45017 ), #1704, .T. ) ;
#7776=CARTESIAN_POINT ( 'NONE',  ( -208.4459734468149463, 0.000000000000000000, 39.06828755692798438 ) ) ;
#7778=VERTEX_POINT ( 'NONE', #9897 ) ;
#7782=CYLINDRICAL_SURFACE ( 'NONE', #2471, 1.750000000000008438 ) ;
#7784=ADVANCED_FACE ( 'NONE', ( #17597 ), #17344, .T. ) ;
#7785=ORIENTED_EDGE ( 'NONE', *, *, #16846, .T. ) ;
#7789=EDGE_LOOP ( 'NONE', ( #28828, #46978, #40860, #45894, #4480, #44245 ) ) ;
#7795=EDGE_LOOP ( 'NONE', ( #1160, #48452, #44718, #2006, #6896 ) ) ;
#7802=ORIENTED_EDGE ( 'NONE', *, *, #1385, .T. ) ;
#7805=CARTESIAN_POINT ( 'NONE',  ( 193.3040265531851105, -1.750000000000009992, 160.8182875569279702 ) ) ;
#7807=VERTEX_POINT ( 'NONE', #5030 ) ;
#7810=EDGE_CURVE ( 'NONE', #48234, #4486, #7137, .T. ) ;
#7812=VERTEX_POINT ( 'NONE', #21438 ) ;
#7813=DIRECTION ( 'NONE',  ( 0.000000000000000000, 0.000000000000000000, 1.000000000000000000 ) ) ;
#7814=FACE_OUTER_BOUND ( 'NONE', #22893, .T. ) ;
#7821=DIRECTION ( 'NONE',  ( -0.000000000000000000, -0.000000000000000000, -1.000000000000000000 ) ) ;
#7823=DIRECTION ( 'NONE',  ( -1.000000000000000000, -0.000000000000000000, -0.000000000000000000 ) ) ;
#7825=ADVANCED_FACE ( 'NONE', ( #20948 ), #25057, .T. ) ;
#7827=ADVANCED_FACE ( 'NONE', ( #20427 ), #13741, .T. ) ;
#7832=EDGE_CURVE ( 'NONE', #25636, #33167, #6500, .T. ) ;
#7836=CARTESIAN_POINT ( 'NONE',  ( 115.0540265531850395, -1.025126265847081442, -160.9317124430720014 ) ) ;
#7837=VECTOR ( 'NONE', #38188, 1000.000000000000000 ) ;
#7839=EDGE_CURVE ( 'NONE', #39727, #19789, #22454, .T. ) ;
#7844=CARTESIAN_POINT ( 'NONE',  ( 193.3040265531851105, 0.000000000000000000, 165.0000000000000000 ) ) ;
#7848=ORIENTED_EDGE ( 'NONE', *, *, #15588, .T. ) ;
#7849=CARTESIAN_POINT ( 'NONE',  ( -45.67084718096785423, 1.750000000000009548, -38.15658617722494483 ) ) ;
#7851=DIRECTION ( 'NONE',  ( -1.000000000000000000, -0.000000000000000000, -0.000000000000000000 ) ) ;
#7856=EDGE_LOOP ( 'NONE', ( #44937, #7082, #31814, #26393, #39662, #17897 ) ) ;
#7857=ORIENTED_EDGE ( 'NONE', *, *, #39672, .T. ) ;
#7867=LINE ( 'NONE', #26842, #12318 ) ;
#7869=VERTEX_POINT ( 'NONE', #49604 ) ;
#7873=ORIENTED_EDGE ( 'NONE', *, *, #13659, .F. ) ;
#7874=VECTOR ( 'NONE', #46285, 1000.000000000000000 ) ;
#7875=DIRECTION ( 'NONE',  ( -1.000000000000000000, -0.000000000000000000, -0.000000000000000000 ) ) ;
#7893=( BOUNDED_CURVE ( )  B_SPLINE_CURVE ( 3, ( #31641, #12125, #27770, #35993 ),
 .UNSPECIFIED., .F., .F. ) 
 B_SPLINE_CURVE_WITH_KNOTS ( ( 4, 4 ),
 ( 3.141592653589793116, 4.712388980384689674 ),
 .UNSPECIFIED. ) 
 CURVE ( )  GEOMETRIC_REPRESENTATION_ITEM ( )  RATIONAL_B_SPLINE_CURVE ( ( 1.000000000000000000, 0.8047378541243649375, 0.8047378541243649375, 1.000000000000000000 ) ) 
 REPRESENTATION_ITEM ( '' )  );
#7898=CARTESIAN_POINT ( 'NONE',  ( 33.30402655318503946, -1.750000000000010214, 40.81828755692798438 ) ) ;
#7902=( BOUNDED_CURVE ( )  B_SPLINE_CURVE ( 3, ( #9074, #13167, #20615, #12165 ),
 .UNSPECIFIED., .F., .F. ) 
 B_SPLINE_CURVE_WITH_KNOTS ( ( 4, 4 ),
 ( 4.712388980384689674, 6.283185307179586232 ),
 .UNSPECIFIED. ) 
 CURVE ( )  GEOMETRIC_REPRESENTATION_ITEM ( )  RATIONAL_B_SPLINE_CURVE ( ( 1.000000000000000000, 0.8047378541243649375, 0.8047378541243649375, 1.000000000000000000 ) ) 
 REPRESENTATION_ITEM ( '' )  );
#7908=CARTESIAN_POINT ( 'NONE',  ( 210.0000000000000568, 0.000000000000000000, 160.8182875569279702 ) ) ;
#7911=ORIENTED_EDGE ( 'NONE', *, *, #33741, .T. ) ;
#7915=( BOUNDED_CURVE ( )  B_SPLINE_CURVE ( 3, ( #26402, #41554, #14601, #3300 ),
 .UNSPECIFIED., .F., .F. ) 
 B_SPLINE_CURVE_WITH_KNOTS ( ( 4, 4 ),
 ( 4.712388980384689674, 6.283185307179586232 ),
 .UNSPECIFIED. ) 
 CURVE ( )  GEOMETRIC_REPRESENTATION_ITEM ( )  RATIONAL_B_SPLINE_CURVE ( ( 1.000000000000000000, 0.8047378541243649375, 0.8047378541243649375, 1.000000000000000000 ) ) 
 REPRESENTATION_ITEM ( '' )  );
#7918=CARTESIAN_POINT ( 'NONE',  ( -206.6959734468149463, 1.750000000000010658, 120.8182875569279702 ) ) ;
#7919=CARTESIAN_POINT ( 'NONE',  ( 113.3040265531850537, -1.749999999999997335, -119.1817124430720440 ) ) ;
#7929=CARTESIAN_POINT ( 'NONE',  ( 115.0540265531850395, 2.143131898507842906E-16, 165.0000000000000000 ) ) ;
#7933=CARTESIAN_POINT ( 'NONE',  ( -164.9459734468149463, 2.143131898507880377E-16, -77.43171244307204404 ) ) ;
#7942=CARTESIAN_POINT ( 'NONE',  ( -204.9459734468148895, -1.025126265847089435, -117.4317124430720156 ) ) ;
#7944=VECTOR ( 'NONE', #7089, 1000.000000000000000 ) ;
#7946=DIRECTION ( 'NONE',  ( 1.000000000000000000, 0.000000000000000000, 0.000000000000000000 ) ) ;
#7947=ORIENTED_EDGE ( 'NONE', *, *, #7832, .T. ) ;
#7949=CARTESIAN_POINT ( 'NONE',  ( 115.0540265531850395, -1.025126265847081219, 159.0682875569279418 ) ) ;
#7950=CARTESIAN_POINT ( 'NONE',  ( 71.55402655318505367, 0.000000000000000000, 159.0682875569279702 ) ) ;
#7953=DIRECTION ( 'NONE',  ( -0.000000000000000000, -0.000000000000000000, -1.000000000000000000 ) ) ;
#7963=ORIENTED_EDGE ( 'NONE', *, *, #30073, .T. ) ;
#7964=ADVANCED_FACE ( 'NONE', ( #22705 ), #25808, .T. ) ;
#7966=EDGE_CURVE ( 'NONE', #34589, #41828, #25124, .T. ) ;
#7969=CARTESIAN_POINT ( 'NONE',  ( -206.6959734468149463, 1.750000000000010214, 40.81828755692798438 ) ) ;
#7972=CARTESIAN_POINT ( 'NONE',  ( 115.0540265531850395, 2.143131898507847836E-16, -77.43171244307204404 ) ) ;
#7977=DIRECTION ( 'NONE',  ( -1.000000000000000000, -0.000000000000000000, -0.000000000000000000 ) ) ;
#7978=ORIENTED_EDGE ( 'NONE', *, *, #534, .F. ) ;
#7980=CARTESIAN_POINT ( 'NONE',  ( 210.0000000000000568, 0.000000000000000000, 162.5682875569279702 ) ) ;
#7982=ORIENTED_EDGE ( 'NONE', *, *, #45528, .F. ) ;
#7987=EDGE_CURVE ( 'NONE', #37507, #23383, #12372, .T. ) ;
#7990=CARTESIAN_POINT ( 'NONE',  ( 111.5540265531850679, 0.000000000000000000, -117.4317124430720725 ) ) ;
#7993=EDGE_CURVE ( 'NONE', #40596, #27788, #49341, .T. ) ;
#7994=ORIENTED_EDGE ( 'NONE', *, *, #48677, .T. ) ;
#7995=( BOUNDED_CURVE ( )  B_SPLINE_CURVE ( 3, ( #47585, #27883, #43512, #4522 ),
 .UNSPECIFIED., .F., .F. ) 
 B_SPLINE_CURVE_WITH_KNOTS ( ( 4, 4 ),
 ( 4.712388980384689674, 6.283185307179586232 ),
 .UNSPECIFIED. ) 
 CURVE ( )  GEOMETRIC_REPRESENTATION_ITEM ( )  RATIONAL_B_SPLINE_CURVE ( ( 1.000000000000000000, 0.8047378541243649375, 0.8047378541243649375, 1.000000000000000000 ) ) 
 REPRESENTATION_ITEM ( '' )  );
#7999=EDGE_CURVE ( 'NONE', #48485, #48152, #37290, .T. ) ;
#8000=DIRECTION ( 'NONE',  ( -0.000000000000000000, -0.000000000000000000, -1.000000000000000000 ) ) ;
#8006=CARTESIAN_POINT ( 'NONE',  ( 191.5540265531851105, 0.000000000000000000, 39.06828755692798438 ) ) ;
#8007=CARTESIAN_POINT ( 'NONE',  ( -204.9459734468148895, -1.025126265847088991, -157.4317124430720582 ) ) ;
#8010=CARTESIAN_POINT ( 'NONE',  ( -48.44597344681495343, 0.000000000000000000, -77.43171244307198720 ) ) ;
#8012=FACE_OUTER_BOUND ( 'NONE', #29019, .T. ) ;
#8017=CARTESIAN_POINT ( 'NONE',  ( 210.0000000000000568, 2.143131898507880377E-16, -160.9317124430720298 ) ) ;
#8018=CIRCLE ( 'NONE', #48092, 1.750000000000015543 ) ;
#8020=EDGE_CURVE ( 'NONE', #39370, #47399, #16281, .T. ) ;
#8021=DIRECTION ( 'NONE',  ( -1.000000000000000000, 0.000000000000000000, 0.000000000000000000 ) ) ;
#8022=ORIENTED_EDGE ( 'NONE', *, *, #36864, .F. ) ;
#8034=VECTOR ( 'NONE', #50342, 1000.000000000000000 ) ;
#8035=ORIENTED_EDGE ( 'NONE', *, *, #13046, .T. ) ;
#8042=PLANE ( 'NONE',  #14972 ) ;
#8044=EDGE_LOOP ( 'NONE', ( #49176, #49626, #22471, #10972, #32273, #48504 ) ) ;
#8045=CARTESIAN_POINT ( 'NONE',  ( -48.44597344681495343, 0.000000000000000000, 165.0000000000000000 ) ) ;
#8046=ORIENTED_EDGE ( 'NONE', *, *, #23529, .F. ) ;
#8049=( BOUNDED_CURVE ( )  B_SPLINE_CURVE ( 3, ( #46417, #33904, #6947, #18985 ),
 .UNSPECIFIED., .F., .F. ) 
 B_SPLINE_CURVE_WITH_KNOTS ( ( 4, 4 ),
 ( 0.000000000000000000, 1.570796326794896558 ),
 .UNSPECIFIED. ) 
 CURVE ( )  GEOMETRIC_REPRESENTATION_ITEM ( )  RATIONAL_B_SPLINE_CURVE ( ( 1.000000000000000000, 0.8047378541243649375, 0.8047378541243649375, 1.000000000000000000 ) ) 
 REPRESENTATION_ITEM ( '' )  );
#8053=ORIENTED_EDGE ( 'NONE', *, *, #1852, .F. ) ;
#8056=ORIENTED_EDGE ( 'NONE', *, *, #40839, .T. ) ;
#8057=LINE ( 'NONE', #16001, #38629 ) ;
#8058=( BOUNDED_CURVE ( )  B_SPLINE_CURVE ( 3, ( #2815, #10026, #33890, #14885 ),
 .UNSPECIFIED., .F., .F. ) 
 B_SPLINE_CURVE_WITH_KNOTS ( ( 4, 4 ),
 ( 1.570796326794896558, 3.141592653589793116 ),
 .UNSPECIFIED. ) 
 CURVE ( )  GEOMETRIC_REPRESENTATION_ITEM ( )  RATIONAL_B_SPLINE_CURVE ( ( 1.000000000000000000, 0.8047378541243649375, 0.8047378541243649375, 1.000000000000000000 ) ) 
 REPRESENTATION_ITEM ( '' )  );
#8062=CARTESIAN_POINT ( 'NONE',  ( 115.0540265531850679, 0.000000000000000000, 162.5682875569279702 ) ) ;
#8066=ORIENTED_EDGE ( 'NONE', *, *, #1572, .F. ) ;
#8070=LINE ( 'NONE', #23708, #17639 ) ;
#8075=DIRECTION ( 'NONE',  ( -0.000000000000000000, -0.000000000000000000, -1.000000000000000000 ) ) ;
#8078=CARTESIAN_POINT ( 'NONE',  ( 114.3291528190321173, -1.749999999999996669, 41.84341382277508359 ) ) ;
#8083=FACE_OUTER_BOUND ( 'NONE', #49608, .T. ) ;
#8084=EDGE_LOOP ( 'NONE', ( #47393, #9425, #35742, #33035, #8592 ) ) ;
#8085=AXIS2_PLACEMENT_3D ( 'NONE', #29140, #26299, #33502 ) ;
#8091=ORIENTED_EDGE ( 'NONE', *, *, #26570, .F. ) ;
#8096=CARTESIAN_POINT ( 'NONE',  ( 210.0000000000000568, 0.000000000000000000, 122.5682875569279844 ) ) ;
#8097=FACE_OUTER_BOUND ( 'NONE', #37955, .T. ) ;
#8103=CARTESIAN_POINT ( 'NONE',  ( -6.695973446814940111, -1.750000000000023759, 40.81828755692798438 ) ) ;
#8105=EDGE_CURVE ( 'NONE', #47659, #26079, #19557, .T. ) ;
#8108=CARTESIAN_POINT ( 'NONE',  ( 31.55402655318503236, 0.000000000000000000, 165.0000000000000000 ) ) ;
#8111=VERTEX_POINT ( 'NONE', #1897 ) ;
#8112=DIRECTION ( 'NONE',  ( -0.000000000000000000, -0.000000000000000000, -1.000000000000000000 ) ) ;
#8113=CARTESIAN_POINT ( 'NONE',  ( -6.695973446814940111, 0.000000000000000000, 165.0000000000000000 ) ) ;
#8119=CARTESIAN_POINT ( 'NONE',  ( 193.3040265531851105, 1.750000000000010658, 120.8182875569279702 ) ) ;
#8120=CARTESIAN_POINT ( 'NONE',  ( -165.6708471809677974, 1.750000000000010214, -80.20683870891910772 ) ) ;
#8122=ORIENTED_EDGE ( 'NONE', *, *, #22908, .F. ) ;
#8126=DIRECTION ( 'NONE',  ( 1.000000000000000000, 0.000000000000000000, 0.000000000000000000 ) ) ;
#8127=VECTOR ( 'NONE', #27437, 1000.000000000000000 ) ;
#8132=CARTESIAN_POINT ( 'NONE',  ( 191.5540265531851105, 2.143131898507880377E-16, -160.9317124430720298 ) ) ;
#8133=CARTESIAN_POINT ( 'NONE',  ( -47.72109971266203132, 1.750000000000010436, -80.20683870891910772 ) ) ;
#8135=FACE_OUTER_BOUND ( 'NONE', #29371, .T. ) ;
#8139=LINE ( 'NONE', #44261, #14689 ) ;
#8140=CARTESIAN_POINT ( 'NONE',  ( 113.3040265531850537, 1.749999999999997113, 40.81828755692798438 ) ) ;
#8144=ORIENTED_EDGE ( 'NONE', *, *, #852, .F. ) ;
#8145=CARTESIAN_POINT ( 'NONE',  ( -84.94597344681493212, -1.025126265847089435, -77.43171244307200141 ) ) ;
#8146=CARTESIAN_POINT ( 'NONE',  ( -208.4459734468149463, 0.000000000000000000, 162.5682875569279702 ) ) ;
#8147=CARTESIAN_POINT ( 'NONE',  ( -84.94597344681493212, -1.025126265847089435, 82.56828755692798438 ) ) ;
#8153=ADVANCED_FACE ( 'NONE', ( #13436 ), #36571, .F. ) ;
#8155=AXIS2_PLACEMENT_3D ( 'NONE', #8265, #35740, #27761 ) ;
#8157=ORIENTED_EDGE ( 'NONE', *, *, #46351, .F. ) ;
#8158=DIRECTION ( 'NONE',  ( -0.000000000000000000, -0.000000000000000000, -1.000000000000000000 ) ) ;
#8161=CIRCLE ( 'NONE', #31085, 1.749999999999987566 ) ;
#8162=LINE ( 'NONE', #46602, #40702 ) ;
#8176=VERTEX_POINT ( 'NONE', #1149 ) ;
#8181=CARTESIAN_POINT ( 'NONE',  ( 210.0000000000000568, 0.000000000000000000, -79.18171244307201562 ) ) ;
#8182=CARTESIAN_POINT ( 'NONE',  ( 153.3040265531850537, -1.750000000000010658, 120.8182875569279702 ) ) ;
#8183=CARTESIAN_POINT ( 'NONE',  ( -208.4459734468149463, 0.000000000000000000, 39.06828755692798438 ) ) ;
#8184=CARTESIAN_POINT ( 'NONE',  ( -86.69597344681494633, -1.750000000000009992, 160.8182875569279702 ) ) ;
#8185=EDGE_CURVE ( 'NONE', #10383, #26504, #17036, .T. ) ;
#8191=DIRECTION ( 'NONE',  ( -1.000000000000000000, -0.000000000000000000, -0.000000000000000000 ) ) ;
#8192=( BOUNDED_CURVE ( )  B_SPLINE_CURVE ( 3, ( #38602, #30904, #42415, #34757 ),
 .UNSPECIFIED., .F., .F. ) 
 B_SPLINE_CURVE_WITH_KNOTS ( ( 4, 4 ),
 ( 4.712388980384689674, 6.283185307179586232 ),
 .UNSPECIFIED. ) 
 CURVE ( )  GEOMETRIC_REPRESENTATION_ITEM ( )  RATIONAL_B_SPLINE_CURVE ( ( 1.000000000000000000, 0.8047378541243649375, 0.8047378541243649375, 1.000000000000000000 ) ) 
 REPRESENTATION_ITEM ( '' )  );
#8193=CARTESIAN_POINT ( 'NONE',  ( 153.3040265531850537, 1.750000000000009992, 0.8182875569279768335 ) ) ;
#8194=AXIS2_PLACEMENT_3D ( 'NONE', #2869, #49030, #33947 ) ;
#8200=( BOUNDED_CURVE ( )  B_SPLINE_CURVE ( 3, ( #40921, #10120, #9868, #6013 ),
 .UNSPECIFIED., .F., .F. ) 
 B_SPLINE_CURVE_WITH_KNOTS ( ( 4, 4 ),
 ( 0.000000000000000000, 1.570796326794896558 ),
 .UNSPECIFIED. ) 
 CURVE ( )  GEOMETRIC_REPRESENTATION_ITEM ( )  RATIONAL_B_SPLINE_CURVE ( ( 1.000000000000000000, 0.8047378541243649375, 0.8047378541243649375, 1.000000000000000000 ) ) 
 REPRESENTATION_ITEM ( '' )  );
#8205=ORIENTED_EDGE ( 'NONE', *, *, #8923, .F. ) ;
#8211=CARTESIAN_POINT ( 'NONE',  ( 115.0540265531850395, 2.143131898507847836E-16, -0.9317124430719969652 ) ) ;
#8212=( BOUNDED_CURVE ( )  B_SPLINE_CURVE ( 3, ( #24221, #16261, #28563, #24474 ),
 .UNSPECIFIED., .F., .F. ) 
 B_SPLINE_CURVE_WITH_KNOTS ( ( 4, 4 ),
 ( 3.141592653589793116, 4.712388980384689674 ),
 .UNSPECIFIED. ) 
 CURVE ( )  GEOMETRIC_REPRESENTATION_ITEM ( )  RATIONAL_B_SPLINE_CURVE ( ( 1.000000000000000000, 0.8047378541243649375, 0.8047378541243649375, 1.000000000000000000 ) ) 
 REPRESENTATION_ITEM ( '' )  );
#8216=ADVANCED_FACE ( 'NONE', ( #5484 ), #34217, .T. ) ;
#8218=CARTESIAN_POINT ( 'NONE',  ( -164.9459734468149463, 2.143131898507880377E-16, 159.0682875569279702 ) ) ;
#8224=AXIS2_PLACEMENT_3D ( 'NONE', #33779, #18351, #41716 ) ;
#8225=LINE ( 'NONE', #39785, #29672 ) ;
#8227=ORIENTED_EDGE ( 'NONE', *, *, #28048, .T. ) ;
#8234=AXIS2_PLACEMENT_3D ( 'NONE', #29245, #25150, #48690 ) ;
#8241=VERTEX_POINT ( 'NONE', #22394 ) ;
#8246=ORIENTED_EDGE ( 'NONE', *, *, #19219, .T. ) ;
#8251=CARTESIAN_POINT ( 'NONE',  ( 154.3291528190321458, -1.750000000000010436, -120.2068387089191219 ) ) ;
#8256=CARTESIAN_POINT ( 'NONE',  ( 31.55402655318503236, 0.000000000000000000, 82.56828755692798438 ) ) ;
#8257=DIRECTION ( 'NONE',  ( -1.000000000000000000, -0.000000000000000000, -0.000000000000000000 ) ) ;
#8263=CARTESIAN_POINT ( 'NONE',  ( -45.67084718096785423, -1.750000000000009548, -0.2068387089191121020 ) ) ;
#8264=ORIENTED_EDGE ( 'NONE', *, *, #27156, .T. ) ;
#8265=CARTESIAN_POINT ( 'NONE',  ( -206.6959734468149463, 0.000000000000000000, 165.0000000000000000 ) ) ;
#8272=CARTESIAN_POINT ( 'NONE',  ( -6.695973446814940111, -1.750000000000023315, -159.1817124430720298 ) ) ;
#8277=CYLINDRICAL_SURFACE ( 'NONE', #26978, 1.750000000000001554 ) ;
#8279=ORIENTED_EDGE ( 'NONE', *, *, #17961, .F. ) ;
#8283=FACE_OUTER_BOUND ( 'NONE', #47795, .T. ) ;
#8286=ORIENTED_EDGE ( 'NONE', *, *, #35125, .T. ) ;
#8287=CARTESIAN_POINT ( 'NONE',  ( 195.0540265531851105, 2.143131898507880377E-16, 165.0000000000000000 ) ) ;
#8289=CARTESIAN_POINT ( 'NONE',  ( -46.69597344681494633, -1.750000000000010658, -79.18171244307201562 ) ) ;
#8290=CARTESIAN_POINT ( 'NONE',  ( 155.0540265531850537, -1.025126265847089435, 82.56828755692798438 ) ) ;
#8292=( BOUNDED_CURVE ( )  B_SPLINE_CURVE ( 3, ( #42673, #27033, #7548, #23185 ),
 .UNSPECIFIED., .F., .F. ) 
 B_SPLINE_CURVE_WITH_KNOTS ( ( 4, 4 ),
 ( 0.000000000000000000, 1.570796326794896558 ),
 .UNSPECIFIED. ) 
 CURVE ( )  GEOMETRIC_REPRESENTATION_ITEM ( )  RATIONAL_B_SPLINE_CURVE ( ( 1.000000000000000000, 0.8047378541243649375, 0.8047378541243649375, 1.000000000000000000 ) ) 
 REPRESENTATION_ITEM ( '' )  );
#8297=ADVANCED_FACE ( 'NONE', ( #45711 ), #29591, .T. ) ;
#8298=CARTESIAN_POINT ( 'NONE',  ( 153.3040265531850537, -1.750000000000010214, -39.18171244307202983 ) ) ;
#8307=CARTESIAN_POINT ( 'NONE',  ( 210.0000000000000568, 0.000000000000000000, 120.8182875569279702 ) ) ;
#8312=CARTESIAN_POINT ( 'NONE',  ( -166.6959734468149463, -1.750000000000010214, -39.18171244307202983 ) ) ;
#8314=VERTEX_POINT ( 'NONE', #5987 ) ;
#8323=ORIENTED_EDGE ( 'NONE', *, *, #34328, .F. ) ;
#8325=CARTESIAN_POINT ( 'NONE',  ( -47.72109971266203132, -1.750000000000009548, 1.843413822775065825 ) ) ;
#8327=DIRECTION ( 'NONE',  ( -1.000000000000000000, 0.000000000000000000, 0.000000000000000000 ) ) ;
#8328=ADVANCED_FACE ( 'NONE', ( #26760 ), #15976, .T. ) ;
#8329=DIRECTION ( 'NONE',  ( 1.000000000000000000, 0.000000000000000000, 0.000000000000000000 ) ) ;
#8330=ORIENTED_EDGE ( 'NONE', *, *, #35477, .T. ) ;
#8334=EDGE_CURVE ( 'NONE', #32609, #43847, #2487, .T. ) ;
#8337=EDGE_CURVE ( 'NONE', #36323, #9039, #3657, .T. ) ;
#8341=ADVANCED_FACE ( 'NONE', ( #11355 ), #7782, .T. ) ;
#8345=CYLINDRICAL_SURFACE ( 'NONE', #1335, 1.750000000000001554 ) ;
#8348=( BOUNDED_CURVE ( )  B_SPLINE_CURVE ( 3, ( #8940, #6348, #21237, #9692 ),
 .UNSPECIFIED., .F., .F. ) 
 B_SPLINE_CURVE_WITH_KNOTS ( ( 4, 4 ),
 ( 1.570796326794896558, 3.141592653589793116 ),
 .UNSPECIFIED. ) 
 CURVE ( )  GEOMETRIC_REPRESENTATION_ITEM ( )  RATIONAL_B_SPLINE_CURVE ( ( 1.000000000000000000, 0.8047378541243649375, 0.8047378541243649375, 1.000000000000000000 ) ) 
 REPRESENTATION_ITEM ( '' )  );
#8350=ORIENTED_EDGE ( 'NONE', *, *, #43073, .T. ) ;
#8357=ORIENTED_EDGE ( 'NONE', *, *, #4279, .F. ) ;
#8360=( BOUNDED_CURVE ( )  B_SPLINE_CURVE ( 3, ( #24421, #4893, #20556, #1062 ),
 .UNSPECIFIED., .F., .F. ) 
 B_SPLINE_CURVE_WITH_KNOTS ( ( 4, 4 ),
 ( 3.141592653589793116, 4.712388980384689674 ),
 .UNSPECIFIED. ) 
 CURVE ( )  GEOMETRIC_REPRESENTATION_ITEM ( )  RATIONAL_B_SPLINE_CURVE ( ( 1.000000000000000000, 0.8047378541243649375, 0.8047378541243649375, 1.000000000000000000 ) ) 
 REPRESENTATION_ITEM ( '' )  );
#8363=EDGE_CURVE ( 'NONE', #41009, #38609, #3833, .T. ) ;
#8364=CARTESIAN_POINT ( 'NONE',  ( 72.27890028733797578, 1.750000000000010436, -120.2068387089191219 ) ) ;
#8365=ORIENTED_EDGE ( 'NONE', *, *, #7332, .T. ) ;
#8366=ORIENTED_EDGE ( 'NONE', *, *, #10815, .T. ) ;
#8369=AXIS2_PLACEMENT_3D ( 'NONE', #6214, #5439, #21093 ) ;
#8370=CARTESIAN_POINT ( 'NONE',  ( 210.0000000000000568, 0.000000000000000000, 80.81828755692798438 ) ) ;
#8371=ORIENTED_EDGE ( 'NONE', *, *, #20884, .F. ) ;
#8375=CARTESIAN_POINT ( 'NONE',  ( 34.32915281903212446, 1.750000000000009548, -158.1565861772249377 ) ) ;
#8376=ORIENTED_EDGE ( 'NONE', *, *, #14890, .F. ) ;
#8378=CARTESIAN_POINT ( 'NONE',  ( 151.5540265531850537, 1.025126265847089435, 122.5682875569280128 ) ) ;
#8382=EDGE_CURVE ( 'NONE', #2039, #16293, #33963, .T. ) ;
#8390=VERTEX_POINT ( 'NONE', #22900 ) ;
#8392=EDGE_CURVE ( 'NONE', #48110, #9081, #39090, .T. ) ;
#8394=CARTESIAN_POINT ( 'NONE',  ( -86.69597344681494633, 1.750000000000009992, 160.8182875569279702 ) ) ;
#8403=CARTESIAN_POINT ( 'NONE',  ( -126.6959734468149321, -1.749999999999997113, -39.18171244307202983 ) ) ;
#8409=CARTESIAN_POINT ( 'NONE',  ( 73.30402655318508209, -1.750000000000009992, -159.1817124430720298 ) ) ;
#8410=EDGE_CURVE ( 'NONE', #37272, #36401, #12129, .T. ) ;
#8411=EDGE_LOOP ( 'NONE', ( #32390, #1352, #5238, #6441, #29699, #9781 ) ) ;
#8423=FACE_OUTER_BOUND ( 'NONE', #49059, .T. ) ;
#8432=CARTESIAN_POINT ( 'NONE',  ( 210.0000000000000568, 0.000000000000000000, 40.81828755692798438 ) ) ;
#8433=DIRECTION ( 'NONE',  ( 0.000000000000000000, 0.000000000000000000, 1.000000000000000000 ) ) ;
#8441=LINE ( 'NONE', #35902, #38224 ) ;
#8443=CARTESIAN_POINT ( 'NONE',  ( 210.0000000000000568, 2.143131898507881856E-16, -80.93171244307202983 ) ) ;
#8452=DIRECTION ( 'NONE',  ( -1.000000000000000000, -0.000000000000000000, -0.000000000000000000 ) ) ;
#8453=LINE ( 'NONE', #28201, #34461 ) ;
#8454=ORIENTED_EDGE ( 'NONE', *, *, #12863, .T. ) ;
#8456=ADVANCED_FACE ( 'NONE', ( #1588 ), #17235, .T. ) ;
#8458=VECTOR ( 'NONE', #2296, 1000.000000000000000 ) ;
#8459=LINE ( 'NONE', #48404, #28649 ) ;
#8465=CARTESIAN_POINT ( 'NONE',  ( -88.44597344681497475, 0.000000000000000000, 165.0000000000000000 ) ) ;
#8467=EDGE_CURVE ( 'NONE', #37272, #21250, #8535, .T. ) ;
#8469=VERTEX_POINT ( 'NONE', #32900 ) ;
#8471=CARTESIAN_POINT ( 'NONE',  ( -4.945973446814917018, -1.025126265847097207, 162.5682875569279986 ) ) ;
#8473=EDGE_LOOP ( 'NONE', ( #2104, #35133, #16095, #20960, #8205 ) ) ;
#8482=CARTESIAN_POINT ( 'NONE',  ( -85.67084718096784002, -1.750000000000009548, -118.1565861772249519 ) ) ;
#8484=CIRCLE ( 'NONE', #2708, 1.750000000000001554 ) ;
#8485=PLANE ( 'NONE',  #14444 ) ;
#8494=DIRECTION ( 'NONE',  ( 0.000000000000000000, 0.000000000000000000, -1.000000000000000000 ) ) ;
#8495=( BOUNDED_CURVE ( )  B_SPLINE_CURVE ( 3, ( #10371, #49309, #14193, #26021 ),
 .UNSPECIFIED., .F., .F. ) 
 B_SPLINE_CURVE_WITH_KNOTS ( ( 4, 4 ),
 ( 3.141592653589793116, 4.712388980384689674 ),
 .UNSPECIFIED. ) 
 CURVE ( )  GEOMETRIC_REPRESENTATION_ITEM ( )  RATIONAL_B_SPLINE_CURVE ( ( 1.000000000000000000, 0.8047378541243649375, 0.8047378541243649375, 1.000000000000000000 ) ) 
 REPRESENTATION_ITEM ( '' )  );
#8497=AXIS2_PLACEMENT_3D ( 'NONE', #30640, #42671, #27800 ) ;
#8501=( BOUNDED_CURVE ( )  B_SPLINE_CURVE ( 3, ( #3887, #34202, #49776, #6983 ),
 .UNSPECIFIED., .F., .F. ) 
 B_SPLINE_CURVE_WITH_KNOTS ( ( 4, 4 ),
 ( 1.570796326794896558, 3.141592653589793116 ),
 .UNSPECIFIED. ) 
 CURVE ( )  GEOMETRIC_REPRESENTATION_ITEM ( )  RATIONAL_B_SPLINE_CURVE ( ( 1.000000000000000000, 0.8047378541243649375, 0.8047378541243649375, 1.000000000000000000 ) ) 
 REPRESENTATION_ITEM ( '' )  );
#8508=CARTESIAN_POINT ( 'NONE',  ( 193.3040265531851105, -1.750000000000010658, -119.1817124430720440 ) ) ;
#8515=( BOUNDED_CURVE ( )  B_SPLINE_CURVE ( 3, ( #49278, #38561, #41381, #41881 ),
 .UNSPECIFIED., .F., .F. ) 
 B_SPLINE_CURVE_WITH_KNOTS ( ( 4, 4 ),
 ( 1.570796326794896558, 3.141592653589793116 ),
 .UNSPECIFIED. ) 
 CURVE ( )  GEOMETRIC_REPRESENTATION_ITEM ( )  RATIONAL_B_SPLINE_CURVE ( ( 1.000000000000000000, 0.8047378541243649375, 0.8047378541243649375, 1.000000000000000000 ) ) 
 REPRESENTATION_ITEM ( '' )  );
#8518=CARTESIAN_POINT ( 'NONE',  ( -6.695973446814940111, 0.000000000000000000, 165.0000000000000000 ) ) ;
#8521=VERTEX_POINT ( 'NONE', #24689 ) ;
#8526=CARTESIAN_POINT ( 'NONE',  ( 210.0000000000000568, 0.000000000000000000, -119.1817124430720440 ) ) ;
#8527=FACE_OUTER_BOUND ( 'NONE', #12146, .T. ) ;
#8530=FACE_OUTER_BOUND ( 'NONE', #16618, .T. ) ;
#8531=LINE ( 'NONE', #4678, #46670 ) ;
#8535=LINE ( 'NONE', #44406, #13093 ) ;
#8537=ADVANCED_FACE ( 'NONE', ( #16724 ), #20820, .T. ) ;
#8539=ORIENTED_EDGE ( 'NONE', *, *, #1410, .F. ) ;
#8540=CYLINDRICAL_SURFACE ( 'NONE', #11181, 1.750000000000015543 ) ;
#8544=AXIS2_PLACEMENT_3D ( 'NONE', #13061, #28478, #48423 ) ;
#8551=VECTOR ( 'NONE', #11805, 1000.000000000000000 ) ;
#8552=EDGE_CURVE ( 'NONE', #28177, #7812, #35997, .T. ) ;
#8555=ORIENTED_EDGE ( 'NONE', *, *, #46158, .F. ) ;
#8557=ORIENTED_EDGE ( 'NONE', *, *, #35287, .F. ) ;
#8560=CARTESIAN_POINT ( 'NONE',  ( -7.721099712662037540, -1.750000000000023537, 81.84341382277507648 ) ) ;
#8561=ORIENTED_EDGE ( 'NONE', *, *, #21222, .T. ) ;
#8572=CARTESIAN_POINT ( 'NONE',  ( -88.44597344681497475, 0.000000000000000000, 165.0000000000000000 ) ) ;
#8573=ORIENTED_EDGE ( 'NONE', *, *, #31944, .T. ) ;
#8574=EDGE_LOOP ( 'NONE', ( #24485, #28154, #49555, #41710, #41523, #20240 ) ) ;
#8576=CARTESIAN_POINT ( 'NONE',  ( -48.44597344681496054, -1.025126265847089657, 79.06828755692797017 ) ) ;
#8577=CARTESIAN_POINT ( 'NONE',  ( 210.0000000000000568, 0.000000000000000000, 160.8182875569279702 ) ) ;
#8578=DIRECTION ( 'NONE',  ( 0.000000000000000000, 0.000000000000000000, 1.000000000000000000 ) ) ;
#8583=DIRECTION ( 'NONE',  ( 1.000000000000000000, 0.000000000000000000, 0.000000000000000000 ) ) ;
#8584=CIRCLE ( 'NONE', #2809, 1.749999999999987566 ) ;
#8585=ORIENTED_EDGE ( 'NONE', *, *, #42131, .T. ) ;
#8592=ORIENTED_EDGE ( 'NONE', *, *, #12028, .T. ) ;
#8594=CARTESIAN_POINT ( 'NONE',  ( 195.0540265531851105, -1.025126265847089435, -77.43171244307200141 ) ) ;
#8599=ORIENTED_EDGE ( 'NONE', *, *, #45662, .F. ) ;
#8600=ORIENTED_EDGE ( 'NONE', *, *, #25887, .F. ) ;
#8602=DIRECTION ( 'NONE',  ( -0.000000000000000000, -0.000000000000000000, -1.000000000000000000 ) ) ;
#8611=CARTESIAN_POINT ( 'NONE',  ( -126.6959734468149321, 1.749999999999996891, 0.8182875569279768335 ) ) ;
#8614=ORIENTED_EDGE ( 'NONE', *, *, #46158, .T. ) ;
#8620=ORIENTED_EDGE ( 'NONE', *, *, #1170, .T. ) ;
#8621=VECTOR ( 'NONE', #26035, 1000.000000000000000 ) ;
#8624=EDGE_LOOP ( 'NONE', ( #43173, #11443, #44184, #37020, #16233, #13090 ) ) ;
#8625=EDGE_CURVE ( 'NONE', #14767, #6332, #39218, .T. ) ;
#8626=LINE ( 'NONE', #4008, #31394 ) ;
#8629=EDGE_CURVE ( 'NONE', #16858, #5180, #49642, .T. ) ;
#8630=CARTESIAN_POINT ( 'NONE',  ( -166.6959734468149463, -1.750000000000010658, 80.81828755692798438 ) ) ;
#8636=CARTESIAN_POINT ( 'NONE',  ( -166.6959734468149463, 1.750000000000010658, -119.1817124430720440 ) ) ;
#8637=CARTESIAN_POINT ( 'NONE',  ( 193.3040265531851105, -1.750000000000010214, -39.18171244307202983 ) ) ;
#8638=AXIS2_PLACEMENT_3D ( 'NONE', #42271, #11734, #49913 ) ;
#8639=AXIS2_PLACEMENT_3D ( 'NONE', #1004, #2001, #49896 ) ;
#8640=FACE_OUTER_BOUND ( 'NONE', #18034, .T. ) ;
#8643=EDGE_CURVE ( 'NONE', #40814, #47093, #21329, .T. ) ;
#8647=( BOUNDED_CURVE ( )  B_SPLINE_CURVE ( 3, ( #50529, #46183, #46441, #3625 ),
 .UNSPECIFIED., .F., .F. ) 
 B_SPLINE_CURVE_WITH_KNOTS ( ( 4, 4 ),
 ( 0.000000000000000000, 1.570796326794896558 ),
 .UNSPECIFIED. ) 
 CURVE ( )  GEOMETRIC_REPRESENTATION_ITEM ( )  RATIONAL_B_SPLINE_CURVE ( ( 1.000000000000000000, 0.8047378541243649375, 0.8047378541243649375, 1.000000000000000000 ) ) 
 REPRESENTATION_ITEM ( '' )  );
#8652=AXIS2_PLACEMENT_3D ( 'NONE', #21934, #49328, #10626 ) ;
#8655=CARTESIAN_POINT ( 'NONE',  ( -128.4459734468149179, 0.000000000000000000, -80.93171244307201562 ) ) ;
#8657=( BOUNDED_CURVE ( )  B_SPLINE_CURVE ( 3, ( #32555, #1500, #16898, #44069 ),
 .UNSPECIFIED., .F., .F. ) 
 B_SPLINE_CURVE_WITH_KNOTS ( ( 4, 4 ),
 ( 4.712388980384689674, 6.283185307179586232 ),
 .UNSPECIFIED. ) 
 CURVE ( )  GEOMETRIC_REPRESENTATION_ITEM ( )  RATIONAL_B_SPLINE_CURVE ( ( 1.000000000000000000, 0.8047378541243649375, 0.8047378541243649375, 1.000000000000000000 ) ) 
 REPRESENTATION_ITEM ( '' )  );
#8658=ORIENTED_EDGE ( 'NONE', *, *, #48813, .F. ) ;
#8660=CARTESIAN_POINT ( 'NONE',  ( 113.3040265531850537, 1.749999999999997335, -79.18171244307201562 ) ) ;
#8661=ORIENTED_EDGE ( 'NONE', *, *, #17382, .T. ) ;
#8663=VECTOR ( 'NONE', #37044, 1000.000000000000000 ) ;
#8668=ORIENTED_EDGE ( 'NONE', *, *, #20027, .F. ) ;
#8669=ADVANCED_FACE ( 'NONE', ( #29285 ), #44897, .F. ) ;
#8670=CARTESIAN_POINT ( 'NONE',  ( 210.0000000000000568, 0.000000000000000000, 82.56828755692799859 ) ) ;
#8676=VERTEX_POINT ( 'NONE', #25435 ) ;
#8677=LINE ( 'NONE', #4316, #21855 ) ;
#8679=ORIENTED_EDGE ( 'NONE', *, *, #48703, .T. ) ;
#8680=EDGE_CURVE ( 'NONE', #25250, #34536, #4144, .T. ) ;
#8682=VERTEX_POINT ( 'NONE', #5925 ) ;
#8683=ORIENTED_EDGE ( 'NONE', *, *, #22103, .T. ) ;
#8687=ORIENTED_EDGE ( 'NONE', *, *, #22439, .F. ) ;
#8696=CARTESIAN_POINT ( 'NONE',  ( -6.695973446814940111, 0.000000000000000000, 165.0000000000000000 ) ) ;
#8697=CARTESIAN_POINT ( 'NONE',  ( 32.27890028733795447, 1.750000000000009548, 41.84341382277508359 ) ) ;
#8704=EDGE_CURVE ( 'NONE', #19705, #48470, #30366, .T. ) ;
#8708=ORIENTED_EDGE ( 'NONE', *, *, #48405, .T. ) ;
#8722=CARTESIAN_POINT ( 'NONE',  ( -126.6959734468149321, 1.749999999999996891, 160.8182875569279702 ) ) ;
#8723=ORIENTED_EDGE ( 'NONE', *, *, #42189, .F. ) ;
#8728=ORIENTED_EDGE ( 'NONE', *, *, #48562, .T. ) ;
#8734=CARTESIAN_POINT ( 'NONE',  ( -206.6959734468149463, -1.750000000000010658, -119.1817124430720440 ) ) ;
#8744=CARTESIAN_POINT ( 'NONE',  ( 195.0540265531851105, 1.025126265847089879, 82.56828755692798438 ) ) ;
#8752=ORIENTED_EDGE ( 'NONE', *, *, #38823, .T. ) ;
#8754=AXIS2_PLACEMENT_3D ( 'NONE', #39926, #48317, #4756 ) ;
#8758=ORIENTED_EDGE ( 'NONE', *, *, #12442, .T. ) ;
#8760=ADVANCED_FACE ( 'NONE', ( #42081 ), #39024, .T. ) ;
#8764=CARTESIAN_POINT ( 'NONE',  ( 191.5540265531851105, 0.000000000000000000, -120.9317124430720156 ) ) ;
#8767=CARTESIAN_POINT ( 'NONE',  ( 71.55402655318505367, 0.000000000000000000, 165.0000000000000000 ) ) ;
#8774=CARTESIAN_POINT ( 'NONE',  ( 75.05402655318509630, 2.143131898507880377E-16, 82.56828755692799859 ) ) ;
#8776=ORIENTED_EDGE ( 'NONE', *, *, #25370, .T. ) ;
#8777=LINE ( 'NONE', #322, #49325 ) ;
#8778=VERTEX_POINT ( 'NONE', #43105 ) ;
#8781=CARTESIAN_POINT ( 'NONE',  ( 154.3291528190321458, 1.750000000000010214, 119.7931612910808781 ) ) ;
#8783=CARTESIAN_POINT ( 'NONE',  ( -84.94597344681494633, 2.143131898507880377E-16, -80.93171244307201562 ) ) ;
#8784=DIRECTION ( 'NONE',  ( -1.000000000000000000, -0.000000000000000000, -0.000000000000000000 ) ) ;
#8785=ORIENTED_EDGE ( 'NONE', *, *, #40244, .F. ) ;
#8792=ORIENTED_EDGE ( 'NONE', *, *, #24456, .F. ) ;
#8795=EDGE_CURVE ( 'NONE', #6842, #50107, #30550, .T. ) ;
#8796=( BOUNDED_CURVE ( )  B_SPLINE_CURVE ( 3, ( #13615, #43642, #40321, #12861 ),
 .UNSPECIFIED., .F., .F. ) 
 B_SPLINE_CURVE_WITH_KNOTS ( ( 4, 4 ),
 ( 4.712388980384689674, 6.283185307179586232 ),
 .UNSPECIFIED. ) 
 CURVE ( )  GEOMETRIC_REPRESENTATION_ITEM ( )  RATIONAL_B_SPLINE_CURVE ( ( 1.000000000000000000, 0.8047378541243649375, 0.8047378541243649375, 1.000000000000000000 ) ) 
 REPRESENTATION_ITEM ( '' )  );
#8799=CARTESIAN_POINT ( 'NONE',  ( 35.05402655318504657, 2.143131898507880377E-16, -157.4317124430720014 ) ) ;
#8801=ORIENTED_EDGE ( 'NONE', *, *, #45266, .T. ) ;
#8803=( BOUNDED_CURVE ( )  B_SPLINE_CURVE ( 3, ( #20866, #35796, #28565, #43696 ),
 .UNSPECIFIED., .F., .F. ) 
 B_SPLINE_CURVE_WITH_KNOTS ( ( 4, 4 ),
 ( 0.000000000000000000, 1.570796326794896558 ),
 .UNSPECIFIED. ) 
 CURVE ( )  GEOMETRIC_REPRESENTATION_ITEM ( )  RATIONAL_B_SPLINE_CURVE ( ( 1.000000000000000000, 0.8047378541243649375, 0.8047378541243649375, 1.000000000000000000 ) ) 
 REPRESENTATION_ITEM ( '' )  );
#8804=CYLINDRICAL_SURFACE ( 'NONE', #15276, 1.750000000000008438 ) ;
#8807=ORIENTED_EDGE ( 'NONE', *, *, #44670, .F. ) ;
#8808=ORIENTED_EDGE ( 'NONE', *, *, #1667, .T. ) ;
#8810=FACE_OUTER_BOUND ( 'NONE', #10918, .T. ) ;
#8812=( BOUNDED_CURVE ( )  B_SPLINE_CURVE ( 3, ( #10265, #29508, #49962, #33624 ),
 .UNSPECIFIED., .F., .F. ) 
 B_SPLINE_CURVE_WITH_KNOTS ( ( 4, 4 ),
 ( 0.000000000000000000, 1.570796326794896558 ),
 .UNSPECIFIED. ) 
 CURVE ( )  GEOMETRIC_REPRESENTATION_ITEM ( )  RATIONAL_B_SPLINE_CURVE ( ( 1.000000000000000000, 0.8047378541243649375, 0.8047378541243649375, 1.000000000000000000 ) ) 
 REPRESENTATION_ITEM ( '' )  );
#8814=DIRECTION ( 'NONE',  ( 0.000000000000000000, 0.000000000000000000, 1.000000000000000000 ) ) ;
#8816=VERTEX_POINT ( 'NONE', #20760 ) ;
#8817=CARTESIAN_POINT ( 'NONE',  ( -124.9459734468149463, 2.143131898507847836E-16, 79.06828755692798438 ) ) ;
#8833=CARTESIAN_POINT ( 'NONE',  ( -6.695973446814940111, 1.750000000000024203, -79.18171244307201562 ) ) ;
#8836=CARTESIAN_POINT ( 'NONE',  ( -127.7210997126620242, 1.749999999999996669, -38.15658617722495194 ) ) ;
#8857=VERTEX_POINT ( 'NONE', #40030 ) ;
#8860=ORIENTED_EDGE ( 'NONE', *, *, #43388, .F. ) ;
#8866=DIRECTION ( 'NONE',  ( 0.000000000000000000, 0.000000000000000000, 1.000000000000000000 ) ) ;
#8868=DIRECTION ( 'NONE',  ( 0.000000000000000000, 0.000000000000000000, -1.000000000000000000 ) ) ;
#8873=CYLINDRICAL_SURFACE ( 'NONE', #46562, 1.750000000000015543 ) ;
#8882=LINE ( 'NONE', #21187, #14850 ) ;
#8883=ADVANCED_FACE ( 'NONE', ( #1023 ), #12818, .T. ) ;
#8886=DIRECTION ( 'NONE',  ( 0.000000000000000000, 0.000000000000000000, 1.000000000000000000 ) ) ;
#8888=DIRECTION ( 'NONE',  ( 0.000000000000000000, 0.000000000000000000, 1.000000000000000000 ) ) ;
#8889=CARTESIAN_POINT ( 'NONE',  ( -128.4459734468149463, 1.025126265847081886, -40.93171244307202272 ) ) ;
#8890=CARTESIAN_POINT ( 'NONE',  ( 31.55402655318503236, -1.025126265847089879, -77.43171244307200141 ) ) ;
#8896=ORIENTED_EDGE ( 'NONE', *, *, #39529, .F. ) ;
#8901=ORIENTED_EDGE ( 'NONE', *, *, #2950, .T. ) ;
#8906=EDGE_CURVE ( 'NONE', #33474, #41151, #26255, .T. ) ;
#8908=EDGE_LOOP ( 'NONE', ( #47312, #39129, #6170, #41664, #27842 ) ) ;
#8912=CARTESIAN_POINT ( 'NONE',  ( -48.44597344681495343, 0.000000000000000000, 165.0000000000000000 ) ) ;
#8915=FACE_OUTER_BOUND ( 'NONE', #12822, .T. ) ;
#8917=ORIENTED_EDGE ( 'NONE', *, *, #28731, .T. ) ;
#8918=VERTEX_POINT ( 'NONE', #39527 ) ;
#8921=LINE ( 'NONE', #32290, #37352 ) ;
#8922=ORIENTED_EDGE ( 'NONE', *, *, #27708, .F. ) ;
#8923=EDGE_CURVE ( 'NONE', #42464, #3579, #35634, .T. ) ;
#8926=CARTESIAN_POINT ( 'NONE',  ( 195.0540265531851105, 1.025126265847089657, -80.93171244307201562 ) ) ;
#8932=EDGE_CURVE ( 'NONE', #11488, #43863, #40845, .T. ) ;
#8938=DIRECTION ( 'NONE',  ( 1.000000000000000000, 0.000000000000000000, 0.000000000000000000 ) ) ;
#8940=CARTESIAN_POINT ( 'NONE',  ( -6.695973446814940111, 1.750000000000023315, 0.8182875569279768335 ) ) ;
#8944=( BOUNDED_CURVE ( )  B_SPLINE_CURVE ( 3, ( #21258, #1765, #6615, #10467 ),
 .UNSPECIFIED., .F., .F. ) 
 B_SPLINE_CURVE_WITH_KNOTS ( ( 4, 4 ),
 ( 4.712388980384689674, 6.283185307179586232 ),
 .UNSPECIFIED. ) 
 CURVE ( )  GEOMETRIC_REPRESENTATION_ITEM ( )  RATIONAL_B_SPLINE_CURVE ( ( 1.000000000000000000, 0.8047378541243649375, 0.8047378541243649375, 1.000000000000000000 ) ) 
 REPRESENTATION_ITEM ( '' )  );
#8949=AXIS2_PLACEMENT_3D ( 'NONE', #47468, #28008, #8021 ) ;
#8951=CARTESIAN_POINT ( 'NONE',  ( -5.670847180967843570, 1.750000000000023537, 119.7931612910808781 ) ) ;
#8952=CARTESIAN_POINT ( 'NONE',  ( -46.69597344681494633, 1.750000000000009992, -159.1817124430720298 ) ) ;
#8955=AXIS2_PLACEMENT_3D ( 'NONE', #1032, #11826, #23616 ) ;
#8960=ORIENTED_EDGE ( 'NONE', *, *, #41855, .F. ) ;
#8971=CYLINDRICAL_SURFACE ( 'NONE', #25880, 1.750000000000015543 ) ;
#8982=CARTESIAN_POINT ( 'NONE',  ( 155.0540265531850537, -1.025126265847089213, 42.56828755692799149 ) ) ;
#8984=CARTESIAN_POINT ( 'NONE',  ( 193.3040265531851105, 1.750000000000010658, 80.81828755692798438 ) ) ;
#8990=CARTESIAN_POINT ( 'NONE',  ( 33.30402655318503946, 0.000000000000000000, 165.0000000000000000 ) ) ;
#8992=DIRECTION ( 'NONE',  ( 0.000000000000000000, 0.000000000000000000, 1.000000000000000000 ) ) ;
#8996=CARTESIAN_POINT ( 'NONE',  ( -4.945973446814903696, 2.143131898507912917E-16, -40.93171244307205825 ) ) ;
#9004=CARTESIAN_POINT ( 'NONE',  ( 210.0000000000000568, 0.000000000000000000, -39.18171244307202983 ) ) ;
#9005=FACE_OUTER_BOUND ( 'NONE', #29151, .T. ) ;
#9006=CARTESIAN_POINT ( 'NONE',  ( 111.5540265531850679, 0.000000000000000000, 165.0000000000000000 ) ) ;
#9009=LINE ( 'NONE', #36222, #4271 ) ;
#9014=ORIENTED_EDGE ( 'NONE', *, *, #19160, .F. ) ;
#9015=FACE_OUTER_BOUND ( 'NONE', #26441, .T. ) ;
#9018=ORIENTED_EDGE ( 'NONE', *, *, #36200, .F. ) ;
#9023=ORIENTED_EDGE ( 'NONE', *, *, #29806, .T. ) ;
#9029=VERTEX_POINT ( 'NONE', #18918 ) ;
#9031=CARTESIAN_POINT ( 'NONE',  ( 31.55402655318503236, -1.025126265847089657, 42.56828755692799149 ) ) ;
#9032=( BOUNDED_CURVE ( )  B_SPLINE_CURVE ( 3, ( #34397, #49485, #30538, #11034 ),
 .UNSPECIFIED., .F., .F. ) 
 B_SPLINE_CURVE_WITH_KNOTS ( ( 4, 4 ),
 ( 3.141592653589793116, 4.712388980384689674 ),
 .UNSPECIFIED. ) 
 CURVE ( )  GEOMETRIC_REPRESENTATION_ITEM ( )  RATIONAL_B_SPLINE_CURVE ( ( 1.000000000000000000, 0.8047378541243649375, 0.8047378541243649375, 1.000000000000000000 ) ) 
 REPRESENTATION_ITEM ( '' )  );
#9039=VERTEX_POINT ( 'NONE', #646 ) ;
#9041=EDGE_CURVE ( 'NONE', #20654, #43794, #16295, .T. ) ;
#9044=ORIENTED_EDGE ( 'NONE', *, *, #16272, .T. ) ;
#9050=EDGE_CURVE ( 'NONE', #47864, #5399, #7141, .T. ) ;
#9051=DIRECTION ( 'NONE',  ( -0.000000000000000000, -0.000000000000000000, -1.000000000000000000 ) ) ;
#9053=DIRECTION ( 'NONE',  ( -1.000000000000000000, -0.000000000000000000, -0.000000000000000000 ) ) ;
#9056=ORIENTED_EDGE ( 'NONE', *, *, #2878, .T. ) ;
#9062=CARTESIAN_POINT ( 'NONE',  ( -164.9459734468149463, 2.143131898507880377E-16, 79.06828755692797017 ) ) ;
#9067=CARTESIAN_POINT ( 'NONE',  ( 35.05402655318503946, 0.000000000000000000, 162.5682875569279702 ) ) ;
#9074=CARTESIAN_POINT ( 'NONE',  ( -206.6959734468149463, -1.750000000000009992, 160.8182875569279702 ) ) ;
#9081=VERTEX_POINT ( 'NONE', #39652 ) ;
#9087=EDGE_LOOP ( 'NONE', ( #15471, #43522 ) ) ;
#9088=( BOUNDED_CURVE ( )  B_SPLINE_CURVE ( 3, ( #38924, #928, #8120, #12207 ),
 .UNSPECIFIED., .F., .F. ) 
 B_SPLINE_CURVE_WITH_KNOTS ( ( 4, 4 ),
 ( 0.000000000000000000, 1.570796326794896558 ),
 .UNSPECIFIED. ) 
 CURVE ( )  GEOMETRIC_REPRESENTATION_ITEM ( )  RATIONAL_B_SPLINE_CURVE ( ( 1.000000000000000000, 0.8047378541243649375, 0.8047378541243649375, 1.000000000000000000 ) ) 
 REPRESENTATION_ITEM ( '' )  );
#9093=FACE_OUTER_BOUND ( 'NONE', #32831, .T. ) ;
#9094=( BOUNDED_CURVE ( )  B_SPLINE_CURVE ( 3, ( #18467, #15129, #2563, #10768 ),
 .UNSPECIFIED., .F., .F. ) 
 B_SPLINE_CURVE_WITH_KNOTS ( ( 4, 4 ),
 ( 1.570796326794896558, 3.141592653589793116 ),
 .UNSPECIFIED. ) 
 CURVE ( )  GEOMETRIC_REPRESENTATION_ITEM ( )  RATIONAL_B_SPLINE_CURVE ( ( 1.000000000000000000, 0.8047378541243649375, 0.8047378541243649375, 1.000000000000000000 ) ) 
 REPRESENTATION_ITEM ( '' )  );
#9095=ORIENTED_EDGE ( 'NONE', *, *, #26122, .F. ) ;
#9097=FACE_OUTER_BOUND ( 'NONE', #2647, .T. ) ;
#9098=VECTOR ( 'NONE', #25248, 1000.000000000000000 ) ;
#9102=ORIENTED_EDGE ( 'NONE', *, *, #33479, .F. ) ;
#9109=ORIENTED_EDGE ( 'NONE', *, *, #13729, .T. ) ;
#9118=VERTEX_POINT ( 'NONE', #42284 ) ;
#9119=VERTEX_POINT ( 'NONE', #23995 ) ;
#9120=DIRECTION ( 'NONE',  ( 0.000000000000000000, 0.000000000000000000, 1.000000000000000000 ) ) ;
#9123=CARTESIAN_POINT ( 'NONE',  ( 210.0000000000000568, 2.143131898507881856E-16, 119.0682875569279560 ) ) ;
#9125=CARTESIAN_POINT ( 'NONE',  ( 154.3291528190321458, 1.750000000000009548, -158.1565861772249377 ) ) ;
#9126=CARTESIAN_POINT ( 'NONE',  ( 191.5540265531851105, 0.000000000000000000, 165.0000000000000000 ) ) ;
#9127=VERTEX_POINT ( 'NONE', #30483 ) ;
#9132=EDGE_CURVE ( 'NONE', #9194, #24608, #11027, .T. ) ;
#9135=DIRECTION ( 'NONE',  ( -1.000000000000000000, -0.000000000000000000, -0.000000000000000000 ) ) ;
#9137=CARTESIAN_POINT ( 'NONE',  ( -44.94597344681493922, -1.025126265847089657, 79.06828755692797017 ) ) ;
#9144=CARTESIAN_POINT ( 'NONE',  ( -86.69597344681494633, -1.750000000000010658, 80.81828755692798438 ) ) ;
#9146=CARTESIAN_POINT ( 'NONE',  ( -208.4459734468149463, 0.000000000000000000, 2.568287556927978166 ) ) ;
#9148=CYLINDRICAL_SURFACE ( 'NONE', #32474, 1.750000000000010214 ) ;
#9151=CARTESIAN_POINT ( 'NONE',  ( -206.6959734468149463, 0.000000000000000000, 165.0000000000000000 ) ) ;
#9152=DIRECTION ( 'NONE',  ( -1.000000000000000000, 0.000000000000000000, 0.000000000000000000 ) ) ;
#9154=ORIENTED_EDGE ( 'NONE', *, *, #48665, .F. ) ;
#9155=EDGE_CURVE ( 'NONE', #16392, #17311, #563, .T. ) ;
#9156=VECTOR ( 'NONE', #7177, 1000.000000000000000 ) ;
#9159=LINE ( 'NONE', #1967, #44610 ) ;
#9161=LINE ( 'NONE', #33031, #12812 ) ;
#9162=VERTEX_POINT ( 'NONE', #48844 ) ;
#9173=ADVANCED_FACE ( 'NONE', ( #34008 ), #6796, .T. ) ;
#9176=CARTESIAN_POINT ( 'NONE',  ( -128.4459734468149179, 0.000000000000000000, 159.0682875569279986 ) ) ;
#9180=CARTESIAN_POINT ( 'NONE',  ( 33.30402655318503946, 1.750000000000010214, 40.81828755692798438 ) ) ;
#9181=FACE_OUTER_BOUND ( 'NONE', #40669, .T. ) ;
#9186=CARTESIAN_POINT ( 'NONE',  ( 115.0540265531850679, 0.000000000000000000, 162.5682875569279702 ) ) ;
#9187=VECTOR ( 'NONE', #2182, 1000.000000000000000 ) ;
#9189=CARTESIAN_POINT ( 'NONE',  ( -44.94597344681493922, 2.143131898507880377E-16, -0.9317124430720247208 ) ) ;
#9192=DIRECTION ( 'NONE',  ( -1.000000000000000000, -0.000000000000000000, -0.000000000000000000 ) ) ;
#9194=VERTEX_POINT ( 'NONE', #41441 ) ;
#9196=AXIS2_PLACEMENT_3D ( 'NONE', #1536, #40780, #21028 ) ;
#9197=CARTESIAN_POINT ( 'NONE',  ( -127.7210997126620242, -1.749999999999996669, 39.79316129108089228 ) ) ;
#9201=CARTESIAN_POINT ( 'NONE',  ( -127.7210997126620242, 1.749999999999996669, 159.7931612910809065 ) ) ;
#9203=CARTESIAN_POINT ( 'NONE',  ( 32.27890028733795447, -1.750000000000010214, -118.1565861772249519 ) ) ;
#9205=EDGE_CURVE ( 'NONE', #44495, #920, #21509, .T. ) ;
#9206=VERTEX_POINT ( 'NONE', #19284 ) ;
#9208=EDGE_CURVE ( 'NONE', #45429, #47093, #9639, .T. ) ;
#9213=VERTEX_POINT ( 'NONE', #13733 ) ;
#9222=( BOUNDED_CURVE ( )  B_SPLINE_CURVE ( 3, ( #8764, #16689, #28507, #8508 ),
 .UNSPECIFIED., .F., .F. ) 
 B_SPLINE_CURVE_WITH_KNOTS ( ( 4, 4 ),
 ( 0.000000000000000000, 1.570796326794896558 ),
 .UNSPECIFIED. ) 
 CURVE ( )  GEOMETRIC_REPRESENTATION_ITEM ( )  RATIONAL_B_SPLINE_CURVE ( ( 1.000000000000000000, 0.8047378541243649375, 0.8047378541243649375, 1.000000000000000000 ) ) 
 REPRESENTATION_ITEM ( '' )  );
#9229=ORIENTED_EDGE ( 'NONE', *, *, #47227, .F. ) ;
#9230=DIRECTION ( 'NONE',  ( -0.000000000000000000, -0.000000000000000000, -1.000000000000000000 ) ) ;
#9233=VERTEX_POINT ( 'NONE', #49345 ) ;
#9234=AXIS2_PLACEMENT_3D ( 'NONE', #6930, #26177, #34646 ) ;
#9238=VECTOR ( 'NONE', #43633, 1000.000000000000000 ) ;
#9240=CARTESIAN_POINT ( 'NONE',  ( -46.69597344681494633, 1.750000000000010658, 120.8182875569279702 ) ) ;
#9242=( BOUNDED_CURVE ( )  B_SPLINE_CURVE ( 3, ( #27246, #8007, #39061, #46694 ),
 .UNSPECIFIED., .F., .F. ) 
 B_SPLINE_CURVE_WITH_KNOTS ( ( 4, 4 ),
 ( 3.141592653589793116, 4.712388980384689674 ),
 .UNSPECIFIED. ) 
 CURVE ( )  GEOMETRIC_REPRESENTATION_ITEM ( )  RATIONAL_B_SPLINE_CURVE ( ( 1.000000000000000000, 0.8047378541243649375, 0.8047378541243649375, 1.000000000000000000 ) ) 
 REPRESENTATION_ITEM ( '' )  );
#9245=ORIENTED_EDGE ( 'NONE', *, *, #22385, .T. ) ;
#9246=ADVANCED_FACE ( 'NONE', ( #13977 ), #45258, .T. ) ;
#9247=ORIENTED_EDGE ( 'NONE', *, *, #25155, .T. ) ;
#9249=CARTESIAN_POINT ( 'NONE',  ( -88.44597344681497475, 0.000000000000000000, 82.56828755692801280 ) ) ;
#9255=FACE_OUTER_BOUND ( 'NONE', #28715, .T. ) ;
#9257=ADVANCED_FACE ( 'NONE', ( #3387 ), #8277, .T. ) ;
#9261=CARTESIAN_POINT ( 'NONE',  ( -128.4459734468149179, 0.000000000000000000, 122.5682875569279418 ) ) ;
#9267=CARTESIAN_POINT ( 'NONE',  ( -208.4459734468148611, -1.025126265847089657, -37.43171244307202272 ) ) ;
#9269=VERTEX_POINT ( 'NONE', #7776 ) ;
#9270=CARTESIAN_POINT ( 'NONE',  ( -204.9459734468149463, 2.143131898507880377E-16, 159.0682875569279702 ) ) ;
#9276=EDGE_CURVE ( 'NONE', #26090, #7778, #4419, .T. ) ;
#9278=ADVANCED_FACE ( 'NONE', ( #30607 ), #46207, .T. ) ;
#9279=ORIENTED_EDGE ( 'NONE', *, *, #49476, .F. ) ;
#9281=CARTESIAN_POINT ( 'NONE',  ( -128.4459734468149179, 0.000000000000000000, 2.568287556927950632 ) ) ;
#9282=DIRECTION ( 'NONE',  ( -1.000000000000000000, 0.000000000000000000, 0.000000000000000000 ) ) ;
#9284=CARTESIAN_POINT ( 'NONE',  ( 71.55402655318505367, 1.025126265847089435, -40.93171244307204404 ) ) ;
#9289=CARTESIAN_POINT ( 'NONE',  ( 115.0540265531850395, -1.025126265847081664, 82.56828755692798438 ) ) ;
#9292=CARTESIAN_POINT ( 'NONE',  ( 75.05402655318509630, 2.143131898507873721E-16, -165.0000000000000000 ) ) ;
#9293=EDGE_CURVE ( 'NONE', #46541, #12229, #26766, .T. ) ;
#9299=VERTEX_POINT ( 'NONE', #35231 ) ;
#9300=ORIENTED_EDGE ( 'NONE', *, *, #26782, .T. ) ;
#9306=AXIS2_PLACEMENT_3D ( 'NONE', #20675, #44502, #13728 ) ;
#9307=CARTESIAN_POINT ( 'NONE',  ( 191.5540265531851105, 0.000000000000000000, 39.06828755692798438 ) ) ;
#9314=CARTESIAN_POINT ( 'NONE',  ( -208.4459734468149463, 0.000000000000000000, 2.568287556927978166 ) ) ;
#9321=ORIENTED_EDGE ( 'NONE', *, *, #43183, .F. ) ;
#9322=DIRECTION ( 'NONE',  ( 0.000000000000000000, 0.000000000000000000, 1.000000000000000000 ) ) ;
#9324=PRODUCT ( 'wire', 'wire', '', ( #44619 ) ) ;
#9326=CYLINDRICAL_SURFACE ( 'NONE', #15146, 1.749999999999973799 ) ;
#9332=( BOUNDED_CURVE ( )  B_SPLINE_CURVE ( 3, ( #45329, #22266, #34582, #49911 ),
 .UNSPECIFIED., .F., .F. ) 
 B_SPLINE_CURVE_WITH_KNOTS ( ( 4, 4 ),
 ( 3.141592653589793116, 4.712388980384689674 ),
 .UNSPECIFIED. ) 
 CURVE ( )  GEOMETRIC_REPRESENTATION_ITEM ( )  RATIONAL_B_SPLINE_CURVE ( ( 1.000000000000000000, 0.8047378541243649375, 0.8047378541243649375, 1.000000000000000000 ) ) 
 REPRESENTATION_ITEM ( '' )  );
#9335=DIRECTION ( 'NONE',  ( -0.000000000000000000, -0.000000000000000000, -1.000000000000000000 ) ) ;
#9338=DIRECTION ( 'NONE',  ( 0.000000000000000000, 0.000000000000000000, -1.000000000000000000 ) ) ;
#9345=ORIENTED_EDGE ( 'NONE', *, *, #28107, .F. ) ;
#9348=AXIS2_PLACEMENT_3D ( 'NONE', #32521, #13744, #40710 ) ;
#9349=CARTESIAN_POINT ( 'NONE',  ( 73.30402655318508209, 0.000000000000000000, 165.0000000000000000 ) ) ;
#9352=DIRECTION ( 'NONE',  ( -0.000000000000000000, -0.000000000000000000, -1.000000000000000000 ) ) ;
#9355=CARTESIAN_POINT ( 'NONE',  ( 210.0000000000000568, 0.000000000000000000, -77.43171244307200141 ) ) ;
#9356=ORIENTED_EDGE ( 'NONE', *, *, #49111, .F. ) ;
#9366=VERTEX_POINT ( 'NONE', #17229 ) ;
#9378=AXIS2_PLACEMENT_3D ( 'NONE', #33147, #48723, #13620 ) ;
#9386=( BOUNDED_CURVE ( )  B_SPLINE_CURVE ( 3, ( #16461, #47709, #32114, #4895 ),
 .UNSPECIFIED., .F., .F. ) 
 B_SPLINE_CURVE_WITH_KNOTS ( ( 4, 4 ),
 ( 4.712388980384689674, 6.283185307179586232 ),
 .UNSPECIFIED. ) 
 CURVE ( )  GEOMETRIC_REPRESENTATION_ITEM ( )  RATIONAL_B_SPLINE_CURVE ( ( 1.000000000000000000, 0.8047378541243649375, 0.8047378541243649375, 1.000000000000000000 ) ) 
 REPRESENTATION_ITEM ( '' )  );
#9388=ADVANCED_FACE ( 'NONE', ( #8530 ), #25178, .T. ) ;
#9390=FACE_OUTER_BOUND ( 'NONE', #40343, .T. ) ;
#9391=( BOUNDED_CURVE ( )  B_SPLINE_CURVE ( 3, ( #12968, #40700, #36622, #44262 ),
 .UNSPECIFIED., .F., .F. ) 
 B_SPLINE_CURVE_WITH_KNOTS ( ( 4, 4 ),
 ( 4.712388980384689674, 6.283185307179586232 ),
 .UNSPECIFIED. ) 
 CURVE ( )  GEOMETRIC_REPRESENTATION_ITEM ( )  RATIONAL_B_SPLINE_CURVE ( ( 1.000000000000000000, 0.8047378541243649375, 0.8047378541243649375, 1.000000000000000000 ) ) 
 REPRESENTATION_ITEM ( '' )  );
#9394=CARTESIAN_POINT ( 'NONE',  ( 111.5540265531850679, 0.000000000000000000, 122.5682875569279560 ) ) ;
#9399=CARTESIAN_POINT ( 'NONE',  ( 210.0000000000000568, 0.000000000000000000, 160.8182875569279702 ) ) ;
#9401=ORIENTED_EDGE ( 'NONE', *, *, #39108, .F. ) ;
#9402=CARTESIAN_POINT ( 'NONE',  ( -124.9459734468149463, 2.143131898507847836E-16, 165.0000000000000000 ) ) ;
#9405=CARTESIAN_POINT ( 'NONE',  ( -167.7210997126620384, -1.750000000000010214, 121.8434138227750623 ) ) ;
#9411=EDGE_LOOP ( 'NONE', ( #2883, #23134, #14206, #21008, #1950 ) ) ;
#9420=EDGE_LOOP ( 'NONE', ( #2564, #38195, #33601, #14464, #46246, #32992 ) ) ;
#9425=ORIENTED_EDGE ( 'NONE', *, *, #48039, .F. ) ;
#9428=VECTOR ( 'NONE', #22877, 1000.000000000000000 ) ;
#9429=DIRECTION ( 'NONE',  ( -1.000000000000000000, -0.000000000000000000, -0.000000000000000000 ) ) ;
#9432=VECTOR ( 'NONE', #12970, 1000.000000000000000 ) ;
#9433=CARTESIAN_POINT ( 'NONE',  ( -205.6708471809678827, -1.750000000000010436, -80.20683870891910772 ) ) ;
#9434=DIRECTION ( 'NONE',  ( 1.000000000000000000, 0.000000000000000000, 0.000000000000000000 ) ) ;
#9437=CARTESIAN_POINT ( 'NONE',  ( 191.5540265531851105, 0.000000000000000000, 79.06828755692797017 ) ) ;
#9441=EDGE_CURVE ( 'NONE', #45821, #12693, #50693, .T. ) ;
#9442=CYLINDRICAL_SURFACE ( 'NONE', #25351, 1.749999999999973799 ) ;
#9452=CARTESIAN_POINT ( 'NONE',  ( -46.69597344681494633, -1.750000000000010658, -119.1817124430720440 ) ) ;
#9453=FACE_OUTER_BOUND ( 'NONE', #13320, .T. ) ;
#9456=CARTESIAN_POINT ( 'NONE',  ( 73.30402655318508209, -1.750000000000010658, -79.18171244307201562 ) ) ;
#9458=ORIENTED_EDGE ( 'NONE', *, *, #8337, .F. ) ;
#9465=ORIENTED_EDGE ( 'NONE', *, *, #15031, .T. ) ;
#9473=ORIENTED_EDGE ( 'NONE', *, *, #19898, .T. ) ;
#9480=DIRECTION ( 'NONE',  ( -1.000000000000000000, -0.000000000000000000, -0.000000000000000000 ) ) ;
#9486=FACE_OUTER_BOUND ( 'NONE', #35460, .T. ) ;
#9491=CARTESIAN_POINT ( 'NONE',  ( 210.0000000000000568, 0.000000000000000000, -39.18171244307202983 ) ) ;
#9495=DIRECTION ( 'NONE',  ( -1.000000000000000000, -0.000000000000000000, -0.000000000000000000 ) ) ;
#9499=FACE_OUTER_BOUND ( 'NONE', #43321, .T. ) ;
#9500=ORIENTED_EDGE ( 'NONE', *, *, #36183, .T. ) ;
#9502=EDGE_CURVE ( 'NONE', #40469, #21418, #22259, .T. ) ;
#9507=EDGE_CURVE ( 'NONE', #34169, #4486, #27526, .T. ) ;
#9508=VECTOR ( 'NONE', #24567, 1000.000000000000000 ) ;
#9513=VERTEX_POINT ( 'NONE', #28019 ) ;
#9514=CARTESIAN_POINT ( 'NONE',  ( -166.6959734468149463, -1.750000000000010214, 40.81828755692798438 ) ) ;
#9518=ORIENTED_EDGE ( 'NONE', *, *, #50611, .F. ) ;
#9521=( BOUNDED_CURVE ( )  B_SPLINE_CURVE ( 3, ( #46489, #23697, #16249, #19333 ),
 .UNSPECIFIED., .F., .F. ) 
 B_SPLINE_CURVE_WITH_KNOTS ( ( 4, 4 ),
 ( 4.712388980384689674, 6.283185307179586232 ),
 .UNSPECIFIED. ) 
 CURVE ( )  GEOMETRIC_REPRESENTATION_ITEM ( )  RATIONAL_B_SPLINE_CURVE ( ( 1.000000000000000000, 0.8047378541243649375, 0.8047378541243649375, 1.000000000000000000 ) ) 
 REPRESENTATION_ITEM ( '' )  );
#9523=ORIENTED_EDGE ( 'NONE', *, *, #16270, .F. ) ;
#9524=CARTESIAN_POINT ( 'NONE',  ( 151.5540265531850537, 0.000000000000000000, 165.0000000000000000 ) ) ;
#9525=CARTESIAN_POINT ( 'NONE',  ( -124.9459734468149463, 2.143131898507847836E-16, -0.9317124430719969652 ) ) ;
#9528=( BOUNDED_CURVE ( )  B_SPLINE_CURVE ( 3, ( #1257, #17392, #17882, #28694 ),
 .UNSPECIFIED., .F., .F. ) 
 B_SPLINE_CURVE_WITH_KNOTS ( ( 4, 4 ),
 ( 4.712388980384689674, 6.283185307179586232 ),
 .UNSPECIFIED. ) 
 CURVE ( )  GEOMETRIC_REPRESENTATION_ITEM ( )  RATIONAL_B_SPLINE_CURVE ( ( 1.000000000000000000, 0.8047378541243649375, 0.8047378541243649375, 1.000000000000000000 ) ) 
 REPRESENTATION_ITEM ( '' )  );
#9529=DIRECTION ( 'NONE',  ( -0.000000000000000000, -0.000000000000000000, -1.000000000000000000 ) ) ;
#9536=EDGE_CURVE ( 'NONE', #33010, #14624, #32762, .T. ) ;
#9538=AXIS2_PLACEMENT_3D ( 'NONE', #15160, #14905, #41848 ) ;
#9539=DIRECTION ( 'NONE',  ( -1.000000000000000000, -0.000000000000000000, -0.000000000000000000 ) ) ;
#9545=EDGE_CURVE ( 'NONE', #29162, #24955, #45652, .T. ) ;
#9546=( BOUNDED_CURVE ( )  B_SPLINE_CURVE ( 3, ( #15321, #47069, #43509, #30974 ),
 .UNSPECIFIED., .F., .F. ) 
 B_SPLINE_CURVE_WITH_KNOTS ( ( 4, 4 ),
 ( 0.000000000000000000, 1.570796326794896558 ),
 .UNSPECIFIED. ) 
 CURVE ( )  GEOMETRIC_REPRESENTATION_ITEM ( )  RATIONAL_B_SPLINE_CURVE ( ( 1.000000000000000000, 0.8047378541243649375, 0.8047378541243649375, 1.000000000000000000 ) ) 
 REPRESENTATION_ITEM ( '' )  );
#9548=ORIENTED_EDGE ( 'NONE', *, *, #29716, .T. ) ;
#9551=DIRECTION ( 'NONE',  ( -0.000000000000000000, -0.000000000000000000, -1.000000000000000000 ) ) ;
#9553=AXIS2_PLACEMENT_3D ( 'NONE', #24144, #39283, #7729 ) ;
#9555=ORIENTED_EDGE ( 'NONE', *, *, #20537, .T. ) ;
#9558=CARTESIAN_POINT ( 'NONE',  ( -44.94597344681493922, 2.143131898507880377E-16, 42.56828755692798438 ) ) ;
#9563=EDGE_CURVE ( 'NONE', #50334, #39140, #47097, .T. ) ;
#9567=CYLINDRICAL_SURFACE ( 'NONE', #10555, 1.750000000000008438 ) ;
#9568=FACE_OUTER_BOUND ( 'NONE', #13745, .T. ) ;
#9572=FACE_OUTER_BOUND ( 'NONE', #6734, .T. ) ;
#9577=CARTESIAN_POINT ( 'NONE',  ( 71.55402655318505367, 0.000000000000000000, -157.4317124430720014 ) ) ;
#9578=EDGE_CURVE ( 'NONE', #30056, #35621, #22558, .T. ) ;
#9584=CARTESIAN_POINT ( 'NONE',  ( -45.67084718096785423, 1.750000000000010214, 81.84341382277507648 ) ) ;
#9588=ORIENTED_EDGE ( 'NONE', *, *, #6094, .T. ) ;
#9591=ADVANCED_FACE ( 'NONE', ( #33153 ), #30293, .T. ) ;
#9592=CARTESIAN_POINT ( 'NONE',  ( 210.0000000000000568, 0.000000000000000000, 2.568287556927987048 ) ) ;
#9595=VERTEX_POINT ( 'NONE', #33896 ) ;
#9599=EDGE_CURVE ( 'NONE', #41270, #29317, #49490, .T. ) ;
#9613=EDGE_CURVE ( 'NONE', #5706, #29610, #34725, .T. ) ;
#9615=ORIENTED_EDGE ( 'NONE', *, *, #42119, .F. ) ;
#9617=CARTESIAN_POINT ( 'NONE',  ( -48.44597344681495343, 0.000000000000000000, -37.43171244307200141 ) ) ;
#9619=ORIENTED_EDGE ( 'NONE', *, *, #15792, .T. ) ;
#9621=ORIENTED_EDGE ( 'NONE', *, *, #11567, .T. ) ;
#9622=CARTESIAN_POINT ( 'NONE',  ( -84.94597344681494633, 2.143131898507880377E-16, -80.93171244307201562 ) ) ;
#9623=CYLINDRICAL_SURFACE ( 'NONE', #3460, 1.750000000000036193 ) ;
#9624=EDGE_LOOP ( 'NONE', ( #15315, #45539, #18156, #23223, #28370, #39665 ) ) ;
#9630=( BOUNDED_CURVE ( )  B_SPLINE_CURVE ( 3, ( #12989, #24559, #48362, #36124 ),
 .UNSPECIFIED., .F., .F. ) 
 B_SPLINE_CURVE_WITH_KNOTS ( ( 4, 4 ),
 ( 0.000000000000000000, 1.570796326794896780 ),
 .UNSPECIFIED. ) 
 CURVE ( )  GEOMETRIC_REPRESENTATION_ITEM ( )  RATIONAL_B_SPLINE_CURVE ( ( 1.000000000000000000, 0.8047378541243649375, 0.8047378541243649375, 1.000000000000000000 ) ) 
 REPRESENTATION_ITEM ( '' )  );
#9631=CARTESIAN_POINT ( 'NONE',  ( -46.69597344681494633, 0.000000000000000000, 165.0000000000000000 ) ) ;
#9632=ORIENTED_EDGE ( 'NONE', *, *, #34394, .F. ) ;
#9638=DIRECTION ( 'NONE',  ( 0.000000000000000000, 0.000000000000000000, 1.000000000000000000 ) ) ;
#9639=LINE ( 'NONE', #25287, #21229 ) ;
#9641=CARTESIAN_POINT ( 'NONE',  ( -208.4459734468148611, -1.025126265847089657, 119.0682875569279560 ) ) ;
#9647=DIRECTION ( 'NONE',  ( 1.000000000000000000, 0.000000000000000000, 0.000000000000000000 ) ) ;
#9649=CARTESIAN_POINT ( 'NONE',  ( -46.69597344681494633, -1.750000000000010214, -39.18171244307202983 ) ) ;
#9659=ORIENTED_EDGE ( 'NONE', *, *, #8337, .T. ) ;
#9661=EDGE_CURVE ( 'NONE', #30870, #47066, #35372, .T. ) ;
#9667=ORIENTED_EDGE ( 'NONE', *, *, #36268, .T. ) ;
#9670=DIRECTION ( 'NONE',  ( -1.000000000000000000, 0.000000000000000000, 0.000000000000000000 ) ) ;
#9674=CARTESIAN_POINT ( 'NONE',  ( 111.5540265531850537, -1.025126265847081886, -40.93171244307202272 ) ) ;
#9678=EDGE_LOOP ( 'NONE', ( #17514, #35885, #50695, #1901, #5877, #28093 ) ) ;
#9681=( BOUNDED_CURVE ( )  B_SPLINE_CURVE ( 3, ( #159, #8364, #27348, #31969 ),
 .UNSPECIFIED., .F., .F. ) 
 B_SPLINE_CURVE_WITH_KNOTS ( ( 4, 4 ),
 ( 4.712388980384689674, 6.283185307179586232 ),
 .UNSPECIFIED. ) 
 CURVE ( )  GEOMETRIC_REPRESENTATION_ITEM ( )  RATIONAL_B_SPLINE_CURVE ( ( 1.000000000000000000, 0.8047378541243649375, 0.8047378541243649375, 1.000000000000000000 ) ) 
 REPRESENTATION_ITEM ( '' )  );
#9684=AXIS2_PLACEMENT_3D ( 'NONE', #30328, #10566, #49520 ) ;
#9685=CARTESIAN_POINT ( 'NONE',  ( 33.30402655318503946, -1.750000000000010214, -39.18171244307202983 ) ) ;
#9687=CYLINDRICAL_SURFACE ( 'NONE', #35710, 1.749999999999987566 ) ;
#9688=( BOUNDED_CURVE ( )  B_SPLINE_CURVE ( 3, ( #17357, #44034, #47861, #44526 ),
 .UNSPECIFIED., .F., .F. ) 
 B_SPLINE_CURVE_WITH_KNOTS ( ( 4, 4 ),
 ( 4.712388980384689674, 6.283185307179586232 ),
 .UNSPECIFIED. ) 
 CURVE ( )  GEOMETRIC_REPRESENTATION_ITEM ( )  RATIONAL_B_SPLINE_CURVE ( ( 1.000000000000000000, 0.8047378541243649375, 0.8047378541243649375, 1.000000000000000000 ) ) 
 REPRESENTATION_ITEM ( '' )  );
#9689=FACE_OUTER_BOUND ( 'NONE', #42752, .T. ) ;
#9692=CARTESIAN_POINT ( 'NONE',  ( -4.945973446814903696, 2.143131898507912917E-16, 2.568287556928034121 ) ) ;
#9694=EDGE_LOOP ( 'NONE', ( #4665, #15751, #7304, #27447, #4501, #3224 ) ) ;
#9695=DIRECTION ( 'NONE',  ( -1.000000000000000000, 0.000000000000000000, 0.000000000000000000 ) ) ;
#9697=DIRECTION ( 'NONE',  ( -1.000000000000000000, -0.000000000000000000, -0.000000000000000000 ) ) ;
#9702=VERTEX_POINT ( 'NONE', #206 ) ;
#9705=CARTESIAN_POINT ( 'NONE',  ( -126.6959734468149321, 0.000000000000000000, 165.0000000000000000 ) ) ;
#9709=ORIENTED_EDGE ( 'NONE', *, *, #40106, .F. ) ;
#9713=CARTESIAN_POINT ( 'NONE',  ( 192.2789002873380184, -1.750000000000010214, 79.79316129108087807 ) ) ;
#9714=DIRECTION ( 'NONE',  ( -0.000000000000000000, -0.000000000000000000, -1.000000000000000000 ) ) ;
#9715=VERTEX_POINT ( 'NONE', #35115 ) ;
#9720=ORIENTED_EDGE ( 'NONE', *, *, #38891, .T. ) ;
#9728=CYLINDRICAL_SURFACE ( 'NONE', #35237, 1.750000000000001554 ) ;
#9738=CARTESIAN_POINT ( 'NONE',  ( 33.30402655318503946, 1.750000000000009992, 0.8182875569279768335 ) ) ;
#9744=CARTESIAN_POINT ( 'NONE',  ( -204.9459734468148895, -1.025126265847089435, -40.93171244307204404 ) ) ;
#9746=CIRCLE ( 'NONE', #39255, 1.750000000000015543 ) ;
#9748=CYLINDRICAL_SURFACE ( 'NONE', #1919, 1.750000000000015543 ) ;
#9750=AXIS2_PLACEMENT_3D ( 'NONE', #21051, #36738, #12333 ) ;
#9751=AXIS2_PLACEMENT_3D ( 'NONE', #29485, #44357, #6137 ) ;
#9752=DIRECTION ( 'NONE',  ( -1.000000000000000000, -0.000000000000000000, -0.000000000000000000 ) ) ;
#9753=DIRECTION ( 'NONE',  ( 0.000000000000000000, 0.000000000000000000, 1.000000000000000000 ) ) ;
#9754=DIRECTION ( 'NONE',  ( -1.000000000000000000, 0.000000000000000000, 0.000000000000000000 ) ) ;
#9758=ADVANCED_FACE ( 'NONE', ( #13996 ), #9148, .T. ) ;
#9765=DIRECTION ( 'NONE',  ( 0.000000000000000000, 0.000000000000000000, 1.000000000000000000 ) ) ;
#9766=LINE ( 'NONE', #2082, #35627 ) ;
#9768=CARTESIAN_POINT ( 'NONE',  ( 193.3040265531851105, -1.750000000000010658, 80.81828755692798438 ) ) ;
#9770=CARTESIAN_POINT ( 'NONE',  ( 210.0000000000000568, 2.143131898507880377E-16, -0.9317124430720331585 ) ) ;
#9772=CARTESIAN_POINT ( 'NONE',  ( 33.30402655318503946, 0.000000000000000000, -165.0000000000000000 ) ) ;
#9778=ORIENTED_EDGE ( 'NONE', *, *, #30694, .T. ) ;
#9781=ORIENTED_EDGE ( 'NONE', *, *, #43614, .F. ) ;
#9783=VECTOR ( 'NONE', #1482, 1000.000000000000000 ) ;
#9785=AXIS2_PLACEMENT_3D ( 'NONE', #18459, #21820, #9753 ) ;
#9787=CARTESIAN_POINT ( 'NONE',  ( -6.695973446814940111, -1.750000000000023315, -159.1817124430720298 ) ) ;
#9788=CARTESIAN_POINT ( 'NONE',  ( -124.9459734468149463, 2.143131898507847836E-16, -40.93171244307202983 ) ) ;
#9791=CARTESIAN_POINT ( 'NONE',  ( 113.3040265531850537, -1.749999999999997113, 40.81828755692798438 ) ) ;
#9792=ORIENTED_EDGE ( 'NONE', *, *, #21807, .F. ) ;
#9793=ORIENTED_EDGE ( 'NONE', *, *, #49891, .F. ) ;
#9801=VERTEX_POINT ( 'NONE', #21701 ) ;
#9802=CARTESIAN_POINT ( 'NONE',  ( -44.94597344681493922, 2.143131898507880377E-16, -160.9317124430720582 ) ) ;
#9809=DIRECTION ( 'NONE',  ( -1.000000000000000000, -0.000000000000000000, -0.000000000000000000 ) ) ;
#9811=LINE ( 'NONE', #48521, #24010 ) ;
#9813=CARTESIAN_POINT ( 'NONE',  ( 71.55402655318505367, 0.000000000000000000, 39.06828755692795596 ) ) ;
#9819=( BOUNDED_CURVE ( )  B_SPLINE_CURVE ( 3, ( #46561, #22744, #46316, #26087 ),
 .UNSPECIFIED., .F., .F. ) 
 B_SPLINE_CURVE_WITH_KNOTS ( ( 4, 4 ),
 ( 4.712388980384689674, 6.283185307179586232 ),
 .UNSPECIFIED. ) 
 CURVE ( )  GEOMETRIC_REPRESENTATION_ITEM ( )  RATIONAL_B_SPLINE_CURVE ( ( 1.000000000000000000, 0.8047378541243649375, 0.8047378541243649375, 1.000000000000000000 ) ) 
 REPRESENTATION_ITEM ( '' )  );
#9823=CARTESIAN_POINT ( 'NONE',  ( -125.6708471809678542, -1.749999999999996225, 1.843413822775058497 ) ) ;
#9829=( BOUNDED_CURVE ( )  B_SPLINE_CURVE ( 3, ( #3425, #49822, #23454, #14729 ),
 .UNSPECIFIED., .F., .F. ) 
 B_SPLINE_CURVE_WITH_KNOTS ( ( 4, 4 ),
 ( 4.712388980384689674, 6.283185307179586232 ),
 .UNSPECIFIED. ) 
 CURVE ( )  GEOMETRIC_REPRESENTATION_ITEM ( )  RATIONAL_B_SPLINE_CURVE ( ( 1.000000000000000000, 0.8047378541243649375, 0.8047378541243649375, 1.000000000000000000 ) ) 
 REPRESENTATION_ITEM ( '' )  );
#9830=CARTESIAN_POINT ( 'NONE',  ( 74.32915281903215998, -1.750000000000009326, 1.843413822775066269 ) ) ;
#9831=EDGE_CURVE ( 'NONE', #29600, #29991, #26159, .T. ) ;
#9833=VECTOR ( 'NONE', #42899, 1000.000000000000000 ) ;
#9834=CARTESIAN_POINT ( 'NONE',  ( 73.30402655318508209, 0.000000000000000000, 165.0000000000000000 ) ) ;
#9838=( BOUNDED_CURVE ( )  B_SPLINE_CURVE ( 3, ( #3797, #19444, #3278, #45350 ),
 .UNSPECIFIED., .F., .F. ) 
 B_SPLINE_CURVE_WITH_KNOTS ( ( 4, 4 ),
 ( 4.712388980384689674, 6.283185307179586232 ),
 .UNSPECIFIED. ) 
 CURVE ( )  GEOMETRIC_REPRESENTATION_ITEM ( )  RATIONAL_B_SPLINE_CURVE ( ( 1.000000000000000000, 0.8047378541243649375, 0.8047378541243649375, 1.000000000000000000 ) ) 
 REPRESENTATION_ITEM ( '' )  );
#9846=EDGE_CURVE ( 'NONE', #41166, #6332, #42455, .T. ) ;
#9849=CARTESIAN_POINT ( 'NONE',  ( -86.69597344681496054, 0.000000000000000000, 165.0000000000000000 ) ) ;
#9850=CARTESIAN_POINT ( 'NONE',  ( -205.6708471809678827, 1.750000000000010214, 79.79316129108087807 ) ) ;
#9857=VECTOR ( 'NONE', #41189, 1000.000000000000000 ) ;
#9861=ORIENTED_EDGE ( 'NONE', *, *, #28193, .F. ) ;
#9863=CYLINDRICAL_SURFACE ( 'NONE', #20139, 1.750000000000008438 ) ;
#9864=CARTESIAN_POINT ( 'NONE',  ( -206.6959734468149463, 1.750000000000009992, -159.1817124430720298 ) ) ;
#9866=VECTOR ( 'NONE', #26417, 1000.000000000000000 ) ;
#9868=CARTESIAN_POINT ( 'NONE',  ( -125.6708471809678542, 1.749999999999996669, 39.79316129108089228 ) ) ;
#9872=FACE_OUTER_BOUND ( 'NONE', #41409, .T. ) ;
#9874=CARTESIAN_POINT ( 'NONE',  ( 153.3040265531850537, 1.750000000000009992, -159.1817124430720298 ) ) ;
#9877=ORIENTED_EDGE ( 'NONE', *, *, #12, .F. ) ;
#9878=DIRECTION ( 'NONE',  ( 0.000000000000000000, 0.000000000000000000, 1.000000000000000000 ) ) ;
#9885=CYLINDRICAL_SURFACE ( 'NONE', #27333, 1.750000000000036193 ) ;
#9887=ADVANCED_FACE ( 'NONE', ( #46276 ), #34797, .T. ) ;
#9897=CARTESIAN_POINT ( 'NONE',  ( 115.0540265531850395, 2.143131898507847836E-16, -77.43171244307204404 ) ) ;
#9899=CYLINDRICAL_SURFACE ( 'NONE', #47884, 1.750000000000008438 ) ;
#9903=ORIENTED_EDGE ( 'NONE', *, *, #46373, .F. ) ;
#9905=EDGE_LOOP ( 'NONE', ( #12263, #3205, #23516, #26832, #35487, #11554 ) ) ;
#9907=LINE ( 'NONE', #26324, #44233 ) ;
#9908=DIRECTION ( 'NONE',  ( 0.000000000000000000, 0.000000000000000000, 1.000000000000000000 ) ) ;
#9914=CARTESIAN_POINT ( 'NONE',  ( -208.4459734468149463, 0.000000000000000000, -40.93171244307202983 ) ) ;
#9916=ORIENTED_EDGE ( 'NONE', *, *, #26682, .T. ) ;
#9918=CARTESIAN_POINT ( 'NONE',  ( 210.0000000000000568, 0.000000000000000000, -159.1817124430720298 ) ) ;
#9921=( BOUNDED_CURVE ( )  B_SPLINE_CURVE ( 3, ( #36219, #810, #35968, #50605 ),
 .UNSPECIFIED., .F., .F. ) 
 B_SPLINE_CURVE_WITH_KNOTS ( ( 4, 4 ),
 ( 4.712388980384689674, 6.283185307179586232 ),
 .UNSPECIFIED. ) 
 CURVE ( )  GEOMETRIC_REPRESENTATION_ITEM ( )  RATIONAL_B_SPLINE_CURVE ( ( 1.000000000000000000, 0.8047378541243649375, 0.8047378541243649375, 1.000000000000000000 ) ) 
 REPRESENTATION_ITEM ( '' )  );
#9922=ORIENTED_EDGE ( 'NONE', *, *, #20027, .T. ) ;
#9923=PLANE ( 'NONE',  #10667 ) ;
#9924=EDGE_CURVE ( 'NONE', #4803, #15022, #36377, .T. ) ;
#9925=CARTESIAN_POINT ( 'NONE',  ( 113.3040265531850537, -1.749999999999997335, 120.8182875569279702 ) ) ;
#9926=CARTESIAN_POINT ( 'NONE',  ( -84.94597344681494633, 2.143131898507880377E-16, 165.0000000000000000 ) ) ;
#9929=DIRECTION ( 'NONE',  ( -0.000000000000000000, -0.000000000000000000, -1.000000000000000000 ) ) ;
#9931=CARTESIAN_POINT ( 'NONE',  ( -48.44597344681495343, 0.000000000000000000, -165.0000000000000000 ) ) ;
#9936=CARTESIAN_POINT ( 'NONE',  ( -206.6959734468149463, -1.750000000000010658, -79.18171244307201562 ) ) ;
#9939=CARTESIAN_POINT ( 'NONE',  ( -208.4459734468148611, 1.025126265847089213, -160.9317124430720014 ) ) ;
#9942=DIRECTION ( 'NONE',  ( -1.000000000000000000, -0.000000000000000000, -0.000000000000000000 ) ) ;
#9944=EDGE_CURVE ( 'NONE', #3012, #49797, #41593, .T. ) ;
#9947=CARTESIAN_POINT ( 'NONE',  ( -205.6708471809678827, -1.750000000000009548, 81.84341382277507648 ) ) ;
#9948=EDGE_CURVE ( 'NONE', #37343, #16704, #29453, .T. ) ;
#9956=ORIENTED_EDGE ( 'NONE', *, *, #9944, .F. ) ;
#9958=FACE_OUTER_BOUND ( 'NONE', #25464, .T. ) ;
#9962=ADVANCED_FACE ( 'NONE', ( #35303 ), #8345, .T. ) ;
#9969=AXIS2_PLACEMENT_3D ( 'NONE', #4464, #17019, #48022 ) ;
#9971=CARTESIAN_POINT ( 'NONE',  ( -166.6959734468149463, 1.750000000000009992, 160.8182875569279702 ) ) ;
#9974=AXIS2_PLACEMENT_3D ( 'NONE', #42015, #38688, #30212 ) ;
#9979=LINE ( 'NONE', #17915, #29153 ) ;
#9980=( BOUNDED_CURVE ( )  B_SPLINE_CURVE ( 3, ( #7203, #3335, #45659, #26949 ),
 .UNSPECIFIED., .F., .F. ) 
 B_SPLINE_CURVE_WITH_KNOTS ( ( 4, 4 ),
 ( 1.570796326794896558, 3.141592653589793116 ),
 .UNSPECIFIED. ) 
 CURVE ( )  GEOMETRIC_REPRESENTATION_ITEM ( )  RATIONAL_B_SPLINE_CURVE ( ( 1.000000000000000000, 0.8047378541243649375, 0.8047378541243649375, 1.000000000000000000 ) ) 
 REPRESENTATION_ITEM ( '' )  );
#9981=ORIENTED_EDGE ( 'NONE', *, *, #38433, .F. ) ;
#9985=ORIENTED_EDGE ( 'NONE', *, *, #14576, .F. ) ;
#9986=ORIENTED_EDGE ( 'NONE', *, *, #9992, .T. ) ;
#9989=( BOUNDED_CURVE ( )  B_SPLINE_CURVE ( 3, ( #15500, #3436, #39385, #34256 ),
 .UNSPECIFIED., .F., .F. ) 
 B_SPLINE_CURVE_WITH_KNOTS ( ( 4, 4 ),
 ( 1.570796326794896558, 3.141592653589793116 ),
 .UNSPECIFIED. ) 
 CURVE ( )  GEOMETRIC_REPRESENTATION_ITEM ( )  RATIONAL_B_SPLINE_CURVE ( ( 1.000000000000000000, 0.8047378541243649375, 0.8047378541243649375, 1.000000000000000000 ) ) 
 REPRESENTATION_ITEM ( '' )  );
#9990=DIRECTION ( 'NONE',  ( -1.000000000000000000, -0.000000000000000000, -0.000000000000000000 ) ) ;
#9991=ORIENTED_EDGE ( 'NONE', *, *, #28142, .F. ) ;
#9992=EDGE_CURVE ( 'NONE', #47482, #49500, #47295, .T. ) ;
#9993=CARTESIAN_POINT ( 'NONE',  ( -206.6959734468149463, 1.750000000000010658, 80.81828755692798438 ) ) ;
#9996=CARTESIAN_POINT ( 'NONE',  ( 73.30402655318508209, 0.000000000000000000, -165.0000000000000000 ) ) ;
#10010=DIRECTION ( 'NONE',  ( -0.000000000000000000, -0.000000000000000000, -1.000000000000000000 ) ) ;
#10011=ORIENTED_EDGE ( 'NONE', *, *, #2294, .F. ) ;
#10012=CARTESIAN_POINT ( 'NONE',  ( 210.0000000000000568, 0.000000000000000000, -77.43171244307200141 ) ) ;
#10014=CYLINDRICAL_SURFACE ( 'NONE', #10552, 1.750000000000008438 ) ;
#10018=ADVANCED_FACE ( 'NONE', ( #46778 ), #15525, .T. ) ;
#10022=ORIENTED_EDGE ( 'NONE', *, *, #19513, .F. ) ;
#10024=ORIENTED_EDGE ( 'NONE', *, *, #13089, .F. ) ;
#10026=CARTESIAN_POINT ( 'NONE',  ( -7.721099712662037540, -1.750000000000023315, 41.84341382277508359 ) ) ;
#10031=CARTESIAN_POINT ( 'NONE',  ( 192.2789002873380184, -1.750000000000010214, 81.84341382277507648 ) ) ;
#10033=CARTESIAN_POINT ( 'NONE',  ( 192.2789002873380184, -1.750000000000010214, -80.20683870891910772 ) ) ;
#10036=CARTESIAN_POINT ( 'NONE',  ( 115.0540265531850395, 2.143131898507847836E-16, -157.4317124430720582 ) ) ;
#10039=CARTESIAN_POINT ( 'NONE',  ( 210.0000000000000568, 2.143131898507880377E-16, -160.9317124430720298 ) ) ;
#10040=ORIENTED_EDGE ( 'NONE', *, *, #12961, .F. ) ;
#10041=VERTEX_POINT ( 'NONE', #24250 ) ;
#10046=CARTESIAN_POINT ( 'NONE',  ( -128.4459734468149463, -1.025126265847082108, 122.5682875569279702 ) ) ;
#10047=EDGE_LOOP ( 'NONE', ( #11824, #3912, #37045, #19623, #23247, #48530 ) ) ;
#10056=CARTESIAN_POINT ( 'NONE',  ( -205.6708471809678827, 1.750000000000009548, 161.8434138227750907 ) ) ;
#10060=CARTESIAN_POINT ( 'NONE',  ( 153.3040265531850537, 1.750000000000010214, -39.18171244307202983 ) ) ;
#10065=ORIENTED_EDGE ( 'NONE', *, *, #13074, .T. ) ;
#10069=DIRECTION ( 'NONE',  ( 1.000000000000000000, 0.000000000000000000, 0.000000000000000000 ) ) ;
#10071=DIRECTION ( 'NONE',  ( -1.000000000000000000, -0.000000000000000000, -0.000000000000000000 ) ) ;
#10073=DIRECTION ( 'NONE',  ( -0.000000000000000000, -0.000000000000000000, -1.000000000000000000 ) ) ;
#10076=AXIS2_PLACEMENT_3D ( 'NONE', #3303, #38237, #46116 ) ;
#10086=ADVANCED_FACE ( 'NONE', ( #27072 ), #42704, .T. ) ;
#10088=FACE_OUTER_BOUND ( 'NONE', #47952, .T. ) ;
#10094=CARTESIAN_POINT ( 'NONE',  ( -206.6959734468149463, -1.750000000000010214, -39.18171244307202983 ) ) ;
#10095=VERTEX_POINT ( 'NONE', #38896 ) ;
#10096=ORIENTED_EDGE ( 'NONE', *, *, #7057, .F. ) ;
#10098=CARTESIAN_POINT ( 'NONE',  ( -164.9459734468149463, 2.143131898507880377E-16, 119.0682875569279702 ) ) ;
#10099=ORIENTED_EDGE ( 'NONE', *, *, #37230, .T. ) ;
#10101=CARTESIAN_POINT ( 'NONE',  ( 210.0000000000000568, 2.143131898507881856E-16, 79.06828755692797017 ) ) ;
#10103=CARTESIAN_POINT ( 'NONE',  ( -166.6959734468149463, 1.750000000000009992, 160.8182875569279702 ) ) ;
#10107=AXIS2_PLACEMENT_3D ( 'NONE', #12220, #39440, #429 ) ;
#10112=AXIS2_PLACEMENT_3D ( 'NONE', #26304, #21425, #44766 ) ;
#10115=CARTESIAN_POINT ( 'NONE',  ( 111.5540265531850537, -1.025126265847081442, 162.5682875569279133 ) ) ;
#10116=CARTESIAN_POINT ( 'NONE',  ( 192.2789002873380184, -1.750000000000009548, -0.2068387089191121020 ) ) ;
#10117=ORIENTED_EDGE ( 'NONE', *, *, #28149, .F. ) ;
#10120=CARTESIAN_POINT ( 'NONE',  ( -124.9459734468149321, 1.025126265847081886, 39.06828755692799149 ) ) ;
#10123=( BOUNDED_CURVE ( )  B_SPLINE_CURVE ( 3, ( #41592, #10298, #25958, #33907 ),
 .UNSPECIFIED., .F., .F. ) 
 B_SPLINE_CURVE_WITH_KNOTS ( ( 4, 4 ),
 ( 3.141592653589793116, 4.712388980384689674 ),
 .UNSPECIFIED. ) 
 CURVE ( )  GEOMETRIC_REPRESENTATION_ITEM ( )  RATIONAL_B_SPLINE_CURVE ( ( 1.000000000000000000, 0.8047378541243649375, 0.8047378541243649375, 1.000000000000000000 ) ) 
 REPRESENTATION_ITEM ( '' )  );
#10126=DIRECTION ( 'NONE',  ( -1.000000000000000000, -0.000000000000000000, -0.000000000000000000 ) ) ;
#10128=CARTESIAN_POINT ( 'NONE',  ( 73.30402655318508209, 1.750000000000009992, 0.8182875569279768335 ) ) ;
#10131=( BOUNDED_CURVE ( )  B_SPLINE_CURVE ( 3, ( #19900, #42241, #7100, #46811 ),
 .UNSPECIFIED., .F., .F. ) 
 B_SPLINE_CURVE_WITH_KNOTS ( ( 4, 4 ),
 ( 0.000000000000000000, 1.570796326794896558 ),
 .UNSPECIFIED. ) 
 CURVE ( )  GEOMETRIC_REPRESENTATION_ITEM ( )  RATIONAL_B_SPLINE_CURVE ( ( 1.000000000000000000, 0.8047378541243649375, 0.8047378541243649375, 1.000000000000000000 ) ) 
 REPRESENTATION_ITEM ( '' )  );
#10132=CARTESIAN_POINT ( 'NONE',  ( 71.55402655318505367, -1.025126265847089435, -40.93171244307204404 ) ) ;
#10133=DIRECTION ( 'NONE',  ( -0.000000000000000000, -0.000000000000000000, -1.000000000000000000 ) ) ;
#10140=ADVANCED_FACE ( 'NONE', ( #9097 ), #25494, .T. ) ;
#10143=( BOUNDED_CURVE ( )  B_SPLINE_CURVE ( 3, ( #46331, #11226, #26865, #34842 ),
 .UNSPECIFIED., .F., .F. ) 
 B_SPLINE_CURVE_WITH_KNOTS ( ( 4, 4 ),
 ( 0.000000000000000000, 1.570796326794896558 ),
 .UNSPECIFIED. ) 
 CURVE ( )  GEOMETRIC_REPRESENTATION_ITEM ( )  RATIONAL_B_SPLINE_CURVE ( ( 1.000000000000000000, 0.8047378541243649375, 0.8047378541243649375, 1.000000000000000000 ) ) 
 REPRESENTATION_ITEM ( '' )  );
#10146=ADVANCED_FACE ( 'NONE', ( #44469 ), #21140, .T. ) ;
#10147=VECTOR ( 'NONE', #38491, 1000.000000000000000 ) ;
#10151=LINE ( 'NONE', #33767, #9857 ) ;
#10152=DIRECTION ( 'NONE',  ( -1.000000000000000000, -0.000000000000000000, -0.000000000000000000 ) ) ;
#10159=CARTESIAN_POINT ( 'NONE',  ( 73.30402655318508209, 1.750000000000010214, 40.81828755692798438 ) ) ;
#10160=VECTOR ( 'NONE', #46877, 1000.000000000000000 ) ;
#10166=EDGE_LOOP ( 'NONE', ( #4937, #42763, #45111, #44914, #25432 ) ) ;
#10179=ORIENTED_EDGE ( 'NONE', *, *, #3344, .F. ) ;
#10186=CARTESIAN_POINT ( 'NONE',  ( 72.27890028733797578, -1.750000000000010214, 79.79316129108087807 ) ) ;
#10188=CARTESIAN_POINT ( 'NONE',  ( 155.0540265531850537, 2.143131898507880377E-16, 165.0000000000000000 ) ) ;
#10190=DIRECTION ( 'NONE',  ( -0.000000000000000000, -0.000000000000000000, -1.000000000000000000 ) ) ;
#10198=EDGE_CURVE ( 'NONE', #7355, #9513, #38621, .T. ) ;
#10208=CARTESIAN_POINT ( 'NONE',  ( 155.0540265531850537, 1.025126265847089657, -120.9317124430720440 ) ) ;
#10209=EDGE_LOOP ( 'NONE', ( #39783, #1652, #49691, #25955, #43220, #35433 ) ) ;
#10216=CARTESIAN_POINT ( 'NONE',  ( -124.9459734468149321, 1.025126265847081664, 2.568287556927973281 ) ) ;
#10218=FACE_OUTER_BOUND ( 'NONE', #40098, .T. ) ;
#10225=EDGE_LOOP ( 'NONE', ( #39027, #17856, #46245, #17934, #591, #27097 ) ) ;
#10226=CARTESIAN_POINT ( 'NONE',  ( -48.44597344681495343, 0.000000000000000000, -157.4317124430720014 ) ) ;
#10227=DIRECTION ( 'NONE',  ( -1.000000000000000000, -0.000000000000000000, -0.000000000000000000 ) ) ;
#10232=ORIENTED_EDGE ( 'NONE', *, *, #2632, .F. ) ;
#10236=EDGE_CURVE ( 'NONE', #7661, #18090, #37575, .T. ) ;
#10243=CIRCLE ( 'NONE', #38938, 1.750000000000008438 ) ;
#10244=ORIENTED_EDGE ( 'NONE', *, *, #19075, .F. ) ;
#10248=ORIENTED_EDGE ( 'NONE', *, *, #33122, .F. ) ;
#10249=EDGE_CURVE ( 'NONE', #10420, #47806, #24522, .T. ) ;
#10252=ADVANCED_FACE ( 'NONE', ( #14963 ), #26506, .F. ) ;
#10258=CYLINDRICAL_SURFACE ( 'NONE', #41492, 1.750000000000008438 ) ;
#10260=CARTESIAN_POINT ( 'NONE',  ( 153.3040265531850537, 1.750000000000009992, 160.8182875569279702 ) ) ;
#10263=ORIENTED_EDGE ( 'NONE', *, *, #13985, .F. ) ;
#10265=CARTESIAN_POINT ( 'NONE',  ( -124.9459734468149463, 2.143131898507847836E-16, 119.0682875569279844 ) ) ;
#10268=CARTESIAN_POINT ( 'NONE',  ( -125.6708471809678542, 1.749999999999996891, -118.1565861772249661 ) ) ;
#10270=CARTESIAN_POINT ( 'NONE',  ( 195.0540265531851105, -1.025126265847089213, 42.56828755692799149 ) ) ;
#10279=EDGE_LOOP ( 'NONE', ( #4296, #37742, #15771, #5995, #30125, #42949 ) ) ;
#10280=LINE ( 'NONE', #25684, #35306 ) ;
#10285=( BOUNDED_CURVE ( )  B_SPLINE_CURVE ( 3, ( #15940, #19511, #4138, #35200 ),
 .UNSPECIFIED., .F., .F. ) 
 B_SPLINE_CURVE_WITH_KNOTS ( ( 4, 4 ),
 ( 0.000000000000000000, 1.570796326794896558 ),
 .UNSPECIFIED. ) 
 CURVE ( )  GEOMETRIC_REPRESENTATION_ITEM ( )  RATIONAL_B_SPLINE_CURVE ( ( 1.000000000000000000, 0.8047378541243649375, 0.8047378541243649375, 1.000000000000000000 ) ) 
 REPRESENTATION_ITEM ( '' )  );
#10291=VECTOR ( 'NONE', #34293, 1000.000000000000000 ) ;
#10292=CARTESIAN_POINT ( 'NONE',  ( -165.6708471809677974, 1.750000000000010214, -78.15658617722490931 ) ) ;
#10295=( BOUNDED_CURVE ( )  B_SPLINE_CURVE ( 3, ( #7364, #27635, #3489, #42741 ),
 .UNSPECIFIED., .F., .F. ) 
 B_SPLINE_CURVE_WITH_KNOTS ( ( 4, 4 ),
 ( 1.570796326794896558, 3.141592653589793116 ),
 .UNSPECIFIED. ) 
 CURVE ( )  GEOMETRIC_REPRESENTATION_ITEM ( )  RATIONAL_B_SPLINE_CURVE ( ( 1.000000000000000000, 0.8047378541243649375, 0.8047378541243649375, 1.000000000000000000 ) ) 
 REPRESENTATION_ITEM ( '' )  );
#10298=CARTESIAN_POINT ( 'NONE',  ( 35.05402655318504657, -1.025126265847089435, 122.5682875569280128 ) ) ;
#10303=CARTESIAN_POINT ( 'NONE',  ( 191.5540265531851105, 0.000000000000000000, -157.4317124430720582 ) ) ;
#10317=AXIS2_PLACEMENT_3D ( 'NONE', #35935, #43348, #16172 ) ;
#10320=DIRECTION ( 'NONE',  ( 1.000000000000000000, 0.000000000000000000, -0.000000000000000000 ) ) ;
#10325=EDGE_CURVE ( 'NONE', #38882, #7516, #46794, .T. ) ;
#10329=EDGE_LOOP ( 'NONE', ( #37635, #17282, #14035, #18306, #43259, #13127 ) ) ;
#10330=CARTESIAN_POINT ( 'NONE',  ( 210.0000000000000568, 0.000000000000000000, 162.5682875569279702 ) ) ;
#10332=FACE_OUTER_BOUND ( 'NONE', #24987, .T. ) ;
#10335=CARTESIAN_POINT ( 'NONE',  ( 75.05402655318509630, 2.143131898507880377E-16, 165.0000000000000000 ) ) ;
#10338=ORIENTED_EDGE ( 'NONE', *, *, #24370, .F. ) ;
#10340=CARTESIAN_POINT ( 'NONE',  ( 72.27890028733797578, 1.750000000000009326, -158.1565861772249377 ) ) ;
#10345=ORIENTED_EDGE ( 'NONE', *, *, #2980, .T. ) ;
#10346=FACE_OUTER_BOUND ( 'NONE', #38478, .T. ) ;
#10348=CARTESIAN_POINT ( 'NONE',  ( 193.3040265531851105, 0.000000000000000000, 165.0000000000000000 ) ) ;
#10349=CARTESIAN_POINT ( 'NONE',  ( -168.4459734468149463, 0.000000000000000000, 165.0000000000000000 ) ) ;
#10350=CYLINDRICAL_SURFACE ( 'NONE', #37042, 1.750000000000008438 ) ;
#10352=EDGE_CURVE ( 'NONE', #29314, #5869, #12134, .T. ) ;
#10357=AXIS2_PLACEMENT_3D ( 'NONE', #10933, #42987, #30965 ) ;
#10358=DIRECTION ( 'NONE',  ( -1.000000000000000000, -0.000000000000000000, -0.000000000000000000 ) ) ;
#10359=CARTESIAN_POINT ( 'NONE',  ( -4.945973446814917018, -1.025126265847096763, 2.568287556927999926 ) ) ;
#10367=CARTESIAN_POINT ( 'NONE',  ( 33.30402655318503946, -1.750000000000010658, -79.18171244307201562 ) ) ;
#10368=CARTESIAN_POINT ( 'NONE',  ( -84.94597344681494633, 2.143131898507880377E-16, -37.43171244307205825 ) ) ;
#10371=CARTESIAN_POINT ( 'NONE',  ( 115.0540265531850395, 2.143131898507847836E-16, -157.4317124430720582 ) ) ;
#10372=VERTEX_POINT ( 'NONE', #43175 ) ;
#10376=ORIENTED_EDGE ( 'NONE', *, *, #17666, .F. ) ;
#10380=CARTESIAN_POINT ( 'NONE',  ( 210.0000000000000568, 2.143131898507881116E-16, 39.06828755692797728 ) ) ;
#10383=VERTEX_POINT ( 'NONE', #23672 ) ;
#10384=DIRECTION ( 'NONE',  ( -0.000000000000000000, -0.000000000000000000, -1.000000000000000000 ) ) ;
#10385=CYLINDRICAL_SURFACE ( 'NONE', #17434, 1.750000000000015543 ) ;
#10394=CARTESIAN_POINT ( 'NONE',  ( 151.5540265531850537, 0.000000000000000000, 119.0682875569279702 ) ) ;
#10395=DIRECTION ( 'NONE',  ( -1.000000000000000000, 0.000000000000000000, 0.000000000000000000 ) ) ;
#10396=CYLINDRICAL_SURFACE ( 'NONE', #5607, 1.750000000000008438 ) ;
#10408=CARTESIAN_POINT ( 'NONE',  ( -125.6708471809678542, -1.749999999999996669, 41.84341382277508359 ) ) ;
#10411=ORIENTED_EDGE ( 'NONE', *, *, #26811, .F. ) ;
#10414=AXIS2_PLACEMENT_3D ( 'NONE', #13645, #13387, #25197 ) ;
#10418=ORIENTED_EDGE ( 'NONE', *, *, #21596, .T. ) ;
#10420=VERTEX_POINT ( 'NONE', #35240 ) ;
#10421=CARTESIAN_POINT ( 'NONE',  ( -204.9459734468149463, 2.143131898507880377E-16, -37.43171244307205825 ) ) ;
#10424=( BOUNDED_CURVE ( )  B_SPLINE_CURVE ( 3, ( #1199, #35354, #47334, #16838 ),
 .UNSPECIFIED., .F., .F. ) 
 B_SPLINE_CURVE_WITH_KNOTS ( ( 4, 4 ),
 ( 4.712388980384689674, 6.283185307179586232 ),
 .UNSPECIFIED. ) 
 CURVE ( )  GEOMETRIC_REPRESENTATION_ITEM ( )  RATIONAL_B_SPLINE_CURVE ( ( 1.000000000000000000, 0.8047378541243649375, 0.8047378541243649375, 1.000000000000000000 ) ) 
 REPRESENTATION_ITEM ( '' )  );
#10431=EDGE_CURVE ( 'NONE', #18861, #7763, #7074, .T. ) ;
#10433=CARTESIAN_POINT ( 'NONE',  ( -4.945973446814903696, 2.143131898507912917E-16, -40.93171244307205825 ) ) ;
#10434=CARTESIAN_POINT ( 'NONE',  ( 151.5540265531850537, 0.000000000000000000, 119.0682875569279702 ) ) ;
#10436=CARTESIAN_POINT ( 'NONE',  ( 31.55402655318503236, 0.000000000000000000, 165.0000000000000000 ) ) ;
#10442=EDGE_CURVE ( 'NONE', #25305, #4914, #15672, .T. ) ;
#10444=CARTESIAN_POINT ( 'NONE',  ( -47.72109971266203132, 1.750000000000009548, -118.1565861772249519 ) ) ;
#10446=( BOUNDED_CURVE ( )  B_SPLINE_CURVE ( 3, ( #48368, #20448, #972, #39978 ),
 .UNSPECIFIED., .F., .F. ) 
 B_SPLINE_CURVE_WITH_KNOTS ( ( 4, 4 ),
 ( 1.570796326794896558, 3.141592653589793116 ),
 .UNSPECIFIED. ) 
 CURVE ( )  GEOMETRIC_REPRESENTATION_ITEM ( )  RATIONAL_B_SPLINE_CURVE ( ( 1.000000000000000000, 0.8047378541243649375, 0.8047378541243649375, 1.000000000000000000 ) ) 
 REPRESENTATION_ITEM ( '' )  );
#10454=CYLINDRICAL_SURFACE ( 'NONE', #436, 1.750000000000001554 ) ;
#10464=CARTESIAN_POINT ( 'NONE',  ( 113.3040265531850537, 1.749999999999996891, 160.8182875569279702 ) ) ;
#10467=CARTESIAN_POINT ( 'NONE',  ( -44.94597344681493922, 2.143131898507880377E-16, -40.93171244307205825 ) ) ;
#10470=LINE ( 'NONE', #22772, #26559 ) ;
#10477=LINE ( 'NONE', #31450, #226 ) ;
#10478=CARTESIAN_POINT ( 'NONE',  ( 31.55402655318503236, 0.000000000000000000, 2.568287556927978166 ) ) ;
#10479=EDGE_CURVE ( 'NONE', #41719, #25164, #2171, .T. ) ;
#10482=FACE_OUTER_BOUND ( 'NONE', #8908, .T. ) ;
#10483=DIRECTION ( 'NONE',  ( 0.000000000000000000, 0.000000000000000000, 1.000000000000000000 ) ) ;
#10484=ADVANCED_FACE ( 'NONE', ( #11879 ), #27538, .T. ) ;
#10491=EDGE_LOOP ( 'NONE', ( #7476, #37100, #24736, #22797, #46403 ) ) ;
#10494=LINE ( 'NONE', #25906, #17645 ) ;
#10495=ORIENTED_EDGE ( 'NONE', *, *, #25612, .T. ) ;
#10498=CARTESIAN_POINT ( 'NONE',  ( 112.2789002873379758, 1.749999999999997113, 79.79316129108087807 ) ) ;
#10500=CARTESIAN_POINT ( 'NONE',  ( 114.3291528190321173, 1.749999999999996891, 119.7931612910809065 ) ) ;
#10506=EDGE_CURVE ( 'NONE', #11997, #22181, #27823, .T. ) ;
#10507=DIRECTION ( 'NONE',  ( 1.000000000000000000, 0.000000000000000000, 0.000000000000000000 ) ) ;
#10509=FACE_OUTER_BOUND ( 'NONE', #4176, .T. ) ;
#10510=CARTESIAN_POINT ( 'NONE',  ( -204.9459734468148895, 1.025126265847089879, 82.56828755692798438 ) ) ;
#10513=EDGE_CURVE ( 'NONE', #42224, #14015, #47986, .T. ) ;
#10515=CARTESIAN_POINT ( 'NONE',  ( -4.945973446814903696, 2.143131898507912917E-16, 119.0682875569279418 ) ) ;
#10523=CARTESIAN_POINT ( 'NONE',  ( 35.05402655318504657, 2.143131898507880377E-16, -80.93171244307204404 ) ) ;
#10532=CARTESIAN_POINT ( 'NONE',  ( -126.6959734468149321, 0.000000000000000000, -165.0000000000000000 ) ) ;
#10538=CARTESIAN_POINT ( 'NONE',  ( 191.5540265531851105, 0.000000000000000000, 159.0682875569279702 ) ) ;
#10541=ADVANCED_FACE ( 'NONE', ( #13379 ), #8540, .T. ) ;
#10544=ORIENTED_EDGE ( 'NONE', *, *, #17490, .F. ) ;
#10545=CARTESIAN_POINT ( 'NONE',  ( 153.3040265531850537, 1.750000000000010658, -79.18171244307201562 ) ) ;
#10551=CARTESIAN_POINT ( 'NONE',  ( 210.0000000000000568, 0.000000000000000000, 162.5682875569279702 ) ) ;
#10552=AXIS2_PLACEMENT_3D ( 'NONE', #48464, #48712, #18201 ) ;
#10555=AXIS2_PLACEMENT_3D ( 'NONE', #1873, #37046, #28560 ) ;
#10565=CARTESIAN_POINT ( 'NONE',  ( -126.6959734468149321, 0.000000000000000000, 165.0000000000000000 ) ) ;
#10566=DIRECTION ( 'NONE',  ( -1.000000000000000000, -0.000000000000000000, -0.000000000000000000 ) ) ;
#10571=CARTESIAN_POINT ( 'NONE',  ( 71.55402655318505367, -1.025126265847089435, 39.06828755692797728 ) ) ;
#10582=( BOUNDED_CURVE ( )  B_SPLINE_CURVE ( 3, ( #14698, #45966, #18278, #26503 ),
 .UNSPECIFIED., .F., .F. ) 
 B_SPLINE_CURVE_WITH_KNOTS ( ( 4, 4 ),
 ( 1.570796326794896558, 3.141592653589793116 ),
 .UNSPECIFIED. ) 
 CURVE ( )  GEOMETRIC_REPRESENTATION_ITEM ( )  RATIONAL_B_SPLINE_CURVE ( ( 1.000000000000000000, 0.8047378541243649375, 0.8047378541243649375, 1.000000000000000000 ) ) 
 REPRESENTATION_ITEM ( '' )  );
#10585=ORIENTED_EDGE ( 'NONE', *, *, #23297, .T. ) ;
#10591=DIRECTION ( 'NONE',  ( 0.000000000000000000, 0.000000000000000000, -1.000000000000000000 ) ) ;
#10593=CARTESIAN_POINT ( 'NONE',  ( -164.9459734468149463, 2.143131898507880377E-16, 2.568287556927978166 ) ) ;
#10600=VERTEX_POINT ( 'NONE', #25698 ) ;
#10604=VERTEX_POINT ( 'NONE', #22598 ) ;
#10607=CARTESIAN_POINT ( 'NONE',  ( 210.0000000000000568, 0.000000000000000000, 0.8182875569279768335 ) ) ;
#10609=DIRECTION ( 'NONE',  ( -1.000000000000000000, 0.000000000000000000, 0.000000000000000000 ) ) ;
#10610=ORIENTED_EDGE ( 'NONE', *, *, #29275, .F. ) ;
#10614=ORIENTED_EDGE ( 'NONE', *, *, #7011, .F. ) ;
#10617=CARTESIAN_POINT ( 'NONE',  ( -208.4459734468149463, 0.000000000000000000, -157.4317124430720582 ) ) ;
#10618=ORIENTED_EDGE ( 'NONE', *, *, #30207, .F. ) ;
#10622=EDGE_CURVE ( 'NONE', #50239, #3325, #49034, .T. ) ;
#10625=ORIENTED_EDGE ( 'NONE', *, *, #35773, .T. ) ;
#10626=DIRECTION ( 'NONE',  ( -1.000000000000000000, 0.000000000000000000, 0.000000000000000000 ) ) ;
#10627=DIRECTION ( 'NONE',  ( 1.000000000000000000, 0.000000000000000000, 0.000000000000000000 ) ) ;
#10631=CARTESIAN_POINT ( 'NONE',  ( -206.6959734468149463, 0.000000000000000000, 165.0000000000000000 ) ) ;
#10632=EDGE_LOOP ( 'NONE', ( #45945, #21619 ) ) ;
#10633=CARTESIAN_POINT ( 'NONE',  ( 153.3040265531850537, -1.750000000000009992, -159.1817124430720298 ) ) ;
#10634=CIRCLE ( 'NONE', #32769, 1.750000000000015543 ) ;
#10636=CARTESIAN_POINT ( 'NONE',  ( -165.6708471809677974, -1.750000000000009548, 121.8434138227750623 ) ) ;
#10637=CARTESIAN_POINT ( 'NONE',  ( 210.0000000000000568, 0.000000000000000000, 122.5682875569279844 ) ) ;
#10642=CARTESIAN_POINT ( 'NONE',  ( 33.30402655318503946, -1.750000000000010658, -79.18171244307201562 ) ) ;
#10644=CARTESIAN_POINT ( 'NONE',  ( 111.5540265531850537, 2.143131898507880377E-16, -160.9317124430720298 ) ) ;
#10645=ADVANCED_FACE ( 'NONE', ( #45154 ), #45664, .T. ) ;
#10654=ORIENTED_EDGE ( 'NONE', *, *, #48394, .F. ) ;
#10655=ORIENTED_EDGE ( 'NONE', *, *, #45948, .T. ) ;
#10662=CARTESIAN_POINT ( 'NONE',  ( 191.5540265531850537, -1.025126265847089435, 2.568287556927986159 ) ) ;
#10664=AXIS2_PLACEMENT_3D ( 'NONE', #44002, #44753, #28376 ) ;
#10667=AXIS2_PLACEMENT_3D ( 'NONE', #25328, #41221, #41730 ) ;
#10669=VECTOR ( 'NONE', #35714, 1000.000000000000000 ) ;
#10678=EDGE_LOOP ( 'NONE', ( #7193, #39157, #24508, #46612, #9300, #47349 ) ) ;
#10679=ORIENTED_EDGE ( 'NONE', *, *, #45717, .T. ) ;
#10680=DIRECTION ( 'NONE',  ( -0.000000000000000000, -0.000000000000000000, -1.000000000000000000 ) ) ;
#10682=CARTESIAN_POINT ( 'NONE',  ( -47.72109971266203132, 1.750000000000009548, -40.20683870891912193 ) ) ;
#10685=EDGE_CURVE ( 'NONE', #32767, #19888, #10123, .T. ) ;
#10688=DIRECTION ( 'NONE',  ( -0.000000000000000000, -0.000000000000000000, -1.000000000000000000 ) ) ;
#10690=ORIENTED_EDGE ( 'NONE', *, *, #16557, .F. ) ;
#10692=CARTESIAN_POINT ( 'NONE',  ( -46.69597344681494633, 1.750000000000010658, -119.1817124430720440 ) ) ;
#10693=CARTESIAN_POINT ( 'NONE',  ( -167.7210997126620384, 1.750000000000009548, -0.2068387089191121020 ) ) ;
#10694=AXIS2_PLACEMENT_3D ( 'NONE', #34588, #27395, #50170 ) ;
#10695=CYLINDRICAL_SURFACE ( 'NONE', #46772, 1.750000000000008438 ) ;
#10699=DIRECTION ( 'NONE',  ( -1.000000000000000000, -0.000000000000000000, -0.000000000000000000 ) ) ;
#10705=FACE_OUTER_BOUND ( 'NONE', #35812, .T. ) ;
#10706=CYLINDRICAL_SURFACE ( 'NONE', #2426, 1.750000000000001554 ) ;
#10708=CARTESIAN_POINT ( 'NONE',  ( -48.44597344681495343, 0.000000000000000000, 39.06828755692798438 ) ) ;
#10713=CARTESIAN_POINT ( 'NONE',  ( 210.0000000000000568, 0.000000000000000000, 160.8182875569279702 ) ) ;
#10714=ORIENTED_EDGE ( 'NONE', *, *, #7810, .T. ) ;
#10715=ORIENTED_EDGE ( 'NONE', *, *, #18836, .T. ) ;
#10716=CARTESIAN_POINT ( 'NONE',  ( -6.695973446814940111, -1.750000000000024203, -119.1817124430720440 ) ) ;
#10717=( BOUNDED_CURVE ( )  B_SPLINE_CURVE ( 3, ( #10840, #6997, #329, #26752 ),
 .UNSPECIFIED., .F., .F. ) 
 B_SPLINE_CURVE_WITH_KNOTS ( ( 4, 4 ),
 ( 1.570796326794896558, 3.141592653589793116 ),
 .UNSPECIFIED. ) 
 CURVE ( )  GEOMETRIC_REPRESENTATION_ITEM ( )  RATIONAL_B_SPLINE_CURVE ( ( 1.000000000000000000, 0.8047378541243649375, 0.8047378541243649375, 1.000000000000000000 ) ) 
 REPRESENTATION_ITEM ( '' )  );
#10718=ORIENTED_EDGE ( 'NONE', *, *, #25802, .F. ) ;
#10722=CARTESIAN_POINT ( 'NONE',  ( -4.945973446814903696, 2.143131898507912917E-16, 119.0682875569279418 ) ) ;
#10723=( BOUNDED_CURVE ( )  B_SPLINE_CURVE ( 3, ( #12355, #31633, #13110, #24431 ),
 .UNSPECIFIED., .F., .F. ) 
 B_SPLINE_CURVE_WITH_KNOTS ( ( 4, 4 ),
 ( 0.000000000000000000, 1.570796326794896558 ),
 .UNSPECIFIED. ) 
 CURVE ( )  GEOMETRIC_REPRESENTATION_ITEM ( )  RATIONAL_B_SPLINE_CURVE ( ( 1.000000000000000000, 0.8047378541243649375, 0.8047378541243649375, 1.000000000000000000 ) ) 
 REPRESENTATION_ITEM ( '' )  );
#10727=DIRECTION ( 'NONE',  ( -1.000000000000000000, 0.000000000000000000, 0.000000000000000000 ) ) ;
#10729=CYLINDRICAL_SURFACE ( 'NONE', #16775, 1.750000000000008438 ) ;
#10730=ORIENTED_EDGE ( 'NONE', *, *, #50611, .T. ) ;
#10737=VECTOR ( 'NONE', #738, 1000.000000000000000 ) ;
#10741=EDGE_CURVE ( 'NONE', #30190, #11666, #35787, .T. ) ;
#10744=LINE ( 'NONE', #43567, #45197 ) ;
#10754=CARTESIAN_POINT ( 'NONE',  ( 71.55402655318505367, 0.000000000000000000, 165.0000000000000000 ) ) ;
#10763=FACE_OUTER_BOUND ( 'NONE', #21919, .T. ) ;
#10764=CARTESIAN_POINT ( 'NONE',  ( -86.69597344681494633, 1.750000000000009992, 160.8182875569279702 ) ) ;
#10768=CARTESIAN_POINT ( 'NONE',  ( -48.44597344681495343, 0.000000000000000000, 122.5682875569279702 ) ) ;
#10772=ORIENTED_EDGE ( 'NONE', *, *, #46373, .T. ) ;
#10774=ADVANCED_FACE ( 'NONE', ( #20010 ), #7206, .T. ) ;
#10776=AXIS2_PLACEMENT_3D ( 'NONE', #20813, #5163, #36240 ) ;
#10777=ORIENTED_EDGE ( 'NONE', *, *, #28205, .F. ) ;
#10782=CARTESIAN_POINT ( 'NONE',  ( 191.5540265531850537, -1.025126265847089879, 82.56828755692798438 ) ) ;
#10788=LINE ( 'NONE', #26438, #30832 ) ;
#10790=ORIENTED_EDGE ( 'NONE', *, *, #24617, .F. ) ;
#10798=AXIS2_PLACEMENT_3D ( 'NONE', #11321, #26217, #38544 ) ;
#10800=CARTESIAN_POINT ( 'NONE',  ( -207.7210997126620384, 1.750000000000009548, -78.15658617722490931 ) ) ;
#10802=ORIENTED_EDGE ( 'NONE', *, *, #42123, .T. ) ;
#10804=CARTESIAN_POINT ( 'NONE',  ( 35.05402655318504657, -1.025126265847088991, -157.4317124430720582 ) ) ;
#10805=CARTESIAN_POINT ( 'NONE',  ( 193.3040265531851105, 1.750000000000010658, 120.8182875569279702 ) ) ;
#10810=VECTOR ( 'NONE', #35732, 1000.000000000000000 ) ;
#10815=EDGE_CURVE ( 'NONE', #28808, #22009, #3515, .T. ) ;
#10817=ORIENTED_EDGE ( 'NONE', *, *, #21100, .T. ) ;
#10823=CYLINDRICAL_SURFACE ( 'NONE', #18478, 1.750000000000008438 ) ;
#10826=ORIENTED_EDGE ( 'NONE', *, *, #37488, .F. ) ;
#10830=EDGE_CURVE ( 'NONE', #45408, #33571, #15154, .T. ) ;
#10836=VERTEX_POINT ( 'NONE', #34933 ) ;
#10837=DIRECTION ( 'NONE',  ( 0.000000000000000000, 0.000000000000000000, 1.000000000000000000 ) ) ;
#10839=DIRECTION ( 'NONE',  ( -1.000000000000000000, -0.000000000000000000, -0.000000000000000000 ) ) ;
#10840=CARTESIAN_POINT ( 'NONE',  ( 193.3040265531851105, -1.750000000000009992, -159.1817124430720298 ) ) ;
#10841=VERTEX_POINT ( 'NONE', #31067 ) ;
#10847=LINE ( 'NONE', #11620, #1276 ) ;
#10849=VERTEX_POINT ( 'NONE', #27968 ) ;
#10854=EDGE_LOOP ( 'NONE', ( #36656, #31780, #33923, #26999, #2398, #49852 ) ) ;
#10855=CARTESIAN_POINT ( 'NONE',  ( 74.32915281903215998, -1.750000000000009548, 161.8434138227750907 ) ) ;
#10856=DIRECTION ( 'NONE',  ( -1.000000000000000000, -0.000000000000000000, -0.000000000000000000 ) ) ;
#10857=CARTESIAN_POINT ( 'NONE',  ( -164.9459734468149463, -1.025126265847088991, -157.4317124430720582 ) ) ;
#10859=VERTEX_POINT ( 'NONE', #1533 ) ;
#10882=CARTESIAN_POINT ( 'NONE',  ( 155.0540265531850537, 2.143131898507890731E-16, 165.0000000000000000 ) ) ;
#10887=CARTESIAN_POINT ( 'NONE',  ( 31.55402655318503236, 0.000000000000000000, -77.43171244307198720 ) ) ;
#10888=ORIENTED_EDGE ( 'NONE', *, *, #7021, .T. ) ;
#10889=CARTESIAN_POINT ( 'NONE',  ( 153.3040265531850537, -1.750000000000010658, 120.8182875569279702 ) ) ;
#10890=CARTESIAN_POINT ( 'NONE',  ( 154.3291528190321458, -1.750000000000009548, 161.8434138227750907 ) ) ;
#10891=EDGE_CURVE ( 'NONE', #20980, #7223, #48441, .T. ) ;
#10892=( BOUNDED_CURVE ( )  B_SPLINE_CURVE ( 3, ( #17747, #9289, #13872, #17245 ),
 .UNSPECIFIED., .F., .F. ) 
 B_SPLINE_CURVE_WITH_KNOTS ( ( 4, 4 ),
 ( 3.141592653589793116, 4.712388980384689674 ),
 .UNSPECIFIED. ) 
 CURVE ( )  GEOMETRIC_REPRESENTATION_ITEM ( )  RATIONAL_B_SPLINE_CURVE ( ( 1.000000000000000000, 0.8047378541243649375, 0.8047378541243649375, 1.000000000000000000 ) ) 
 REPRESENTATION_ITEM ( '' )  );
#10894=DIRECTION ( 'NONE',  ( 0.000000000000000000, 0.000000000000000000, 1.000000000000000000 ) ) ;
#10897=CARTESIAN_POINT ( 'NONE',  ( 153.3040265531850537, -1.750000000000009992, 0.8182875569279768335 ) ) ;
#10900=ORIENTED_EDGE ( 'NONE', *, *, #16846, .F. ) ;
#10906=VERTEX_POINT ( 'NONE', #4855 ) ;
#10911=CARTESIAN_POINT ( 'NONE',  ( 71.55402655318505367, -1.025126265847089657, 119.0682875569279560 ) ) ;
#10912=ORIENTED_EDGE ( 'NONE', *, *, #35665, .T. ) ;
#10914=ORIENTED_EDGE ( 'NONE', *, *, #21144, .F. ) ;
#10918=EDGE_LOOP ( 'NONE', ( #14148, #36766, #10544, #40916, #33946, #28719 ) ) ;
#10919=ORIENTED_EDGE ( 'NONE', *, *, #25664, .T. ) ;
#10928=CARTESIAN_POINT ( 'NONE',  ( 31.55402655318503236, -1.025126265847089879, 82.56828755692798438 ) ) ;
#10929=CARTESIAN_POINT ( 'NONE',  ( 31.55402655318503236, 0.000000000000000000, -37.43171244307200141 ) ) ;
#10931=EDGE_LOOP ( 'NONE', ( #49545, #30264, #10715, #5625, #16523, #7393 ) ) ;
#10933=CARTESIAN_POINT ( 'NONE',  ( 210.0000000000000568, 0.000000000000000000, -39.18171244307202983 ) ) ;
#10934=CARTESIAN_POINT ( 'NONE',  ( 151.5540265531850537, -1.025126265847089657, 119.0682875569279560 ) ) ;
#10941=ADVANCED_FACE ( 'NONE', ( #45345 ), #6628, .T. ) ;
#10943=CARTESIAN_POINT ( 'NONE',  ( -44.94597344681493922, 2.143131898507880377E-16, 165.0000000000000000 ) ) ;
#10945=CARTESIAN_POINT ( 'NONE',  ( -204.9459734468149463, 2.143131898507880377E-16, -77.43171244307204404 ) ) ;
#10946=ORIENTED_EDGE ( 'NONE', *, *, #6036, .F. ) ;
#10950=CARTESIAN_POINT ( 'NONE',  ( 113.3040265531850537, -1.749999999999996891, 0.8182875569279768335 ) ) ;
#10956=CARTESIAN_POINT ( 'NONE',  ( 155.0540265531850537, 2.143131898507880377E-16, -157.4317124430720582 ) ) ;
#10957=ORIENTED_EDGE ( 'NONE', *, *, #3765, .F. ) ;
#10962=CARTESIAN_POINT ( 'NONE',  ( -126.6959734468149321, 0.000000000000000000, 165.0000000000000000 ) ) ;
#10965=( BOUNDED_CURVE ( )  B_SPLINE_CURVE ( 3, ( #46035, #22725, #29667, #26580 ),
 .UNSPECIFIED., .F., .F. ) 
 B_SPLINE_CURVE_WITH_KNOTS ( ( 4, 4 ),
 ( 4.712388980384689674, 6.283185307179586232 ),
 .UNSPECIFIED. ) 
 CURVE ( )  GEOMETRIC_REPRESENTATION_ITEM ( )  RATIONAL_B_SPLINE_CURVE ( ( 1.000000000000000000, 0.8047378541243649375, 0.8047378541243649375, 1.000000000000000000 ) ) 
 REPRESENTATION_ITEM ( '' )  );
#10966=EDGE_LOOP ( 'NONE', ( #43301, #13050, #16203, #22838, #50684, #43431 ) ) ;
#10967=CARTESIAN_POINT ( 'NONE',  ( -84.94597344681494633, 2.143131898507880377E-16, -77.43171244307204404 ) ) ;
#10972=ORIENTED_EDGE ( 'NONE', *, *, #19516, .T. ) ;
#10977=DIRECTION ( 'NONE',  ( -0.000000000000000000, -0.000000000000000000, -1.000000000000000000 ) ) ;
#10989=CARTESIAN_POINT ( 'NONE',  ( -87.72109971266203843, 1.750000000000009548, 81.84341382277507648 ) ) ;
#10993=CARTESIAN_POINT ( 'NONE',  ( -6.695973446814940111, -1.750000000000024203, 80.81828755692798438 ) ) ;
#10995=EDGE_LOOP ( 'NONE', ( #43594, #20599, #24573, #46147, #36648, #42124 ) ) ;
#10997=ORIENTED_EDGE ( 'NONE', *, *, #12488, .T. ) ;
#10999=DIRECTION ( 'NONE',  ( 1.000000000000000000, 0.000000000000000000, 0.000000000000000000 ) ) ;
#11007=CARTESIAN_POINT ( 'NONE',  ( -88.44597344681494633, -1.025126265847089879, 82.56828755692798438 ) ) ;
#11018=ORIENTED_EDGE ( 'NONE', *, *, #15933, .F. ) ;
#11020=AXIS2_PLACEMENT_3D ( 'NONE', #21257, #36946, #1763 ) ;
#11027=( BOUNDED_CURVE ( )  B_SPLINE_CURVE ( 3, ( #38455, #33261, #15443, #40943 ),
 .UNSPECIFIED., .F., .F. ) 
 B_SPLINE_CURVE_WITH_KNOTS ( ( 4, 4 ),
 ( 1.570796326794896558, 3.141592653589793116 ),
 .UNSPECIFIED. ) 
 CURVE ( )  GEOMETRIC_REPRESENTATION_ITEM ( )  RATIONAL_B_SPLINE_CURVE ( ( 1.000000000000000000, 0.8047378541243649375, 0.8047378541243649375, 1.000000000000000000 ) ) 
 REPRESENTATION_ITEM ( '' )  );
#11028=EDGE_LOOP ( 'NONE', ( #25500, #21412, #23274, #13786, #15362, #15842 ) ) ;
#11034=CARTESIAN_POINT ( 'NONE',  ( 73.30402655318508209, -1.750000000000010214, -39.18171244307202983 ) ) ;
#11036=ORIENTED_EDGE ( 'NONE', *, *, #26643, .T. ) ;
#11037=DIRECTION ( 'NONE',  ( -1.000000000000000000, -0.000000000000000000, -0.000000000000000000 ) ) ;
#11039=VECTOR ( 'NONE', #7555, 1000.000000000000000 ) ;
#11041=CARTESIAN_POINT ( 'NONE',  ( 75.05402655318509630, 1.025126265847089879, -77.43171244307200141 ) ) ;
#11043=CIRCLE ( 'NONE', #49525, 1.750000000000001554 ) ;
#11051=CARTESIAN_POINT ( 'NONE',  ( 151.5540265531850537, 1.025126265847088991, 2.568287556927986159 ) ) ;
#11055=CARTESIAN_POINT ( 'NONE',  ( 115.0540265531850395, 2.143131898507847836E-16, 159.0682875569279702 ) ) ;
#11059=EDGE_LOOP ( 'NONE', ( #37773, #41139, #44429, #7001, #34543, #28666 ) ) ;
#11061=CARTESIAN_POINT ( 'NONE',  ( 155.0540265531850537, 1.025126265847089879, -117.4317124430720156 ) ) ;
#11069=ORIENTED_EDGE ( 'NONE', *, *, #5194, .F. ) ;
#11079=CARTESIAN_POINT ( 'NONE',  ( -8.445973446814976526, 0.000000000000000000, 165.0000000000000000 ) ) ;
#11088=EDGE_CURVE ( 'NONE', #40814, #2042, #1302, .T. ) ;
#11098=CARTESIAN_POINT ( 'NONE',  ( 115.0540265531850395, 1.025126265847081442, -0.9317124430720195027 ) ) ;
#11101=EDGE_LOOP ( 'NONE', ( #45921, #36318 ) ) ;
#11102=EDGE_CURVE ( 'NONE', #8469, #32098, #14323, .T. ) ;
#11104=CARTESIAN_POINT ( 'NONE',  ( -164.9459734468149463, -1.025126265847089657, -80.93171244307201562 ) ) ;
#11105=CARTESIAN_POINT ( 'NONE',  ( -125.6708471809678542, 1.749999999999996225, 161.8434138227750907 ) ) ;
#11118=CARTESIAN_POINT ( 'NONE',  ( 75.05402655318509630, 2.143131898507880377E-16, -0.9317124430720524764 ) ) ;
#11119=CARTESIAN_POINT ( 'NONE',  ( 191.5540265531851105, 0.000000000000000000, 39.06828755692798438 ) ) ;
#11124=VERTEX_POINT ( 'NONE', #3793 ) ;
#11131=EDGE_CURVE ( 'NONE', #9299, #25919, #8162, .T. ) ;
#11138=EDGE_CURVE ( 'NONE', #47505, #17018, #26638, .T. ) ;
#11139=CARTESIAN_POINT ( 'NONE',  ( -168.4459734468149747, 1.025126265847089657, -120.9317124430720440 ) ) ;
#11141=CARTESIAN_POINT ( 'NONE',  ( 34.32915281903212446, 1.750000000000010214, 121.8434138227750623 ) ) ;
#11152=CARTESIAN_POINT ( 'NONE',  ( 31.55402655318503236, 0.000000000000000000, 122.5682875569279702 ) ) ;
#11155=DIRECTION ( 'NONE',  ( 0.000000000000000000, 0.000000000000000000, 1.000000000000000000 ) ) ;
#11163=VECTOR ( 'NONE', #15992, 1000.000000000000000 ) ;
#11166=CARTESIAN_POINT ( 'NONE',  ( -88.44597344681497475, 0.000000000000000000, -117.4317124430720156 ) ) ;
#11167=DIRECTION ( 'NONE',  ( -1.000000000000000000, 0.000000000000000000, 0.000000000000000000 ) ) ;
#11168=ORIENTED_EDGE ( 'NONE', *, *, #38287, .F. ) ;
#11171=EDGE_CURVE ( 'NONE', #6144, #35686, #28120, .T. ) ;
#11172=CARTESIAN_POINT ( 'NONE',  ( 113.3040265531850537, 1.749999999999996891, -159.1817124430720298 ) ) ;
#11173=VECTOR ( 'NONE', #37234, 1000.000000000000000 ) ;
#11181=AXIS2_PLACEMENT_3D ( 'NONE', #44655, #32643, #44411 ) ;
#11184=( BOUNDED_CURVE ( )  B_SPLINE_CURVE ( 3, ( #29102, #45716, #49552, #5992 ),
 .UNSPECIFIED., .F., .F. ) 
 B_SPLINE_CURVE_WITH_KNOTS ( ( 4, 4 ),
 ( 1.570796326794896558, 3.141592653589793116 ),
 .UNSPECIFIED. ) 
 CURVE ( )  GEOMETRIC_REPRESENTATION_ITEM ( )  RATIONAL_B_SPLINE_CURVE ( ( 1.000000000000000000, 0.8047378541243649375, 0.8047378541243649375, 1.000000000000000000 ) ) 
 REPRESENTATION_ITEM ( '' )  );
#11188=CARTESIAN_POINT ( 'NONE',  ( 210.0000000000000568, 0.000000000000000000, 160.8182875569279702 ) ) ;
#11190=VERTEX_POINT ( 'NONE', #48112 ) ;
#11191=ORIENTED_EDGE ( 'NONE', *, *, #34594, .F. ) ;
#11195=VERTEX_POINT ( 'NONE', #12756 ) ;
#11196=DIRECTION ( 'NONE',  ( -1.000000000000000000, -0.000000000000000000, -0.000000000000000000 ) ) ;
#11197=AXIS2_PLACEMENT_3D ( 'NONE', #39981, #23816, #36132 ) ;
#11198=EDGE_CURVE ( 'NONE', #17256, #5743, #31428, .T. ) ;
#11199=DIRECTION ( 'NONE',  ( 0.000000000000000000, 0.000000000000000000, 1.000000000000000000 ) ) ;
#11205=CARTESIAN_POINT ( 'NONE',  ( -208.4459734468148611, 1.025126265847088991, 162.5682875569279133 ) ) ;
#11206=( BOUNDED_CURVE ( )  B_SPLINE_CURVE ( 3, ( #43312, #11775, #15375, #8183 ),
 .UNSPECIFIED., .F., .F. ) 
 B_SPLINE_CURVE_WITH_KNOTS ( ( 4, 4 ),
 ( 4.712388980384689674, 6.283185307179586232 ),
 .UNSPECIFIED. ) 
 CURVE ( )  GEOMETRIC_REPRESENTATION_ITEM ( )  RATIONAL_B_SPLINE_CURVE ( ( 1.000000000000000000, 0.8047378541243649375, 0.8047378541243649375, 1.000000000000000000 ) ) 
 REPRESENTATION_ITEM ( '' )  );
#11212=CARTESIAN_POINT ( 'NONE',  ( 193.3040265531851105, 0.000000000000000000, 165.0000000000000000 ) ) ;
#11218=DIRECTION ( 'NONE',  ( -0.000000000000000000, -0.000000000000000000, -1.000000000000000000 ) ) ;
#11221=AXIS2_PLACEMENT_3D ( 'NONE', #32272, #35628, #466 ) ;
#11222=DIRECTION ( 'NONE',  ( -0.000000000000000000, -0.000000000000000000, -1.000000000000000000 ) ) ;
#11226=CARTESIAN_POINT ( 'NONE',  ( 31.55402655318503236, -1.025126265847089657, 79.06828755692797017 ) ) ;
#11229=ADVANCED_FACE ( 'NONE', ( #36651 ), #20207, .T. ) ;
#11235=CARTESIAN_POINT ( 'NONE',  ( -124.9459734468149463, 2.143131898507847836E-16, 122.5682875569279560 ) ) ;
#11238=EDGE_CURVE ( 'NONE', #14892, #4637, #23808, .T. ) ;
#11241=ORIENTED_EDGE ( 'NONE', *, *, #24293, .F. ) ;
#11244=LINE ( 'NONE', #26631, #30378 ) ;
#11247=CYLINDRICAL_SURFACE ( 'NONE', #3288, 1.750000000000001554 ) ;
#11248=CARTESIAN_POINT ( 'NONE',  ( 210.0000000000000568, 2.143131898507890731E-16, 159.0682875569279702 ) ) ;
#11255=ORIENTED_EDGE ( 'NONE', *, *, #30061, .T. ) ;
#11267=CARTESIAN_POINT ( 'NONE',  ( -128.4459734468149463, 1.025126265847081886, 119.0682875569279702 ) ) ;
#11279=LINE ( 'NONE', #45877, #29816 ) ;
#11281=ORIENTED_EDGE ( 'NONE', *, *, #42546, .F. ) ;
#11291=EDGE_LOOP ( 'NONE', ( #38732, #23193, #40320, #47664, #7383, #45127 ) ) ;
#11294=VERTEX_POINT ( 'NONE', #36385 ) ;
#11295=ORIENTED_EDGE ( 'NONE', *, *, #36336, .F. ) ;
#11299=CARTESIAN_POINT ( 'NONE',  ( -84.94597344681493212, 1.025126265847089657, -37.43171244307202272 ) ) ;
#11300=CARTESIAN_POINT ( 'NONE',  ( 191.5540265531851105, 0.000000000000000000, 162.5682875569279702 ) ) ;
#11304=ADVANCED_FACE ( 'NONE', ( #40213 ), #39721, .T. ) ;
#11305=CARTESIAN_POINT ( 'NONE',  ( -8.445973446814976526, 0.000000000000000000, -80.93171244307204404 ) ) ;
#11310=ORIENTED_EDGE ( 'NONE', *, *, #49595, .T. ) ;
#11318=CARTESIAN_POINT ( 'NONE',  ( 191.5540265531851105, 2.143131898507880377E-16, -160.9317124430720298 ) ) ;
#11319=CARTESIAN_POINT ( 'NONE',  ( 73.30402655318508209, 1.750000000000009992, 160.8182875569279702 ) ) ;
#11321=CARTESIAN_POINT ( 'NONE',  ( 210.0000000000000568, 0.000000000000000000, 0.8182875569279768335 ) ) ;
#11324=CARTESIAN_POINT ( 'NONE',  ( 112.2789002873379758, -1.749999999999996669, 1.843413822775057609 ) ) ;
#11325=CARTESIAN_POINT ( 'NONE',  ( -128.4459734468149179, 2.143131898507880377E-16, -160.9317124430720298 ) ) ;
#11330=CARTESIAN_POINT ( 'NONE',  ( -168.4459734468149463, 0.000000000000000000, 165.0000000000000000 ) ) ;
#11331=( BOUNDED_CURVE ( )  B_SPLINE_CURVE ( 3, ( #48632, #25588, #16887, #44303 ),
 .UNSPECIFIED., .F., .F. ) 
 B_SPLINE_CURVE_WITH_KNOTS ( ( 4, 4 ),
 ( 1.570796326794896558, 3.141592653589793116 ),
 .UNSPECIFIED. ) 
 CURVE ( )  GEOMETRIC_REPRESENTATION_ITEM ( )  RATIONAL_B_SPLINE_CURVE ( ( 1.000000000000000000, 0.8047378541243649375, 0.8047378541243649375, 1.000000000000000000 ) ) 
 REPRESENTATION_ITEM ( '' )  );
#11336=CARTESIAN_POINT ( 'NONE',  ( 32.27890028733795447, 1.750000000000009548, -40.20683870891912193 ) ) ;
#11339=( BOUNDED_CURVE ( )  B_SPLINE_CURVE ( 3, ( #17418, #33086, #9713, #36438 ),
 .UNSPECIFIED., .F., .F. ) 
 B_SPLINE_CURVE_WITH_KNOTS ( ( 4, 4 ),
 ( 0.000000000000000000, 1.570796326794896558 ),
 .UNSPECIFIED. ) 
 CURVE ( )  GEOMETRIC_REPRESENTATION_ITEM ( )  RATIONAL_B_SPLINE_CURVE ( ( 1.000000000000000000, 0.8047378541243649375, 0.8047378541243649375, 1.000000000000000000 ) ) 
 REPRESENTATION_ITEM ( '' )  );
#11343=VERTEX_POINT ( 'NONE', #16869 ) ;
#11344=CARTESIAN_POINT ( 'NONE',  ( 71.55402655318505367, 0.000000000000000000, 159.0682875569279702 ) ) ;
#11348=CARTESIAN_POINT ( 'NONE',  ( 210.0000000000000568, 0.000000000000000000, 42.56828755692799149 ) ) ;
#11349=DIRECTION ( 'NONE',  ( 0.000000000000000000, 0.000000000000000000, 1.000000000000000000 ) ) ;
#11355=FACE_OUTER_BOUND ( 'NONE', #21072, .T. ) ;
#11357=EDGE_CURVE ( 'NONE', #11761, #4874, #28165, .T. ) ;
#11359=ORIENTED_EDGE ( 'NONE', *, *, #39646, .T. ) ;
#11364=ORIENTED_EDGE ( 'NONE', *, *, #19964, .T. ) ;
#11365=CARTESIAN_POINT ( 'NONE',  ( -44.94597344681493922, 2.143131898507880377E-16, -77.43171244307198720 ) ) ;
#11367=CARTESIAN_POINT ( 'NONE',  ( 35.05402655318504657, 2.143131898507880377E-16, 39.06828755692798438 ) ) ;
#11373=AXIS2_PLACEMENT_3D ( 'NONE', #48760, #37294, #10320 ) ;
#11389=ORIENTED_EDGE ( 'NONE', *, *, #47410, .T. ) ;
#11390=ADVANCED_FACE ( 'NONE', ( #41663 ), #42155, .T. ) ;
#11391=LINE ( 'NONE', #3945, #44867 ) ;
#11392=CARTESIAN_POINT ( 'NONE',  ( -8.445973446814976526, 0.000000000000000000, 119.0682875569279418 ) ) ;
#11398=CARTESIAN_POINT ( 'NONE',  ( 155.0540265531850537, -1.025126265847089657, 119.0682875569279560 ) ) ;
#11404=CARTESIAN_POINT ( 'NONE',  ( 194.3291528190321742, -1.750000000000010436, 79.79316129108087807 ) ) ;
#11405=VECTOR ( 'NONE', #27990, 1000.000000000000000 ) ;
#11416=CYLINDRICAL_SURFACE ( 'NONE', #32804, 1.750000000000008438 ) ;
#11420=ORIENTED_EDGE ( 'NONE', *, *, #8105, .T. ) ;
#11427=ORIENTED_EDGE ( 'NONE', *, *, #32148, .F. ) ;
#11434=AXIS2_PLACEMENT_3D ( 'NONE', #28473, #5867, #1773 ) ;
#11435=CARTESIAN_POINT ( 'NONE',  ( 112.2789002873379758, -1.749999999999996669, -38.15658617722495194 ) ) ;
#11439=VECTOR ( 'NONE', #3126, 1000.000000000000000 ) ;
#11441=CARTESIAN_POINT ( 'NONE',  ( 155.0540265531850537, 2.143131898507880377E-16, 165.0000000000000000 ) ) ;
#11442=CARTESIAN_POINT ( 'NONE',  ( 111.5540265531850679, 0.000000000000000000, -117.4317124430720725 ) ) ;
#11443=ORIENTED_EDGE ( 'NONE', *, *, #40636, .T. ) ;
#11444=EDGE_CURVE ( 'NONE', #6332, #17123, #8495, .T. ) ;
#11445=ORIENTED_EDGE ( 'NONE', *, *, #11890, .F. ) ;
#11451=CARTESIAN_POINT ( 'NONE',  ( 151.5540265531850537, 1.025126265847089657, -120.9317124430720440 ) ) ;
#11453=ADVANCED_FACE ( 'NONE', ( #2652 ), #33970, .T. ) ;
#11455=CARTESIAN_POINT ( 'NONE',  ( 71.55402655318505367, 0.000000000000000000, -157.4317124430720014 ) ) ;
#11459=ORIENTED_EDGE ( 'NONE', *, *, #4252, .F. ) ;
#11463=CYLINDRICAL_SURFACE ( 'NONE', #10107, 1.750000000000001554 ) ;
#11465=DIRECTION ( 'NONE',  ( -0.000000000000000000, -0.000000000000000000, -1.000000000000000000 ) ) ;
#11466=ORIENTED_EDGE ( 'NONE', *, *, #50322, .F. ) ;
#11467=CYLINDRICAL_SURFACE ( 'NONE', #787, 1.750000000000015543 ) ;
#11472=( BOUNDED_CURVE ( )  B_SPLINE_CURVE ( 3, ( #31245, #42751, #49907, #18903 ),
 .UNSPECIFIED., .F., .F. ) 
 B_SPLINE_CURVE_WITH_KNOTS ( ( 4, 4 ),
 ( 1.570796326794896558, 3.141592653589793116 ),
 .UNSPECIFIED. ) 
 CURVE ( )  GEOMETRIC_REPRESENTATION_ITEM ( )  RATIONAL_B_SPLINE_CURVE ( ( 1.000000000000000000, 0.8047378541243649375, 0.8047378541243649375, 1.000000000000000000 ) ) 
 REPRESENTATION_ITEM ( '' )  );
#11473=VERTEX_POINT ( 'NONE', #23683 ) ;
#11474=CARTESIAN_POINT ( 'NONE',  ( -4.945973446814903696, 2.143131898507912917E-16, 159.0682875569279418 ) ) ;
#11476=CARTESIAN_POINT ( 'NONE',  ( -126.6959734468149321, 1.749999999999997113, -39.18171244307202983 ) ) ;
#11483=( BOUNDED_CURVE ( )  B_SPLINE_CURVE ( 3, ( #29550, #42358, #14139, #18241 ),
 .UNSPECIFIED., .F., .F. ) 
 B_SPLINE_CURVE_WITH_KNOTS ( ( 4, 4 ),
 ( 3.141592653589793116, 4.712388980384689674 ),
 .UNSPECIFIED. ) 
 CURVE ( )  GEOMETRIC_REPRESENTATION_ITEM ( )  RATIONAL_B_SPLINE_CURVE ( ( 1.000000000000000000, 0.8047378541243649375, 0.8047378541243649375, 1.000000000000000000 ) ) 
 REPRESENTATION_ITEM ( '' )  );
#11484=VECTOR ( 'NONE', #20283, 1000.000000000000000 ) ;
#11488=VERTEX_POINT ( 'NONE', #27284 ) ;
#11490=CYLINDRICAL_SURFACE ( 'NONE', #10694, 1.750000000000008438 ) ;
#11494=DIRECTION ( 'NONE',  ( 0.000000000000000000, 0.000000000000000000, 1.000000000000000000 ) ) ;
#11498=DIRECTION ( 'NONE',  ( -0.000000000000000000, -0.000000000000000000, -1.000000000000000000 ) ) ;
#11504=CYLINDRICAL_SURFACE ( 'NONE', #4677, 1.750000000000008438 ) ;
#11509=ORIENTED_EDGE ( 'NONE', *, *, #36233, .T. ) ;
#11513=AXIS2_PLACEMENT_3D ( 'NONE', #4289, #35610, #17093 ) ;
#11524=LINE ( 'NONE', #42803, #39062 ) ;
#11527=VECTOR ( 'NONE', #19391, 1000.000000000000000 ) ;
#11529=FACE_OUTER_BOUND ( 'NONE', #26711, .T. ) ;
#11533=EDGE_CURVE ( 'NONE', #46777, #12549, #4872, .T. ) ;
#11534=EDGE_CURVE ( 'NONE', #26183, #35621, #851, .T. ) ;
#11536=CARTESIAN_POINT ( 'NONE',  ( 210.0000000000000568, 0.000000000000000000, 40.81828755692798438 ) ) ;
#11537=CARTESIAN_POINT ( 'NONE',  ( -88.44597344681494633, -1.025126265847089213, -0.9317124430720324924 ) ) ;
#11538=ORIENTED_EDGE ( 'NONE', *, *, #26445, .T. ) ;
#11540=FACE_OUTER_BOUND ( 'NONE', #41201, .T. ) ;
#11543=FACE_OUTER_BOUND ( 'NONE', #34422, .T. ) ;
#11549=ORIENTED_EDGE ( 'NONE', *, *, #31539, .F. ) ;
#11554=ORIENTED_EDGE ( 'NONE', *, *, #49299, .T. ) ;
#11556=VECTOR ( 'NONE', #47979, 1000.000000000000000 ) ;
#11564=ORIENTED_EDGE ( 'NONE', *, *, #17707, .F. ) ;
#11567=EDGE_CURVE ( 'NONE', #47489, #15143, #35502, .T. ) ;
#11569=ORIENTED_EDGE ( 'NONE', *, *, #11766, .T. ) ;
#11573=LINE ( 'NONE', #33109, #42563 ) ;
#11583=( BOUNDED_CURVE ( )  B_SPLINE_CURVE ( 3, ( #47384, #4342, #39501, #741 ),
 .UNSPECIFIED., .F., .F. ) 
 B_SPLINE_CURVE_WITH_KNOTS ( ( 4, 4 ),
 ( 4.712388980384689674, 6.283185307179586232 ),
 .UNSPECIFIED. ) 
 CURVE ( )  GEOMETRIC_REPRESENTATION_ITEM ( )  RATIONAL_B_SPLINE_CURVE ( ( 1.000000000000000000, 0.8047378541243649375, 0.8047378541243649375, 1.000000000000000000 ) ) 
 REPRESENTATION_ITEM ( '' )  );
#11589=ORIENTED_EDGE ( 'NONE', *, *, #42773, .F. ) ;
#11590=EDGE_CURVE ( 'NONE', #48199, #42713, #29758, .T. ) ;
#11596=EDGE_LOOP ( 'NONE', ( #16940, #15100, #32530, #5356, #27897, #5139 ) ) ;
#11599=CARTESIAN_POINT ( 'NONE',  ( 193.3040265531851105, -1.750000000000010658, 120.8182875569279702 ) ) ;
#11602=CIRCLE ( 'NONE', #9974, 1.750000000000008438 ) ;
#11603=DIRECTION ( 'NONE',  ( 0.000000000000000000, 0.000000000000000000, 1.000000000000000000 ) ) ;
#11607=FACE_OUTER_BOUND ( 'NONE', #47098, .T. ) ;
#11610=CARTESIAN_POINT ( 'NONE',  ( -88.44597344681491791, 2.143131898507880377E-16, -160.9317124430720298 ) ) ;
#11612=CARTESIAN_POINT ( 'NONE',  ( -8.445973446814914354, 0.000000000000000000, 162.5682875569279702 ) ) ;
#11615=PLANE ( 'NONE',  #27074 ) ;
#11616=ORIENTED_EDGE ( 'NONE', *, *, #26864, .F. ) ;
#11618=CARTESIAN_POINT ( 'NONE',  ( 34.32915281903212446, 1.750000000000010214, 81.84341382277507648 ) ) ;
#11620=CARTESIAN_POINT ( 'NONE',  ( 31.55402655318503236, 0.000000000000000000, 165.0000000000000000 ) ) ;
#11628=AXIS2_PLACEMENT_3D ( 'NONE', #28823, #44444, #9322 ) ;
#11629=DIRECTION ( 'NONE',  ( -1.000000000000000000, -0.000000000000000000, -0.000000000000000000 ) ) ;
#11636=CARTESIAN_POINT ( 'NONE',  ( -126.6959734468149321, -1.749999999999997113, -39.18171244307202983 ) ) ;
#11637=( BOUNDED_CURVE ( )  B_SPLINE_CURVE ( 3, ( #30023, #41055, #29254, #49210 ),
 .UNSPECIFIED., .F., .F. ) 
 B_SPLINE_CURVE_WITH_KNOTS ( ( 4, 4 ),
 ( 1.570796326794896558, 3.141592653589793116 ),
 .UNSPECIFIED. ) 
 CURVE ( )  GEOMETRIC_REPRESENTATION_ITEM ( )  RATIONAL_B_SPLINE_CURVE ( ( 1.000000000000000000, 0.8047378541243649375, 0.8047378541243649375, 1.000000000000000000 ) ) 
 REPRESENTATION_ITEM ( '' )  );
#11639=VERTEX_POINT ( 'NONE', #24704 ) ;
#11642=CYLINDRICAL_SURFACE ( 'NONE', #34520, 1.750000000000015543 ) ;
#11644=( BOUNDED_CURVE ( )  B_SPLINE_CURVE ( 3, ( #1436, #44498, #4764, #28122 ),
 .UNSPECIFIED., .F., .F. ) 
 B_SPLINE_CURVE_WITH_KNOTS ( ( 4, 4 ),
 ( 4.712388980384689674, 6.283185307179586232 ),
 .UNSPECIFIED. ) 
 CURVE ( )  GEOMETRIC_REPRESENTATION_ITEM ( )  RATIONAL_B_SPLINE_CURVE ( ( 1.000000000000000000, 0.8047378541243649375, 0.8047378541243649375, 1.000000000000000000 ) ) 
 REPRESENTATION_ITEM ( '' )  );
#11647=CARTESIAN_POINT ( 'NONE',  ( 195.0540265531851105, 2.143131898507880377E-16, 39.06828755692798438 ) ) ;
#11651=DIRECTION ( 'NONE',  ( -0.000000000000000000, -0.000000000000000000, -1.000000000000000000 ) ) ;
#11666=VERTEX_POINT ( 'NONE', #9292 ) ;
#11670=CARTESIAN_POINT ( 'NONE',  ( 114.3291528190321173, -1.749999999999996669, -160.2068387089191219 ) ) ;
#11672=VECTOR ( 'NONE', #25764, 1000.000000000000000 ) ;
#11673=ORIENTED_EDGE ( 'NONE', *, *, #29003, .F. ) ;
#11675=CARTESIAN_POINT ( 'NONE',  ( -86.69597344681496054, 0.000000000000000000, 165.0000000000000000 ) ) ;
#11679=CARTESIAN_POINT ( 'NONE',  ( 194.3291528190321742, -1.750000000000009326, -158.1565861772249377 ) ) ;
#11680=CARTESIAN_POINT ( 'NONE',  ( -126.6959734468149321, -1.749999999999996891, -159.1817124430720298 ) ) ;
#11683=VECTOR ( 'NONE', #12457, 1000.000000000000000 ) ;
#11693=CYLINDRICAL_SURFACE ( 'NONE', #13479, 1.749999999999987566 ) ;
#11694=CARTESIAN_POINT ( 'NONE',  ( 113.3040265531850537, 1.749999999999997335, -119.1817124430720440 ) ) ;
#11698=CARTESIAN_POINT ( 'NONE',  ( -207.7210997126620384, 1.750000000000009326, 161.8434138227750907 ) ) ;
#11701=ORIENTED_EDGE ( 'NONE', *, *, #34184, .T. ) ;
#11705=ORIENTED_EDGE ( 'NONE', *, *, #22067, .F. ) ;
#11706=DIRECTION ( 'NONE',  ( 1.000000000000000000, 0.000000000000000000, -0.000000000000000000 ) ) ;
#11711=EDGE_LOOP ( 'NONE', ( #47855, #4087, #15393, #45401, #48375, #15700 ) ) ;
#11717=CARTESIAN_POINT ( 'NONE',  ( -46.69597344681494633, 0.000000000000000000, 165.0000000000000000 ) ) ;
#11719=ORIENTED_EDGE ( 'NONE', *, *, #12666, .T. ) ;
#11720=DIRECTION ( 'NONE',  ( 0.000000000000000000, 0.000000000000000000, 1.000000000000000000 ) ) ;
#11729=CARTESIAN_POINT ( 'NONE',  ( 73.30402655318508209, -1.750000000000009992, 0.8182875569279768335 ) ) ;
#11730=ORIENTED_EDGE ( 'NONE', *, *, #47843, .F. ) ;
#11734=DIRECTION ( 'NONE',  ( -0.000000000000000000, -0.000000000000000000, -1.000000000000000000 ) ) ;
#11739=ADVANCED_FACE ( 'NONE', ( #28797 ), #24952, .T. ) ;
#11740=VERTEX_POINT ( 'NONE', #40600 ) ;
#11750=EDGE_CURVE ( 'NONE', #47505, #7355, #13720, .T. ) ;
#11751=DIRECTION ( 'NONE',  ( -0.000000000000000000, -0.000000000000000000, -1.000000000000000000 ) ) ;
#11761=VERTEX_POINT ( 'NONE', #3094 ) ;
#11763=AXIS2_PLACEMENT_3D ( 'NONE', #35347, #39689, #28129 ) ;
#11766=EDGE_CURVE ( 'NONE', #41541, #20063, #25861, .T. ) ;
#11770=EDGE_CURVE ( 'NONE', #14892, #50433, #10634, .T. ) ;
#11771=CARTESIAN_POINT ( 'NONE',  ( -128.4459734468149463, 1.025126265847081219, -157.4317124430720582 ) ) ;
#11774=DIRECTION ( 'NONE',  ( -1.000000000000000000, -0.000000000000000000, -0.000000000000000000 ) ) ;
#11775=CARTESIAN_POINT ( 'NONE',  ( -207.7210997126620384, 1.750000000000009548, 39.79316129108089228 ) ) ;
#11780=ORIENTED_EDGE ( 'NONE', *, *, #41446, .T. ) ;
#11781=CARTESIAN_POINT ( 'NONE',  ( 210.0000000000000568, 0.000000000000000000, 82.56828755692799859 ) ) ;
#11782=( BOUNDED_CURVE ( )  B_SPLINE_CURVE ( 3, ( #21428, #45259, #17335, #13482 ),
 .UNSPECIFIED., .F., .F. ) 
 B_SPLINE_CURVE_WITH_KNOTS ( ( 4, 4 ),
 ( 1.570796326794896558, 3.141592653589793116 ),
 .UNSPECIFIED. ) 
 CURVE ( )  GEOMETRIC_REPRESENTATION_ITEM ( )  RATIONAL_B_SPLINE_CURVE ( ( 1.000000000000000000, 0.8047378541243649375, 0.8047378541243649375, 1.000000000000000000 ) ) 
 REPRESENTATION_ITEM ( '' )  );
#11786=CARTESIAN_POINT ( 'NONE',  ( -210.0000000000000568, 0.000000000000000000, 160.8182875569279702 ) ) ;
#11787=EDGE_LOOP ( 'NONE', ( #37573, #42010, #7245, #32965, #35867, #44418 ) ) ;
#11789=( BOUNDED_CURVE ( )  B_SPLINE_CURVE ( 3, ( #14987, #38862, #50076, #3685 ),
 .UNSPECIFIED., .F., .F. ) 
 B_SPLINE_CURVE_WITH_KNOTS ( ( 4, 4 ),
 ( 1.570796326794896558, 3.141592653589793116 ),
 .UNSPECIFIED. ) 
 CURVE ( )  GEOMETRIC_REPRESENTATION_ITEM ( )  RATIONAL_B_SPLINE_CURVE ( ( 1.000000000000000000, 0.8047378541243649375, 0.8047378541243649375, 1.000000000000000000 ) ) 
 REPRESENTATION_ITEM ( '' )  );
#11800=DIRECTION ( 'NONE',  ( -1.000000000000000000, -0.000000000000000000, -0.000000000000000000 ) ) ;
#11801=AXIS2_PLACEMENT_3D ( 'NONE', #31038, #10507, #46632 ) ;
#11803=( BOUNDED_CURVE ( )  B_SPLINE_CURVE ( 3, ( #36663, #5570, #982, #5827 ),
 .UNSPECIFIED., .F., .F. ) 
 B_SPLINE_CURVE_WITH_KNOTS ( ( 4, 4 ),
 ( 4.712388980384689674, 6.283185307179586232 ),
 .UNSPECIFIED. ) 
 CURVE ( )  GEOMETRIC_REPRESENTATION_ITEM ( )  RATIONAL_B_SPLINE_CURVE ( ( 1.000000000000000000, 0.8047378541243649375, 0.8047378541243649375, 1.000000000000000000 ) ) 
 REPRESENTATION_ITEM ( '' )  );
#11804=ORIENTED_EDGE ( 'NONE', *, *, #36530, .F. ) ;
#11805=DIRECTION ( 'NONE',  ( -1.000000000000000000, -0.000000000000000000, -0.000000000000000000 ) ) ;
#11810=EDGE_CURVE ( 'NONE', #43432, #41850, #33914, .T. ) ;
#11812=CARTESIAN_POINT ( 'NONE',  ( 72.27890028733797578, -1.750000000000009548, 161.8434138227750907 ) ) ;
#11813=CARTESIAN_POINT ( 'NONE',  ( -6.695973446814940111, -1.750000000000023315, 160.8182875569279702 ) ) ;
#11821=EDGE_CURVE ( 'NONE', #33571, #32944, #14008, .T. ) ;
#11824=ORIENTED_EDGE ( 'NONE', *, *, #19223, .F. ) ;
#11826=DIRECTION ( 'NONE',  ( -0.000000000000000000, -0.000000000000000000, -1.000000000000000000 ) ) ;
#11834=CARTESIAN_POINT ( 'NONE',  ( 73.30402655318508209, -1.750000000000010658, -79.18171244307201562 ) ) ;
#11835=EDGE_CURVE ( 'NONE', #44684, #29600, #17022, .T. ) ;
#11840=AXIS2_PLACEMENT_3D ( 'NONE', #19294, #10839, #34210 ) ;
#11841=CARTESIAN_POINT ( 'NONE',  ( 75.05402655318509630, 1.025126265847089657, 79.06828755692797017 ) ) ;
#11845=CARTESIAN_POINT ( 'NONE',  ( -86.69597344681496054, 0.000000000000000000, -165.0000000000000000 ) ) ;
#11849=( BOUNDED_CURVE ( )  B_SPLINE_CURVE ( 3, ( #35208, #7744, #39301, #34697 ),
 .UNSPECIFIED., .F., .F. ) 
 B_SPLINE_CURVE_WITH_KNOTS ( ( 4, 4 ),
 ( 4.712388980384689674, 6.283185307179586232 ),
 .UNSPECIFIED. ) 
 CURVE ( )  GEOMETRIC_REPRESENTATION_ITEM ( )  RATIONAL_B_SPLINE_CURVE ( ( 1.000000000000000000, 0.8047378541243649375, 0.8047378541243649375, 1.000000000000000000 ) ) 
 REPRESENTATION_ITEM ( '' )  );
#11851=ORIENTED_EDGE ( 'NONE', *, *, #5106, .F. ) ;
#11855=ORIENTED_EDGE ( 'NONE', *, *, #16786, .F. ) ;
#11856=CIRCLE ( 'NONE', #48678, 1.750000000000001554 ) ;
#11857=DIRECTION ( 'NONE',  ( 1.000000000000000000, 0.000000000000000000, -0.000000000000000000 ) ) ;
#11872=AXIS2_PLACEMENT_3D ( 'NONE', #36583, #8602, #16550 ) ;
#11875=CARTESIAN_POINT ( 'NONE',  ( -204.9459734468149463, 2.143131898507880377E-16, -0.9317124430720247208 ) ) ;
#11879=FACE_OUTER_BOUND ( 'NONE', #13245, .T. ) ;
#11881=EDGE_CURVE ( 'NONE', #26878, #41657, #26958, .T. ) ;
#11884=CARTESIAN_POINT ( 'NONE',  ( -164.9459734468149463, 2.143131898507880377E-16, 39.06828755692798438 ) ) ;
#11885=CARTESIAN_POINT ( 'NONE',  ( 31.55402655318503236, 0.000000000000000000, 165.0000000000000000 ) ) ;
#11886=( BOUNDED_CURVE ( )  B_SPLINE_CURVE ( 3, ( #39117, #11141, #15249, #14726 ),
 .UNSPECIFIED., .F., .F. ) 
 B_SPLINE_CURVE_WITH_KNOTS ( ( 4, 4 ),
 ( 1.570796326794896558, 3.141592653589793116 ),
 .UNSPECIFIED. ) 
 CURVE ( )  GEOMETRIC_REPRESENTATION_ITEM ( )  RATIONAL_B_SPLINE_CURVE ( ( 1.000000000000000000, 0.8047378541243649375, 0.8047378541243649375, 1.000000000000000000 ) ) 
 REPRESENTATION_ITEM ( '' )  );
#11889=EDGE_LOOP ( 'NONE', ( #48669, #17921, #3906, #28103, #8555, #6966 ) ) ;
#11890=EDGE_CURVE ( 'NONE', #34485, #14566, #20621, .T. ) ;
#11895=ORIENTED_EDGE ( 'NONE', *, *, #7214, .T. ) ;
#11898=CIRCLE ( 'NONE', #36487, 1.750000000000015543 ) ;
#11904=ORIENTED_EDGE ( 'NONE', *, *, #19967, .F. ) ;
#11905=FACE_OUTER_BOUND ( 'NONE', #34844, .T. ) ;
#11906=EDGE_LOOP ( 'NONE', ( #31769, #27455, #15439, #8808, #15851 ) ) ;
#11908=CARTESIAN_POINT ( 'NONE',  ( -48.44597344681496054, -1.025126265847089879, 82.56828755692798438 ) ) ;
#11916=ORIENTED_EDGE ( 'NONE', *, *, #35597, .F. ) ;
#11927=DIRECTION ( 'NONE',  ( 0.000000000000000000, 0.000000000000000000, 1.000000000000000000 ) ) ;
#11940=( BOUNDED_CURVE ( )  B_SPLINE_CURVE ( 3, ( #46301, #6834, #6580, #21975 ),
 .UNSPECIFIED., .F., .F. ) 
 B_SPLINE_CURVE_WITH_KNOTS ( ( 4, 4 ),
 ( 1.570796326794896558, 3.141592653589793116 ),
 .UNSPECIFIED. ) 
 CURVE ( )  GEOMETRIC_REPRESENTATION_ITEM ( )  RATIONAL_B_SPLINE_CURVE ( ( 1.000000000000000000, 0.8047378541243649375, 0.8047378541243649375, 1.000000000000000000 ) ) 
 REPRESENTATION_ITEM ( '' )  );
#11942=ORIENTED_EDGE ( 'NONE', *, *, #31827, .F. ) ;
#11943=ORIENTED_EDGE ( 'NONE', *, *, #41215, .T. ) ;
#11944=CARTESIAN_POINT ( 'NONE',  ( -125.6708471809678542, -1.749999999999996891, 39.79316129108089228 ) ) ;
#11946=DIRECTION ( 'NONE',  ( -1.000000000000000000, 0.000000000000000000, 0.000000000000000000 ) ) ;
#11951=ADVANCED_FACE ( 'NONE', ( #31596 ), #12080, .T. ) ;
#11953=( BOUNDED_CURVE ( )  B_SPLINE_CURVE ( 3, ( #12777, #48383, #36407, #35897 ),
 .UNSPECIFIED., .F., .F. ) 
 B_SPLINE_CURVE_WITH_KNOTS ( ( 4, 4 ),
 ( 1.570796326794896558, 3.141592653589793116 ),
 .UNSPECIFIED. ) 
 CURVE ( )  GEOMETRIC_REPRESENTATION_ITEM ( )  RATIONAL_B_SPLINE_CURVE ( ( 1.000000000000000000, 0.8047378541243649375, 0.8047378541243649375, 1.000000000000000000 ) ) 
 REPRESENTATION_ITEM ( '' )  );
#11956=ORIENTED_EDGE ( 'NONE', *, *, #7420, .F. ) ;
#11958=CARTESIAN_POINT ( 'NONE',  ( 115.0540265531850395, 2.143131898507847836E-16, -40.93171244307202983 ) ) ;
#11961=ORIENTED_EDGE ( 'NONE', *, *, #39339, .T. ) ;
#11963=CARTESIAN_POINT ( 'NONE',  ( -206.6959734468149463, 1.750000000000009992, 160.8182875569279702 ) ) ;
#11965=VERTEX_POINT ( 'NONE', #46924 ) ;
#11966=ORIENTED_EDGE ( 'NONE', *, *, #15701, .T. ) ;
#11971=DIRECTION ( 'NONE',  ( -0.000000000000000000, -0.000000000000000000, -1.000000000000000000 ) ) ;
#11972=DIRECTION ( 'NONE',  ( -1.000000000000000000, 0.000000000000000000, 0.000000000000000000 ) ) ;
#11974=CARTESIAN_POINT ( 'NONE',  ( 35.05402655318504657, 2.143131898507880377E-16, 165.0000000000000000 ) ) ;
#11988=LINE ( 'NONE', #31753, #42045 ) ;
#11991=CARTESIAN_POINT ( 'NONE',  ( 155.0540265531850537, 2.143131898507880377E-16, -40.93171244307202983 ) ) ;
#11993=CARTESIAN_POINT ( 'NONE',  ( -84.94597344681494633, 2.143131898507880377E-16, 82.56828755692798438 ) ) ;
#11994=ORIENTED_EDGE ( 'NONE', *, *, #17078, .T. ) ;
#11995=DIRECTION ( 'NONE',  ( -0.000000000000000000, -0.000000000000000000, -1.000000000000000000 ) ) ;
#11997=VERTEX_POINT ( 'NONE', #20019 ) ;
#12000=VECTOR ( 'NONE', #34742, 1000.000000000000000 ) ;
#12001=CIRCLE ( 'NONE', #47988, 1.750000000000015543 ) ;
#12003=LINE ( 'NONE', #31007, #32802 ) ;
#12004=CARTESIAN_POINT ( 'NONE',  ( -48.44597344681495343, 0.000000000000000000, -40.93171244307205825 ) ) ;
#12008=ORIENTED_EDGE ( 'NONE', *, *, #17207, .F. ) ;
#12010=DIRECTION ( 'NONE',  ( -1.000000000000000000, -0.000000000000000000, -0.000000000000000000 ) ) ;
#12012=AXIS2_PLACEMENT_3D ( 'NONE', #12319, #50513, #784 ) ;
#12014=DIRECTION ( 'NONE',  ( -0.000000000000000000, -0.000000000000000000, -1.000000000000000000 ) ) ;
#12018=ORIENTED_EDGE ( 'NONE', *, *, #49620, .F. ) ;
#12020=CARTESIAN_POINT ( 'NONE',  ( 75.05402655318509630, 2.143131898507880377E-16, -37.43171244307200141 ) ) ;
#12028=EDGE_CURVE ( 'NONE', #8778, #39465, #31122, .T. ) ;
#12030=CARTESIAN_POINT ( 'NONE',  ( 31.55402655318503236, -1.025126265847089657, -80.93171244307201562 ) ) ;
#12031=CARTESIAN_POINT ( 'NONE',  ( -86.69597344681494633, -1.750000000000009992, 160.8182875569279702 ) ) ;
#12035=CARTESIAN_POINT ( 'NONE',  ( 192.2789002873380184, 1.750000000000009548, -38.15658617722494483 ) ) ;
#12036=DIRECTION ( 'NONE',  ( -1.000000000000000000, 0.000000000000000000, 0.000000000000000000 ) ) ;
#12038=CARTESIAN_POINT ( 'NONE',  ( -46.69597344681494633, -1.750000000000009992, 160.8182875569279702 ) ) ;
#12040=CARTESIAN_POINT ( 'NONE',  ( -205.6708471809678827, -1.750000000000009548, -118.1565861772249519 ) ) ;
#12042=EDGE_CURVE ( 'NONE', #4637, #38939, #11573, .T. ) ;
#12049=DIRECTION ( 'NONE',  ( 1.000000000000000000, 0.000000000000000000, -0.000000000000000000 ) ) ;
#12050=CARTESIAN_POINT ( 'NONE',  ( 33.30402655318503946, 1.750000000000010658, -79.18171244307201562 ) ) ;
#12052=CYLINDRICAL_SURFACE ( 'NONE', #15789, 1.750000000000001554 ) ;
#12057=CARTESIAN_POINT ( 'NONE',  ( 210.0000000000000568, 0.000000000000000000, 0.8182875569279768335 ) ) ;
#12062=EDGE_CURVE ( 'NONE', #12549, #38939, #38015, .T. ) ;
#12066=CARTESIAN_POINT ( 'NONE',  ( -204.9459734468149463, 2.143131898507880377E-16, 39.06828755692798438 ) ) ;
#12073=EDGE_CURVE ( 'NONE', #17197, #13383, #43239, .T. ) ;
#12077=LINE ( 'NONE', #27722, #50439 ) ;
#12078=DIRECTION ( 'NONE',  ( 1.000000000000000000, 0.000000000000000000, 0.000000000000000000 ) ) ;
#12079=VERTEX_POINT ( 'NONE', #44855 ) ;
#12080=CYLINDRICAL_SURFACE ( 'NONE', #1641, 1.750000000000008438 ) ;
#12084=DIRECTION ( 'NONE',  ( -0.000000000000000000, -0.000000000000000000, -1.000000000000000000 ) ) ;
#12085=CARTESIAN_POINT ( 'NONE',  ( 151.5540265531850537, 0.000000000000000000, -157.4317124430720582 ) ) ;
#12087=CARTESIAN_POINT ( 'NONE',  ( 193.3040265531851105, 1.750000000000010214, 40.81828755692798438 ) ) ;
#12090=CYLINDRICAL_SURFACE ( 'NONE', #36820, 1.750000000000015543 ) ;
#12092=( BOUNDED_CURVE ( )  B_SPLINE_CURVE ( 3, ( #4148, #54, #47456, #20297 ),
 .UNSPECIFIED., .F., .F. ) 
 B_SPLINE_CURVE_WITH_KNOTS ( ( 4, 4 ),
 ( 1.570796326794896558, 3.141592653589793116 ),
 .UNSPECIFIED. ) 
 CURVE ( )  GEOMETRIC_REPRESENTATION_ITEM ( )  RATIONAL_B_SPLINE_CURVE ( ( 1.000000000000000000, 0.8047378541243649375, 0.8047378541243649375, 1.000000000000000000 ) ) 
 REPRESENTATION_ITEM ( '' )  );
#12095=ORIENTED_EDGE ( 'NONE', *, *, #30895, .T. ) ;
#12108=( BOUNDED_CURVE ( )  B_SPLINE_CURVE ( 3, ( #7225, #45930, #2846, #14412 ),
 .UNSPECIFIED., .F., .F. ) 
 B_SPLINE_CURVE_WITH_KNOTS ( ( 4, 4 ),
 ( 1.570796326794896558, 3.141592653589793116 ),
 .UNSPECIFIED. ) 
 CURVE ( )  GEOMETRIC_REPRESENTATION_ITEM ( )  RATIONAL_B_SPLINE_CURVE ( ( 1.000000000000000000, 0.8047378541243649375, 0.8047378541243649375, 1.000000000000000000 ) ) 
 REPRESENTATION_ITEM ( '' )  );
#12109=CARTESIAN_POINT ( 'NONE',  ( -46.69597344681494633, -1.750000000000010214, 40.81828755692798438 ) ) ;
#12110=CYLINDRICAL_SURFACE ( 'NONE', #42167, 1.750000000000010214 ) ;
#12111=DIRECTION ( 'NONE',  ( -1.000000000000000000, 0.000000000000000000, 0.000000000000000000 ) ) ;
#12112=EDGE_CURVE ( 'NONE', #19110, #11639, #5626, .T. ) ;
#12113=ORIENTED_EDGE ( 'NONE', *, *, #29275, .T. ) ;
#12119=CARTESIAN_POINT ( 'NONE',  ( -208.4459734468149463, 0.000000000000000000, 159.0682875569279702 ) ) ;
#12120=CARTESIAN_POINT ( 'NONE',  ( -210.0000000000000568, 0.000000000000000000, -39.18171244307202983 ) ) ;
#12123=CARTESIAN_POINT ( 'NONE',  ( -165.6708471809677974, -1.750000000000010436, -80.20683870891910772 ) ) ;
#12124=ADVANCED_FACE ( 'NONE', ( #32855 ), #9728, .T. ) ;
#12125=CARTESIAN_POINT ( 'NONE',  ( 151.5540265531850537, 1.025126265847089435, -77.43171244307200141 ) ) ;
#12129=LINE ( 'NONE', #27774, #44250 ) ;
#12132=EDGE_LOOP ( 'NONE', ( #40590, #12113, #26433, #28424, #43043, #33286 ) ) ;
#12134=LINE ( 'NONE', #8287, #17732 ) ;
#12135=ORIENTED_EDGE ( 'NONE', *, *, #40276, .F. ) ;
#12136=CARTESIAN_POINT ( 'NONE',  ( 192.2789002873380184, 1.750000000000009548, -78.15658617722490931 ) ) ;
#12138=CARTESIAN_POINT ( 'NONE',  ( 210.0000000000000568, 0.000000000000000000, -159.1817124430720298 ) ) ;
#12146=EDGE_LOOP ( 'NONE', ( #47141, #8661, #39195, #9095, #31528 ) ) ;
#12147=CIRCLE ( 'NONE', #20341, 1.750000000000001554 ) ;
#12154=ORIENTED_EDGE ( 'NONE', *, *, #49194, .F. ) ;
#12161=CARTESIAN_POINT ( 'NONE',  ( 33.30402655318503946, 0.000000000000000000, 165.0000000000000000 ) ) ;
#12163=ORIENTED_EDGE ( 'NONE', *, *, #45596, .T. ) ;
#12165=CARTESIAN_POINT ( 'NONE',  ( -204.9459734468149463, 2.143131898507880377E-16, 159.0682875569279702 ) ) ;
#12169=FACE_OUTER_BOUND ( 'NONE', #30701, .T. ) ;
#12176=EDGE_CURVE ( 'NONE', #29610, #49500, #36685, .T. ) ;
#12185=DIRECTION ( 'NONE',  ( -1.000000000000000000, -0.000000000000000000, -0.000000000000000000 ) ) ;
#12188=EDGE_LOOP ( 'NONE', ( #27948, #32644, #47740, #31346, #12018, #29269 ) ) ;
#12189=DIRECTION ( 'NONE',  ( -0.000000000000000000, -0.000000000000000000, -1.000000000000000000 ) ) ;
#12193=CARTESIAN_POINT ( 'NONE',  ( 72.27890028733797578, 1.750000000000010436, 119.7931612910808781 ) ) ;
#12199=ORIENTED_EDGE ( 'NONE', *, *, #12648, .F. ) ;
#12201=ORIENTED_EDGE ( 'NONE', *, *, #30487, .T. ) ;
#12203=CARTESIAN_POINT ( 'NONE',  ( 191.5540265531850537, 1.025126265847089435, -117.4317124430720156 ) ) ;
#12207=CARTESIAN_POINT ( 'NONE',  ( -166.6959734468149463, 1.750000000000010658, -79.18171244307201562 ) ) ;
#12211=CARTESIAN_POINT ( 'NONE',  ( -46.69597344681494633, 1.750000000000010658, 120.8182875569279702 ) ) ;
#12213=AXIS2_PLACEMENT_3D ( 'NONE', #37055, #1881, #17525 ) ;
#12214=EDGE_CURVE ( 'NONE', #32429, #43783, #18180, .T. ) ;
#12215=FACE_OUTER_BOUND ( 'NONE', #33019, .T. ) ;
#12220=CARTESIAN_POINT ( 'NONE',  ( -206.6959734468149463, 0.000000000000000000, 165.0000000000000000 ) ) ;
#12222=EDGE_CURVE ( 'NONE', #9233, #36841, #49447, .T. ) ;
#12229=VERTEX_POINT ( 'NONE', #30249 ) ;
#12235=( BOUNDED_CURVE ( )  B_SPLINE_CURVE ( 3, ( #43609, #20769, #17917, #33349 ),
 .UNSPECIFIED., .F., .F. ) 
 B_SPLINE_CURVE_WITH_KNOTS ( ( 4, 4 ),
 ( 4.712388980384689674, 6.283185307179586232 ),
 .UNSPECIFIED. ) 
 CURVE ( )  GEOMETRIC_REPRESENTATION_ITEM ( )  RATIONAL_B_SPLINE_CURVE ( ( 1.000000000000000000, 0.8047378541243649375, 0.8047378541243649375, 1.000000000000000000 ) ) 
 REPRESENTATION_ITEM ( '' )  );
#12241=CARTESIAN_POINT ( 'NONE',  ( -4.945973446814903696, 2.143131898507912917E-16, 165.0000000000000000 ) ) ;
#12243=VECTOR ( 'NONE', #41887, 1000.000000000000000 ) ;
#12254=CARTESIAN_POINT ( 'NONE',  ( -84.94597344681493212, -1.025126265847089657, -120.9317124430720440 ) ) ;
#12255=CARTESIAN_POINT ( 'NONE',  ( 115.0540265531850395, 2.143131898507847836E-16, 159.0682875569279702 ) ) ;
#12262=EDGE_LOOP ( 'NONE', ( #16607, #7848, #21845, #27651, #42861, #43104 ) ) ;
#12263=ORIENTED_EDGE ( 'NONE', *, *, #25852, .F. ) ;
#12264=CARTESIAN_POINT ( 'NONE',  ( -8.445973446814962315, -1.025126265847096985, 159.0682875569279418 ) ) ;
#12266=EDGE_LOOP ( 'NONE', ( #5500, #29529, #14429, #20643, #8668 ) ) ;
#12270=CARTESIAN_POINT ( 'NONE',  ( -46.69597344681494633, 1.750000000000010214, 40.81828755692798438 ) ) ;
#12281=CARTESIAN_POINT ( 'NONE',  ( 71.55402655318505367, 0.000000000000000000, 165.0000000000000000 ) ) ;
#12282=ORIENTED_EDGE ( 'NONE', *, *, #34345, .T. ) ;
#12284=VECTOR ( 'NONE', #3036, 1000.000000000000000 ) ;
#12287=CARTESIAN_POINT ( 'NONE',  ( -88.44597344681494633, 1.025126265847088991, 2.568287556927986159 ) ) ;
#12288=DIRECTION ( 'NONE',  ( -1.000000000000000000, -0.000000000000000000, -0.000000000000000000 ) ) ;
#12291=CARTESIAN_POINT ( 'NONE',  ( -6.695973446814940111, 1.750000000000024203, 120.8182875569279702 ) ) ;
#12292=CARTESIAN_POINT ( 'NONE',  ( -128.4459734468149179, 0.000000000000000000, 39.06828755692801280 ) ) ;
#12294=DIRECTION ( 'NONE',  ( -1.000000000000000000, -0.000000000000000000, -0.000000000000000000 ) ) ;
#12297=ORIENTED_EDGE ( 'NONE', *, *, #4698, .F. ) ;
#12306=CARTESIAN_POINT ( 'NONE',  ( 115.0540265531850395, 1.025126265847082108, -77.43171244307201562 ) ) ;
#12307=DIRECTION ( 'NONE',  ( 0.000000000000000000, 0.000000000000000000, -1.000000000000000000 ) ) ;
#12315=CARTESIAN_POINT ( 'NONE',  ( -128.4459734468149463, -1.025126265847081886, -80.93171244307201562 ) ) ;
#12318=VECTOR ( 'NONE', #43246, 1000.000000000000000 ) ;
#12319=CARTESIAN_POINT ( 'NONE',  ( -166.6959734468149463, 0.000000000000000000, 165.0000000000000000 ) ) ;
#12322=CARTESIAN_POINT ( 'NONE',  ( -44.94597344681493922, 2.143131898507880377E-16, 79.06828755692797017 ) ) ;
#12329=CARTESIAN_POINT ( 'NONE',  ( 73.30402655318508209, 1.750000000000010658, 80.81828755692798438 ) ) ;
#12331=ORIENTED_EDGE ( 'NONE', *, *, #5582, .F. ) ;
#12333=DIRECTION ( 'NONE',  ( 1.000000000000000000, 0.000000000000000000, 0.000000000000000000 ) ) ;
#12342=CARTESIAN_POINT ( 'NONE',  ( 115.0540265531850395, 1.025126265847081886, -40.93171244307202272 ) ) ;
#12350=CARTESIAN_POINT ( 'NONE',  ( 31.55402655318503236, 0.000000000000000000, -80.93171244307204404 ) ) ;
#12351=ORIENTED_EDGE ( 'NONE', *, *, #16338, .T. ) ;
#12355=CARTESIAN_POINT ( 'NONE',  ( -84.94597344681494633, 2.143131898507880377E-16, 39.06828755692798438 ) ) ;
#12356=CARTESIAN_POINT ( 'NONE',  ( -124.9459734468149463, 2.143131898507847836E-16, -77.43171244307204404 ) ) ;
#12357=ORIENTED_EDGE ( 'NONE', *, *, #31517, .T. ) ;
#12358=CARTESIAN_POINT ( 'NONE',  ( -124.9459734468149463, 2.143131898507847836E-16, -0.9317124430719969652 ) ) ;
#12360=ORIENTED_EDGE ( 'NONE', *, *, #1470, .T. ) ;
#12365=VERTEX_POINT ( 'NONE', #12020 ) ;
#12372=( BOUNDED_CURVE ( )  B_SPLINE_CURVE ( 3, ( #20124, #39142, #7574, #39398 ),
 .UNSPECIFIED., .F., .F. ) 
 B_SPLINE_CURVE_WITH_KNOTS ( ( 4, 4 ),
 ( 4.712388980384689674, 6.283185307179586232 ),
 .UNSPECIFIED. ) 
 CURVE ( )  GEOMETRIC_REPRESENTATION_ITEM ( )  RATIONAL_B_SPLINE_CURVE ( ( 1.000000000000000000, 0.8047378541243649375, 0.8047378541243649375, 1.000000000000000000 ) ) 
 REPRESENTATION_ITEM ( '' )  );
#12374=ADVANCED_FACE ( 'NONE', ( #42539 ), #15102, .T. ) ;
#12376=CYLINDRICAL_SURFACE ( 'NONE', #1222, 1.750000000000008438 ) ;
#12382=( BOUNDED_CURVE ( )  B_SPLINE_CURVE ( 3, ( #44942, #49026, #9823, #6242 ),
 .UNSPECIFIED., .F., .F. ) 
 B_SPLINE_CURVE_WITH_KNOTS ( ( 4, 4 ),
 ( 3.141592653589793116, 4.712388980384689674 ),
 .UNSPECIFIED. ) 
 CURVE ( )  GEOMETRIC_REPRESENTATION_ITEM ( )  RATIONAL_B_SPLINE_CURVE ( ( 1.000000000000000000, 0.8047378541243649375, 0.8047378541243649375, 1.000000000000000000 ) ) 
 REPRESENTATION_ITEM ( '' )  );
#12392=( BOUNDED_CURVE ( )  B_SPLINE_CURVE ( 3, ( #35404, #7682, #3557, #4339 ),
 .UNSPECIFIED., .F., .F. ) 
 B_SPLINE_CURVE_WITH_KNOTS ( ( 4, 4 ),
 ( 1.570796326794896558, 3.141592653589793116 ),
 .UNSPECIFIED. ) 
 CURVE ( )  GEOMETRIC_REPRESENTATION_ITEM ( )  RATIONAL_B_SPLINE_CURVE ( ( 1.000000000000000000, 0.8047378541243649375, 0.8047378541243649375, 1.000000000000000000 ) ) 
 REPRESENTATION_ITEM ( '' )  );
#12394=ORIENTED_EDGE ( 'NONE', *, *, #2602, .T. ) ;
#12401=CARTESIAN_POINT ( 'NONE',  ( -128.4459734468149179, 0.000000000000000000, 39.06828755692801280 ) ) ;
#12402=CARTESIAN_POINT ( 'NONE',  ( -84.94597344681494633, 2.143131898507880377E-16, 119.0682875569279702 ) ) ;
#12411=DIRECTION ( 'NONE',  ( -0.000000000000000000, -0.000000000000000000, -1.000000000000000000 ) ) ;
#12418=CARTESIAN_POINT ( 'NONE',  ( 195.0540265531851105, -1.025126265847089213, -160.9317124430720014 ) ) ;
#12425=ORIENTED_EDGE ( 'NONE', *, *, #44165, .T. ) ;
#12429=CARTESIAN_POINT ( 'NONE',  ( -47.72109971266203132, 1.750000000000009326, -158.1565861772249377 ) ) ;
#12431=EDGE_CURVE ( 'NONE', #4734, #30864, #4321, .T. ) ;
#12435=DIRECTION ( 'NONE',  ( -0.000000000000000000, -0.000000000000000000, -1.000000000000000000 ) ) ;
#12436=CARTESIAN_POINT ( 'NONE',  ( -206.6959734468149463, -1.750000000000010214, 40.81828755692798438 ) ) ;
#12437=CARTESIAN_POINT ( 'NONE',  ( 71.55402655318505367, 1.025126265847089657, 119.0682875569279560 ) ) ;
#12438=VERTEX_POINT ( 'NONE', #7929 ) ;
#12442=EDGE_CURVE ( 'NONE', #49361, #40327, #31112, .T. ) ;
#12457=DIRECTION ( 'NONE',  ( -1.000000000000000000, -0.000000000000000000, -0.000000000000000000 ) ) ;
#12458=ORIENTED_EDGE ( 'NONE', *, *, #20221, .T. ) ;
#12467=CARTESIAN_POINT ( 'NONE',  ( 155.0540265531850537, 2.143131898507880377E-16, 122.5682875569279702 ) ) ;
#12469=CARTESIAN_POINT ( 'NONE',  ( 210.0000000000000568, 0.000000000000000000, -159.1817124430720298 ) ) ;
#12471=CARTESIAN_POINT ( 'NONE',  ( -164.9459734468149463, 1.025126265847088991, 162.5682875569279133 ) ) ;
#12473=EDGE_LOOP ( 'NONE', ( #17167, #20280, #39150, #34773, #26833, #3058 ) ) ;
#12475=CARTESIAN_POINT ( 'NONE',  ( 193.3040265531851105, -1.750000000000009992, 160.8182875569279702 ) ) ;
#12480=FACE_OUTER_BOUND ( 'NONE', #11059, .T. ) ;
#12488=EDGE_CURVE ( 'NONE', #3794, #20580, #38322, .T. ) ;
#12495=ADVANCED_FACE ( 'NONE', ( #24830 ), #47878, .T. ) ;
#12506=ORIENTED_EDGE ( 'NONE', *, *, #33479, .T. ) ;
#12508=ORIENTED_EDGE ( 'NONE', *, *, #38535, .F. ) ;
#12513=VERTEX_POINT ( 'NONE', #32543 ) ;
#12527=DIRECTION ( 'NONE',  ( 0.000000000000000000, 0.000000000000000000, 1.000000000000000000 ) ) ;
#12528=VECTOR ( 'NONE', #5712, 1000.000000000000000 ) ;
#12531=ORIENTED_EDGE ( 'NONE', *, *, #32860, .F. ) ;
#12532=LINE ( 'NONE', #28455, #4049 ) ;
#12538=EDGE_CURVE ( 'NONE', #40406, #37272, #45155, .T. ) ;
#12540=DIRECTION ( 'NONE',  ( 0.000000000000000000, 0.000000000000000000, -1.000000000000000000 ) ) ;
#12542=ORIENTED_EDGE ( 'NONE', *, *, #49464, .F. ) ;
#12544=CARTESIAN_POINT ( 'NONE',  ( -126.6959734468149321, 1.749999999999997113, 40.81828755692798438 ) ) ;
#12547=DIRECTION ( 'NONE',  ( -1.000000000000000000, 0.000000000000000000, 0.000000000000000000 ) ) ;
#12549=VERTEX_POINT ( 'NONE', #43559 ) ;
#12564=CARTESIAN_POINT ( 'NONE',  ( -128.4459734468149179, 0.000000000000000000, -80.93171244307201562 ) ) ;
#12574=CARTESIAN_POINT ( 'NONE',  ( 210.0000000000000568, 0.000000000000000000, 80.81828755692798438 ) ) ;
#12576=VERTEX_POINT ( 'NONE', #16366 ) ;
#12577=CARTESIAN_POINT ( 'NONE',  ( 210.0000000000000568, 0.000000000000000000, 80.81828755692798438 ) ) ;
#12585=CARTESIAN_POINT ( 'NONE',  ( -126.6959734468149321, 0.000000000000000000, 165.0000000000000000 ) ) ;
#12587=CARTESIAN_POINT ( 'NONE',  ( 191.5540265531851105, 0.000000000000000000, 42.56828755692798438 ) ) ;
#12590=DIRECTION ( 'NONE',  ( -0.000000000000000000, -0.000000000000000000, -1.000000000000000000 ) ) ;
#12593=DIRECTION ( 'NONE',  ( 0.000000000000000000, 0.000000000000000000, 1.000000000000000000 ) ) ;
#12599=CARTESIAN_POINT ( 'NONE',  ( 153.3040265531850537, 1.750000000000010214, -39.18171244307202983 ) ) ;
#12600=ORIENTED_EDGE ( 'NONE', *, *, #5388, .T. ) ;
#12606=FACE_OUTER_BOUND ( 'NONE', #42519, .T. ) ;
#12607=ORIENTED_EDGE ( 'NONE', *, *, #7627, .F. ) ;
#12609=DIRECTION ( 'NONE',  ( 0.000000000000000000, 0.000000000000000000, 1.000000000000000000 ) ) ;
#12613=CARTESIAN_POINT ( 'NONE',  ( -4.945973446814917018, 1.025126265847096985, -160.9317124430720014 ) ) ;
#12614=( BOUNDED_CURVE ( )  B_SPLINE_CURVE ( 3, ( #37202, #1527, #28721, #44580 ),
 .UNSPECIFIED., .F., .F. ) 
 B_SPLINE_CURVE_WITH_KNOTS ( ( 4, 4 ),
 ( 4.712388980384689674, 6.283185307179586232 ),
 .UNSPECIFIED. ) 
 CURVE ( )  GEOMETRIC_REPRESENTATION_ITEM ( )  RATIONAL_B_SPLINE_CURVE ( ( 1.000000000000000000, 0.8047378541243649375, 0.8047378541243649375, 1.000000000000000000 ) ) 
 REPRESENTATION_ITEM ( '' )  );
#12621=DIRECTION ( 'NONE',  ( -1.000000000000000000, 0.000000000000000000, 0.000000000000000000 ) ) ;
#12622=CARTESIAN_POINT ( 'NONE',  ( -87.72109971266203843, -1.750000000000009548, 41.84341382277508359 ) ) ;
#12625=DIRECTION ( 'NONE',  ( 0.000000000000000000, 0.000000000000000000, -1.000000000000000000 ) ) ;
#12628=ADVANCED_FACE ( 'NONE', ( #26341 ), #9923, .T. ) ;
#12629=CARTESIAN_POINT ( 'NONE',  ( -84.94597344681494633, 2.143131898507880377E-16, 159.0682875569279702 ) ) ;
#12642=EDGE_CURVE ( 'NONE', #38442, #37949, #1594, .T. ) ;
#12644=DIRECTION ( 'NONE',  ( -1.000000000000000000, -0.000000000000000000, -0.000000000000000000 ) ) ;
#12647=ORIENTED_EDGE ( 'NONE', *, *, #49194, .T. ) ;
#12648=EDGE_CURVE ( 'NONE', #35861, #25110, #50386, .T. ) ;
#12650=CARTESIAN_POINT ( 'NONE',  ( -210.0000000000000568, 0.000000000000000000, -159.1817124430720298 ) ) ;
#12653=AXIS2_PLACEMENT_3D ( 'NONE', #8577, #7823, #43211 ) ;
#12657=CARTESIAN_POINT ( 'NONE',  ( 195.0540265531851105, 2.143131898507880377E-16, 122.5682875569279702 ) ) ;
#12659=EDGE_CURVE ( 'NONE', #34063, #33842, #22857, .T. ) ;
#12662=ADVANCED_FACE ( 'NONE', ( #5826 ), #49384, .T. ) ;
#12663=VERTEX_POINT ( 'NONE', #33539 ) ;
#12666=EDGE_CURVE ( 'NONE', #25919, #7318, #37909, .T. ) ;
#12668=LINE ( 'NONE', #1142, #29498 ) ;
#12673=( BOUNDED_CURVE ( )  B_SPLINE_CURVE ( 3, ( #34843, #15332, #190, #32245 ),
 .UNSPECIFIED., .F., .F. ) 
 B_SPLINE_CURVE_WITH_KNOTS ( ( 4, 4 ),
 ( 4.712388980384689674, 6.283185307179586232 ),
 .UNSPECIFIED. ) 
 CURVE ( )  GEOMETRIC_REPRESENTATION_ITEM ( )  RATIONAL_B_SPLINE_CURVE ( ( 1.000000000000000000, 0.8047378541243649375, 0.8047378541243649375, 1.000000000000000000 ) ) 
 REPRESENTATION_ITEM ( '' )  );
#12678=( BOUNDED_CURVE ( )  B_SPLINE_CURVE ( 3, ( #12849, #8251, #23392, #3885 ),
 .UNSPECIFIED., .F., .F. ) 
 B_SPLINE_CURVE_WITH_KNOTS ( ( 4, 4 ),
 ( 4.712388980384689674, 6.283185307179586232 ),
 .UNSPECIFIED. ) 
 CURVE ( )  GEOMETRIC_REPRESENTATION_ITEM ( )  RATIONAL_B_SPLINE_CURVE ( ( 1.000000000000000000, 0.8047378541243649375, 0.8047378541243649375, 1.000000000000000000 ) ) 
 REPRESENTATION_ITEM ( '' )  );
#12687=EDGE_CURVE ( 'NONE', #14142, #50479, #45297, .T. ) ;
#12688=ORIENTED_EDGE ( 'NONE', *, *, #6036, .T. ) ;
#12693=VERTEX_POINT ( 'NONE', #6837 ) ;
#12696=ADVANCED_FACE ( 'NONE', ( #33038 ), #17624, .T. ) ;
#12697=ORIENTED_EDGE ( 'NONE', *, *, #48838, .F. ) ;
#12699=ADVANCED_FACE ( 'NONE', ( #38655 ), #50647, .T. ) ;
#12701=VECTOR ( 'NONE', #29089, 1000.000000000000000 ) ;
#12705=CARTESIAN_POINT ( 'NONE',  ( 111.5540265531850537, 1.025126265847081886, -40.93171244307202272 ) ) ;
#12712=VERTEX_POINT ( 'NONE', #15551 ) ;
#12713=CARTESIAN_POINT ( 'NONE',  ( -166.6959734468149463, 0.000000000000000000, 165.0000000000000000 ) ) ;
#12714=CARTESIAN_POINT ( 'NONE',  ( -206.6959734468149463, 1.750000000000010658, 120.8182875569279702 ) ) ;
#12717=FACE_OUTER_BOUND ( 'NONE', #43851, .T. ) ;
#12718=ORIENTED_EDGE ( 'NONE', *, *, #6252, .F. ) ;
#12720=CARTESIAN_POINT ( 'NONE',  ( 34.32915281903212446, -1.750000000000009548, -118.1565861772249519 ) ) ;
#12723=EDGE_CURVE ( 'NONE', #46038, #11473, #33067, .T. ) ;
#12725=EDGE_CURVE ( 'NONE', #5511, #31646, #7867, .T. ) ;
#12727=EDGE_CURVE ( 'NONE', #33842, #40358, #41893, .T. ) ;
#12737=CARTESIAN_POINT ( 'NONE',  ( 154.3291528190321458, 1.750000000000009548, 41.84341382277508359 ) ) ;
#12740=CARTESIAN_POINT ( 'NONE',  ( -86.69597344681496054, 0.000000000000000000, 165.0000000000000000 ) ) ;
#12741=CARTESIAN_POINT ( 'NONE',  ( 75.05402655318509630, 2.143131898507880377E-16, 2.568287556928006143 ) ) ;
#12744=CARTESIAN_POINT ( 'NONE',  ( 195.0540265531851105, 2.143131898507880377E-16, -117.4317124430720725 ) ) ;
#12747=VECTOR ( 'NONE', #11218, 1000.000000000000000 ) ;
#12751=ADVANCED_FACE ( 'NONE', ( #3744 ), #39425, .T. ) ;
#12756=CARTESIAN_POINT ( 'NONE',  ( -4.945973446814903696, 2.143131898507912917E-16, -80.93171244307204404 ) ) ;
#12759=CARTESIAN_POINT ( 'NONE',  ( -86.69597344681494633, -1.750000000000010658, -119.1817124430720440 ) ) ;
#12763=DIRECTION ( 'NONE',  ( 1.000000000000000000, 0.000000000000000000, -0.000000000000000000 ) ) ;
#12764=CARTESIAN_POINT ( 'NONE',  ( -88.44597344681497475, 0.000000000000000000, -77.43171244307198720 ) ) ;
#12769=CARTESIAN_POINT ( 'NONE',  ( 210.0000000000000568, 0.000000000000000000, -79.18171244307201562 ) ) ;
#12770=EDGE_CURVE ( 'NONE', #48741, #10841, #30347, .T. ) ;
#12772=ORIENTED_EDGE ( 'NONE', *, *, #1865, .T. ) ;
#12774=DIRECTION ( 'NONE',  ( -1.000000000000000000, 0.000000000000000000, 0.000000000000000000 ) ) ;
#12775=DIRECTION ( 'NONE',  ( -0.000000000000000000, -0.000000000000000000, -1.000000000000000000 ) ) ;
#12777=CARTESIAN_POINT ( 'NONE',  ( 113.3040265531850537, -1.749999999999996891, -159.1817124430720298 ) ) ;
#12780=CARTESIAN_POINT ( 'NONE',  ( -86.69597344681494633, -1.750000000000010658, 80.81828755692798438 ) ) ;
#12782=CARTESIAN_POINT ( 'NONE',  ( 33.30402655318503946, 1.750000000000010658, 120.8182875569279702 ) ) ;
#12784=VECTOR ( 'NONE', #33716, 1000.000000000000000 ) ;
#12800=DIRECTION ( 'NONE',  ( -1.000000000000000000, 0.000000000000000000, 0.000000000000000000 ) ) ;
#12805=CARTESIAN_POINT ( 'NONE',  ( 74.32915281903215998, -1.750000000000010436, -120.2068387089191219 ) ) ;
#12806=CARTESIAN_POINT ( 'NONE',  ( 111.5540265531850679, 0.000000000000000000, -157.4317124430720582 ) ) ;
#12810=ORIENTED_EDGE ( 'NONE', *, *, #14396, .T. ) ;
#12812=VECTOR ( 'NONE', #16873, 1000.000000000000000 ) ;
#12817=ORIENTED_EDGE ( 'NONE', *, *, #16180, .F. ) ;
#12818=CYLINDRICAL_SURFACE ( 'NONE', #13129, 1.750000000000015543 ) ;
#12822=EDGE_LOOP ( 'NONE', ( #42067, #21206 ) ) ;
#12823=AXIS2_PLACEMENT_3D ( 'NONE', #3915, #31389, #46980 ) ;
#12825=( BOUNDED_CURVE ( )  B_SPLINE_CURVE ( 3, ( #14024, #32796, #33553, #29685 ),
 .UNSPECIFIED., .F., .F. ) 
 B_SPLINE_CURVE_WITH_KNOTS ( ( 4, 4 ),
 ( 4.712388980384689674, 6.283185307179586232 ),
 .UNSPECIFIED. ) 
 CURVE ( )  GEOMETRIC_REPRESENTATION_ITEM ( )  RATIONAL_B_SPLINE_CURVE ( ( 1.000000000000000000, 0.8047378541243649375, 0.8047378541243649375, 1.000000000000000000 ) ) 
 REPRESENTATION_ITEM ( '' )  );
#12827=CARTESIAN_POINT ( 'NONE',  ( 154.3291528190321458, -1.750000000000009548, -38.15658617722494483 ) ) ;
#12831=ORIENTED_EDGE ( 'NONE', *, *, #5906, .F. ) ;
#12832=EDGE_CURVE ( 'NONE', #11124, #8521, #6830, .T. ) ;
#12835=CARTESIAN_POINT ( 'NONE',  ( -44.94597344681493922, 2.143131898507880377E-16, -80.93171244307204404 ) ) ;
#12836=CARTESIAN_POINT ( 'NONE',  ( 195.0540265531851105, 1.025126265847089435, 159.0682875569279418 ) ) ;
#12840=( BOUNDED_CURVE ( )  B_SPLINE_CURVE ( 3, ( #17557, #44973, #9850, #5998 ),
 .UNSPECIFIED., .F., .F. ) 
 B_SPLINE_CURVE_WITH_KNOTS ( ( 4, 4 ),
 ( 0.000000000000000000, 1.570796326794896558 ),
 .UNSPECIFIED. ) 
 CURVE ( )  GEOMETRIC_REPRESENTATION_ITEM ( )  RATIONAL_B_SPLINE_CURVE ( ( 1.000000000000000000, 0.8047378541243649375, 0.8047378541243649375, 1.000000000000000000 ) ) 
 REPRESENTATION_ITEM ( '' )  );
#12842=VERTEX_POINT ( 'NONE', #413 ) ;
#12849=CARTESIAN_POINT ( 'NONE',  ( 153.3040265531850537, -1.750000000000010658, -119.1817124430720440 ) ) ;
#12850=VERTEX_POINT ( 'NONE', #16061 ) ;
#12854=CARTESIAN_POINT ( 'NONE',  ( -48.44597344681496054, 1.025126265847089657, 79.06828755692797017 ) ) ;
#12859=CARTESIAN_POINT ( 'NONE',  ( -44.94597344681493922, 2.143131898507880377E-16, -0.9317124430720247208 ) ) ;
#12861=CARTESIAN_POINT ( 'NONE',  ( 115.0540265531850395, 2.143131898507847836E-16, -40.93171244307202983 ) ) ;
#12863=EDGE_CURVE ( 'NONE', #4897, #5706, #4258, .T. ) ;
#12869=DIRECTION ( 'NONE',  ( -1.000000000000000000, -0.000000000000000000, -0.000000000000000000 ) ) ;
#12871=ORIENTED_EDGE ( 'NONE', *, *, #45666, .T. ) ;
#12873=CARTESIAN_POINT ( 'NONE',  ( -126.6959734468149321, -1.749999999999996891, 0.8182875569279768335 ) ) ;
#12893=LINE ( 'NONE', #5200, #45133 ) ;
#12897=EDGE_LOOP ( 'NONE', ( #13725, #17754, #21507, #18547, #30438 ) ) ;
#12898=CARTESIAN_POINT ( 'NONE',  ( -168.4459734468149747, 1.025126265847089435, -40.93171244307204404 ) ) ;
#12901=LINE ( 'NONE', #36541, #31793 ) ;
#12902=CARTESIAN_POINT ( 'NONE',  ( -44.94597344681493922, 2.143131898507880377E-16, -117.4317124430720156 ) ) ;
#12908=LINE ( 'NONE', #44199, #29640 ) ;
#12910=DIRECTION ( 'NONE',  ( 0.000000000000000000, 0.000000000000000000, -1.000000000000000000 ) ) ;
#12911=ORIENTED_EDGE ( 'NONE', *, *, #35342, .T. ) ;
#12912=( BOUNDED_CURVE ( )  B_SPLINE_CURVE ( 3, ( #20187, #42510, #7386, #5800 ),
 .UNSPECIFIED., .F., .F. ) 
 B_SPLINE_CURVE_WITH_KNOTS ( ( 4, 4 ),
 ( 4.712388980384689674, 6.283185307179586232 ),
 .UNSPECIFIED. ) 
 CURVE ( )  GEOMETRIC_REPRESENTATION_ITEM ( )  RATIONAL_B_SPLINE_CURVE ( ( 1.000000000000000000, 0.8047378541243649375, 0.8047378541243649375, 1.000000000000000000 ) ) 
 REPRESENTATION_ITEM ( '' )  );
#12913=CARTESIAN_POINT ( 'NONE',  ( 73.30402655318508209, 1.750000000000010658, -79.18171244307201562 ) ) ;
#12917=CARTESIAN_POINT ( 'NONE',  ( 210.0000000000000568, 0.000000000000000000, -157.4317124430720298 ) ) ;
#12919=ORIENTED_EDGE ( 'NONE', *, *, #22425, .F. ) ;
#12923=CARTESIAN_POINT ( 'NONE',  ( 210.0000000000000568, 0.000000000000000000, -119.1817124430720440 ) ) ;
#12925=ORIENTED_EDGE ( 'NONE', *, *, #38753, .F. ) ;
#12930=AXIS2_PLACEMENT_3D ( 'NONE', #17267, #21358, #1625 ) ;
#12931=ORIENTED_EDGE ( 'NONE', *, *, #23360, .T. ) ;
#12934=CARTESIAN_POINT ( 'NONE',  ( 33.30402655318503946, 1.750000000000010214, 40.81828755692798438 ) ) ;
#12945=ORIENTED_EDGE ( 'NONE', *, *, #39947, .F. ) ;
#12946=EDGE_LOOP ( 'NONE', ( #17899, #20592, #29465, #14791, #1576, #31421 ) ) ;
#12950=DIRECTION ( 'NONE',  ( -1.000000000000000000, -0.000000000000000000, -0.000000000000000000 ) ) ;
#12953=DIRECTION ( 'NONE',  ( -0.000000000000000000, -0.000000000000000000, -1.000000000000000000 ) ) ;
#12956=DIRECTION ( 'NONE',  ( -0.000000000000000000, -0.000000000000000000, -1.000000000000000000 ) ) ;
#12957=ORIENTED_EDGE ( 'NONE', *, *, #20181, .T. ) ;
#12959=DIRECTION ( 'NONE',  ( -1.000000000000000000, 0.000000000000000000, 0.000000000000000000 ) ) ;
#12961=EDGE_CURVE ( 'NONE', #5769, #4874, #20922, .T. ) ;
#12962=( BOUNDED_CURVE ( )  B_SPLINE_CURVE ( 3, ( #22145, #6738, #37814, #37566 ),
 .UNSPECIFIED., .F., .F. ) 
 B_SPLINE_CURVE_WITH_KNOTS ( ( 4, 4 ),
 ( 1.570796326794896558, 3.141592653589793116 ),
 .UNSPECIFIED. ) 
 CURVE ( )  GEOMETRIC_REPRESENTATION_ITEM ( )  RATIONAL_B_SPLINE_CURVE ( ( 1.000000000000000000, 0.8047378541243649375, 0.8047378541243649375, 1.000000000000000000 ) ) 
 REPRESENTATION_ITEM ( '' )  );
#12965=ADVANCED_FACE ( 'NONE', ( #37988 ), #25415, .T. ) ;
#12966=CARTESIAN_POINT ( 'NONE',  ( 32.27890028733795447, 1.750000000000010436, 119.7931612910808781 ) ) ;
#12967=ADVANCED_FACE ( 'NONE', ( #37736 ), #29262, .T. ) ;
#12968=CARTESIAN_POINT ( 'NONE',  ( -126.6959734468149321, 1.749999999999997335, 80.81828755692798438 ) ) ;
#12969=( BOUNDED_CURVE ( )  B_SPLINE_CURVE ( 3, ( #47717, #44394, #37008, #40076 ),
 .UNSPECIFIED., .F., .F. ) 
 B_SPLINE_CURVE_WITH_KNOTS ( ( 4, 4 ),
 ( 1.570796326794896558, 3.141592653589793116 ),
 .UNSPECIFIED. ) 
 CURVE ( )  GEOMETRIC_REPRESENTATION_ITEM ( )  RATIONAL_B_SPLINE_CURVE ( ( 1.000000000000000000, 0.8047378541243649375, 0.8047378541243649375, 1.000000000000000000 ) ) 
 REPRESENTATION_ITEM ( '' )  );
#12970=DIRECTION ( 'NONE',  ( -1.000000000000000000, -0.000000000000000000, -0.000000000000000000 ) ) ;
#12976=CARTESIAN_POINT ( 'NONE',  ( -88.44597344681494633, 1.025126265847089213, 159.0682875569279418 ) ) ;
#12978=CARTESIAN_POINT ( 'NONE',  ( -126.6959734468149321, 1.749999999999996891, 0.8182875569279768335 ) ) ;
#12980=CARTESIAN_POINT ( 'NONE',  ( -85.67084718096784002, -1.750000000000009548, 81.84341382277507648 ) ) ;
#12988=DIRECTION ( 'NONE',  ( -0.000000000000000000, -0.000000000000000000, -1.000000000000000000 ) ) ;
#12989=CARTESIAN_POINT ( 'NONE',  ( -168.4459734468149463, 0.000000000000000000, -0.9317124430720247208 ) ) ;
#12990=ORIENTED_EDGE ( 'NONE', *, *, #25437, .T. ) ;
#12994=ADVANCED_FACE ( 'NONE', ( #11540 ), #39248, .T. ) ;
#12995=ORIENTED_EDGE ( 'NONE', *, *, #20801, .F. ) ;
#13000=ADVANCED_FACE ( 'NONE', ( #46395 ), #43077, .T. ) ;
#13005=CARTESIAN_POINT ( 'NONE',  ( -204.9459734468149463, 2.143131898507880377E-16, 165.0000000000000000 ) ) ;
#13006=ORIENTED_EDGE ( 'NONE', *, *, #35978, .T. ) ;
#13015=DIRECTION ( 'NONE',  ( -1.000000000000000000, -0.000000000000000000, -0.000000000000000000 ) ) ;
#13017=FACE_OUTER_BOUND ( 'NONE', #24126, .T. ) ;
#13019=CARTESIAN_POINT ( 'NONE',  ( 111.5540265531850537, 1.025126265847081664, -37.43171244307203693 ) ) ;
#13021=LINE ( 'NONE', #21732, #33942 ) ;
#13022=CARTESIAN_POINT ( 'NONE',  ( -46.69597344681494633, -1.750000000000009992, 0.8182875569279768335 ) ) ;
#13024=DIRECTION ( 'NONE',  ( -1.000000000000000000, -0.000000000000000000, -0.000000000000000000 ) ) ;
#13032=DIRECTION ( 'NONE',  ( -1.000000000000000000, -0.000000000000000000, -0.000000000000000000 ) ) ;
#13036=CYLINDRICAL_SURFACE ( 'NONE', #30389, 1.750000000000001554 ) ;
#13039=CARTESIAN_POINT ( 'NONE',  ( -124.9459734468149463, 2.143131898507847836E-16, -80.93171244307201562 ) ) ;
#13042=EDGE_LOOP ( 'NONE', ( #2643, #17963, #15624, #41173, #24862, #41071 ) ) ;
#13043=VECTOR ( 'NONE', #34872, 1000.000000000000000 ) ;
#13046=EDGE_CURVE ( 'NONE', #38061, #47848, #33373, .T. ) ;
#13050=ORIENTED_EDGE ( 'NONE', *, *, #17834, .T. ) ;
#13055=ORIENTED_EDGE ( 'NONE', *, *, #13944, .T. ) ;
#13061=CARTESIAN_POINT ( 'NONE',  ( 210.0000000000000568, 0.000000000000000000, -39.18171244307202983 ) ) ;
#13067=ADVANCED_FACE ( 'NONE', ( #34385 ), #26678, .T. ) ;
#13071=ORIENTED_EDGE ( 'NONE', *, *, #7454, .F. ) ;
#13073=CARTESIAN_POINT ( 'NONE',  ( -4.945973446814903696, 2.143131898507912917E-16, 79.06828755692795596 ) ) ;
#13074=EDGE_CURVE ( 'NONE', #7169, #12438, #8161, .T. ) ;
#13076=ORIENTED_EDGE ( 'NONE', *, *, #39357, .F. ) ;
#13080=DIRECTION ( 'NONE',  ( -1.000000000000000000, 0.000000000000000000, 0.000000000000000000 ) ) ;
#13083=CARTESIAN_POINT ( 'NONE',  ( -206.6959734468149463, -1.750000000000009992, -159.1817124430720298 ) ) ;
#13085=VERTEX_POINT ( 'NONE', #32307 ) ;
#13086=CARTESIAN_POINT ( 'NONE',  ( -6.695973446814940111, 1.750000000000023759, -39.18171244307202983 ) ) ;
#13087=DIRECTION ( 'NONE',  ( -1.000000000000000000, 0.000000000000000000, 0.000000000000000000 ) ) ;
#13089=EDGE_CURVE ( 'NONE', #8176, #31607, #5341, .T. ) ;
#13090=ORIENTED_EDGE ( 'NONE', *, *, #7987, .F. ) ;
#13093=VECTOR ( 'NONE', #5423, 1000.000000000000000 ) ;
#13094=CARTESIAN_POINT ( 'NONE',  ( -8.445973446814964092, 1.025126265847096985, -37.43171244307200851 ) ) ;
#13103=EDGE_LOOP ( 'NONE', ( #16694, #30931, #15536, #6396, #48931, #7033 ) ) ;
#13104=CARTESIAN_POINT ( 'NONE',  ( 71.55402655318505367, 0.000000000000000000, 39.06828755692795596 ) ) ;
#13106=CARTESIAN_POINT ( 'NONE',  ( -206.6959734468149463, -1.750000000000010214, -39.18171244307202983 ) ) ;
#13107=EDGE_LOOP ( 'NONE', ( #19490, #3596, #652, #29520, #45733, #20899 ) ) ;
#13108=CARTESIAN_POINT ( 'NONE',  ( -204.9459734468148895, 1.025126265847089213, 159.0682875569279418 ) ) ;
#13109=CARTESIAN_POINT ( 'NONE',  ( -208.4459734468148611, -1.025126265847089213, -160.9317124430720014 ) ) ;
#13110=CARTESIAN_POINT ( 'NONE',  ( -85.67084718096784002, 1.750000000000009548, 39.79316129108089228 ) ) ;
#13111=AXIS2_PLACEMENT_3D ( 'NONE', #33025, #12988, #17105 ) ;
#13113=EDGE_CURVE ( 'NONE', #45829, #39370, #20487, .T. ) ;
#13114=VECTOR ( 'NONE', #50300, 1000.000000000000000 ) ;
#13115=( BOUNDED_CURVE ( )  B_SPLINE_CURVE ( 3, ( #36891, #17103, #5299, #25066 ),
 .UNSPECIFIED., .F., .F. ) 
 B_SPLINE_CURVE_WITH_KNOTS ( ( 4, 4 ),
 ( 0.000000000000000000, 1.570796326794896558 ),
 .UNSPECIFIED. ) 
 CURVE ( )  GEOMETRIC_REPRESENTATION_ITEM ( )  RATIONAL_B_SPLINE_CURVE ( ( 1.000000000000000000, 0.8047378541243649375, 0.8047378541243649375, 1.000000000000000000 ) ) 
 REPRESENTATION_ITEM ( '' )  );
#13123=( BOUNDED_CURVE ( )  B_SPLINE_CURVE ( 3, ( #20868, #8325, #27819, #36548 ),
 .UNSPECIFIED., .F., .F. ) 
 B_SPLINE_CURVE_WITH_KNOTS ( ( 4, 4 ),
 ( 1.570796326794896558, 3.141592653589793116 ),
 .UNSPECIFIED. ) 
 CURVE ( )  GEOMETRIC_REPRESENTATION_ITEM ( )  RATIONAL_B_SPLINE_CURVE ( ( 1.000000000000000000, 0.8047378541243649375, 0.8047378541243649375, 1.000000000000000000 ) ) 
 REPRESENTATION_ITEM ( '' )  );
#13124=DIRECTION ( 'NONE',  ( -1.000000000000000000, 0.000000000000000000, 0.000000000000000000 ) ) ;
#13125=AXIS2_PLACEMENT_3D ( 'NONE', #725, #32039, #16371 ) ;
#13126=VERTEX_POINT ( 'NONE', #506 ) ;
#13127=ORIENTED_EDGE ( 'NONE', *, *, #24035, .T. ) ;
#13129=AXIS2_PLACEMENT_3D ( 'NONE', #43347, #28723, #4368 ) ;
#13132=EDGE_CURVE ( 'NONE', #49775, #4462, #12532, .T. ) ;
#13136=ORIENTED_EDGE ( 'NONE', *, *, #30906, .T. ) ;
#13138=( BOUNDED_CURVE ( )  B_SPLINE_CURVE ( 3, ( #38930, #3756, #23773, #28124 ),
 .UNSPECIFIED., .F., .F. ) 
 B_SPLINE_CURVE_WITH_KNOTS ( ( 4, 4 ),
 ( 1.570796326794896558, 3.141592653589793116 ),
 .UNSPECIFIED. ) 
 CURVE ( )  GEOMETRIC_REPRESENTATION_ITEM ( )  RATIONAL_B_SPLINE_CURVE ( ( 1.000000000000000000, 0.8047378541243649375, 0.8047378541243649375, 1.000000000000000000 ) ) 
 REPRESENTATION_ITEM ( '' )  );
#13139=FACE_OUTER_BOUND ( 'NONE', #1418, .T. ) ;
#13143=CARTESIAN_POINT ( 'NONE',  ( 33.30402655318503946, -1.750000000000009992, 160.8182875569279702 ) ) ;
#13146=VERTEX_POINT ( 'NONE', #9189 ) ;
#13149=CARTESIAN_POINT ( 'NONE',  ( -168.4459734468149463, 0.000000000000000000, -117.4317124430720725 ) ) ;
#13153=CARTESIAN_POINT ( 'NONE',  ( 72.27890028733797578, -1.750000000000009548, 1.843413822775065825 ) ) ;
#13156=AXIS2_PLACEMENT_3D ( 'NONE', #4302, #3264, #35620 ) ;
#13160=DIRECTION ( 'NONE',  ( 0.000000000000000000, 0.000000000000000000, 1.000000000000000000 ) ) ;
#13162=AXIS2_PLACEMENT_3D ( 'NONE', #49537, #6993, #10837 ) ;
#13164=CYLINDRICAL_SURFACE ( 'NONE', #26609, 1.750000000000015543 ) ;
#13166=ORIENTED_EDGE ( 'NONE', *, *, #23723, .F. ) ;
#13167=CARTESIAN_POINT ( 'NONE',  ( -205.6708471809678827, -1.750000000000009548, 159.7931612910809065 ) ) ;
#13176=DIRECTION ( 'NONE',  ( -0.000000000000000000, -0.000000000000000000, -1.000000000000000000 ) ) ;
#13184=CARTESIAN_POINT ( 'NONE',  ( 153.3040265531850537, 0.000000000000000000, -165.0000000000000000 ) ) ;
#13185=CARTESIAN_POINT ( 'NONE',  ( 210.0000000000000568, 0.000000000000000000, -119.1817124430720440 ) ) ;
#13190=CYLINDRICAL_SURFACE ( 'NONE', #21389, 1.750000000000015543 ) ;
#13192=VERTEX_POINT ( 'NONE', #43829 ) ;
#13195=CARTESIAN_POINT ( 'NONE',  ( 210.0000000000000568, 0.000000000000000000, -159.1817124430720298 ) ) ;
#13197=LINE ( 'NONE', #9355, #37086 ) ;
#13199=ORIENTED_EDGE ( 'NONE', *, *, #1487, .T. ) ;
#13206=ADVANCED_FACE ( 'NONE', ( #1000 ), #40249, .T. ) ;
#13212=CARTESIAN_POINT ( 'NONE',  ( -128.4459734468149463, 1.025126265847081664, 82.56828755692798438 ) ) ;
#13215=CARTESIAN_POINT ( 'NONE',  ( -86.69597344681496054, 0.000000000000000000, 165.0000000000000000 ) ) ;
#13218=( BOUNDED_CURVE ( )  B_SPLINE_CURVE ( 3, ( #37925, #3492, #34313, #26610 ),
 .UNSPECIFIED., .F., .F. ) 
 B_SPLINE_CURVE_WITH_KNOTS ( ( 4, 4 ),
 ( 0.000000000000000000, 1.570796326794896558 ),
 .UNSPECIFIED. ) 
 CURVE ( )  GEOMETRIC_REPRESENTATION_ITEM ( )  RATIONAL_B_SPLINE_CURVE ( ( 1.000000000000000000, 0.8047378541243649375, 0.8047378541243649375, 1.000000000000000000 ) ) 
 REPRESENTATION_ITEM ( '' )  );
#13219=CARTESIAN_POINT ( 'NONE',  ( 153.3040265531850537, -1.750000000000009992, 0.8182875569279768335 ) ) ;
#13223=DIRECTION ( 'NONE',  ( 1.000000000000000000, 0.000000000000000000, 0.000000000000000000 ) ) ;
#13226=AXIS2_PLACEMENT_3D ( 'NONE', #8181, #23573, #16374 ) ;
#13229=AXIS2_PLACEMENT_3D ( 'NONE', #39578, #2254, #16476 ) ;
#13234=CARTESIAN_POINT ( 'NONE',  ( -168.4459734468149463, 0.000000000000000000, -165.0000000000000000 ) ) ;
#13240=DIRECTION ( 'NONE',  ( -1.000000000000000000, -0.000000000000000000, -0.000000000000000000 ) ) ;
#13243=FACE_OUTER_BOUND ( 'NONE', #26757, .T. ) ;
#13244=CARTESIAN_POINT ( 'NONE',  ( 35.05402655318504657, 2.143131898507880377E-16, 2.568287556927978166 ) ) ;
#13245=EDGE_LOOP ( 'NONE', ( #44673, #34491, #1629, #27606, #20204, #20705 ) ) ;
#13247=VECTOR ( 'NONE', #37781, 1000.000000000000000 ) ;
#13250=DIRECTION ( 'NONE',  ( -0.000000000000000000, -0.000000000000000000, -1.000000000000000000 ) ) ;
#13251=ORIENTED_EDGE ( 'NONE', *, *, #15140, .T. ) ;
#13253=CARTESIAN_POINT ( 'NONE',  ( 113.3040265531850537, -1.749999999999997335, 80.81828755692798438 ) ) ;
#13256=ORIENTED_EDGE ( 'NONE', *, *, #17337, .T. ) ;
#13257=ORIENTED_EDGE ( 'NONE', *, *, #11835, .F. ) ;
#13258=ORIENTED_EDGE ( 'NONE', *, *, #7072, .F. ) ;
#13264=LINE ( 'NONE', #16622, #6117 ) ;
#13267=( BOUNDED_CURVE ( )  B_SPLINE_CURVE ( 3, ( #17674, #25633, #21271, #45096 ),
 .UNSPECIFIED., .F., .F. ) 
 B_SPLINE_CURVE_WITH_KNOTS ( ( 4, 4 ),
 ( 3.141592653589793116, 4.712388980384689674 ),
 .UNSPECIFIED. ) 
 CURVE ( )  GEOMETRIC_REPRESENTATION_ITEM ( )  RATIONAL_B_SPLINE_CURVE ( ( 1.000000000000000000, 0.8047378541243649375, 0.8047378541243649375, 1.000000000000000000 ) ) 
 REPRESENTATION_ITEM ( '' )  );
#13268=CARTESIAN_POINT ( 'NONE',  ( -44.94597344681493922, 2.143131898507880377E-16, 42.56828755692798438 ) ) ;
#13272=( BOUNDED_CURVE ( )  B_SPLINE_CURVE ( 3, ( #29088, #9584, #25230, #40880 ),
 .UNSPECIFIED., .F., .F. ) 
 B_SPLINE_CURVE_WITH_KNOTS ( ( 4, 4 ),
 ( 1.570796326794896558, 3.141592653589793116 ),
 .UNSPECIFIED. ) 
 CURVE ( )  GEOMETRIC_REPRESENTATION_ITEM ( )  RATIONAL_B_SPLINE_CURVE ( ( 1.000000000000000000, 0.8047378541243649375, 0.8047378541243649375, 1.000000000000000000 ) ) 
 REPRESENTATION_ITEM ( '' )  );
#13273=CYLINDRICAL_SURFACE ( 'NONE', #5971, 1.750000000000015543 ) ;
#13280=DIRECTION ( 'NONE',  ( -0.000000000000000000, -0.000000000000000000, -1.000000000000000000 ) ) ;
#13281=CARTESIAN_POINT ( 'NONE',  ( -84.94597344681494633, 2.143131898507880377E-16, -157.4317124430720582 ) ) ;
#13284=EDGE_CURVE ( 'NONE', #6842, #41828, #49154, .T. ) ;
#13289=CARTESIAN_POINT ( 'NONE',  ( -125.6708471809678542, 1.749999999999996891, -80.20683870891909351 ) ) ;
#13295=FACE_OUTER_BOUND ( 'NONE', #12473, .T. ) ;
#13298=ADVANCED_FACE ( 'NONE', ( #45068 ), #41245, .T. ) ;
#13299=ORIENTED_EDGE ( 'NONE', *, *, #37460, .T. ) ;
#13306=CARTESIAN_POINT ( 'NONE',  ( 75.05402655318509630, 1.025126265847089657, -80.93171244307201562 ) ) ;
#13315=CARTESIAN_POINT ( 'NONE',  ( -46.69597344681494633, 0.000000000000000000, 165.0000000000000000 ) ) ;
#13316=EDGE_CURVE ( 'NONE', #4874, #40803, #19257, .T. ) ;
#13317=ORIENTED_EDGE ( 'NONE', *, *, #8467, .T. ) ;
#13320=EDGE_LOOP ( 'NONE', ( #31388, #2354, #17250, #12331, #27032, #48552 ) ) ;
#13331=CARTESIAN_POINT ( 'NONE',  ( -84.94597344681494633, 2.143131898507880377E-16, 79.06828755692797017 ) ) ;
#13332=DIRECTION ( 'NONE',  ( -0.000000000000000000, -0.000000000000000000, -1.000000000000000000 ) ) ;
#13338=EDGE_LOOP ( 'NONE', ( #4031, #28848, #46401, #45540, #37037, #27413 ) ) ;
#13340=ORIENTED_EDGE ( 'NONE', *, *, #47793, .T. ) ;
#13342=LINE ( 'NONE', #28255, #36815 ) ;
#13348=CYLINDRICAL_SURFACE ( 'NONE', #30441, 1.750000000000001554 ) ;
#13359=ORIENTED_EDGE ( 'NONE', *, *, #18113, .F. ) ;
#13360=CARTESIAN_POINT ( 'NONE',  ( -124.9459734468149463, 2.143131898507847836E-16, 165.0000000000000000 ) ) ;
#13362=CARTESIAN_POINT ( 'NONE',  ( -86.69597344681496054, 0.000000000000000000, 165.0000000000000000 ) ) ;
#13363=ADVANCED_FACE ( 'NONE', ( #45319 ), #9442, .T. ) ;
#13365=VERTEX_POINT ( 'NONE', #5849 ) ;
#13370=AXIS2_PLACEMENT_3D ( 'NONE', #4658, #4889, #47701 ) ;
#13375=CYLINDRICAL_SURFACE ( 'NONE', #19311, 1.750000000000008438 ) ;
#13379=FACE_OUTER_BOUND ( 'NONE', #18837, .T. ) ;
#13380=ORIENTED_EDGE ( 'NONE', *, *, #12112, .T. ) ;
#13383=VERTEX_POINT ( 'NONE', #49659 ) ;
#13385=CARTESIAN_POINT ( 'NONE',  ( 151.5540265531850537, 0.000000000000000000, 79.06828755692797017 ) ) ;
#13387=DIRECTION ( 'NONE',  ( -0.000000000000000000, -0.000000000000000000, -1.000000000000000000 ) ) ;
#13390=CARTESIAN_POINT ( 'NONE',  ( 75.05402655318509630, -1.025126265847088991, -157.4317124430720582 ) ) ;
#13395=DIRECTION ( 'NONE',  ( -0.000000000000000000, -0.000000000000000000, -1.000000000000000000 ) ) ;
#13397=VECTOR ( 'NONE', #37088, 1000.000000000000000 ) ;
#13402=EDGE_LOOP ( 'NONE', ( #16924, #21158, #33097, #40111, #37212, #36131 ) ) ;
#13404=DIRECTION ( 'NONE',  ( -1.000000000000000000, -0.000000000000000000, -0.000000000000000000 ) ) ;
#13407=DIRECTION ( 'NONE',  ( -1.000000000000000000, -0.000000000000000000, -0.000000000000000000 ) ) ;
#13408=CARTESIAN_POINT ( 'NONE',  ( -128.4459734468149179, 0.000000000000000000, 165.0000000000000000 ) ) ;
#13412=CYLINDRICAL_SURFACE ( 'NONE', #12213, 1.750000000000001554 ) ;
#13415=( BOUNDED_CURVE ( )  B_SPLINE_CURVE ( 3, ( #15211, #30875, #31115, #22897 ),
 .UNSPECIFIED., .F., .F. ) 
 B_SPLINE_CURVE_WITH_KNOTS ( ( 4, 4 ),
 ( 0.000000000000000000, 1.570796326794896558 ),
 .UNSPECIFIED. ) 
 CURVE ( )  GEOMETRIC_REPRESENTATION_ITEM ( )  RATIONAL_B_SPLINE_CURVE ( ( 1.000000000000000000, 0.8047378541243649375, 0.8047378541243649375, 1.000000000000000000 ) ) 
 REPRESENTATION_ITEM ( '' )  );
#13419=ADVANCED_FACE ( 'NONE', ( #14548 ), #11467, .T. ) ;
#13421=CARTESIAN_POINT ( 'NONE',  ( 193.3040265531851105, 0.000000000000000000, -165.0000000000000000 ) ) ;
#13423=CARTESIAN_POINT ( 'NONE',  ( -4.945973446814903696, 2.143131898507912917E-16, -77.43171244307198720 ) ) ;
#13424=( BOUNDED_CURVE ( )  B_SPLINE_CURVE ( 3, ( #7933, #38721, #31281, #229 ),
 .UNSPECIFIED., .F., .F. ) 
 B_SPLINE_CURVE_WITH_KNOTS ( ( 4, 4 ),
 ( 3.141592653589793116, 4.712388980384689674 ),
 .UNSPECIFIED. ) 
 CURVE ( )  GEOMETRIC_REPRESENTATION_ITEM ( )  RATIONAL_B_SPLINE_CURVE ( ( 1.000000000000000000, 0.8047378541243649375, 0.8047378541243649375, 1.000000000000000000 ) ) 
 REPRESENTATION_ITEM ( '' )  );
#13435=VECTOR ( 'NONE', #25312, 1000.000000000000000 ) ;
#13436=FACE_OUTER_BOUND ( 'NONE', #18168, .T. ) ;
#13440=( BOUNDED_CURVE ( )  B_SPLINE_CURVE ( 3, ( #31672, #3160, #11139, #18810 ),
 .UNSPECIFIED., .F., .F. ) 
 B_SPLINE_CURVE_WITH_KNOTS ( ( 4, 4 ),
 ( 4.712388980384689674, 6.283185307179586232 ),
 .UNSPECIFIED. ) 
 CURVE ( )  GEOMETRIC_REPRESENTATION_ITEM ( )  RATIONAL_B_SPLINE_CURVE ( ( 1.000000000000000000, 0.8047378541243649375, 0.8047378541243649375, 1.000000000000000000 ) ) 
 REPRESENTATION_ITEM ( '' )  );
#13442=ORIENTED_EDGE ( 'NONE', *, *, #28625, .F. ) ;
#13448=CARTESIAN_POINT ( 'NONE',  ( -84.94597344681494633, 2.143131898507880377E-16, -40.93171244307202983 ) ) ;
#13449=CARTESIAN_POINT ( 'NONE',  ( 191.5540265531851105, 0.000000000000000000, 165.0000000000000000 ) ) ;
#13462=ORIENTED_EDGE ( 'NONE', *, *, #41488, .F. ) ;
#13465=LINE ( 'NONE', #37597, #22519 ) ;
#13466=FACE_OUTER_BOUND ( 'NONE', #28327, .T. ) ;
#13467=ORIENTED_EDGE ( 'NONE', *, *, #44930, .T. ) ;
#13473=DIRECTION ( 'NONE',  ( -1.000000000000000000, 0.000000000000000000, 0.000000000000000000 ) ) ;
#13475=VECTOR ( 'NONE', #7510, 1000.000000000000000 ) ;
#13477=CYLINDRICAL_SURFACE ( 'NONE', #28970, 1.750000000000008438 ) ;
#13479=AXIS2_PLACEMENT_3D ( 'NONE', #19125, #15547, #34814 ) ;
#13480=DIRECTION ( 'NONE',  ( -0.000000000000000000, -0.000000000000000000, -1.000000000000000000 ) ) ;
#13481=( BOUNDED_CURVE ( )  B_SPLINE_CURVE ( 3, ( #49002, #29554, #25976, #10060 ),
 .UNSPECIFIED., .F., .F. ) 
 B_SPLINE_CURVE_WITH_KNOTS ( ( 4, 4 ),
 ( 3.141592653589793116, 4.712388980384689674 ),
 .UNSPECIFIED. ) 
 CURVE ( )  GEOMETRIC_REPRESENTATION_ITEM ( )  RATIONAL_B_SPLINE_CURVE ( ( 1.000000000000000000, 0.8047378541243649375, 0.8047378541243649375, 1.000000000000000000 ) ) 
 REPRESENTATION_ITEM ( '' )  );
#13482=CARTESIAN_POINT ( 'NONE',  ( 31.55402655318503236, 0.000000000000000000, 122.5682875569279702 ) ) ;
#13485=VERTEX_POINT ( 'NONE', #32242 ) ;
#13490=DIRECTION ( 'NONE',  ( -1.000000000000000000, 0.000000000000000000, 0.000000000000000000 ) ) ;
#13493=CARTESIAN_POINT ( 'NONE',  ( 195.0540265531851105, 2.143131898507880377E-16, 39.06828755692798438 ) ) ;
#13495=LINE ( 'NONE', #25062, #40486 ) ;
#13499=ORIENTED_EDGE ( 'NONE', *, *, #11102, .F. ) ;
#13506=DIRECTION ( 'NONE',  ( 0.000000000000000000, 0.000000000000000000, 1.000000000000000000 ) ) ;
#13510=CARTESIAN_POINT ( 'NONE',  ( 33.30402655318503946, -1.750000000000009992, -159.1817124430720298 ) ) ;
#13512=VERTEX_POINT ( 'NONE', #35855 ) ;
#13515=ORIENTED_EDGE ( 'NONE', *, *, #18113, .T. ) ;
#13516=CARTESIAN_POINT ( 'NONE',  ( 153.3040265531850537, -1.750000000000009992, 160.8182875569279702 ) ) ;
#13522=VECTOR ( 'NONE', #18339, 1000.000000000000000 ) ;
#13527=AXIS2_PLACEMENT_3D ( 'NONE', #28631, #16841, #47592 ) ;
#13530=CARTESIAN_POINT ( 'NONE',  ( -48.44597344681495343, 0.000000000000000000, 165.0000000000000000 ) ) ;
#13536=ORIENTED_EDGE ( 'NONE', *, *, #37344, .T. ) ;
#13539=VERTEX_POINT ( 'NONE', #42679 ) ;
#13543=CARTESIAN_POINT ( 'NONE',  ( 31.55402655318503236, 0.000000000000000000, -80.93171244307204404 ) ) ;
#13546=CARTESIAN_POINT ( 'NONE',  ( -7.721099712662037540, -1.750000000000023537, 119.7931612910808781 ) ) ;
#13547=ADVANCED_FACE ( 'NONE', ( #8640 ), #20420, .T. ) ;
#13551=CARTESIAN_POINT ( 'NONE',  ( -208.4459734468149463, 0.000000000000000000, 122.5682875569279702 ) ) ;
#13559=AXIS2_PLACEMENT_3D ( 'NONE', #36069, #36592, #43492 ) ;
#13562=CARTESIAN_POINT ( 'NONE',  ( 31.55402655318503236, 1.025126265847089213, -0.9317124430720324924 ) ) ;
#13564=LINE ( 'NONE', #33340, #26551 ) ;
#13566=EDGE_CURVE ( 'NONE', #38882, #2039, #8139, .T. ) ;
#13567=CARTESIAN_POINT ( 'NONE',  ( 32.27890028733795447, 1.750000000000009326, 1.843413822775066269 ) ) ;
#13568=ORIENTED_EDGE ( 'NONE', *, *, #2632, .T. ) ;
#13569=PLANE ( 'NONE',  #9196 ) ;
#13571=( BOUNDED_CURVE ( )  B_SPLINE_CURVE ( 3, ( #6598, #22253, #1997, #17881 ),
 .UNSPECIFIED., .F., .F. ) 
 B_SPLINE_CURVE_WITH_KNOTS ( ( 4, 4 ),
 ( 3.141592653589793116, 4.712388980384689674 ),
 .UNSPECIFIED. ) 
 CURVE ( )  GEOMETRIC_REPRESENTATION_ITEM ( )  RATIONAL_B_SPLINE_CURVE ( ( 1.000000000000000000, 0.8047378541243649375, 0.8047378541243649375, 1.000000000000000000 ) ) 
 REPRESENTATION_ITEM ( '' )  );
#13578=ORIENTED_EDGE ( 'NONE', *, *, #34700, .T. ) ;
#13583=EDGE_CURVE ( 'NONE', #43433, #9119, #6526, .T. ) ;
#13584=ORIENTED_EDGE ( 'NONE', *, *, #41556, .F. ) ;
#13587=VECTOR ( 'NONE', #13857, 1000.000000000000000 ) ;
#13595=CARTESIAN_POINT ( 'NONE',  ( 33.30402655318503946, 0.000000000000000000, 165.0000000000000000 ) ) ;
#13596=EDGE_CURVE ( 'NONE', #34539, #28572, #10424, .T. ) ;
#13597=CARTESIAN_POINT ( 'NONE',  ( 73.30402655318508209, 1.750000000000010658, -119.1817124430720440 ) ) ;
#13599=CARTESIAN_POINT ( 'NONE',  ( -206.6959734468149463, -1.750000000000010214, -39.18171244307202983 ) ) ;
#13603=DIRECTION ( 'NONE',  ( -1.000000000000000000, 0.000000000000000000, 0.000000000000000000 ) ) ;
#13612=LINE ( 'NONE', #14107, #5932 ) ;
#13613=EDGE_LOOP ( 'NONE', ( #7551, #43012, #2246, #21443, #32571, #1736 ) ) ;
#13615=CARTESIAN_POINT ( 'NONE',  ( 113.3040265531850537, -1.749999999999997113, -39.18171244307202983 ) ) ;
#13618=DIRECTION ( 'NONE',  ( -1.000000000000000000, -0.000000000000000000, -0.000000000000000000 ) ) ;
#13620=DIRECTION ( 'NONE',  ( 0.000000000000000000, 0.000000000000000000, -1.000000000000000000 ) ) ;
#13625=VERTEX_POINT ( 'NONE', #26052 ) ;
#13626=FACE_OUTER_BOUND ( 'NONE', #35626, .T. ) ;
#13627=FACE_OUTER_BOUND ( 'NONE', #30325, .T. ) ;
#13629=DIRECTION ( 'NONE',  ( 0.000000000000000000, 0.000000000000000000, 1.000000000000000000 ) ) ;
#13632=VERTEX_POINT ( 'NONE', #1693 ) ;
#13637=DIRECTION ( 'NONE',  ( -0.000000000000000000, -0.000000000000000000, -1.000000000000000000 ) ) ;
#13642=DIRECTION ( 'NONE',  ( -1.000000000000000000, -0.000000000000000000, -0.000000000000000000 ) ) ;
#13645=CARTESIAN_POINT ( 'NONE',  ( -86.69597344681496054, 0.000000000000000000, 165.0000000000000000 ) ) ;
#13647=CARTESIAN_POINT ( 'NONE',  ( 35.05402655318504657, 2.143131898507880377E-16, 159.0682875569279702 ) ) ;
#13650=EDGE_CURVE ( 'NONE', #19888, #25919, #11782, .T. ) ;
#13659=EDGE_CURVE ( 'NONE', #26096, #31600, #35040, .T. ) ;
#13660=CYLINDRICAL_SURFACE ( 'NONE', #34623, 1.750000000000015543 ) ;
#13662=AXIS2_PLACEMENT_3D ( 'NONE', #41773, #18421, #37954 ) ;
#13665=DIRECTION ( 'NONE',  ( -0.000000000000000000, -0.000000000000000000, -1.000000000000000000 ) ) ;
#13666=DIRECTION ( 'NONE',  ( -1.000000000000000000, -0.000000000000000000, -0.000000000000000000 ) ) ;
#13668=FACE_OUTER_BOUND ( 'NONE', #1328, .T. ) ;
#13669=LINE ( 'NONE', #25731, #17594 ) ;
#13671=ORIENTED_EDGE ( 'NONE', *, *, #31288, .T. ) ;
#13673=FACE_OUTER_BOUND ( 'NONE', #11787, .T. ) ;
#13683=ORIENTED_EDGE ( 'NONE', *, *, #28630, .T. ) ;
#13686=CARTESIAN_POINT ( 'NONE',  ( 210.0000000000000568, 0.000000000000000000, 160.8182875569279702 ) ) ;
#13698=CARTESIAN_POINT ( 'NONE',  ( 195.0540265531851105, 2.143131898507880377E-16, -77.43171244307204404 ) ) ;
#13700=ORIENTED_EDGE ( 'NONE', *, *, #8625, .T. ) ;
#13708=EDGE_LOOP ( 'NONE', ( #24468, #48629, #46981, #15725, #48721, #14470 ) ) ;
#13709=CARTESIAN_POINT ( 'NONE',  ( 210.0000000000000568, 0.000000000000000000, -39.18171244307202983 ) ) ;
#13712=VERTEX_POINT ( 'NONE', #12350 ) ;
#13714=EDGE_CURVE ( 'NONE', #45927, #19269, #40253, .T. ) ;
#13717=VERTEX_POINT ( 'NONE', #23407 ) ;
#13720=( BOUNDED_CURVE ( )  B_SPLINE_CURVE ( 3, ( #37774, #26208, #14401, #25704 ),
 .UNSPECIFIED., .F., .F. ) 
 B_SPLINE_CURVE_WITH_KNOTS ( ( 4, 4 ),
 ( 0.000000000000000000, 1.570796326794896558 ),
 .UNSPECIFIED. ) 
 CURVE ( )  GEOMETRIC_REPRESENTATION_ITEM ( )  RATIONAL_B_SPLINE_CURVE ( ( 1.000000000000000000, 0.8047378541243649375, 0.8047378541243649375, 1.000000000000000000 ) ) 
 REPRESENTATION_ITEM ( '' )  );
#13723=CARTESIAN_POINT ( 'NONE',  ( -126.6959734468149321, 0.000000000000000000, 165.0000000000000000 ) ) ;
#13724=CARTESIAN_POINT ( 'NONE',  ( 210.0000000000000568, 0.000000000000000000, 80.81828755692798438 ) ) ;
#13725=ORIENTED_EDGE ( 'NONE', *, *, #7489, .F. ) ;
#13728=DIRECTION ( 'NONE',  ( -1.000000000000000000, 0.000000000000000000, 0.000000000000000000 ) ) ;
#13729=EDGE_CURVE ( 'NONE', #39145, #14767, #43837, .T. ) ;
#13730=LINE ( 'NONE', #48584, #27747 ) ;
#13733=CARTESIAN_POINT ( 'NONE',  ( 151.5540265531850537, 0.000000000000000000, -80.93171244307201562 ) ) ;
#13735=DIRECTION ( 'NONE',  ( 0.000000000000000000, 0.000000000000000000, 1.000000000000000000 ) ) ;
#13736=( BOUNDED_CURVE ( )  B_SPLINE_CURVE ( 3, ( #6168, #7181, #22822, #49474 ),
 .UNSPECIFIED., .F., .F. ) 
 B_SPLINE_CURVE_WITH_KNOTS ( ( 4, 4 ),
 ( 3.141592653589793116, 4.712388980384689674 ),
 .UNSPECIFIED. ) 
 CURVE ( )  GEOMETRIC_REPRESENTATION_ITEM ( )  RATIONAL_B_SPLINE_CURVE ( ( 1.000000000000000000, 0.8047378541243649375, 0.8047378541243649375, 1.000000000000000000 ) ) 
 REPRESENTATION_ITEM ( '' )  );
#13741=CYLINDRICAL_SURFACE ( 'NONE', #49092, 1.749999999999987566 ) ;
#13743=ORIENTED_EDGE ( 'NONE', *, *, #24341, .F. ) ;
#13744=DIRECTION ( 'NONE',  ( -1.000000000000000000, -0.000000000000000000, -0.000000000000000000 ) ) ;
#13745=EDGE_LOOP ( 'NONE', ( #24062, #21241, #1176, #1806, #4669, #48041 ) ) ;
#13747=ADVANCED_FACE ( 'NONE', ( #11607 ), #64, .T. ) ;
#13749=ORIENTED_EDGE ( 'NONE', *, *, #15563, .F. ) ;
#13752=ORIENTED_EDGE ( 'NONE', *, *, #34971, .F. ) ;
#13760=ADVANCED_FACE ( 'NONE', ( #39318 ), #43393, .F. ) ;
#13763=VERTEX_POINT ( 'NONE', #42632 ) ;
#13770=ADVANCED_FACE ( 'NONE', ( #575 ), #15201, .T. ) ;
#13771=CARTESIAN_POINT ( 'NONE',  ( 111.5540265531850679, 0.000000000000000000, 165.0000000000000000 ) ) ;
#13773=VECTOR ( 'NONE', #36413, 1000.000000000000000 ) ;
#13777=CARTESIAN_POINT ( 'NONE',  ( -86.69597344681494633, -1.750000000000009992, -159.1817124430720298 ) ) ;
#13779=CARTESIAN_POINT ( 'NONE',  ( 191.5540265531850537, 1.025126265847089657, 79.06828755692797017 ) ) ;
#13781=VERTEX_POINT ( 'NONE', #27513 ) ;
#13784=CARTESIAN_POINT ( 'NONE',  ( 153.3040265531850537, 0.000000000000000000, 165.0000000000000000 ) ) ;
#13786=ORIENTED_EDGE ( 'NONE', *, *, #41008, .F. ) ;
#13789=ORIENTED_EDGE ( 'NONE', *, *, #29996, .T. ) ;
#13790=CARTESIAN_POINT ( 'NONE',  ( 153.3040265531850537, -1.750000000000010658, -119.1817124430720440 ) ) ;
#13793=CYLINDRICAL_SURFACE ( 'NONE', #34015, 1.750000000000008438 ) ;
#13802=CARTESIAN_POINT ( 'NONE',  ( -168.4459734468149463, 0.000000000000000000, 42.56828755692798438 ) ) ;
#13804=ORIENTED_EDGE ( 'NONE', *, *, #6040, .T. ) ;
#13810=FACE_OUTER_BOUND ( 'NONE', #40579, .T. ) ;
#13819=CARTESIAN_POINT ( 'NONE',  ( 151.5540265531850537, 2.143131898507880377E-16, -160.9317124430720298 ) ) ;
#13822=LINE ( 'NONE', #6145, #31560 ) ;
#13824=DIRECTION ( 'NONE',  ( -1.000000000000000000, -0.000000000000000000, -0.000000000000000000 ) ) ;
#13826=ORIENTED_EDGE ( 'NONE', *, *, #27439, .F. ) ;
#13827=CARTESIAN_POINT ( 'NONE',  ( 35.05402655318504657, 1.025126265847089213, -0.9317124430720324924 ) ) ;
#13828=CYLINDRICAL_SURFACE ( 'NONE', #19367, 1.750000000000001554 ) ;
#13840=CARTESIAN_POINT ( 'NONE',  ( -46.69597344681494633, 0.000000000000000000, 165.0000000000000000 ) ) ;
#13842=CARTESIAN_POINT ( 'NONE',  ( -206.6959734468149463, 1.750000000000010658, 80.81828755692798438 ) ) ;
#13845=CARTESIAN_POINT ( 'NONE',  ( -47.72109971266203132, 1.750000000000010436, 79.79316129108087807 ) ) ;
#13846=AXIS2_PLACEMENT_3D ( 'NONE', #21944, #37616, #2445 ) ;
#13852=LINE ( 'NONE', #14111, #4119 ) ;
#13854=CARTESIAN_POINT ( 'NONE',  ( 75.05402655318509630, 2.143131898507880377E-16, 119.0682875569279560 ) ) ;
#13856=( BOUNDED_CURVE ( )  B_SPLINE_CURVE ( 3, ( #13898, #49519, #45685, #37303 ),
 .UNSPECIFIED., .F., .F. ) 
 B_SPLINE_CURVE_WITH_KNOTS ( ( 4, 4 ),
 ( 3.141592653589793116, 4.712388980384689674 ),
 .UNSPECIFIED. ) 
 CURVE ( )  GEOMETRIC_REPRESENTATION_ITEM ( )  RATIONAL_B_SPLINE_CURVE ( ( 1.000000000000000000, 0.8047378541243649375, 0.8047378541243649375, 1.000000000000000000 ) ) 
 REPRESENTATION_ITEM ( '' )  );
#13857=DIRECTION ( 'NONE',  ( -1.000000000000000000, -0.000000000000000000, -0.000000000000000000 ) ) ;
#13859=CARTESIAN_POINT ( 'NONE',  ( 210.0000000000000568, 2.143131898507880377E-16, -160.9317124430720298 ) ) ;
#13864=( BOUNDED_CURVE ( )  B_SPLINE_CURVE ( 3, ( #25655, #30506, #45115, #14597 ),
 .UNSPECIFIED., .F., .F. ) 
 B_SPLINE_CURVE_WITH_KNOTS ( ( 4, 4 ),
 ( 4.712388980384689674, 6.283185307179586232 ),
 .UNSPECIFIED. ) 
 CURVE ( )  GEOMETRIC_REPRESENTATION_ITEM ( )  RATIONAL_B_SPLINE_CURVE ( ( 1.000000000000000000, 0.8047378541243649375, 0.8047378541243649375, 1.000000000000000000 ) ) 
 REPRESENTATION_ITEM ( '' )  );
#13866=ORIENTED_EDGE ( 'NONE', *, *, #30254, .T. ) ;
#13872=CARTESIAN_POINT ( 'NONE',  ( 114.3291528190321173, -1.749999999999996669, 81.84341382277506227 ) ) ;
#13873=LINE ( 'NONE', #37026, #1868 ) ;
#13875=CARTESIAN_POINT ( 'NONE',  ( -168.4459734468149463, 0.000000000000000000, -37.43171244307205825 ) ) ;
#13876=VECTOR ( 'NONE', #9480, 1000.000000000000000 ) ;
#13878=CARTESIAN_POINT ( 'NONE',  ( 71.55402655318506788, 2.143131898507880377E-16, -160.9317124430720298 ) ) ;
#13888=EDGE_LOOP ( 'NONE', ( #32093, #6282, #12542, #13896, #963, #8091 ) ) ;
#13889=CARTESIAN_POINT ( 'NONE',  ( -45.67084718096785423, -1.750000000000009548, 41.84341382277508359 ) ) ;
#13893=ORIENTED_EDGE ( 'NONE', *, *, #28193, .T. ) ;
#13896=ORIENTED_EDGE ( 'NONE', *, *, #2030, .F. ) ;
#13898=CARTESIAN_POINT ( 'NONE',  ( 195.0540265531851105, 2.143131898507880377E-16, -117.4317124430720725 ) ) ;
#13899=CARTESIAN_POINT ( 'NONE',  ( 210.0000000000000568, 0.000000000000000000, -159.1817124430720298 ) ) ;
#13901=FACE_OUTER_BOUND ( 'NONE', #27817, .T. ) ;
#13903=LINE ( 'NONE', #33688, #12528 ) ;
#13905=CARTESIAN_POINT ( 'NONE',  ( 74.32915281903215998, -1.750000000000009548, 39.79316129108089228 ) ) ;
#13909=AXIS2_PLACEMENT_3D ( 'NONE', #40446, #5283, #48591 ) ;
#13920=EDGE_CURVE ( 'NONE', #25110, #40222, #8796, .T. ) ;
#13929=DIRECTION ( 'NONE',  ( 0.000000000000000000, 0.000000000000000000, 1.000000000000000000 ) ) ;
#13930=EDGE_CURVE ( 'NONE', #25904, #40604, #17320, .T. ) ;
#13931=ORIENTED_EDGE ( 'NONE', *, *, #33839, .T. ) ;
#13932=ORIENTED_EDGE ( 'NONE', *, *, #32620, .T. ) ;
#13934=CARTESIAN_POINT ( 'NONE',  ( -128.4459734468149179, 0.000000000000000000, 165.0000000000000000 ) ) ;
#13937=CARTESIAN_POINT ( 'NONE',  ( -84.94597344681493212, -1.025126265847089435, -40.93171244307204404 ) ) ;
#13939=CARTESIAN_POINT ( 'NONE',  ( 33.30402655318503946, 1.750000000000009992, 160.8182875569279702 ) ) ;
#13941=EDGE_LOOP ( 'NONE', ( #9778, #7947 ) ) ;
#13942=DIRECTION ( 'NONE',  ( 0.000000000000000000, 0.000000000000000000, 1.000000000000000000 ) ) ;
#13944=EDGE_CURVE ( 'NONE', #8857, #47433, #43536, .T. ) ;
#13949=EDGE_CURVE ( 'NONE', #42411, #21262, #18950, .T. ) ;
#13950=ADVANCED_FACE ( 'NONE', ( #34155 ), #2077, .T. ) ;
#13951=ORIENTED_EDGE ( 'NONE', *, *, #40394, .F. ) ;
#13956=VECTOR ( 'NONE', #36595, 1000.000000000000000 ) ;
#13962=DIRECTION ( 'NONE',  ( -0.000000000000000000, -0.000000000000000000, -1.000000000000000000 ) ) ;
#13965=FACE_OUTER_BOUND ( 'NONE', #24128, .T. ) ;
#13966=CARTESIAN_POINT ( 'NONE',  ( 113.3040265531850537, -1.749999999999997335, 120.8182875569279702 ) ) ;
#13972=CARTESIAN_POINT ( 'NONE',  ( -208.4459734468149463, 0.000000000000000000, -80.93171244307201562 ) ) ;
#13973=CARTESIAN_POINT ( 'NONE',  ( 155.0540265531850537, -1.025126265847089435, 162.5682875569279133 ) ) ;
#13974=CARTESIAN_POINT ( 'NONE',  ( -164.9459734468149463, -1.025126265847089435, 122.5682875569280128 ) ) ;
#13977=FACE_OUTER_BOUND ( 'NONE', #8044, .T. ) ;
#13980=CARTESIAN_POINT ( 'NONE',  ( 210.0000000000000568, 0.000000000000000000, 2.568287556927987048 ) ) ;
#13983=VERTEX_POINT ( 'NONE', #18469 ) ;
#13985=EDGE_CURVE ( 'NONE', #29337, #39755, #22319, .T. ) ;
#13996=FACE_OUTER_BOUND ( 'NONE', #10047, .T. ) ;
#13998=CARTESIAN_POINT ( 'NONE',  ( 75.05402655318509630, 1.025126265847089435, 39.06828755692797728 ) ) ;
#13999=ORIENTED_EDGE ( 'NONE', *, *, #11102, .T. ) ;
#14002=VERTEX_POINT ( 'NONE', #42068 ) ;
#14003=ORIENTED_EDGE ( 'NONE', *, *, #31058, .T. ) ;
#14008=( BOUNDED_CURVE ( )  B_SPLINE_CURVE ( 3, ( #26454, #26716, #22606, #22098 ),
 .UNSPECIFIED., .F., .F. ) 
 B_SPLINE_CURVE_WITH_KNOTS ( ( 4, 4 ),
 ( 0.000000000000000000, 1.570796326794896558 ),
 .UNSPECIFIED. ) 
 CURVE ( )  GEOMETRIC_REPRESENTATION_ITEM ( )  RATIONAL_B_SPLINE_CURVE ( ( 1.000000000000000000, 0.8047378541243649375, 0.8047378541243649375, 1.000000000000000000 ) ) 
 REPRESENTATION_ITEM ( '' )  );
#14010=CARTESIAN_POINT ( 'NONE',  ( -168.4459734468149463, 0.000000000000000000, -37.43171244307205825 ) ) ;
#14015=VERTEX_POINT ( 'NONE', #37501 ) ;
#14017=( BOUNDED_CURVE ( )  B_SPLINE_CURVE ( 3, ( #27904, #39959, #27649, #46843 ),
 .UNSPECIFIED., .F., .F. ) 
 B_SPLINE_CURVE_WITH_KNOTS ( ( 4, 4 ),
 ( 3.141592653589793116, 4.712388980384689674 ),
 .UNSPECIFIED. ) 
 CURVE ( )  GEOMETRIC_REPRESENTATION_ITEM ( )  RATIONAL_B_SPLINE_CURVE ( ( 1.000000000000000000, 0.8047378541243649375, 0.8047378541243649375, 1.000000000000000000 ) ) 
 REPRESENTATION_ITEM ( '' )  );
#14020=ORIENTED_EDGE ( 'NONE', *, *, #20481, .F. ) ;
#14022=DIRECTION ( 'NONE',  ( -0.000000000000000000, -0.000000000000000000, -1.000000000000000000 ) ) ;
#14024=CARTESIAN_POINT ( 'NONE',  ( -46.69597344681494633, -1.750000000000009992, -159.1817124430720298 ) ) ;
#14025=LINE ( 'NONE', #41741, #30654 ) ;
#14030=( BOUNDED_CURVE ( )  B_SPLINE_CURVE ( 3, ( #20652, #19887, #15790, #8103 ),
 .UNSPECIFIED., .F., .F. ) 
 B_SPLINE_CURVE_WITH_KNOTS ( ( 4, 4 ),
 ( 3.141592653589793116, 4.712388980384689674 ),
 .UNSPECIFIED. ) 
 CURVE ( )  GEOMETRIC_REPRESENTATION_ITEM ( )  RATIONAL_B_SPLINE_CURVE ( ( 1.000000000000000000, 0.8047378541243649375, 0.8047378541243649375, 1.000000000000000000 ) ) 
 REPRESENTATION_ITEM ( '' )  );
#14031=AXIS2_PLACEMENT_3D ( 'NONE', #50552, #26997, #38574 ) ;
#14032=CARTESIAN_POINT ( 'NONE',  ( -168.4459734468149747, 1.025126265847089213, -0.9317124430720324924 ) ) ;
#14035=ORIENTED_EDGE ( 'NONE', *, *, #9205, .T. ) ;
#14040=CARTESIAN_POINT ( 'NONE',  ( 32.27890028733795447, 1.750000000000010436, -80.20683870891910772 ) ) ;
#14043=CARTESIAN_POINT ( 'NONE',  ( -48.44597344681492501, 0.000000000000000000, 162.5682875569279702 ) ) ;
#14045=CARTESIAN_POINT ( 'NONE',  ( -46.69597344681494633, -1.750000000000010214, 40.81828755692798438 ) ) ;
#14046=CARTESIAN_POINT ( 'NONE',  ( 113.3040265531850537, 0.000000000000000000, 165.0000000000000000 ) ) ;
#14047=CARTESIAN_POINT ( 'NONE',  ( 73.30402655318508209, 0.000000000000000000, 165.0000000000000000 ) ) ;
#14048=CYLINDRICAL_SURFACE ( 'NONE', #25006, 1.749999999999973799 ) ;
#14052=ORIENTED_EDGE ( 'NONE', *, *, #8629, .T. ) ;
#14060=VECTOR ( 'NONE', #12590, 1000.000000000000000 ) ;
#14062=DIRECTION ( 'NONE',  ( 0.000000000000000000, 0.000000000000000000, 1.000000000000000000 ) ) ;
#14063=ORIENTED_EDGE ( 'NONE', *, *, #26843, .T. ) ;
#14064=CARTESIAN_POINT ( 'NONE',  ( 155.0540265531850537, -1.025126265847089657, 79.06828755692797017 ) ) ;
#14065=EDGE_CURVE ( 'NONE', #10600, #17731, #39513, .T. ) ;
#14074=ORIENTED_EDGE ( 'NONE', *, *, #5253, .F. ) ;
#14077=VERTEX_POINT ( 'NONE', #7188 ) ;
#14079=EDGE_LOOP ( 'NONE', ( #3321, #31110 ) ) ;
#14086=PLANE ( 'NONE',  #45624 ) ;
#14089=CARTESIAN_POINT ( 'NONE',  ( 152.2789002873379900, -1.750000000000010214, -80.20683870891910772 ) ) ;
#14091=DIRECTION ( 'NONE',  ( -1.000000000000000000, -0.000000000000000000, -0.000000000000000000 ) ) ;
#14094=ORIENTED_EDGE ( 'NONE', *, *, #27370, .T. ) ;
#14095=LINE ( 'NONE', #10754, #27371 ) ;
#14101=CARTESIAN_POINT ( 'NONE',  ( 73.30402655318508209, 0.000000000000000000, 165.0000000000000000 ) ) ;
#14104=CARTESIAN_POINT ( 'NONE',  ( 210.0000000000000568, 0.000000000000000000, 120.8182875569279702 ) ) ;
#14106=EDGE_LOOP ( 'NONE', ( #19858, #28986, #37562, #9621, #1656, #38329 ) ) ;
#14107=CARTESIAN_POINT ( 'NONE',  ( 210.0000000000000568, 0.000000000000000000, -77.43171244307200141 ) ) ;
#14111=CARTESIAN_POINT ( 'NONE',  ( 210.0000000000000568, 0.000000000000000000, 162.5682875569279702 ) ) ;
#14114=CARTESIAN_POINT ( 'NONE',  ( -4.945973446814916130, 1.025126265847097429, -80.93171244307204404 ) ) ;
#14115=ORIENTED_EDGE ( 'NONE', *, *, #29082, .F. ) ;
#14116=DIRECTION ( 'NONE',  ( -0.000000000000000000, -0.000000000000000000, -1.000000000000000000 ) ) ;
#14117=ORIENTED_EDGE ( 'NONE', *, *, #42448, .T. ) ;
#14122=DIRECTION ( 'NONE',  ( -0.000000000000000000, -0.000000000000000000, -1.000000000000000000 ) ) ;
#14125=CARTESIAN_POINT ( 'NONE',  ( 210.0000000000000568, 2.143131898507881116E-16, -40.93171244307203693 ) ) ;
#14128=DIRECTION ( 'NONE',  ( 0.000000000000000000, 0.000000000000000000, 1.000000000000000000 ) ) ;
#14130=VECTOR ( 'NONE', #41876, 1000.000000000000000 ) ;
#14132=DIRECTION ( 'NONE',  ( 0.000000000000000000, 0.000000000000000000, 1.000000000000000000 ) ) ;
#14136=ORIENTED_EDGE ( 'NONE', *, *, #36268, .F. ) ;
#14139=CARTESIAN_POINT ( 'NONE',  ( 32.27890028733795447, 1.750000000000009548, -118.1565861772249519 ) ) ;
#14142=VERTEX_POINT ( 'NONE', #50488 ) ;
#14145=CARTESIAN_POINT ( 'NONE',  ( 210.0000000000000568, 0.000000000000000000, -77.43171244307200141 ) ) ;
#14148=ORIENTED_EDGE ( 'NONE', *, *, #9050, .F. ) ;
#14151=EDGE_LOOP ( 'NONE', ( #46547, #5274, #31066, #22344, #4899 ) ) ;
#14157=CARTESIAN_POINT ( 'NONE',  ( 31.55402655318503236, 0.000000000000000000, 82.56828755692798438 ) ) ;
#14159=CARTESIAN_POINT ( 'NONE',  ( -6.695973446814940111, -1.750000000000023759, 40.81828755692798438 ) ) ;
#14164=CARTESIAN_POINT ( 'NONE',  ( -88.44597344681497475, 0.000000000000000000, 42.56828755692799859 ) ) ;
#14166=CARTESIAN_POINT ( 'NONE',  ( -46.69597344681494633, 0.000000000000000000, 165.0000000000000000 ) ) ;
#14168=CARTESIAN_POINT ( 'NONE',  ( 111.5540265531850679, 0.000000000000000000, 165.0000000000000000 ) ) ;
#14179=EDGE_CURVE ( 'NONE', #47386, #26837, #48744, .T. ) ;
#14182=CARTESIAN_POINT ( 'NONE',  ( -207.7210997126620384, -1.750000000000009548, 161.8434138227750907 ) ) ;
#14193=CARTESIAN_POINT ( 'NONE',  ( 114.3291528190321173, -1.749999999999996225, -158.1565861772249377 ) ) ;
#14199=CARTESIAN_POINT ( 'NONE',  ( -6.695973446814940111, -1.750000000000023759, -39.18171244307202983 ) ) ;
#14200=EDGE_CURVE ( 'NONE', #8390, #15732, #3210, .T. ) ;
#14206=ORIENTED_EDGE ( 'NONE', *, *, #23297, .F. ) ;
#14209=ADVANCED_FACE ( 'NONE', ( #31815 ), #25113, .F. ) ;
#14210=EDGE_LOOP ( 'NONE', ( #33498, #358, #9588, #8683, #46131 ) ) ;
#14212=CARTESIAN_POINT ( 'NONE',  ( -8.445973446814976526, 0.000000000000000000, -157.4317124430720014 ) ) ;
#14215=EDGE_CURVE ( 'NONE', #936, #45355, #24232, .T. ) ;
#14216=FACE_OUTER_BOUND ( 'NONE', #29720, .T. ) ;
#14217=PLANE ( 'NONE',  #38345 ) ;
#14220=VECTOR ( 'NONE', #7035, 1000.000000000000000 ) ;
#14223=CARTESIAN_POINT ( 'NONE',  ( -164.9459734468149463, 2.143131898507880377E-16, 82.56828755692798438 ) ) ;
#14226=CARTESIAN_POINT ( 'NONE',  ( -164.9459734468149463, 2.143131898507880377E-16, 122.5682875569279702 ) ) ;
#14228=CYLINDRICAL_SURFACE ( 'NONE', #49368, 1.750000000000001554 ) ;
#14230=AXIS2_PLACEMENT_3D ( 'NONE', #34924, #43102, #31830 ) ;
#14235=CARTESIAN_POINT ( 'NONE',  ( -6.695973446814940111, -1.750000000000023759, -39.18171244307202983 ) ) ;
#14239=EDGE_CURVE ( 'NONE', #7572, #8778, #8459, .T. ) ;
#14255=CARTESIAN_POINT ( 'NONE',  ( 194.3291528190321742, 1.750000000000009548, -38.15658617722494483 ) ) ;
#14256=( BOUNDED_CURVE ( )  B_SPLINE_CURVE ( 3, ( #41454, #17846, #10408, #25553 ),
 .UNSPECIFIED., .F., .F. ) 
 B_SPLINE_CURVE_WITH_KNOTS ( ( 4, 4 ),
 ( 3.141592653589793116, 4.712388980384689674 ),
 .UNSPECIFIED. ) 
 CURVE ( )  GEOMETRIC_REPRESENTATION_ITEM ( )  RATIONAL_B_SPLINE_CURVE ( ( 1.000000000000000000, 0.8047378541243649375, 0.8047378541243649375, 1.000000000000000000 ) ) 
 REPRESENTATION_ITEM ( '' )  );
#14257=ORIENTED_EDGE ( 'NONE', *, *, #36242, .F. ) ;
#14260=EDGE_CURVE ( 'NONE', #13781, #29572, #45028, .T. ) ;
#14264=ORIENTED_EDGE ( 'NONE', *, *, #9132, .T. ) ;
#14266=FACE_OUTER_BOUND ( 'NONE', #23228, .T. ) ;
#14272=CARTESIAN_POINT ( 'NONE',  ( 113.3040265531850537, -1.749999999999997113, -39.18171244307202983 ) ) ;
#14276=CARTESIAN_POINT ( 'NONE',  ( 210.0000000000000568, 2.143131898507880377E-16, -0.9317124430720331585 ) ) ;
#14291=AXIS2_PLACEMENT_3D ( 'NONE', #37798, #49017, #49773 ) ;
#14299=DIRECTION ( 'NONE',  ( -0.000000000000000000, -0.000000000000000000, -1.000000000000000000 ) ) ;
#14306=DIRECTION ( 'NONE',  ( -1.000000000000000000, 0.000000000000000000, 0.000000000000000000 ) ) ;
#14310=ORIENTED_EDGE ( 'NONE', *, *, #35069, .T. ) ;
#14313=CARTESIAN_POINT ( 'NONE',  ( -88.44597344681497475, 0.000000000000000000, -37.43171244307200141 ) ) ;
#14314=( BOUNDED_CURVE ( )  B_SPLINE_CURVE ( 3, ( #16534, #17030, #39632, #4471 ),
 .UNSPECIFIED., .F., .F. ) 
 B_SPLINE_CURVE_WITH_KNOTS ( ( 4, 4 ),
 ( 4.712388980384689674, 6.283185307179586232 ),
 .UNSPECIFIED. ) 
 CURVE ( )  GEOMETRIC_REPRESENTATION_ITEM ( )  RATIONAL_B_SPLINE_CURVE ( ( 1.000000000000000000, 0.8047378541243649375, 0.8047378541243649375, 1.000000000000000000 ) ) 
 REPRESENTATION_ITEM ( '' )  );
#14320=ADVANCED_FACE ( 'NONE', ( #17891 ), #10706, .T. ) ;
#14321=CARTESIAN_POINT ( 'NONE',  ( 75.05402655318509630, 2.143131898507880377E-16, -0.9317124430720524764 ) ) ;
#14322=( BOUNDED_CURVE ( )  B_SPLINE_CURVE ( 3, ( #4343, #24103, #43320, #4595 ),
 .UNSPECIFIED., .F., .F. ) 
 B_SPLINE_CURVE_WITH_KNOTS ( ( 4, 4 ),
 ( 4.712388980384689674, 6.283185307179586232 ),
 .UNSPECIFIED. ) 
 CURVE ( )  GEOMETRIC_REPRESENTATION_ITEM ( )  RATIONAL_B_SPLINE_CURVE ( ( 1.000000000000000000, 0.8047378541243649375, 0.8047378541243649375, 1.000000000000000000 ) ) 
 REPRESENTATION_ITEM ( '' )  );
#14323=LINE ( 'NONE', #3022, #39105 ) ;
#14326=FACE_OUTER_BOUND ( 'NONE', #35509, .T. ) ;
#14339=FACE_OUTER_BOUND ( 'NONE', #41399, .T. ) ;
#14340=CARTESIAN_POINT ( 'NONE',  ( 33.30402655318503946, 1.750000000000009992, 160.8182875569279702 ) ) ;
#14344=CARTESIAN_POINT ( 'NONE',  ( 115.0540265531850395, 2.143131898507847836E-16, 119.0682875569279844 ) ) ;
#14346=EDGE_LOOP ( 'NONE', ( #31218, #14772, #24561, #22270, #46906, #10888 ) ) ;
#14355=ADVANCED_FACE ( 'NONE', ( #29710 ), #25614, .T. ) ;
#14358=CARTESIAN_POINT ( 'NONE',  ( 71.55402655318505367, 0.000000000000000000, 165.0000000000000000 ) ) ;
#14370=ORIENTED_EDGE ( 'NONE', *, *, #9613, .T. ) ;
#14372=DIRECTION ( 'NONE',  ( -0.000000000000000000, -0.000000000000000000, -1.000000000000000000 ) ) ;
#14380=ORIENTED_EDGE ( 'NONE', *, *, #24389, .T. ) ;
#14381=ORIENTED_EDGE ( 'NONE', *, *, #21460, .F. ) ;
#14382=AXIS2_PLACEMENT_3D ( 'NONE', #12585, #35966, #809 ) ;
#14386=VECTOR ( 'NONE', #16132, 1000.000000000000000 ) ;
#14387=DIRECTION ( 'NONE',  ( 0.000000000000000000, 0.000000000000000000, 1.000000000000000000 ) ) ;
#14391=FACE_OUTER_BOUND ( 'NONE', #24777, .T. ) ;
#14396=EDGE_CURVE ( 'NONE', #24760, #30683, #40996, .T. ) ;
#14401=CARTESIAN_POINT ( 'NONE',  ( 152.2789002873379900, -1.750000000000010214, -120.2068387089191219 ) ) ;
#14408=EDGE_CURVE ( 'NONE', #7516, #38646, #28559, .T. ) ;
#14410=ORIENTED_EDGE ( 'NONE', *, *, #15637, .F. ) ;
#14412=CARTESIAN_POINT ( 'NONE',  ( 115.0540265531850395, 2.143131898507847836E-16, 2.568287556927950632 ) ) ;
#14422=DIRECTION ( 'NONE',  ( -0.000000000000000000, -0.000000000000000000, -1.000000000000000000 ) ) ;
#14423=CARTESIAN_POINT ( 'NONE',  ( 154.3291528190321458, 1.750000000000009548, 1.843413822775065825 ) ) ;
#14426=CARTESIAN_POINT ( 'NONE',  ( 191.5540265531851105, 0.000000000000000000, 119.0682875569279702 ) ) ;
#14429=ORIENTED_EDGE ( 'NONE', *, *, #4628, .F. ) ;
#14430=EDGE_CURVE ( 'NONE', #36214, #8241, #11472, .T. ) ;
#14439=CYLINDRICAL_SURFACE ( 'NONE', #13162, 1.750000000000001554 ) ;
#14440=LINE ( 'NONE', #10349, #7739 ) ;
#14443=AXIS2_PLACEMENT_3D ( 'NONE', #50313, #10856, #42910 ) ;
#14444=AXIS2_PLACEMENT_3D ( 'NONE', #7725, #23364, #35945 ) ;
#14451=ORIENTED_EDGE ( 'NONE', *, *, #40735, .T. ) ;
#14453=CARTESIAN_POINT ( 'NONE',  ( -44.94597344681493922, 2.143131898507880377E-16, 165.0000000000000000 ) ) ;
#14454=EDGE_CURVE ( 'NONE', #23796, #36589, #4287, .T. ) ;
#14458=CARTESIAN_POINT ( 'NONE',  ( -86.69597344681494633, 1.750000000000010658, -79.18171244307201562 ) ) ;
#14464=ORIENTED_EDGE ( 'NONE', *, *, #18350, .F. ) ;
#14469=ORIENTED_EDGE ( 'NONE', *, *, #42131, .F. ) ;
#14470=ORIENTED_EDGE ( 'NONE', *, *, #40472, .T. ) ;
#14471=CARTESIAN_POINT ( 'NONE',  ( 210.0000000000000568, 0.000000000000000000, -117.4317124430720298 ) ) ;
#14472=CARTESIAN_POINT ( 'NONE',  ( 155.0540265531850537, 2.143131898507880377E-16, 165.0000000000000000 ) ) ;
#14474=CYLINDRICAL_SURFACE ( 'NONE', #46032, 1.750000000000015543 ) ;
#14480=CARTESIAN_POINT ( 'NONE',  ( 115.0540265531850395, -1.025126265847081886, 119.0682875569279702 ) ) ;
#14484=CARTESIAN_POINT ( 'NONE',  ( 33.30402655318503946, 1.750000000000010658, -79.18171244307201562 ) ) ;
#14487=CARTESIAN_POINT ( 'NONE',  ( 210.0000000000000568, 0.000000000000000000, 160.8182875569279702 ) ) ;
#14489=( BOUNDED_CURVE ( )  B_SPLINE_CURVE ( 3, ( #43658, #4918, #31645, #11875 ),
 .UNSPECIFIED., .F., .F. ) 
 B_SPLINE_CURVE_WITH_KNOTS ( ( 4, 4 ),
 ( 4.712388980384689674, 6.283185307179586232 ),
 .UNSPECIFIED. ) 
 CURVE ( )  GEOMETRIC_REPRESENTATION_ITEM ( )  RATIONAL_B_SPLINE_CURVE ( ( 1.000000000000000000, 0.8047378541243649375, 0.8047378541243649375, 1.000000000000000000 ) ) 
 REPRESENTATION_ITEM ( '' )  );
#14490=CARTESIAN_POINT ( 'NONE',  ( -166.6959734468149463, 1.750000000000009992, -159.1817124430720298 ) ) ;
#14491=LINE ( 'NONE', #10637, #36575 ) ;
#14493=DIRECTION ( 'NONE',  ( 0.000000000000000000, 0.000000000000000000, 1.000000000000000000 ) ) ;
#14494=CARTESIAN_POINT ( 'NONE',  ( 115.0540265531850395, -1.025126265847081442, -0.9317124430720195027 ) ) ;
#14506=VERTEX_POINT ( 'NONE', #34320 ) ;
#14514=CARTESIAN_POINT ( 'NONE',  ( 33.30402655318503946, 1.750000000000009992, 0.8182875569279768335 ) ) ;
#14516=ORIENTED_EDGE ( 'NONE', *, *, #27381, .T. ) ;
#14522=CYLINDRICAL_SURFACE ( 'NONE', #30062, 1.750000000000010214 ) ;
#14525=VERTEX_POINT ( 'NONE', #7125 ) ;
#14530=CARTESIAN_POINT ( 'NONE',  ( 210.0000000000000568, 0.000000000000000000, -119.1817124430720440 ) ) ;
#14531=CARTESIAN_POINT ( 'NONE',  ( 152.2789002873379900, 1.750000000000010436, -120.2068387089191219 ) ) ;
#14533=CARTESIAN_POINT ( 'NONE',  ( -5.670847180967843570, 1.750000000000023537, 121.8434138227750623 ) ) ;
#14540=DIRECTION ( 'NONE',  ( -0.000000000000000000, -0.000000000000000000, -1.000000000000000000 ) ) ;
#14541=CARTESIAN_POINT ( 'NONE',  ( -46.69597344681494633, 1.750000000000009992, -159.1817124430720298 ) ) ;
#14542=FACE_OUTER_BOUND ( 'NONE', #47913, .T. ) ;
#14546=CARTESIAN_POINT ( 'NONE',  ( 210.0000000000000568, 0.000000000000000000, -119.1817124430720440 ) ) ;
#14548=FACE_OUTER_BOUND ( 'NONE', #7606, .T. ) ;
#14550=CARTESIAN_POINT ( 'NONE',  ( 153.3040265531850537, 1.750000000000010658, -119.1817124430720440 ) ) ;
#14554=( BOUNDED_CURVE ( )  B_SPLINE_CURVE ( 3, ( #19809, #31889, #24688, #24439 ),
 .UNSPECIFIED., .F., .F. ) 
 B_SPLINE_CURVE_WITH_KNOTS ( ( 4, 4 ),
 ( 1.570796326794896558, 3.141592653589793116 ),
 .UNSPECIFIED. ) 
 CURVE ( )  GEOMETRIC_REPRESENTATION_ITEM ( )  RATIONAL_B_SPLINE_CURVE ( ( 1.000000000000000000, 0.8047378541243649375, 0.8047378541243649375, 1.000000000000000000 ) ) 
 REPRESENTATION_ITEM ( '' )  );
#14557=CYLINDRICAL_SURFACE ( 'NONE', #41833, 1.750000000000001554 ) ;
#14558=CARTESIAN_POINT ( 'NONE',  ( 31.55402655318503236, 0.000000000000000000, -37.43171244307200141 ) ) ;
#14561=VERTEX_POINT ( 'NONE', #11476 ) ;
#14563=EDGE_CURVE ( 'NONE', #40360, #559, #14731, .T. ) ;
#14565=ORIENTED_EDGE ( 'NONE', *, *, #18160, .T. ) ;
#14566=VERTEX_POINT ( 'NONE', #39703 ) ;
#14569=ADVANCED_FACE ( 'NONE', ( #39953 ), #1458, .T. ) ;
#14571=LINE ( 'NONE', #49429, #28646 ) ;
#14574=EDGE_CURVE ( 'NONE', #42421, #21654, #5919, .T. ) ;
#14576=EDGE_CURVE ( 'NONE', #6375, #40138, #27215, .T. ) ;
#14578=ORIENTED_EDGE ( 'NONE', *, *, #34416, .T. ) ;
#14580=CARTESIAN_POINT ( 'NONE',  ( 75.05402655318509630, 1.025126265847089435, 159.0682875569279418 ) ) ;
#14586=ORIENTED_EDGE ( 'NONE', *, *, #41387, .F. ) ;
#14597=CARTESIAN_POINT ( 'NONE',  ( 111.5540265531850679, 0.000000000000000000, 39.06828755692798438 ) ) ;
#14601=CARTESIAN_POINT ( 'NONE',  ( -124.9459734468149321, -1.025126265847081886, 79.06828755692797017 ) ) ;
#14608=CYLINDRICAL_SURFACE ( 'NONE', #4401, 1.750000000000008438 ) ;
#14612=EDGE_CURVE ( 'NONE', #48914, #4790, #16420, .T. ) ;
#14616=CARTESIAN_POINT ( 'NONE',  ( -88.44597344681494633, 1.025126265847089213, 162.5682875569279133 ) ) ;
#14617=( BOUNDED_CURVE ( )  B_SPLINE_CURVE ( 3, ( #28701, #36160, #25109, #40757 ),
 .UNSPECIFIED., .F., .F. ) 
 B_SPLINE_CURVE_WITH_KNOTS ( ( 4, 4 ),
 ( 3.141592653589793116, 4.712388980384689674 ),
 .UNSPECIFIED. ) 
 CURVE ( )  GEOMETRIC_REPRESENTATION_ITEM ( )  RATIONAL_B_SPLINE_CURVE ( ( 1.000000000000000000, 0.8047378541243649375, 0.8047378541243649375, 1.000000000000000000 ) ) 
 REPRESENTATION_ITEM ( '' )  );
#14618=ORIENTED_EDGE ( 'NONE', *, *, #39469, .F. ) ;
#14619=CARTESIAN_POINT ( 'NONE',  ( 155.0540265531850537, 2.143131898507880377E-16, -37.43171244307205825 ) ) ;
#14624=VERTEX_POINT ( 'NONE', #35860 ) ;
#14625=CARTESIAN_POINT ( 'NONE',  ( -6.695973446814940111, 0.000000000000000000, -165.0000000000000000 ) ) ;
#14627=( BOUNDED_CURVE ( )  B_SPLINE_CURVE ( 3, ( #34516, #11404, #47022, #382 ),
 .UNSPECIFIED., .F., .F. ) 
 B_SPLINE_CURVE_WITH_KNOTS ( ( 4, 4 ),
 ( 4.712388980384689674, 6.283185307179586232 ),
 .UNSPECIFIED. ) 
 CURVE ( )  GEOMETRIC_REPRESENTATION_ITEM ( )  RATIONAL_B_SPLINE_CURVE ( ( 1.000000000000000000, 0.8047378541243649375, 0.8047378541243649375, 1.000000000000000000 ) ) 
 REPRESENTATION_ITEM ( '' )  );
#14629=LINE ( 'NONE', #3580, #42075 ) ;
#14631=ORIENTED_EDGE ( 'NONE', *, *, #49627, .T. ) ;
#14637=CARTESIAN_POINT ( 'NONE',  ( -166.6959734468149463, -1.750000000000010658, 120.8182875569279702 ) ) ;
#14640=DIRECTION ( 'NONE',  ( -0.000000000000000000, -0.000000000000000000, -1.000000000000000000 ) ) ;
#14642=ADVANCED_FACE ( 'NONE', ( #32250 ), #28400, .T. ) ;
#14643=ORIENTED_EDGE ( 'NONE', *, *, #24692, .F. ) ;
#14647=ORIENTED_EDGE ( 'NONE', *, *, #1173, .T. ) ;
#14649=CYLINDRICAL_SURFACE ( 'NONE', #46058, 1.750000000000015543 ) ;
#14650=ORIENTED_EDGE ( 'NONE', *, *, #8680, .T. ) ;
#14652=DIRECTION ( 'NONE',  ( -1.000000000000000000, -0.000000000000000000, -0.000000000000000000 ) ) ;
#14654=CARTESIAN_POINT ( 'NONE',  ( -124.9459734468149321, -1.025126265847081664, -117.4317124430720440 ) ) ;
#14660=ORIENTED_EDGE ( 'NONE', *, *, #9599, .F. ) ;
#14661=CARTESIAN_POINT ( 'NONE',  ( -84.94597344681494633, 2.143131898507880377E-16, 82.56828755692798438 ) ) ;
#14666=AXIS2_PLACEMENT_3D ( 'NONE', #35718, #24407, #4875 ) ;
#14667=EDGE_LOOP ( 'NONE', ( #39976, #21218, #34390, #34231, #44832, #43367 ) ) ;
#14675=VERTEX_POINT ( 'NONE', #18093 ) ;
#14684=VERTEX_POINT ( 'NONE', #34018 ) ;
#14689=VECTOR ( 'NONE', #24537, 1000.000000000000000 ) ;
#14690=EDGE_CURVE ( 'NONE', #45274, #16704, #10151, .T. ) ;
#14693=DIRECTION ( 'NONE',  ( 1.000000000000000000, 0.000000000000000000, 0.000000000000000000 ) ) ;
#14698=CARTESIAN_POINT ( 'NONE',  ( -86.69597344681494633, -1.750000000000010658, 120.8182875569279702 ) ) ;
#14699=AXIS2_PLACEMENT_3D ( 'NONE', #34902, #7821, #42817 ) ;
#14708=ORIENTED_EDGE ( 'NONE', *, *, #49365, .T. ) ;
#14709=VERTEX_POINT ( 'NONE', #17595 ) ;
#14715=EDGE_CURVE ( 'NONE', #28470, #17971, #17844, .T. ) ;
#14719=CARTESIAN_POINT ( 'NONE',  ( 153.3040265531850537, 1.750000000000010658, -79.18171244307201562 ) ) ;
#14726=CARTESIAN_POINT ( 'NONE',  ( 35.05402655318504657, 2.143131898507880377E-16, 122.5682875569279702 ) ) ;
#14728=ORIENTED_EDGE ( 'NONE', *, *, #719, .T. ) ;
#14729=CARTESIAN_POINT ( 'NONE',  ( -8.445973446814914354, 2.143131898507880377E-16, -160.9317124430720298 ) ) ;
#14731=CIRCLE ( 'NONE', #43402, 1.750000000000008438 ) ;
#14734=CARTESIAN_POINT ( 'NONE',  ( 115.0540265531850395, 2.143131898507847836E-16, 119.0682875569279844 ) ) ;
#14737=AXIS2_PLACEMENT_3D ( 'NONE', #38570, #38058, #30348 ) ;
#14738=CARTESIAN_POINT ( 'NONE',  ( 32.27890028733795447, 1.750000000000009548, -78.15658617722490931 ) ) ;
#14740=CARTESIAN_POINT ( 'NONE',  ( -208.4459734468149463, 0.000000000000000000, 42.56828755692798438 ) ) ;
#14749=CARTESIAN_POINT ( 'NONE',  ( -210.0000000000000568, 0.000000000000000000, 160.8182875569279702 ) ) ;
#14757=LINE ( 'NONE', #46020, #44631 ) ;
#14764=( BOUNDED_CURVE ( )  B_SPLINE_CURVE ( 3, ( #17851, #18102, #34028, #33022 ),
 .UNSPECIFIED., .F., .F. ) 
 B_SPLINE_CURVE_WITH_KNOTS ( ( 4, 4 ),
 ( 4.712388980384689674, 6.283185307179586232 ),
 .UNSPECIFIED. ) 
 CURVE ( )  GEOMETRIC_REPRESENTATION_ITEM ( )  RATIONAL_B_SPLINE_CURVE ( ( 1.000000000000000000, 0.8047378541243649375, 0.8047378541243649375, 1.000000000000000000 ) ) 
 REPRESENTATION_ITEM ( '' )  );
#14767=VERTEX_POINT ( 'NONE', #11172 ) ;
#14768=CARTESIAN_POINT ( 'NONE',  ( -124.9459734468149463, 2.143131898507847836E-16, 82.56828755692797017 ) ) ;
#14772=ORIENTED_EDGE ( 'NONE', *, *, #37169, .T. ) ;
#14774=AXIS2_PLACEMENT_3D ( 'NONE', #23234, #18620, #38915 ) ;
#14775=( BOUNDED_CURVE ( )  B_SPLINE_CURVE ( 3, ( #11647, #3423, #35022, #19072 ),
 .UNSPECIFIED., .F., .F. ) 
 B_SPLINE_CURVE_WITH_KNOTS ( ( 4, 4 ),
 ( 0.000000000000000000, 1.570796326794896558 ),
 .UNSPECIFIED. ) 
 CURVE ( )  GEOMETRIC_REPRESENTATION_ITEM ( )  RATIONAL_B_SPLINE_CURVE ( ( 1.000000000000000000, 0.8047378541243649375, 0.8047378541243649375, 1.000000000000000000 ) ) 
 REPRESENTATION_ITEM ( '' )  );
#14776=ORIENTED_EDGE ( 'NONE', *, *, #39401, .T. ) ;
#14778=FACE_OUTER_BOUND ( 'NONE', #23548, .T. ) ;
#14781=FACE_OUTER_BOUND ( 'NONE', #30496, .T. ) ;
#14782=CARTESIAN_POINT ( 'NONE',  ( 32.27890028733795447, -1.750000000000010214, 81.84341382277507648 ) ) ;
#14786=CARTESIAN_POINT ( 'NONE',  ( 111.5540265531850679, 0.000000000000000000, 159.0682875569279702 ) ) ;
#14787=CARTESIAN_POINT ( 'NONE',  ( -126.6959734468149321, -1.749999999999996891, 160.8182875569279702 ) ) ;
#14788=( BOUNDED_CURVE ( )  B_SPLINE_CURVE ( 3, ( #49273, #36793, #49016, #41624 ),
 .UNSPECIFIED., .F., .F. ) 
 B_SPLINE_CURVE_WITH_KNOTS ( ( 4, 4 ),
 ( 4.712388980384689674, 6.283185307179586232 ),
 .UNSPECIFIED. ) 
 CURVE ( )  GEOMETRIC_REPRESENTATION_ITEM ( )  RATIONAL_B_SPLINE_CURVE ( ( 1.000000000000000000, 0.8047378541243649375, 0.8047378541243649375, 1.000000000000000000 ) ) 
 REPRESENTATION_ITEM ( '' )  );
#14789=CARTESIAN_POINT ( 'NONE',  ( 152.2789002873379900, -1.750000000000010214, 119.7931612910808781 ) ) ;
#14791=ORIENTED_EDGE ( 'NONE', *, *, #28995, .T. ) ;
#14793=CARTESIAN_POINT ( 'NONE',  ( 34.32915281903212446, 1.750000000000010214, -118.1565861772249519 ) ) ;
#14796=ORIENTED_EDGE ( 'NONE', *, *, #50042, .F. ) ;
#14802=CARTESIAN_POINT ( 'NONE',  ( -86.69597344681494633, 1.750000000000010658, -79.18171244307201562 ) ) ;
#14808=VECTOR ( 'NONE', #21001, 1000.000000000000000 ) ;
#14812=CARTESIAN_POINT ( 'NONE',  ( 115.0540265531850395, 2.143131898507847836E-16, 165.0000000000000000 ) ) ;
#14814=ORIENTED_EDGE ( 'NONE', *, *, #35565, .F. ) ;
#14819=ORIENTED_EDGE ( 'NONE', *, *, #39731, .T. ) ;
#14823=ORIENTED_EDGE ( 'NONE', *, *, #11590, .F. ) ;
#14827=FACE_OUTER_BOUND ( 'NONE', #16748, .T. ) ;
#14829=ADVANCED_FACE ( 'NONE', ( #7312 ), #46769, .T. ) ;
#14830=DIRECTION ( 'NONE',  ( -0.000000000000000000, -0.000000000000000000, -1.000000000000000000 ) ) ;
#14834=DIRECTION ( 'NONE',  ( -1.000000000000000000, -0.000000000000000000, -0.000000000000000000 ) ) ;
#14838=EDGE_CURVE ( 'NONE', #15868, #34290, #16716, .T. ) ;
#14840=ORIENTED_EDGE ( 'NONE', *, *, #40939, .F. ) ;
#14843=EDGE_LOOP ( 'NONE', ( #43942, #17241, #42924, #29425, #22482, #39673 ) ) ;
#14844=ORIENTED_EDGE ( 'NONE', *, *, #10830, .T. ) ;
#14847=AXIS2_PLACEMENT_3D ( 'NONE', #5928, #9529, #5174 ) ;
#14848=EDGE_CURVE ( 'NONE', #17123, #39145, #39661, .T. ) ;
#14850=VECTOR ( 'NONE', #1453, 1000.000000000000000 ) ;
#14852=LINE ( 'NONE', #30503, #27404 ) ;
#14854=ADVANCED_FACE ( 'NONE', ( #23483 ), #11416, .T. ) ;
#14858=CARTESIAN_POINT ( 'NONE',  ( 72.27890028733797578, -1.750000000000010214, 81.84341382277507648 ) ) ;
#14864=CARTESIAN_POINT ( 'NONE',  ( -88.44597344681497475, 0.000000000000000000, 165.0000000000000000 ) ) ;
#14868=EDGE_CURVE ( 'NONE', #13365, #14561, #44860, .T. ) ;
#14869=( BOUNDED_CURVE ( )  B_SPLINE_CURVE ( 3, ( #48109, #36647, #45033, #13244 ),
 .UNSPECIFIED., .F., .F. ) 
 B_SPLINE_CURVE_WITH_KNOTS ( ( 4, 4 ),
 ( 1.570796326794896558, 3.141592653589793116 ),
 .UNSPECIFIED. ) 
 CURVE ( )  GEOMETRIC_REPRESENTATION_ITEM ( )  RATIONAL_B_SPLINE_CURVE ( ( 1.000000000000000000, 0.8047378541243649375, 0.8047378541243649375, 1.000000000000000000 ) ) 
 REPRESENTATION_ITEM ( '' )  );
#14870=DIRECTION ( 'NONE',  ( 0.000000000000000000, 0.000000000000000000, 1.000000000000000000 ) ) ;
#14874=CARTESIAN_POINT ( 'NONE',  ( 210.0000000000000568, 0.000000000000000000, -159.1817124430720298 ) ) ;
#14881=CARTESIAN_POINT ( 'NONE',  ( 73.30402655318508209, 0.000000000000000000, 165.0000000000000000 ) ) ;
#14882=VERTEX_POINT ( 'NONE', #24241 ) ;
#14885=CARTESIAN_POINT ( 'NONE',  ( -8.445973446814976526, 0.000000000000000000, 42.56828755692802702 ) ) ;
#14886=VECTOR ( 'NONE', #34723, 1000.000000000000000 ) ;
#14889=ORIENTED_EDGE ( 'NONE', *, *, #19941, .T. ) ;
#14890=EDGE_CURVE ( 'NONE', #42480, #28309, #46198, .T. ) ;
#14892=VERTEX_POINT ( 'NONE', #47030 ) ;
#14898=CARTESIAN_POINT ( 'NONE',  ( 73.30402655318508209, 1.750000000000010658, 120.8182875569279702 ) ) ;
#14905=DIRECTION ( 'NONE',  ( 1.000000000000000000, 0.000000000000000000, 0.000000000000000000 ) ) ;
#14906=CARTESIAN_POINT ( 'NONE',  ( -6.695973446814940111, 1.750000000000024203, -79.18171244307201562 ) ) ;
#14907=ORIENTED_EDGE ( 'NONE', *, *, #25258, .F. ) ;
#14913=CARTESIAN_POINT ( 'NONE',  ( 210.0000000000000568, 0.000000000000000000, 120.8182875569279702 ) ) ;
#14923=ORIENTED_EDGE ( 'NONE', *, *, #5504, .T. ) ;
#14924=ORIENTED_EDGE ( 'NONE', *, *, #1173, .F. ) ;
#14925=CARTESIAN_POINT ( 'NONE',  ( -124.9459734468149321, -1.025126265847081664, 82.56828755692798438 ) ) ;
#14926=( BOUNDED_CURVE ( )  B_SPLINE_CURVE ( 3, ( #25888, #26123, #30484, #37695 ),
 .UNSPECIFIED., .F., .F. ) 
 B_SPLINE_CURVE_WITH_KNOTS ( ( 4, 4 ),
 ( 0.000000000000000000, 1.570796326794896558 ),
 .UNSPECIFIED. ) 
 CURVE ( )  GEOMETRIC_REPRESENTATION_ITEM ( )  RATIONAL_B_SPLINE_CURVE ( ( 1.000000000000000000, 0.8047378541243649375, 0.8047378541243649375, 1.000000000000000000 ) ) 
 REPRESENTATION_ITEM ( '' )  );
#14930=ADVANCED_FACE ( 'NONE', ( #43718 ), #21902, .T. ) ;
#14931=LINE ( 'NONE', #46189, #9428 ) ;
#14936=( BOUNDED_CURVE ( )  B_SPLINE_CURVE ( 3, ( #5554, #16349, #21203, #36895 ),
 .UNSPECIFIED., .F., .F. ) 
 B_SPLINE_CURVE_WITH_KNOTS ( ( 4, 4 ),
 ( 0.000000000000000000, 1.570796326794896558 ),
 .UNSPECIFIED. ) 
 CURVE ( )  GEOMETRIC_REPRESENTATION_ITEM ( )  RATIONAL_B_SPLINE_CURVE ( ( 1.000000000000000000, 0.8047378541243649375, 0.8047378541243649375, 1.000000000000000000 ) ) 
 REPRESENTATION_ITEM ( '' )  );
#14937=AXIS2_PLACEMENT_3D ( 'NONE', #31716, #32207, #4248 ) ;
#14943=ORIENTED_EDGE ( 'NONE', *, *, #29985, .T. ) ;
#14952=DIRECTION ( 'NONE',  ( -0.000000000000000000, -0.000000000000000000, -1.000000000000000000 ) ) ;
#14956=CARTESIAN_POINT ( 'NONE',  ( 75.05402655318509630, 2.143131898507880377E-16, 42.56828755692799859 ) ) ;
#14959=CARTESIAN_POINT ( 'NONE',  ( -208.4459734468149463, 0.000000000000000000, -0.9317124430720247208 ) ) ;
#14960=CARTESIAN_POINT ( 'NONE',  ( -4.945973446814938335, 0.000000000000000000, 162.5682875569279702 ) ) ;
#14962=ORIENTED_EDGE ( 'NONE', *, *, #44762, .T. ) ;
#14963=FACE_OUTER_BOUND ( 'NONE', #45504, .T. ) ;
#14967=LINE ( 'NONE', #23165, #39717 ) ;
#14969=ORIENTED_EDGE ( 'NONE', *, *, #23161, .F. ) ;
#14970=DIRECTION ( 'NONE',  ( -0.000000000000000000, -0.000000000000000000, -1.000000000000000000 ) ) ;
#14971=EDGE_LOOP ( 'NONE', ( #46730, #2668 ) ) ;
#14972=AXIS2_PLACEMENT_3D ( 'NONE', #28035, #43422, #12625 ) ;
#14974=FACE_OUTER_BOUND ( 'NONE', #47122, .T. ) ;
#14983=ORIENTED_EDGE ( 'NONE', *, *, #38823, .F. ) ;
#14985=ORIENTED_EDGE ( 'NONE', *, *, #49476, .T. ) ;
#14987=CARTESIAN_POINT ( 'NONE',  ( -166.6959734468149463, 1.750000000000010214, 40.81828755692798438 ) ) ;
#14998=CARTESIAN_POINT ( 'NONE',  ( -5.670847180967843570, -1.750000000000023981, 79.79316129108087807 ) ) ;
#14999=CARTESIAN_POINT ( 'NONE',  ( 32.27890028733795447, 1.750000000000009548, -160.2068387089191219 ) ) ;
#15022=VERTEX_POINT ( 'NONE', #14956 ) ;
#15023=AXIS2_PLACEMENT_3D ( 'NONE', #33129, #10010, #13603 ) ;
#15031=EDGE_CURVE ( 'NONE', #49578, #41405, #34988, .T. ) ;
#15040=ORIENTED_EDGE ( 'NONE', *, *, #6672, .F. ) ;
#15044=EDGE_LOOP ( 'NONE', ( #29479, #22470, #7680, #23232, #10777, #9956 ) ) ;
#15047=DIRECTION ( 'NONE',  ( -0.000000000000000000, -0.000000000000000000, -1.000000000000000000 ) ) ;
#15049=AXIS2_PLACEMENT_3D ( 'NONE', #1021, #16, #35932 ) ;
#15051=ORIENTED_EDGE ( 'NONE', *, *, #8629, .F. ) ;
#15053=AXIS2_PLACEMENT_3D ( 'NONE', #14546, #26095, #46062 ) ;
#15057=AXIS2_PLACEMENT_3D ( 'NONE', #20237, #8191, #23840 ) ;
#15058=LINE ( 'NONE', #39189, #16508 ) ;
#15062=EDGE_CURVE ( 'NONE', #40502, #46038, #13415, .T. ) ;
#15068=ORIENTED_EDGE ( 'NONE', *, *, #31474, .T. ) ;
#15070=VECTOR ( 'NONE', #6343, 1000.000000000000000 ) ;
#15075=LINE ( 'NONE', #29714, #27324 ) ;
#15077=( BOUNDED_CURVE ( )  B_SPLINE_CURVE ( 3, ( #33607, #49703, #34365, #9993 ),
 .UNSPECIFIED., .F., .F. ) 
 B_SPLINE_CURVE_WITH_KNOTS ( ( 4, 4 ),
 ( 3.141592653589793116, 4.712388980384689674 ),
 .UNSPECIFIED. ) 
 CURVE ( )  GEOMETRIC_REPRESENTATION_ITEM ( )  RATIONAL_B_SPLINE_CURVE ( ( 1.000000000000000000, 0.8047378541243649375, 0.8047378541243649375, 1.000000000000000000 ) ) 
 REPRESENTATION_ITEM ( '' )  );
#15082=CYLINDRICAL_SURFACE ( 'NONE', #60, 1.750000000000001554 ) ;
#15087=CARTESIAN_POINT ( 'NONE',  ( 155.0540265531850537, 2.143131898507880377E-16, 165.0000000000000000 ) ) ;
#15089=( BOUNDED_CURVE ( )  B_SPLINE_CURVE ( 3, ( #7337, #38649, #19384, #12629 ),
 .UNSPECIFIED., .F., .F. ) 
 B_SPLINE_CURVE_WITH_KNOTS ( ( 4, 4 ),
 ( 1.570796326794896558, 3.141592653589793116 ),
 .UNSPECIFIED. ) 
 CURVE ( )  GEOMETRIC_REPRESENTATION_ITEM ( )  RATIONAL_B_SPLINE_CURVE ( ( 1.000000000000000000, 0.8047378541243649375, 0.8047378541243649375, 1.000000000000000000 ) ) 
 REPRESENTATION_ITEM ( '' )  );
#15091=ORIENTED_EDGE ( 'NONE', *, *, #43970, .T. ) ;
#15092=VECTOR ( 'NONE', #25365, 1000.000000000000000 ) ;
#15095=CARTESIAN_POINT ( 'NONE',  ( 114.3291528190321173, -1.749999999999997113, -120.2068387089191219 ) ) ;
#15097=CARTESIAN_POINT ( 'NONE',  ( 153.3040265531850537, 1.750000000000010658, 120.8182875569279702 ) ) ;
#15099=ORIENTED_EDGE ( 'NONE', *, *, #30254, .F. ) ;
#15100=ORIENTED_EDGE ( 'NONE', *, *, #9599, .T. ) ;
#15102=CYLINDRICAL_SURFACE ( 'NONE', #26250, 1.750000000000001554 ) ;
#15113=CARTESIAN_POINT ( 'NONE',  ( 113.3040265531850537, -1.749999999999997113, -39.18171244307202983 ) ) ;
#15114=CARTESIAN_POINT ( 'NONE',  ( -124.9459734468149463, 2.143131898507847836E-16, 165.0000000000000000 ) ) ;
#15119=LINE ( 'NONE', #23061, #16767 ) ;
#15129=CARTESIAN_POINT ( 'NONE',  ( -47.72109971266203132, -1.750000000000010214, 121.8434138227750623 ) ) ;
#15131=CARTESIAN_POINT ( 'NONE',  ( 195.0540265531851105, -1.025126265847089435, 39.06828755692797728 ) ) ;
#15134=CARTESIAN_POINT ( 'NONE',  ( -124.9459734468149605, 0.000000000000000000, 162.5682875569279702 ) ) ;
#15135=EDGE_CURVE ( 'NONE', #43286, #14525, #42135, .T. ) ;
#15140=EDGE_CURVE ( 'NONE', #18077, #9162, #44553, .T. ) ;
#15143=VERTEX_POINT ( 'NONE', #19300 ) ;
#15144=CARTESIAN_POINT ( 'NONE',  ( 193.3040265531851105, 1.750000000000010658, 80.81828755692798438 ) ) ;
#15146=AXIS2_PLACEMENT_3D ( 'NONE', #16772, #1632, #32432 ) ;
#15149=CARTESIAN_POINT ( 'NONE',  ( -86.69597344681494633, -1.750000000000010658, -119.1817124430720440 ) ) ;
#15151=ORIENTED_EDGE ( 'NONE', *, *, #31834, .F. ) ;
#15152=ADVANCED_FACE ( 'NONE', ( #41894 ), #11615, .F. ) ;
#15153=ORIENTED_EDGE ( 'NONE', *, *, #9502, .T. ) ;
#15154=LINE ( 'NONE', #15411, #16085 ) ;
#15155=EDGE_CURVE ( 'NONE', #19177, #34969, #32476, .T. ) ;
#15159=ORIENTED_EDGE ( 'NONE', *, *, #113, .T. ) ;
#15160=CARTESIAN_POINT ( 'NONE',  ( 210.0000000000000568, 0.000000000000000000, 40.81828755692798438 ) ) ;
#15165=CARTESIAN_POINT ( 'NONE',  ( -6.695973446814940111, -1.750000000000024203, 80.81828755692798438 ) ) ;
#15173=( BOUNDED_CURVE ( )  B_SPLINE_CURVE ( 3, ( #30519, #45633, #34897, #35153 ),
 .UNSPECIFIED., .F., .F. ) 
 B_SPLINE_CURVE_WITH_KNOTS ( ( 4, 4 ),
 ( 3.141592653589793116, 4.712388980384689674 ),
 .UNSPECIFIED. ) 
 CURVE ( )  GEOMETRIC_REPRESENTATION_ITEM ( )  RATIONAL_B_SPLINE_CURVE ( ( 1.000000000000000000, 0.8047378541243649375, 0.8047378541243649375, 1.000000000000000000 ) ) 
 REPRESENTATION_ITEM ( '' )  );
#15178=ADVANCED_FACE ( 'NONE', ( #21264 ), #23916, .T. ) ;
#15181=LINE ( 'NONE', #11330, #31903 ) ;
#15189=CARTESIAN_POINT ( 'NONE',  ( -167.7210997126620384, -1.750000000000010214, -120.2068387089191219 ) ) ;
#15192=EDGE_CURVE ( 'NONE', #30683, #36281, #8531, .T. ) ;
#15197=AXIS2_PLACEMENT_3D ( 'NONE', #44693, #21616, #40866 ) ;
#15198=CARTESIAN_POINT ( 'NONE',  ( -167.7210997126620384, 1.750000000000009548, 81.84341382277507648 ) ) ;
#15199=ORIENTED_EDGE ( 'NONE', *, *, #5224, .T. ) ;
#15201=CYLINDRICAL_SURFACE ( 'NONE', #8949, 1.750000000000008438 ) ;
#15210=CARTESIAN_POINT ( 'NONE',  ( 153.3040265531850537, 0.000000000000000000, 165.0000000000000000 ) ) ;
#15211=CARTESIAN_POINT ( 'NONE',  ( 35.05402655318504657, 2.143131898507880377E-16, -40.93171244307205825 ) ) ;
#15212=ORIENTED_EDGE ( 'NONE', *, *, #14715, .F. ) ;
#15216=UNCERTAINTY_MEASURE_WITH_UNIT (LENGTH_MEASURE( 1.000000000000000082E-05 ), #32165, 'distance_accuracy_value', 'NONE');
#15220=ADVANCED_FACE ( 'NONE', ( #16224 ), #16480, .T. ) ;
#15227=DIRECTION ( 'NONE',  ( -0.000000000000000000, -0.000000000000000000, -1.000000000000000000 ) ) ;
#15243=ORIENTED_EDGE ( 'NONE', *, *, #31140, .F. ) ;
#15246=( BOUNDED_CURVE ( )  B_SPLINE_CURVE ( 3, ( #30924, #46508, #27313, #23467 ),
 .UNSPECIFIED., .F., .F. ) 
 B_SPLINE_CURVE_WITH_KNOTS ( ( 4, 4 ),
 ( 0.000000000000000000, 1.570796326794896558 ),
 .UNSPECIFIED. ) 
 CURVE ( )  GEOMETRIC_REPRESENTATION_ITEM ( )  RATIONAL_B_SPLINE_CURVE ( ( 1.000000000000000000, 0.8047378541243649375, 0.8047378541243649375, 1.000000000000000000 ) ) 
 REPRESENTATION_ITEM ( '' )  );
#15247=CARTESIAN_POINT ( 'NONE',  ( -164.9459734468149463, 2.143131898507880377E-16, -40.93171244307202983 ) ) ;
#15249=CARTESIAN_POINT ( 'NONE',  ( 35.05402655318504657, 1.025126265847089879, 122.5682875569280128 ) ) ;
#15251=VECTOR ( 'NONE', #43787, 1000.000000000000000 ) ;
#15252=CYLINDRICAL_SURFACE ( 'NONE', #38956, 1.750000000000015543 ) ;
#15253=ORIENTED_EDGE ( 'NONE', *, *, #25881, .T. ) ;
#15263=LINE ( 'NONE', #9006, #49398 ) ;
#15265=DIRECTION ( 'NONE',  ( 1.000000000000000000, 0.000000000000000000, 0.000000000000000000 ) ) ;
#15275=ORIENTED_EDGE ( 'NONE', *, *, #30006, .T. ) ;
#15276=AXIS2_PLACEMENT_3D ( 'NONE', #40107, #35322, #155 ) ;
#15277=CARTESIAN_POINT ( 'NONE',  ( -164.9459734468149463, -1.025126265847089213, 42.56828755692799149 ) ) ;
#15281=ORIENTED_EDGE ( 'NONE', *, *, #2030, .T. ) ;
#15287=EDGE_CURVE ( 'NONE', #26090, #35055, #7893, .T. ) ;
#15290=ORIENTED_EDGE ( 'NONE', *, *, #19615, .F. ) ;
#15296=ORIENTED_EDGE ( 'NONE', *, *, #39850, .F. ) ;
#15313=CARTESIAN_POINT ( 'NONE',  ( -6.695973446814940111, -1.750000000000024203, 120.8182875569279702 ) ) ;
#15315=ORIENTED_EDGE ( 'NONE', *, *, #172, .F. ) ;
#15318=CARTESIAN_POINT ( 'NONE',  ( 115.0540265531850395, 1.025126265847081886, 39.06828755692799149 ) ) ;
#15321=CARTESIAN_POINT ( 'NONE',  ( 151.5540265531850537, 0.000000000000000000, -40.93171244307202983 ) ) ;
#15332=CARTESIAN_POINT ( 'NONE',  ( 152.2789002873379900, 1.750000000000009548, 39.79316129108089228 ) ) ;
#15333=EDGE_CURVE ( 'NONE', #43762, #33571, #2915, .T. ) ;
#15336=CARTESIAN_POINT ( 'NONE',  ( 155.0540265531850537, 2.143131898507880377E-16, -37.43171244307205825 ) ) ;
#15340=DIRECTION ( 'NONE',  ( -1.000000000000000000, -0.000000000000000000, -0.000000000000000000 ) ) ;
#15344=VERTEX_POINT ( 'NONE', #18663 ) ;
#15346=CARTESIAN_POINT ( 'NONE',  ( -87.72109971266203843, -1.750000000000009548, -40.20683870891912193 ) ) ;
#15354=CARTESIAN_POINT ( 'NONE',  ( -126.6959734468149321, -1.749999999999996891, -159.1817124430720298 ) ) ;
#15355=ADVANCED_FACE ( 'NONE', ( #38205 ), #45088, .T. ) ;
#15358=CARTESIAN_POINT ( 'NONE',  ( 115.0540265531850395, 1.025126265847081664, 159.0682875569279418 ) ) ;
#15362=ORIENTED_EDGE ( 'NONE', *, *, #12222, .F. ) ;
#15364=EDGE_LOOP ( 'NONE', ( #33220, #46533, #44468, #45318, #42478 ) ) ;
#15368=ORIENTED_EDGE ( 'NONE', *, *, #24684, .F. ) ;
#15373=VECTOR ( 'NONE', #41169, 1000.000000000000000 ) ;
#15375=CARTESIAN_POINT ( 'NONE',  ( -208.4459734468148611, 1.025126265847089435, 39.06828755692797728 ) ) ;
#15377=CARTESIAN_POINT ( 'NONE',  ( 33.30402655318503946, -1.750000000000009992, -159.1817124430720298 ) ) ;
#15388=( BOUNDED_CURVE ( )  B_SPLINE_CURVE ( 3, ( #5579, #36411, #28445, #20992 ),
 .UNSPECIFIED., .F., .F. ) 
 B_SPLINE_CURVE_WITH_KNOTS ( ( 4, 4 ),
 ( 3.141592653589793116, 4.712388980384689674 ),
 .UNSPECIFIED. ) 
 CURVE ( )  GEOMETRIC_REPRESENTATION_ITEM ( )  RATIONAL_B_SPLINE_CURVE ( ( 1.000000000000000000, 0.8047378541243649375, 0.8047378541243649375, 1.000000000000000000 ) ) 
 REPRESENTATION_ITEM ( '' )  );
#15390=CARTESIAN_POINT ( 'NONE',  ( 195.0540265531851105, -1.025126265847089657, -120.9317124430720440 ) ) ;
#15393=ORIENTED_EDGE ( 'NONE', *, *, #15466, .T. ) ;
#15398=( BOUNDED_CURVE ( )  B_SPLINE_CURVE ( 3, ( #21456, #37642, #49124, #6574 ),
 .UNSPECIFIED., .F., .F. ) 
 B_SPLINE_CURVE_WITH_KNOTS ( ( 4, 4 ),
 ( 1.570796326794896558, 3.141592653589793116 ),
 .UNSPECIFIED. ) 
 CURVE ( )  GEOMETRIC_REPRESENTATION_ITEM ( )  RATIONAL_B_SPLINE_CURVE ( ( 1.000000000000000000, 0.8047378541243649375, 0.8047378541243649375, 1.000000000000000000 ) ) 
 REPRESENTATION_ITEM ( '' )  );
#15401=ORIENTED_EDGE ( 'NONE', *, *, #15626, .T. ) ;
#15403=ORIENTED_EDGE ( 'NONE', *, *, #12863, .F. ) ;
#15405=CARTESIAN_POINT ( 'NONE',  ( -6.695973446814940111, 1.750000000000023759, 40.81828755692798438 ) ) ;
#15409=CARTESIAN_POINT ( 'NONE',  ( 210.0000000000000568, 0.000000000000000000, -159.1817124430720298 ) ) ;
#15411=CARTESIAN_POINT ( 'NONE',  ( 210.0000000000000568, 2.143131898507881856E-16, -120.9317124430720582 ) ) ;
#15424=CARTESIAN_POINT ( 'NONE',  ( 154.3291528190321458, -1.750000000000009548, -118.1565861772249519 ) ) ;
#15425=FACE_OUTER_BOUND ( 'NONE', #35001, .T. ) ;
#15431=ORIENTED_EDGE ( 'NONE', *, *, #50537, .T. ) ;
#15433=CARTESIAN_POINT ( 'NONE',  ( -126.6959734468149321, -1.749999999999997335, 80.81828755692798438 ) ) ;
#15436=DIRECTION ( 'NONE',  ( -1.000000000000000000, -0.000000000000000000, -0.000000000000000000 ) ) ;
#15439=ORIENTED_EDGE ( 'NONE', *, *, #29601, .T. ) ;
#15441=CARTESIAN_POINT ( 'NONE',  ( 153.3040265531850537, 0.000000000000000000, 165.0000000000000000 ) ) ;
#15443=CARTESIAN_POINT ( 'NONE',  ( -204.9459734468148895, 1.025126265847089879, -117.4317124430720156 ) ) ;
#15444=ORIENTED_EDGE ( 'NONE', *, *, #24699, .F. ) ;
#15445=CARTESIAN_POINT ( 'NONE',  ( 115.0540265531850395, 1.025126265847081442, -160.9317124430720014 ) ) ;
#15454=ORIENTED_EDGE ( 'NONE', *, *, #9944, .T. ) ;
#15460=ORIENTED_EDGE ( 'NONE', *, *, #39739, .F. ) ;
#15462=CARTESIAN_POINT ( 'NONE',  ( 111.5540265531850679, 0.000000000000000000, -77.43171244307204404 ) ) ;
#15466=EDGE_CURVE ( 'NONE', #21643, #8176, #18647, .T. ) ;
#15468=CYLINDRICAL_SURFACE ( 'NONE', #381, 1.750000000000015543 ) ;
#15470=CARTESIAN_POINT ( 'NONE',  ( 191.5540265531851105, 0.000000000000000000, 2.568287556927978166 ) ) ;
#15471=ORIENTED_EDGE ( 'NONE', *, *, #18325, .F. ) ;
#15478=DIRECTION ( 'NONE',  ( -0.000000000000000000, -0.000000000000000000, -1.000000000000000000 ) ) ;
#15479=ADVANCED_FACE ( 'NONE', ( #47096 ), #15082, .T. ) ;
#15484=ORIENTED_EDGE ( 'NONE', *, *, #21100, .F. ) ;
#15485=CARTESIAN_POINT ( 'NONE',  ( 115.0540265531850679, 0.000000000000000000, 162.5682875569279702 ) ) ;
#15494=CARTESIAN_POINT ( 'NONE',  ( -84.94597344681494633, 2.143131898507880377E-16, 159.0682875569279702 ) ) ;
#15496=LINE ( 'NONE', #38615, #11039 ) ;
#15499=CARTESIAN_POINT ( 'NONE',  ( -128.4459734468149179, 0.000000000000000000, 165.0000000000000000 ) ) ;
#15500=CARTESIAN_POINT ( 'NONE',  ( 73.30402655318508209, -1.750000000000010658, -119.1817124430720440 ) ) ;
#15506=EDGE_CURVE ( 'NONE', #25636, #36281, #11244, .T. ) ;
#15514=EDGE_CURVE ( 'NONE', #13717, #21643, #2617, .T. ) ;
#15515=FACE_OUTER_BOUND ( 'NONE', #20747, .T. ) ;
#15521=ORIENTED_EDGE ( 'NONE', *, *, #4280, .F. ) ;
#15523=EDGE_LOOP ( 'NONE', ( #46864, #40825, #39064, #2113, #34554, #37085 ) ) ;
#15524=ADVANCED_FACE ( 'NONE', ( #39209 ), #11490, .T. ) ;
#15525=CYLINDRICAL_SURFACE ( 'NONE', #21798, 1.750000000000001554 ) ;
#15529=EDGE_CURVE ( 'NONE', #32098, #36777, #42934, .T. ) ;
#15531=ADVANCED_FACE ( 'NONE', ( #22776 ), #15593, .T. ) ;
#15532=ORIENTED_EDGE ( 'NONE', *, *, #34334, .T. ) ;
#15533=LINE ( 'NONE', #35558, #27235 ) ;
#15534=CARTESIAN_POINT ( 'NONE',  ( 112.2789002873379758, -1.749999999999996669, 39.79316129108089228 ) ) ;
#15536=ORIENTED_EDGE ( 'NONE', *, *, #35291, .T. ) ;
#15538=( BOUNDED_CURVE ( )  B_SPLINE_CURVE ( 3, ( #37903, #6832, #18362, #18615 ),
 .UNSPECIFIED., .F., .F. ) 
 B_SPLINE_CURVE_WITH_KNOTS ( ( 4, 4 ),
 ( 1.570796326794896558, 3.141592653589793116 ),
 .UNSPECIFIED. ) 
 CURVE ( )  GEOMETRIC_REPRESENTATION_ITEM ( )  RATIONAL_B_SPLINE_CURVE ( ( 1.000000000000000000, 0.8047378541243649375, 0.8047378541243649375, 1.000000000000000000 ) ) 
 REPRESENTATION_ITEM ( '' )  );
#15540=EDGE_CURVE ( 'NONE', #19505, #17731, #26882, .T. ) ;
#15547=DIRECTION ( 'NONE',  ( -0.000000000000000000, -0.000000000000000000, -1.000000000000000000 ) ) ;
#15551=CARTESIAN_POINT ( 'NONE',  ( -8.445973446814976526, 0.000000000000000000, -0.9317124430720524764 ) ) ;
#15554=VERTEX_POINT ( 'NONE', #16099 ) ;
#15555=ORIENTED_EDGE ( 'NONE', *, *, #20462, .F. ) ;
#15560=CARTESIAN_POINT ( 'NONE',  ( -126.6959734468149321, 0.000000000000000000, 165.0000000000000000 ) ) ;
#15561=DIRECTION ( 'NONE',  ( 0.000000000000000000, 0.000000000000000000, 1.000000000000000000 ) ) ;
#15562=LINE ( 'NONE', #31984, #34333 ) ;
#15563=EDGE_CURVE ( 'NONE', #37586, #46541, #30819, .T. ) ;
#15565=ORIENTED_EDGE ( 'NONE', *, *, #21501, .F. ) ;
#15568=CARTESIAN_POINT ( 'NONE',  ( -86.69597344681496054, 0.000000000000000000, 165.0000000000000000 ) ) ;
#15570=ADVANCED_FACE ( 'NONE', ( #24317 ), #962, .T. ) ;
#15573=ADVANCED_FACE ( 'NONE', ( #24554 ), #21200, .T. ) ;
#15583=CARTESIAN_POINT ( 'NONE',  ( 153.3040265531850537, -1.750000000000010214, -39.18171244307202983 ) ) ;
#15584=CARTESIAN_POINT ( 'NONE',  ( 71.55402655318505367, 1.025126265847089435, 39.06828755692797728 ) ) ;
#15586=AXIS2_PLACEMENT_3D ( 'NONE', #12769, #40483, #24575 ) ;
#15587=CARTESIAN_POINT ( 'NONE',  ( 210.0000000000000568, 0.000000000000000000, -37.43171244307202272 ) ) ;
#15588=EDGE_CURVE ( 'NONE', #45408, #34855, #13115, .T. ) ;
#15593=CYLINDRICAL_SURFACE ( 'NONE', #13156, 1.749999999999987566 ) ;
#15598=CYLINDRICAL_SURFACE ( 'NONE', #16734, 1.749999999999973799 ) ;
#15601=CARTESIAN_POINT ( 'NONE',  ( -205.6708471809678827, 1.750000000000010214, 119.7931612910808781 ) ) ;
#15605=DIRECTION ( 'NONE',  ( -1.000000000000000000, -0.000000000000000000, -0.000000000000000000 ) ) ;
#15606=CARTESIAN_POINT ( 'NONE',  ( -85.67084718096784002, 1.750000000000009548, 1.843413822775065825 ) ) ;
#15610=DIRECTION ( 'NONE',  ( 0.000000000000000000, 0.000000000000000000, 1.000000000000000000 ) ) ;
#15622=CARTESIAN_POINT ( 'NONE',  ( -166.6959734468149463, -1.750000000000010658, 120.8182875569279702 ) ) ;
#15624=ORIENTED_EDGE ( 'NONE', *, *, #19903, .T. ) ;
#15626=EDGE_CURVE ( 'NONE', #23844, #5437, #683, .T. ) ;
#15627=EDGE_CURVE ( 'NONE', #42197, #27344, #44032, .T. ) ;
#15632=EDGE_CURVE ( 'NONE', #14566, #34169, #40713, .T. ) ;
#15636=EDGE_CURVE ( 'NONE', #7012, #38661, #49182, .T. ) ;
#15637=EDGE_CURVE ( 'NONE', #13383, #16751, #21657, .T. ) ;
#15638=VERTEX_POINT ( 'NONE', #8409 ) ;
#15644=CARTESIAN_POINT ( 'NONE',  ( -124.9459734468149321, 1.025126265847082108, -77.43171244307201562 ) ) ;
#15646=VERTEX_POINT ( 'NONE', #29166 ) ;
#15671=CARTESIAN_POINT ( 'NONE',  ( 151.5540265531850537, 0.000000000000000000, 162.5682875569279702 ) ) ;
#15672=( BOUNDED_CURVE ( )  B_SPLINE_CURVE ( 3, ( #27012, #43661, #4178, #15719 ),
 .UNSPECIFIED., .F., .F. ) 
 B_SPLINE_CURVE_WITH_KNOTS ( ( 4, 4 ),
 ( 1.570796326794896558, 3.141592653589793116 ),
 .UNSPECIFIED. ) 
 CURVE ( )  GEOMETRIC_REPRESENTATION_ITEM ( )  RATIONAL_B_SPLINE_CURVE ( ( 1.000000000000000000, 0.8047378541243649375, 0.8047378541243649375, 1.000000000000000000 ) ) 
 REPRESENTATION_ITEM ( '' )  );
#15674=ORIENTED_EDGE ( 'NONE', *, *, #43183, .T. ) ;
#15677=( BOUNDED_CURVE ( )  B_SPLINE_CURVE ( 3, ( #6608, #22261, #19155, #26618 ),
 .UNSPECIFIED., .F., .F. ) 
 B_SPLINE_CURVE_WITH_KNOTS ( ( 4, 4 ),
 ( 3.141592653589793116, 4.712388980384689674 ),
 .UNSPECIFIED. ) 
 CURVE ( )  GEOMETRIC_REPRESENTATION_ITEM ( )  RATIONAL_B_SPLINE_CURVE ( ( 1.000000000000000000, 0.8047378541243649375, 0.8047378541243649375, 1.000000000000000000 ) ) 
 REPRESENTATION_ITEM ( '' )  );
#15680=AXIS2_PLACEMENT_3D ( 'NONE', #23309, #38725, #46382 ) ;
#15683=CARTESIAN_POINT ( 'NONE',  ( 210.0000000000000568, 0.000000000000000000, -159.1817124430720298 ) ) ;
#15689=CARTESIAN_POINT ( 'NONE',  ( 155.0540265531850537, 1.025126265847089435, 39.06828755692797728 ) ) ;
#15690=( BOUNDED_CURVE ( )  B_SPLINE_CURVE ( 3, ( #24267, #39920, #4999, #16056 ),
 .UNSPECIFIED., .F., .F. ) 
 B_SPLINE_CURVE_WITH_KNOTS ( ( 4, 4 ),
 ( 1.570796326794896558, 3.141592653589793116 ),
 .UNSPECIFIED. ) 
 CURVE ( )  GEOMETRIC_REPRESENTATION_ITEM ( )  RATIONAL_B_SPLINE_CURVE ( ( 1.000000000000000000, 0.8047378541243649375, 0.8047378541243649375, 1.000000000000000000 ) ) 
 REPRESENTATION_ITEM ( '' )  );
#15700=ORIENTED_EDGE ( 'NONE', *, *, #17778, .T. ) ;
#15701=EDGE_CURVE ( 'NONE', #7036, #30495, #14764, .T. ) ;
#15707=ORIENTED_EDGE ( 'NONE', *, *, #22940, .F. ) ;
#15709=DIRECTION ( 'NONE',  ( -1.000000000000000000, -0.000000000000000000, -0.000000000000000000 ) ) ;
#15712=CARTESIAN_POINT ( 'NONE',  ( -6.695973446814940111, 1.750000000000023315, -159.1817124430720298 ) ) ;
#15713=CARTESIAN_POINT ( 'NONE',  ( 155.0540265531850537, 2.143131898507880377E-16, -77.43171244307204404 ) ) ;
#15715=AXIS2_PLACEMENT_3D ( 'NONE', #12574, #41, #28244 ) ;
#15719=CARTESIAN_POINT ( 'NONE',  ( 111.5540265531850679, 0.000000000000000000, -117.4317124430720725 ) ) ;
#15723=CARTESIAN_POINT ( 'NONE',  ( -166.6959734468149463, -1.750000000000010214, 40.81828755692798438 ) ) ;
#15725=ORIENTED_EDGE ( 'NONE', *, *, #49974, .F. ) ;
#15727=ORIENTED_EDGE ( 'NONE', *, *, #21188, .T. ) ;
#15729=EDGE_CURVE ( 'NONE', #31600, #23031, #23914, .T. ) ;
#15730=CARTESIAN_POINT ( 'NONE',  ( 191.5540265531851105, 0.000000000000000000, 165.0000000000000000 ) ) ;
#15732=VERTEX_POINT ( 'NONE', #48860 ) ;
#15738=CARTESIAN_POINT ( 'NONE',  ( -166.6959734468149463, 1.750000000000010214, -39.18171244307202983 ) ) ;
#15743=ORIENTED_EDGE ( 'NONE', *, *, #9661, .T. ) ;
#15747=CARTESIAN_POINT ( 'NONE',  ( 35.05402655318503946, 0.000000000000000000, 162.5682875569279702 ) ) ;
#15751=ORIENTED_EDGE ( 'NONE', *, *, #8932, .F. ) ;
#15752=CARTESIAN_POINT ( 'NONE',  ( -4.945973446814916130, -1.025126265847097429, 79.06828755692792754 ) ) ;
#15755=CYLINDRICAL_SURFACE ( 'NONE', #12653, 1.750000000000001554 ) ;
#15764=ORIENTED_EDGE ( 'NONE', *, *, #18881, .T. ) ;
#15771=ORIENTED_EDGE ( 'NONE', *, *, #50404, .T. ) ;
#15778=LINE ( 'NONE', #31447, #23974 ) ;
#15784=ORIENTED_EDGE ( 'NONE', *, *, #19583, .T. ) ;
#15786=ORIENTED_EDGE ( 'NONE', *, *, #39968, .T. ) ;
#15787=EDGE_CURVE ( 'NONE', #35621, #16704, #45027, .T. ) ;
#15789=AXIS2_PLACEMENT_3D ( 'NONE', #27949, #39004, #12800 ) ;
#15790=CARTESIAN_POINT ( 'NONE',  ( -5.670847180967843570, -1.750000000000023315, 41.84341382277508359 ) ) ;
#15791=DIRECTION ( 'NONE',  ( -1.000000000000000000, -0.000000000000000000, -0.000000000000000000 ) ) ;
#15792=EDGE_CURVE ( 'NONE', #47066, #4803, #48142, .T. ) ;
#15796=AXIS2_PLACEMENT_3D ( 'NONE', #5369, #28481, #32844 ) ;
#15798=CYLINDRICAL_SURFACE ( 'NONE', #35318, 1.750000000000036193 ) ;
#15800=ORIENTED_EDGE ( 'NONE', *, *, #42123, .F. ) ;
#15802=CARTESIAN_POINT ( 'NONE',  ( -44.94597344681493922, 1.025126265847089435, -40.93171244307204404 ) ) ;
#15804=CARTESIAN_POINT ( 'NONE',  ( 151.5540265531850537, 0.000000000000000000, 165.0000000000000000 ) ) ;
#15810=CARTESIAN_POINT ( 'NONE',  ( 155.0540265531850537, 2.143131898507880377E-16, 165.0000000000000000 ) ) ;
#15818=EDGE_CURVE ( 'NONE', #36401, #26375, #26064, .T. ) ;
#15823=ORIENTED_EDGE ( 'NONE', *, *, #22781, .F. ) ;
#15832=AXIS2_PLACEMENT_3D ( 'NONE', #34379, #33878, #49965 ) ;
#15838=( BOUNDED_CURVE ( )  B_SPLINE_CURVE ( 3, ( #42141, #49794, #7004, #22649 ),
 .UNSPECIFIED., .F., .F. ) 
 B_SPLINE_CURVE_WITH_KNOTS ( ( 4, 4 ),
 ( 1.570796326794896558, 3.141592653589793116 ),
 .UNSPECIFIED. ) 
 CURVE ( )  GEOMETRIC_REPRESENTATION_ITEM ( )  RATIONAL_B_SPLINE_CURVE ( ( 1.000000000000000000, 0.8047378541243649375, 0.8047378541243649375, 1.000000000000000000 ) ) 
 REPRESENTATION_ITEM ( '' )  );
#15839=ORIENTED_EDGE ( 'NONE', *, *, #42843, .T. ) ;
#15842=ORIENTED_EDGE ( 'NONE', *, *, #1865, .F. ) ;
#15846=ORIENTED_EDGE ( 'NONE', *, *, #26779, .T. ) ;
#15851=ORIENTED_EDGE ( 'NONE', *, *, #42158, .T. ) ;
#15864=EDGE_CURVE ( 'NONE', #49857, #44495, #2326, .T. ) ;
#15866=ADVANCED_FACE ( 'NONE', ( #144 ), #31444, .T. ) ;
#15868=VERTEX_POINT ( 'NONE', #22713 ) ;
#15875=DIRECTION ( 'NONE',  ( 0.000000000000000000, 0.000000000000000000, 1.000000000000000000 ) ) ;
#15878=CARTESIAN_POINT ( 'NONE',  ( 155.0540265531850537, 2.143131898507880377E-16, -117.4317124430720725 ) ) ;
#15880=CARTESIAN_POINT ( 'NONE',  ( -86.69597344681496054, 0.000000000000000000, 165.0000000000000000 ) ) ;
#15885=EDGE_CURVE ( 'NONE', #43863, #37343, #18346, .T. ) ;
#15901=ORIENTED_EDGE ( 'NONE', *, *, #50683, .T. ) ;
#15910=ORIENTED_EDGE ( 'NONE', *, *, #28156, .T. ) ;
#15920=ADVANCED_FACE ( 'NONE', ( #4985 ), #13190, .T. ) ;
#15925=CARTESIAN_POINT ( 'NONE',  ( 153.3040265531850537, -1.750000000000010214, 40.81828755692798438 ) ) ;
#15929=EDGE_CURVE ( 'NONE', #35915, #8390, #7580, .T. ) ;
#15931=ORIENTED_EDGE ( 'NONE', *, *, #25258, .T. ) ;
#15933=EDGE_CURVE ( 'NONE', #13539, #44183, #47840, .T. ) ;
#15935=CARTESIAN_POINT ( 'NONE',  ( -4.945973446814903696, 2.143131898507912917E-16, -117.4317124430720156 ) ) ;
#15937=CARTESIAN_POINT ( 'NONE',  ( -5.670847180967843570, 1.750000000000023315, 39.79316129108089228 ) ) ;
#15940=CARTESIAN_POINT ( 'NONE',  ( -84.94597344681494633, 2.143131898507880377E-16, -160.9317124430720014 ) ) ;
#15942=VECTOR ( 'NONE', #35425, 1000.000000000000000 ) ;
#15945=ORIENTED_EDGE ( 'NONE', *, *, #26236, .F. ) ;
#15949=DIRECTION ( 'NONE',  ( 0.000000000000000000, 0.000000000000000000, -1.000000000000000000 ) ) ;
#15951=CARTESIAN_POINT ( 'NONE',  ( -204.9459734468148895, 1.025126265847089435, -40.93171244307204404 ) ) ;
#15953=ORIENTED_EDGE ( 'NONE', *, *, #6106, .F. ) ;
#15958=VECTOR ( 'NONE', #39304, 1000.000000000000000 ) ;
#15960=VERTEX_POINT ( 'NONE', #10098 ) ;
#15976=CYLINDRICAL_SURFACE ( 'NONE', #31981, 1.750000000000008438 ) ;
#15977=ORIENTED_EDGE ( 'NONE', *, *, #40688, .F. ) ;
#15978=ORIENTED_EDGE ( 'NONE', *, *, #5106, .T. ) ;
#15980=CIRCLE ( 'NONE', #18414, 1.750000000000008438 ) ;
#15981=( BOUNDED_CURVE ( )  B_SPLINE_CURVE ( 3, ( #3384, #30604, #19036, #46205 ),
 .UNSPECIFIED., .F., .F. ) 
 B_SPLINE_CURVE_WITH_KNOTS ( ( 4, 4 ),
 ( 1.570796326794896558, 3.141592653589793116 ),
 .UNSPECIFIED. ) 
 CURVE ( )  GEOMETRIC_REPRESENTATION_ITEM ( )  RATIONAL_B_SPLINE_CURVE ( ( 1.000000000000000000, 0.8047378541243649375, 0.8047378541243649375, 1.000000000000000000 ) ) 
 REPRESENTATION_ITEM ( '' )  );
#15985=CARTESIAN_POINT ( 'NONE',  ( 195.0540265531851105, 2.143131898507880377E-16, -0.9317124430720247208 ) ) ;
#15986=DIRECTION ( 'NONE',  ( -1.000000000000000000, -0.000000000000000000, -0.000000000000000000 ) ) ;
#15990=( BOUNDED_CURVE ( )  B_SPLINE_CURVE ( 3, ( #21320, #14114, #29277, #41328 ),
 .UNSPECIFIED., .F., .F. ) 
 B_SPLINE_CURVE_WITH_KNOTS ( ( 4, 4 ),
 ( 0.000000000000000000, 1.570796326794896558 ),
 .UNSPECIFIED. ) 
 CURVE ( )  GEOMETRIC_REPRESENTATION_ITEM ( )  RATIONAL_B_SPLINE_CURVE ( ( 1.000000000000000000, 0.8047378541243649375, 0.8047378541243649375, 1.000000000000000000 ) ) 
 REPRESENTATION_ITEM ( '' )  );
#15992=DIRECTION ( 'NONE',  ( -1.000000000000000000, -0.000000000000000000, -0.000000000000000000 ) ) ;
#15999=ORIENTED_EDGE ( 'NONE', *, *, #47287, .F. ) ;
#16001=CARTESIAN_POINT ( 'NONE',  ( 210.0000000000000568, 2.143131898507881116E-16, -40.93171244307203693 ) ) ;
#16002=EDGE_CURVE ( 'NONE', #14561, #31607, #11184, .T. ) ;
#16004=( BOUNDED_CURVE ( )  B_SPLINE_CURVE ( 3, ( #29177, #18114, #33787, #44792 ),
 .UNSPECIFIED., .F., .F. ) 
 B_SPLINE_CURVE_WITH_KNOTS ( ( 4, 4 ),
 ( 4.712388980384689674, 6.283185307179586232 ),
 .UNSPECIFIED. ) 
 CURVE ( )  GEOMETRIC_REPRESENTATION_ITEM ( )  RATIONAL_B_SPLINE_CURVE ( ( 1.000000000000000000, 0.8047378541243649375, 0.8047378541243649375, 1.000000000000000000 ) ) 
 REPRESENTATION_ITEM ( '' )  );
#16007=CARTESIAN_POINT ( 'NONE',  ( -128.4459734468149179, 0.000000000000000000, 165.0000000000000000 ) ) ;
#16013=AXIS2_PLACEMENT_3D ( 'NONE', #25472, #10071, #37306 ) ;
#16014=CARTESIAN_POINT ( 'NONE',  ( 33.30402655318503946, 1.750000000000009992, 160.8182875569279702 ) ) ;
#16019=VERTEX_POINT ( 'NONE', #18283 ) ;
#16021=CARTESIAN_POINT ( 'NONE',  ( 191.5540265531851105, 0.000000000000000000, 165.0000000000000000 ) ) ;
#16024=CYLINDRICAL_SURFACE ( 'NONE', #47962, 1.750000000000001554 ) ;
#16030=DIRECTION ( 'NONE',  ( -1.000000000000000000, -0.000000000000000000, -0.000000000000000000 ) ) ;
#16048=CARTESIAN_POINT ( 'NONE',  ( 151.5540265531850537, 0.000000000000000000, 79.06828755692797017 ) ) ;
#16054=CIRCLE ( 'NONE', #17692, 1.750000000000001554 ) ;
#16056=CARTESIAN_POINT ( 'NONE',  ( 71.55402655318505367, 0.000000000000000000, 42.56828755692799859 ) ) ;
#16057=VERTEX_POINT ( 'NONE', #33222 ) ;
#16061=CARTESIAN_POINT ( 'NONE',  ( -8.445973446814976526, 0.000000000000000000, 82.56828755692801280 ) ) ;
#16069=FACE_OUTER_BOUND ( 'NONE', #2535, .T. ) ;
#16083=EDGE_CURVE ( 'NONE', #46160, #11740, #33465, .T. ) ;
#16084=CARTESIAN_POINT ( 'NONE',  ( 195.0540265531851105, 2.143131898507880377E-16, -160.9317124430720014 ) ) ;
#16085=VECTOR ( 'NONE', #30816, 1000.000000000000000 ) ;
#16086=ORIENTED_EDGE ( 'NONE', *, *, #33873, .T. ) ;
#16088=CARTESIAN_POINT ( 'NONE',  ( 195.0540265531851105, 2.143131898507880377E-16, 162.5682875569279702 ) ) ;
#16089=VERTEX_POINT ( 'NONE', #21388 ) ;
#16095=ORIENTED_EDGE ( 'NONE', *, *, #5158, .T. ) ;
#16099=CARTESIAN_POINT ( 'NONE',  ( 195.0540265531851105, 2.143131898507880377E-16, -80.93171244307201562 ) ) ;
#16101=ORIENTED_EDGE ( 'NONE', *, *, #2771, .T. ) ;
#16108=CARTESIAN_POINT ( 'NONE',  ( 210.0000000000000568, 0.000000000000000000, -79.18171244307201562 ) ) ;
#16109=CARTESIAN_POINT ( 'NONE',  ( 115.0540265531850395, 2.143131898507847836E-16, 122.5682875569279560 ) ) ;
#16110=LINE ( 'NONE', #31775, #44690 ) ;
#16115=FACE_OUTER_BOUND ( 'NONE', #27253, .T. ) ;
#16117=ORIENTED_EDGE ( 'NONE', *, *, #5224, .F. ) ;
#16130=FACE_OUTER_BOUND ( 'NONE', #27477, .T. ) ;
#16131=CARTESIAN_POINT ( 'NONE',  ( -168.4459734468149747, -1.025126265847089435, -157.4317124430720582 ) ) ;
#16132=DIRECTION ( 'NONE',  ( -0.000000000000000000, -0.000000000000000000, -1.000000000000000000 ) ) ;
#16133=CARTESIAN_POINT ( 'NONE',  ( -204.9459734468148895, 1.025126265847089657, -80.93171244307201562 ) ) ;
#16135=DIRECTION ( 'NONE',  ( -1.000000000000000000, 0.000000000000000000, 0.000000000000000000 ) ) ;
#16136=LINE ( 'NONE', #45686, #4771 ) ;
#16144=( BOUNDED_CURVE ( )  B_SPLINE_CURVE ( 3, ( #37514, #21075, #44898, #36760 ),
 .UNSPECIFIED., .F., .F. ) 
 B_SPLINE_CURVE_WITH_KNOTS ( ( 4, 4 ),
 ( 0.000000000000000000, 1.570796326794896558 ),
 .UNSPECIFIED. ) 
 CURVE ( )  GEOMETRIC_REPRESENTATION_ITEM ( )  RATIONAL_B_SPLINE_CURVE ( ( 1.000000000000000000, 0.8047378541243649375, 0.8047378541243649375, 1.000000000000000000 ) ) 
 REPRESENTATION_ITEM ( '' )  );
#16158=CARTESIAN_POINT ( 'NONE',  ( -164.9459734468149463, 2.143131898507880377E-16, -77.43171244307204404 ) ) ;
#16163=CARTESIAN_POINT ( 'NONE',  ( 31.55402655318503236, 0.000000000000000000, 165.0000000000000000 ) ) ;
#16166=VERTEX_POINT ( 'NONE', #19052 ) ;
#16170=VERTEX_POINT ( 'NONE', #22654 ) ;
#16172=DIRECTION ( 'NONE',  ( -1.000000000000000000, 0.000000000000000000, 0.000000000000000000 ) ) ;
#16180=EDGE_CURVE ( 'NONE', #9118, #20525, #49779, .T. ) ;
#16187=CARTESIAN_POINT ( 'NONE',  ( 151.5540265531850537, 0.000000000000000000, 165.0000000000000000 ) ) ;
#16190=CARTESIAN_POINT ( 'NONE',  ( 71.55402655318505367, -1.025126265847089657, -120.9317124430720440 ) ) ;
#16196=ORIENTED_EDGE ( 'NONE', *, *, #39084, .T. ) ;
#16197=VERTEX_POINT ( 'NONE', #27278 ) ;
#16203=ORIENTED_EDGE ( 'NONE', *, *, #9155, .T. ) ;
#16204=LINE ( 'NONE', #43635, #14060 ) ;
#16209=ORIENTED_EDGE ( 'NONE', *, *, #39464, .T. ) ;
#16210=PLANE ( 'NONE',  #34628 ) ;
#16213=ORIENTED_EDGE ( 'NONE', *, *, #34334, .F. ) ;
#16216=CARTESIAN_POINT ( 'NONE',  ( -4.945973446814903696, 2.143131898507912917E-16, 42.56828755692802702 ) ) ;
#16224=FACE_OUTER_BOUND ( 'NONE', #28362, .T. ) ;
#16227=CARTESIAN_POINT ( 'NONE',  ( 113.3040265531850537, 1.749999999999996891, 0.8182875569279768335 ) ) ;
#16228=( BOUNDED_CURVE ( )  B_SPLINE_CURVE ( 3, ( #45541, #6573, #22223, #10421 ),
 .UNSPECIFIED., .F., .F. ) 
 B_SPLINE_CURVE_WITH_KNOTS ( ( 4, 4 ),
 ( 1.570796326794896558, 3.141592653589793116 ),
 .UNSPECIFIED. ) 
 CURVE ( )  GEOMETRIC_REPRESENTATION_ITEM ( )  RATIONAL_B_SPLINE_CURVE ( ( 1.000000000000000000, 0.8047378541243649375, 0.8047378541243649375, 1.000000000000000000 ) ) 
 REPRESENTATION_ITEM ( '' )  );
#16233=ORIENTED_EDGE ( 'NONE', *, *, #50584, .F. ) ;
#16243=LINE ( 'NONE', #15730, #37407 ) ;
#16246=AXIS2_PLACEMENT_3D ( 'NONE', #29320, #13404, #13160 ) ;
#16248=EDGE_LOOP ( 'NONE', ( #31136, #22010, #26108, #11855, #1393, #1167 ) ) ;
#16249=CARTESIAN_POINT ( 'NONE',  ( -208.4459734468148611, 1.025126265847089657, 119.0682875569279560 ) ) ;
#16252=EDGE_LOOP ( 'NONE', ( #40136, #31145, #35512, #3071, #2679 ) ) ;
#16255=ADVANCED_FACE ( 'NONE', ( #3678 ), #11642, .T. ) ;
#16257=EDGE_LOOP ( 'NONE', ( #29104, #1077, #37645, #9555, #14052, #48487 ) ) ;
#16258=CARTESIAN_POINT ( 'NONE',  ( -47.72109971266203132, -1.750000000000010214, 81.84341382277507648 ) ) ;
#16261=CARTESIAN_POINT ( 'NONE',  ( -48.44597344681496054, 1.025126265847089435, 82.56828755692798438 ) ) ;
#16264=VERTEX_POINT ( 'NONE', #15485 ) ;
#16268=DIRECTION ( 'NONE',  ( -1.000000000000000000, 0.000000000000000000, 0.000000000000000000 ) ) ;
#16269=CARTESIAN_POINT ( 'NONE',  ( 33.30402655318503946, -1.750000000000010214, -39.18171244307202983 ) ) ;
#16270=EDGE_CURVE ( 'NONE', #5639, #40502, #8057, .T. ) ;
#16272=EDGE_CURVE ( 'NONE', #28356, #28555, #9521, .T. ) ;
#16273=DIRECTION ( 'NONE',  ( 0.000000000000000000, 0.000000000000000000, 1.000000000000000000 ) ) ;
#16277=CARTESIAN_POINT ( 'NONE',  ( 193.3040265531851105, -1.750000000000009992, -159.1817124430720298 ) ) ;
#16278=EDGE_CURVE ( 'NONE', #42411, #7277, #8192, .T. ) ;
#16281=( BOUNDED_CURVE ( )  B_SPLINE_CURVE ( 3, ( #43222, #23731, #19617, #35298 ),
 .UNSPECIFIED., .F., .F. ) 
 B_SPLINE_CURVE_WITH_KNOTS ( ( 4, 4 ),
 ( 3.141592653589793116, 4.712388980384689674 ),
 .UNSPECIFIED. ) 
 CURVE ( )  GEOMETRIC_REPRESENTATION_ITEM ( )  RATIONAL_B_SPLINE_CURVE ( ( 1.000000000000000000, 0.8047378541243649375, 0.8047378541243649375, 1.000000000000000000 ) ) 
 REPRESENTATION_ITEM ( '' )  );
#16291=DIRECTION ( 'NONE',  ( -1.000000000000000000, 0.000000000000000000, 0.000000000000000000 ) ) ;
#16292=CARTESIAN_POINT ( 'NONE',  ( 155.0540265531850537, 2.143131898507880377E-16, 79.06828755692797017 ) ) ;
#16293=VERTEX_POINT ( 'NONE', #35259 ) ;
#16295=LINE ( 'NONE', #38211, #19573 ) ;
#16298=CARTESIAN_POINT ( 'NONE',  ( 152.2789002873379900, 1.750000000000010436, 79.79316129108087807 ) ) ;
#16300=ORIENTED_EDGE ( 'NONE', *, *, #31288, .F. ) ;
#16311=CYLINDRICAL_SURFACE ( 'NONE', #16680, 1.750000000000008438 ) ;
#16312=ORIENTED_EDGE ( 'NONE', *, *, #6890, .T. ) ;
#16313=VERTEX_POINT ( 'NONE', #9558 ) ;
#16314=EDGE_CURVE ( 'NONE', #12712, #13146, #4940, .T. ) ;
#16318=ORIENTED_EDGE ( 'NONE', *, *, #24293, .T. ) ;
#16327=CARTESIAN_POINT ( 'NONE',  ( -46.69597344681494633, 1.750000000000010658, -79.18171244307201562 ) ) ;
#16329=AXIS2_PLACEMENT_3D ( 'NONE', #27737, #24900, #20783 ) ;
#16332=CARTESIAN_POINT ( 'NONE',  ( -7.721099712662037540, -1.750000000000023537, -118.1565861772249519 ) ) ;
#16334=EDGE_LOOP ( 'NONE', ( #5092, #47746, #12199, #25013, #12817, #8279 ) ) ;
#16337=CARTESIAN_POINT ( 'NONE',  ( -8.445973446814964092, -1.025126265847097429, -120.9317124430720440 ) ) ;
#16338=EDGE_CURVE ( 'NONE', #25029, #3215, #12893, .T. ) ;
#16342=CARTESIAN_POINT ( 'NONE',  ( -206.6959734468149463, 1.750000000000009992, 0.8182875569279768335 ) ) ;
#16343=ORIENTED_EDGE ( 'NONE', *, *, #43469, .T. ) ;
#16345=CARTESIAN_POINT ( 'NONE',  ( 210.0000000000000568, 2.143131898507881116E-16, 39.06828755692797728 ) ) ;
#16346=DIRECTION ( 'NONE',  ( 0.000000000000000000, 0.000000000000000000, 1.000000000000000000 ) ) ;
#16349=CARTESIAN_POINT ( 'NONE',  ( -164.9459734468149463, 1.025126265847089213, -160.9317124430720014 ) ) ;
#16350=CARTESIAN_POINT ( 'NONE',  ( -126.6959734468149321, 1.749999999999996891, 160.8182875569279702 ) ) ;
#16353=AXIS2_PLACEMENT_3D ( 'NONE', #35670, #4822, #47644 ) ;
#16355=DIRECTION ( 'NONE',  ( -1.000000000000000000, -0.000000000000000000, -0.000000000000000000 ) ) ;
#16364=ORIENTED_EDGE ( 'NONE', *, *, #25203, .F. ) ;
#16366=CARTESIAN_POINT ( 'NONE',  ( -210.0000000000000568, 0.000000000000000000, -157.4317124430720298 ) ) ;
#16368=ORIENTED_EDGE ( 'NONE', *, *, #42738, .F. ) ;
#16371=DIRECTION ( 'NONE',  ( -1.000000000000000000, 0.000000000000000000, 0.000000000000000000 ) ) ;
#16374=DIRECTION ( 'NONE',  ( 0.000000000000000000, 0.000000000000000000, 1.000000000000000000 ) ) ;
#16376=LINE ( 'NONE', #43571, #10160 ) ;
#16378=CARTESIAN_POINT ( 'NONE',  ( 115.0540265531850395, 2.143131898507847836E-16, 2.568287556927950632 ) ) ;
#16385=ORIENTED_EDGE ( 'NONE', *, *, #24404, .T. ) ;
#16392=VERTEX_POINT ( 'NONE', #32660 ) ;
#16393=PLANE ( 'NONE',  #39580 ) ;
#16395=VERTEX_POINT ( 'NONE', #36273 ) ;
#16401=CYLINDRICAL_SURFACE ( 'NONE', #20002, 1.750000000000015543 ) ;
#16408=CARTESIAN_POINT ( 'NONE',  ( -205.6708471809678827, 1.750000000000009548, 39.79316129108089228 ) ) ;
#16415=CARTESIAN_POINT ( 'NONE',  ( -166.6959734468149463, -1.750000000000009992, 160.8182875569279702 ) ) ;
#16419=EDGE_CURVE ( 'NONE', #18366, #38893, #29167, .T. ) ;
#16420=( BOUNDED_CURVE ( )  B_SPLINE_CURVE ( 3, ( #43524, #12976, #44269, #8394 ),
 .UNSPECIFIED., .F., .F. ) 
 B_SPLINE_CURVE_WITH_KNOTS ( ( 4, 4 ),
 ( 0.000000000000000000, 1.570796326794896558 ),
 .UNSPECIFIED. ) 
 CURVE ( )  GEOMETRIC_REPRESENTATION_ITEM ( )  RATIONAL_B_SPLINE_CURVE ( ( 1.000000000000000000, 0.8047378541243649375, 0.8047378541243649375, 1.000000000000000000 ) ) 
 REPRESENTATION_ITEM ( '' )  );
#16426=CARTESIAN_POINT ( 'NONE',  ( 195.0540265531851105, 2.143131898507880377E-16, 82.56828755692798438 ) ) ;
#16442=DIRECTION ( 'NONE',  ( 0.000000000000000000, 0.000000000000000000, 1.000000000000000000 ) ) ;
#16445=EDGE_CURVE ( 'NONE', #9595, #40596, #23612, .T. ) ;
#16446=( BOUNDED_CURVE ( )  B_SPLINE_CURVE ( 3, ( #11993, #8147, #12980, #9144 ),
 .UNSPECIFIED., .F., .F. ) 
 B_SPLINE_CURVE_WITH_KNOTS ( ( 4, 4 ),
 ( 3.141592653589793116, 4.712388980384689674 ),
 .UNSPECIFIED. ) 
 CURVE ( )  GEOMETRIC_REPRESENTATION_ITEM ( )  RATIONAL_B_SPLINE_CURVE ( ( 1.000000000000000000, 0.8047378541243649375, 0.8047378541243649375, 1.000000000000000000 ) ) 
 REPRESENTATION_ITEM ( '' )  );
#16448=VERTEX_POINT ( 'NONE', #32927 ) ;
#16454=CARTESIAN_POINT ( 'NONE',  ( -88.44597344681497475, 0.000000000000000000, -80.93171244307204404 ) ) ;
#16456=ORIENTED_EDGE ( 'NONE', *, *, #14612, .F. ) ;
#16459=DIRECTION ( 'NONE',  ( 0.000000000000000000, 0.000000000000000000, 1.000000000000000000 ) ) ;
#16461=CARTESIAN_POINT ( 'NONE',  ( 153.3040265531850537, -1.750000000000010658, -79.18171244307201562 ) ) ;
#16472=EDGE_CURVE ( 'NONE', #37466, #21335, #28859, .T. ) ;
#16476=DIRECTION ( 'NONE',  ( 0.000000000000000000, 0.000000000000000000, 1.000000000000000000 ) ) ;
#16480=CYLINDRICAL_SURFACE ( 'NONE', #38596, 1.750000000000015543 ) ;
#16481=ORIENTED_EDGE ( 'NONE', *, *, #11171, .F. ) ;
#16483=DIRECTION ( 'NONE',  ( -1.000000000000000000, 0.000000000000000000, 0.000000000000000000 ) ) ;
#16486=EDGE_LOOP ( 'NONE', ( #36703, #25483, #19559, #3924, #32725, #40221 ) ) ;
#16489=EDGE_CURVE ( 'NONE', #16293, #26090, #34120, .T. ) ;
#16493=CYLINDRICAL_SURFACE ( 'NONE', #47668, 1.750000000000001554 ) ;
#16498=VECTOR ( 'NONE', #48006, 1000.000000000000000 ) ;
#16500=ADVANCED_FACE ( 'NONE', ( #26400 ), #30771, .T. ) ;
#16506=EDGE_CURVE ( 'NONE', #38568, #17971, #4592, .T. ) ;
#16507=DIRECTION ( 'NONE',  ( -1.000000000000000000, 0.000000000000000000, 0.000000000000000000 ) ) ;
#16508=VECTOR ( 'NONE', #38675, 1000.000000000000000 ) ;
#16516=CARTESIAN_POINT ( 'NONE',  ( -44.94597344681493922, -1.025126265847089435, 82.56828755692798438 ) ) ;
#16523=ORIENTED_EDGE ( 'NONE', *, *, #35069, .F. ) ;
#16529=( BOUNDED_CURVE ( )  B_SPLINE_CURVE ( 3, ( #4423, #12613, #1083, #15712 ),
 .UNSPECIFIED., .F., .F. ) 
 B_SPLINE_CURVE_WITH_KNOTS ( ( 4, 4 ),
 ( 0.000000000000000000, 1.570796326794896558 ),
 .UNSPECIFIED. ) 
 CURVE ( )  GEOMETRIC_REPRESENTATION_ITEM ( )  RATIONAL_B_SPLINE_CURVE ( ( 1.000000000000000000, 0.8047378541243649375, 0.8047378541243649375, 1.000000000000000000 ) ) 
 REPRESENTATION_ITEM ( '' )  );
#16532=LINE ( 'NONE', #27831, #45819 ) ;
#16534=CARTESIAN_POINT ( 'NONE',  ( -166.6959734468149463, 1.750000000000010658, 120.8182875569279702 ) ) ;
#16541=ADVANCED_FACE ( 'NONE', ( #7426 ), #50198, .T. ) ;
#16545=DIRECTION ( 'NONE',  ( -0.000000000000000000, -0.000000000000000000, -1.000000000000000000 ) ) ;
#16550=DIRECTION ( 'NONE',  ( -1.000000000000000000, 0.000000000000000000, 0.000000000000000000 ) ) ;
#16551=CARTESIAN_POINT ( 'NONE',  ( 153.3040265531850537, 1.750000000000010658, 80.81828755692798438 ) ) ;
#16552=DIRECTION ( 'NONE',  ( 1.000000000000000000, 0.000000000000000000, 0.000000000000000000 ) ) ;
#16557=EDGE_CURVE ( 'NONE', #14709, #17646, #26905, .T. ) ;
#16558=EDGE_CURVE ( 'NONE', #22009, #48914, #32166, .T. ) ;
#16560=ORIENTED_EDGE ( 'NONE', *, *, #49972, .F. ) ;
#16561=EDGE_LOOP ( 'NONE', ( #41975, #28467, #8053, #3513, #2263, #42035 ) ) ;
#16565=EDGE_CURVE ( 'NONE', #36281, #4790, #39372, .T. ) ;
#16576=CYLINDRICAL_SURFACE ( 'NONE', #32304, 1.750000000000001554 ) ;
#16578=CARTESIAN_POINT ( 'NONE',  ( -208.4459734468149463, 0.000000000000000000, 79.06828755692797017 ) ) ;
#16579=CARTESIAN_POINT ( 'NONE',  ( 35.05402655318504657, -1.025126265847089435, -117.4317124430720156 ) ) ;
#16581=CARTESIAN_POINT ( 'NONE',  ( 154.3291528190321458, 1.750000000000010214, 121.8434138227750623 ) ) ;
#16582=DIRECTION ( 'NONE',  ( -0.000000000000000000, -0.000000000000000000, -1.000000000000000000 ) ) ;
#16583=( BOUNDED_CURVE ( )  B_SPLINE_CURVE ( 3, ( #7101, #14531, #11451, #26849 ),
 .UNSPECIFIED., .F., .F. ) 
 B_SPLINE_CURVE_WITH_KNOTS ( ( 4, 4 ),
 ( 4.712388980384689674, 6.283185307179586232 ),
 .UNSPECIFIED. ) 
 CURVE ( )  GEOMETRIC_REPRESENTATION_ITEM ( )  RATIONAL_B_SPLINE_CURVE ( ( 1.000000000000000000, 0.8047378541243649375, 0.8047378541243649375, 1.000000000000000000 ) ) 
 REPRESENTATION_ITEM ( '' )  );
#16585=( BOUNDED_CURVE ( )  B_SPLINE_CURVE ( 3, ( #13802, #49679, #33585, #29472 ),
 .UNSPECIFIED., .F., .F. ) 
 B_SPLINE_CURVE_WITH_KNOTS ( ( 4, 4 ),
 ( 3.141592653589793116, 4.712388980384689674 ),
 .UNSPECIFIED. ) 
 CURVE ( )  GEOMETRIC_REPRESENTATION_ITEM ( )  RATIONAL_B_SPLINE_CURVE ( ( 1.000000000000000000, 0.8047378541243649375, 0.8047378541243649375, 1.000000000000000000 ) ) 
 REPRESENTATION_ITEM ( '' )  );
#16587=CARTESIAN_POINT ( 'NONE',  ( 210.0000000000000568, 2.143131898507880377E-16, 159.0682875569279702 ) ) ;
#16594=DIRECTION ( 'NONE',  ( -1.000000000000000000, 0.000000000000000000, 0.000000000000000000 ) ) ;
#16597=CARTESIAN_POINT ( 'NONE',  ( -166.6959734468149463, -1.750000000000010214, -39.18171244307202983 ) ) ;
#16607=ORIENTED_EDGE ( 'NONE', *, *, #10830, .F. ) ;
#16609=ORIENTED_EDGE ( 'NONE', *, *, #17142, .T. ) ;
#16611=CYLINDRICAL_SURFACE ( 'NONE', #47921, 1.749999999999973799 ) ;
#16612=CYLINDRICAL_SURFACE ( 'NONE', #28389, 1.750000000000001554 ) ;
#16615=CARTESIAN_POINT ( 'NONE',  ( 73.30402655318508209, 1.750000000000010658, 120.8182875569279702 ) ) ;
#16616=EDGE_LOOP ( 'NONE', ( #38962, #42538, #28807, #30902, #38013, #32335 ) ) ;
#16618=EDGE_LOOP ( 'NONE', ( #45471, #50451, #40645, #19544, #50228 ) ) ;
#16622=CARTESIAN_POINT ( 'NONE',  ( 210.0000000000000568, 2.143131898507880377E-16, -160.9317124430720298 ) ) ;
#16623=CARTESIAN_POINT ( 'NONE',  ( -46.69597344681494633, 0.000000000000000000, 165.0000000000000000 ) ) ;
#16624=ADVANCED_FACE ( 'NONE', ( #39235 ), #729, .T. ) ;
#16625=DIRECTION ( 'NONE',  ( 0.000000000000000000, 0.000000000000000000, 1.000000000000000000 ) ) ;
#16626=CARTESIAN_POINT ( 'NONE',  ( 210.0000000000000568, 2.143131898507880377E-16, -160.9317124430720298 ) ) ;
#16628=CARTESIAN_POINT ( 'NONE',  ( -204.9459734468149463, 2.143131898507880377E-16, -120.9317124430720156 ) ) ;
#16630=VECTOR ( 'NONE', #19202, 1000.000000000000000 ) ;
#16631=CARTESIAN_POINT ( 'NONE',  ( -210.0000000000000568, 0.000000000000000000, 40.81828755692798438 ) ) ;
#16633=CARTESIAN_POINT ( 'NONE',  ( 195.0540265531851105, 2.143131898507880377E-16, 165.0000000000000000 ) ) ;
#16650=ORIENTED_EDGE ( 'NONE', *, *, #42738, .T. ) ;
#16654=EDGE_CURVE ( 'NONE', #26020, #16170, #20013, .T. ) ;
#16655=VERTEX_POINT ( 'NONE', #27423 ) ;
#16659=ORIENTED_EDGE ( 'NONE', *, *, #21594, .T. ) ;
#16669=CARTESIAN_POINT ( 'NONE',  ( 152.2789002873379900, 1.750000000000009548, 81.84341382277507648 ) ) ;
#16675=ORIENTED_EDGE ( 'NONE', *, *, #41057, .F. ) ;
#16677=CARTESIAN_POINT ( 'NONE',  ( -208.4459734468149463, 0.000000000000000000, -37.43171244307205825 ) ) ;
#16678=LINE ( 'NONE', #48187, #40169 ) ;
#16680=AXIS2_PLACEMENT_3D ( 'NONE', #1179, #32224, #29122 ) ;
#16681=ORIENTED_EDGE ( 'NONE', *, *, #32215, .T. ) ;
#16682=CARTESIAN_POINT ( 'NONE',  ( -128.4459734468149179, 0.000000000000000000, 165.0000000000000000 ) ) ;
#16685=FACE_OUTER_BOUND ( 'NONE', #41798, .T. ) ;
#16689=CARTESIAN_POINT ( 'NONE',  ( 191.5540265531850537, -1.025126265847089657, -120.9317124430720440 ) ) ;
#16693=CARTESIAN_POINT ( 'NONE',  ( -48.44597344681495343, 0.000000000000000000, 42.56828755692798438 ) ) ;
#16694=ORIENTED_EDGE ( 'NONE', *, *, #35811, .T. ) ;
#16698=CARTESIAN_POINT ( 'NONE',  ( -168.4459734468149463, 0.000000000000000000, -77.43171244307204404 ) ) ;
#16700=VECTOR ( 'NONE', #6617, 1000.000000000000000 ) ;
#16704=VERTEX_POINT ( 'NONE', #32550 ) ;
#16705=DIRECTION ( 'NONE',  ( 0.000000000000000000, 0.000000000000000000, 1.000000000000000000 ) ) ;
#16706=ORIENTED_EDGE ( 'NONE', *, *, #12832, .T. ) ;
#16708=ORIENTED_EDGE ( 'NONE', *, *, #19513, .T. ) ;
#16714=EDGE_CURVE ( 'NONE', #14077, #4803, #35790, .T. ) ;
#16716=( BOUNDED_CURVE ( )  B_SPLINE_CURVE ( 3, ( #38889, #15277, #22453, #42201 ),
 .UNSPECIFIED., .F., .F. ) 
 B_SPLINE_CURVE_WITH_KNOTS ( ( 4, 4 ),
 ( 3.141592653589793116, 4.712388980384689674 ),
 .UNSPECIFIED. ) 
 CURVE ( )  GEOMETRIC_REPRESENTATION_ITEM ( )  RATIONAL_B_SPLINE_CURVE ( ( 1.000000000000000000, 0.8047378541243649375, 0.8047378541243649375, 1.000000000000000000 ) ) 
 REPRESENTATION_ITEM ( '' )  );
#16723=CYLINDRICAL_SURFACE ( 'NONE', #37997, 1.750000000000001554 ) ;
#16724=FACE_OUTER_BOUND ( 'NONE', #40262, .T. ) ;
#16726=( BOUNDED_CURVE ( )  B_SPLINE_CURVE ( 3, ( #2790, #37471, #34118, #26659 ),
 .UNSPECIFIED., .F., .F. ) 
 B_SPLINE_CURVE_WITH_KNOTS ( ( 4, 4 ),
 ( 4.712388980384689674, 6.283185307179586232 ),
 .UNSPECIFIED. ) 
 CURVE ( )  GEOMETRIC_REPRESENTATION_ITEM ( )  RATIONAL_B_SPLINE_CURVE ( ( 1.000000000000000000, 0.8047378541243649375, 0.8047378541243649375, 1.000000000000000000 ) ) 
 REPRESENTATION_ITEM ( '' )  );
#16728=ORIENTED_EDGE ( 'NONE', *, *, #22387, .T. ) ;
#16730=VERTEX_POINT ( 'NONE', #40492 ) ;
#16734=AXIS2_PLACEMENT_3D ( 'NONE', #46851, #27398, #32018 ) ;
#16737=CARTESIAN_POINT ( 'NONE',  ( -128.4459734468149179, 0.000000000000000000, -120.9317124430720156 ) ) ;
#16739=( BOUNDED_CURVE ( )  B_SPLINE_CURVE ( 3, ( #10434, #10934, #14789, #22237 ),
 .UNSPECIFIED., .F., .F. ) 
 B_SPLINE_CURVE_WITH_KNOTS ( ( 4, 4 ),
 ( 0.000000000000000000, 1.570796326794896558 ),
 .UNSPECIFIED. ) 
 CURVE ( )  GEOMETRIC_REPRESENTATION_ITEM ( )  RATIONAL_B_SPLINE_CURVE ( ( 1.000000000000000000, 0.8047378541243649375, 0.8047378541243649375, 1.000000000000000000 ) ) 
 REPRESENTATION_ITEM ( '' )  );
#16746=CARTESIAN_POINT ( 'NONE',  ( 151.5540265531850537, 0.000000000000000000, -80.93171244307201562 ) ) ;
#16748=EDGE_LOOP ( 'NONE', ( #11420, #49444, #16385, #1870, #48145, #39735 ) ) ;
#16751=VERTEX_POINT ( 'NONE', #17633 ) ;
#16756=ORIENTED_EDGE ( 'NONE', *, *, #33201, .F. ) ;
#16761=CARTESIAN_POINT ( 'NONE',  ( -124.9459734468149463, 2.143131898507847836E-16, 39.06828755692798438 ) ) ;
#16764=VECTOR ( 'NONE', #31357, 1000.000000000000000 ) ;
#16767=VECTOR ( 'NONE', #23320, 1000.000000000000000 ) ;
#16772=CARTESIAN_POINT ( 'NONE',  ( -126.6959734468149321, 0.000000000000000000, 165.0000000000000000 ) ) ;
#16774=ORIENTED_EDGE ( 'NONE', *, *, #29206, .T. ) ;
#16775=AXIS2_PLACEMENT_3D ( 'NONE', #23033, #2530, #22531 ) ;
#16785=EDGE_CURVE ( 'NONE', #20063, #41652, #12825, .T. ) ;
#16786=EDGE_CURVE ( 'NONE', #12663, #44970, #37424, .T. ) ;
#16790=EDGE_CURVE ( 'NONE', #11473, #25384, #18057, .T. ) ;
#16801=FACE_OUTER_BOUND ( 'NONE', #22829, .T. ) ;
#16807=ORIENTED_EDGE ( 'NONE', *, *, #28702, .T. ) ;
#16808=CARTESIAN_POINT ( 'NONE',  ( -46.69597344681494633, -1.750000000000009992, -159.1817124430720298 ) ) ;
#16809=AXIS2_PLACEMENT_3D ( 'NONE', #28190, #4815, #43820 ) ;
#16815=ORIENTED_EDGE ( 'NONE', *, *, #16506, .F. ) ;
#16824=EDGE_LOOP ( 'NONE', ( #25824, #34587, #22810, #34359, #50045, #16650 ) ) ;
#16827=CARTESIAN_POINT ( 'NONE',  ( -210.0000000000000568, 2.143131898507876926E-16, 79.06828755692797017 ) ) ;
#16828=( BOUNDED_CURVE ( )  B_SPLINE_CURVE ( 3, ( #20993, #36412, #9939, #48889 ),
 .UNSPECIFIED., .F., .F. ) 
 B_SPLINE_CURVE_WITH_KNOTS ( ( 4, 4 ),
 ( 4.712388980384689674, 6.283185307179586232 ),
 .UNSPECIFIED. ) 
 CURVE ( )  GEOMETRIC_REPRESENTATION_ITEM ( )  RATIONAL_B_SPLINE_CURVE ( ( 1.000000000000000000, 0.8047378541243649375, 0.8047378541243649375, 1.000000000000000000 ) ) 
 REPRESENTATION_ITEM ( '' )  );
#16829=FACE_OUTER_BOUND ( 'NONE', #48406, .T. ) ;
#16831=EDGE_CURVE ( 'NONE', #30864, #48470, #18131, .T. ) ;
#16832=DIRECTION ( 'NONE',  ( -0.000000000000000000, -0.000000000000000000, -1.000000000000000000 ) ) ;
#16838=CARTESIAN_POINT ( 'NONE',  ( 195.0540265531851105, 2.143131898507880377E-16, -0.9317124430720247208 ) ) ;
#16839=CARTESIAN_POINT ( 'NONE',  ( 153.3040265531850537, 0.000000000000000000, -165.0000000000000000 ) ) ;
#16840=VECTOR ( 'NONE', #2370, 1000.000000000000000 ) ;
#16841=DIRECTION ( 'NONE',  ( 0.000000000000000000, 0.000000000000000000, 1.000000000000000000 ) ) ;
#16846=EDGE_CURVE ( 'NONE', #5769, #42417, #9819, .T. ) ;
#16847=ADVANCED_FACE ( 'NONE', ( #37916 ), #2732, .T. ) ;
#16853=CARTESIAN_POINT ( 'NONE',  ( -204.9459734468148895, -1.025126265847089435, -77.43171244307200141 ) ) ;
#16858=VERTEX_POINT ( 'NONE', #7358 ) ;
#16863=EDGE_CURVE ( 'NONE', #27926, #41541, #6847, .T. ) ;
#16864=ORIENTED_EDGE ( 'NONE', *, *, #15636, .T. ) ;
#16869=CARTESIAN_POINT ( 'NONE',  ( -8.445973446814976526, 0.000000000000000000, 2.568287556928034121 ) ) ;
#16873=DIRECTION ( 'NONE',  ( -0.000000000000000000, -0.000000000000000000, -1.000000000000000000 ) ) ;
#16878=ORIENTED_EDGE ( 'NONE', *, *, #3110, .T. ) ;
#16887=CARTESIAN_POINT ( 'NONE',  ( -84.94597344681493212, -1.025126265847089435, 162.5682875569279133 ) ) ;
#16888=CARTESIAN_POINT ( 'NONE',  ( -6.695973446814940111, -1.750000000000023315, 0.8182875569279768335 ) ) ;
#16889=( BOUNDED_CURVE ( )  B_SPLINE_CURVE ( 3, ( #48494, #37772, #5684, #45158 ),
 .UNSPECIFIED., .F., .F. ) 
 B_SPLINE_CURVE_WITH_KNOTS ( ( 4, 4 ),
 ( 3.141592653589793116, 4.712388980384689674 ),
 .UNSPECIFIED. ) 
 CURVE ( )  GEOMETRIC_REPRESENTATION_ITEM ( )  RATIONAL_B_SPLINE_CURVE ( ( 1.000000000000000000, 0.8047378541243649375, 0.8047378541243649375, 1.000000000000000000 ) ) 
 REPRESENTATION_ITEM ( '' )  );
#16896=( BOUNDED_CURVE ( )  B_SPLINE_CURVE ( 3, ( #48828, #21415, #41680, #37600 ),
 .UNSPECIFIED., .F., .F. ) 
 B_SPLINE_CURVE_WITH_KNOTS ( ( 4, 4 ),
 ( 4.712388980384689674, 6.283185307179586232 ),
 .UNSPECIFIED. ) 
 CURVE ( )  GEOMETRIC_REPRESENTATION_ITEM ( )  RATIONAL_B_SPLINE_CURVE ( ( 1.000000000000000000, 0.8047378541243649375, 0.8047378541243649375, 1.000000000000000000 ) ) 
 REPRESENTATION_ITEM ( '' )  );
#16897=FACE_OUTER_BOUND ( 'NONE', #26111, .T. ) ;
#16898=CARTESIAN_POINT ( 'NONE',  ( -124.9459734468149321, -1.025126265847081886, 119.0682875569279702 ) ) ;
#16905=DIRECTION ( 'NONE',  ( -0.000000000000000000, -0.000000000000000000, -1.000000000000000000 ) ) ;
#16907=DIRECTION ( 'NONE',  ( -1.000000000000000000, -0.000000000000000000, -0.000000000000000000 ) ) ;
#16916=AXIS2_PLACEMENT_3D ( 'NONE', #1299, #16947, #33300 ) ;
#16919=CARTESIAN_POINT ( 'NONE',  ( 75.05402655318509630, -1.025126265847089657, -120.9317124430720440 ) ) ;
#16920=CARTESIAN_POINT ( 'NONE',  ( -44.94597344681493922, 2.143131898507880377E-16, -0.9317124430720247208 ) ) ;
#16921=ORIENTED_EDGE ( 'NONE', *, *, #16506, .T. ) ;
#16922=LINE ( 'NONE', #31572, #8551 ) ;
#16924=ORIENTED_EDGE ( 'NONE', *, *, #44782, .F. ) ;
#16927=AXIS2_PLACEMENT_3D ( 'NONE', #34285, #33529, #41212 ) ;
#16930=DIRECTION ( 'NONE',  ( 0.000000000000000000, 0.000000000000000000, 1.000000000000000000 ) ) ;
#16937=ORIENTED_EDGE ( 'NONE', *, *, #11810, .T. ) ;
#16940=ORIENTED_EDGE ( 'NONE', *, *, #28017, .T. ) ;
#16941=LINE ( 'NONE', #17180, #2965 ) ;
#16945=CARTESIAN_POINT ( 'NONE',  ( -210.0000000000000568, 2.143131898507890731E-16, 159.0682875569279702 ) ) ;
#16946=VERTEX_POINT ( 'NONE', #43256 ) ;
#16947=DIRECTION ( 'NONE',  ( -1.000000000000000000, -0.000000000000000000, -0.000000000000000000 ) ) ;
#16953=CARTESIAN_POINT ( 'NONE',  ( -4.945973446814917018, 1.025126265847097207, -40.93171244307204404 ) ) ;
#16956=ORIENTED_EDGE ( 'NONE', *, *, #18888, .F. ) ;
#16957=EDGE_CURVE ( 'NONE', #36969, #12576, #3178, .T. ) ;
#16960=CARTESIAN_POINT ( 'NONE',  ( 113.3040265531850537, -1.749999999999997335, -79.18171244307201562 ) ) ;
#16961=CYLINDRICAL_SURFACE ( 'NONE', #7634, 1.750000000000015543 ) ;
#16965=CARTESIAN_POINT ( 'NONE',  ( -164.9459734468149463, 2.143131898507880377E-16, 165.0000000000000000 ) ) ;
#16973=DIRECTION ( 'NONE',  ( -1.000000000000000000, -0.000000000000000000, -0.000000000000000000 ) ) ;
#16975=VERTEX_POINT ( 'NONE', #24285 ) ;
#16985=DIRECTION ( 'NONE',  ( -0.000000000000000000, -0.000000000000000000, -1.000000000000000000 ) ) ;
#16991=CARTESIAN_POINT ( 'NONE',  ( 192.2789002873380184, 1.750000000000009326, -158.1565861772249377 ) ) ;
#16993=ORIENTED_EDGE ( 'NONE', *, *, #13920, .T. ) ;
#16999=DIRECTION ( 'NONE',  ( -1.000000000000000000, 0.000000000000000000, 0.000000000000000000 ) ) ;
#17008=CARTESIAN_POINT ( 'NONE',  ( -44.94597344681493922, 2.143131898507880377E-16, 82.56828755692798438 ) ) ;
#17012=CARTESIAN_POINT ( 'NONE',  ( -6.695973446814940111, 1.750000000000024203, -119.1817124430720440 ) ) ;
#17013=CARTESIAN_POINT ( 'NONE',  ( 153.3040265531850537, -1.750000000000009992, -159.1817124430720298 ) ) ;
#17015=CARTESIAN_POINT ( 'NONE',  ( 195.0540265531851105, 2.143131898507880377E-16, 165.0000000000000000 ) ) ;
#17017=CARTESIAN_POINT ( 'NONE',  ( -126.6959734468149321, 1.749999999999996891, 0.8182875569279768335 ) ) ;
#17018=VERTEX_POINT ( 'NONE', #24025 ) ;
#17019=DIRECTION ( 'NONE',  ( -0.000000000000000000, -0.000000000000000000, -1.000000000000000000 ) ) ;
#17020=CYLINDRICAL_SURFACE ( 'NONE', #37578, 1.750000000000001554 ) ;
#17021=CYLINDRICAL_SURFACE ( 'NONE', #34838, 1.750000000000036193 ) ;
#17022=( BOUNDED_CURVE ( )  B_SPLINE_CURVE ( 3, ( #17984, #21861, #48989, #13875 ),
 .UNSPECIFIED., .F., .F. ) 
 B_SPLINE_CURVE_WITH_KNOTS ( ( 4, 4 ),
 ( 1.570796326794896558, 3.141592653589793116 ),
 .UNSPECIFIED. ) 
 CURVE ( )  GEOMETRIC_REPRESENTATION_ITEM ( )  RATIONAL_B_SPLINE_CURVE ( ( 1.000000000000000000, 0.8047378541243649375, 0.8047378541243649375, 1.000000000000000000 ) ) 
 REPRESENTATION_ITEM ( '' )  );
#17028=( BOUNDED_CURVE ( )  B_SPLINE_CURVE ( 3, ( #17008, #16516, #23704, #48261 ),
 .UNSPECIFIED., .F., .F. ) 
 B_SPLINE_CURVE_WITH_KNOTS ( ( 4, 4 ),
 ( 3.141592653589793116, 4.712388980384689674 ),
 .UNSPECIFIED. ) 
 CURVE ( )  GEOMETRIC_REPRESENTATION_ITEM ( )  RATIONAL_B_SPLINE_CURVE ( ( 1.000000000000000000, 0.8047378541243649375, 0.8047378541243649375, 1.000000000000000000 ) ) 
 REPRESENTATION_ITEM ( '' )  );
#17029=CARTESIAN_POINT ( 'NONE',  ( 73.30402655318508209, -1.750000000000009992, 0.8182875569279768335 ) ) ;
#17030=CARTESIAN_POINT ( 'NONE',  ( -167.7210997126620384, 1.750000000000010436, 119.7931612910808781 ) ) ;
#17032=EDGE_CURVE ( 'NONE', #2259, #10372, #15562, .T. ) ;
#17036=LINE ( 'NONE', #9592, #19613 ) ;
#17037=CARTESIAN_POINT ( 'NONE',  ( -165.6708471809677974, -1.750000000000009548, 81.84341382277507648 ) ) ;
#17039=( BOUNDED_CURVE ( )  B_SPLINE_CURVE ( 3, ( #30182, #42238, #10186, #30442 ),
 .UNSPECIFIED., .F., .F. ) 
 B_SPLINE_CURVE_WITH_KNOTS ( ( 4, 4 ),
 ( 0.000000000000000000, 1.570796326794896558 ),
 .UNSPECIFIED. ) 
 CURVE ( )  GEOMETRIC_REPRESENTATION_ITEM ( )  RATIONAL_B_SPLINE_CURVE ( ( 1.000000000000000000, 0.8047378541243649375, 0.8047378541243649375, 1.000000000000000000 ) ) 
 REPRESENTATION_ITEM ( '' )  );
#17049=CARTESIAN_POINT ( 'NONE',  ( 71.55402655318505367, 0.000000000000000000, 82.56828755692799859 ) ) ;
#17051=CARTESIAN_POINT ( 'NONE',  ( 111.5540265531850679, 0.000000000000000000, -120.9317124430720156 ) ) ;
#17059=EDGE_LOOP ( 'NONE', ( #9401, #2479, #3015, #3540, #43921 ) ) ;
#17060=CARTESIAN_POINT ( 'NONE',  ( -7.721099712662037540, -1.750000000000023537, -78.15658617722490931 ) ) ;
#17068=ORIENTED_EDGE ( 'NONE', *, *, #48982, .T. ) ;
#17077=CARTESIAN_POINT ( 'NONE',  ( 195.0540265531851105, 2.143131898507880377E-16, 165.0000000000000000 ) ) ;
#17078=EDGE_CURVE ( 'NONE', #42683, #46160, #24489, .T. ) ;
#17079=FACE_OUTER_BOUND ( 'NONE', #5664, .T. ) ;
#17083=( BOUNDED_CURVE ( )  B_SPLINE_CURVE ( 3, ( #46944, #19785, #50, #307 ),
 .UNSPECIFIED., .F., .F. ) 
 B_SPLINE_CURVE_WITH_KNOTS ( ( 4, 4 ),
 ( 0.000000000000000000, 1.570796326794896558 ),
 .UNSPECIFIED. ) 
 CURVE ( )  GEOMETRIC_REPRESENTATION_ITEM ( )  RATIONAL_B_SPLINE_CURVE ( ( 1.000000000000000000, 0.8047378541243649375, 0.8047378541243649375, 1.000000000000000000 ) ) 
 REPRESENTATION_ITEM ( '' )  );
#17089=ORIENTED_EDGE ( 'NONE', *, *, #15929, .T. ) ;
#17090=CARTESIAN_POINT ( 'NONE',  ( 72.27890028733797578, -1.750000000000009548, -160.2068387089191219 ) ) ;
#17093=DIRECTION ( 'NONE',  ( -1.000000000000000000, 0.000000000000000000, 0.000000000000000000 ) ) ;
#17095=CYLINDRICAL_SURFACE ( 'NONE', #17580, 1.750000000000001554 ) ;
#17097=EDGE_LOOP ( 'NONE', ( #31766, #10654, #19404, #46347, #34873, #19988 ) ) ;
#17101=CARTESIAN_POINT ( 'NONE',  ( -166.6959734468149463, 1.750000000000010214, -39.18171244307202983 ) ) ;
#17103=CARTESIAN_POINT ( 'NONE',  ( 31.55402655318503236, -1.025126265847089657, -120.9317124430720440 ) ) ;
#17105=DIRECTION ( 'NONE',  ( -1.000000000000000000, 0.000000000000000000, 0.000000000000000000 ) ) ;
#17106=LINE ( 'NONE', #5043, #22442 ) ;
#17107=VERTEX_POINT ( 'NONE', #17823 ) ;
#17112=CARTESIAN_POINT ( 'NONE',  ( 115.0540265531850395, 2.143131898507847836E-16, 79.06828755692798438 ) ) ;
#17113=FACE_OUTER_BOUND ( 'NONE', #14843, .T. ) ;
#17120=( BOUNDED_CURVE ( )  B_SPLINE_CURVE ( 3, ( #26398, #35653, #47631, #23571 ),
 .UNSPECIFIED., .F., .F. ) 
 B_SPLINE_CURVE_WITH_KNOTS ( ( 4, 4 ),
 ( 4.712388980384689674, 6.283185307179586232 ),
 .UNSPECIFIED. ) 
 CURVE ( )  GEOMETRIC_REPRESENTATION_ITEM ( )  RATIONAL_B_SPLINE_CURVE ( ( 1.000000000000000000, 0.8047378541243649375, 0.8047378541243649375, 1.000000000000000000 ) ) 
 REPRESENTATION_ITEM ( '' )  );
#17123=VERTEX_POINT ( 'NONE', #17323 ) ;
#17125=VECTOR ( 'NONE', #22120, 1000.000000000000000 ) ;
#17126=CIRCLE ( 'NONE', #9751, 1.750000000000015543 ) ;
#17134=CARTESIAN_POINT ( 'NONE',  ( 113.3040265531850537, 1.749999999999997113, -39.18171244307202983 ) ) ;
#17136=EDGE_CURVE ( 'NONE', #42553, #46647, #20314, .T. ) ;
#17142=EDGE_CURVE ( 'NONE', #9269, #9029, #44004, .T. ) ;
#17146=ORIENTED_EDGE ( 'NONE', *, *, #25699, .T. ) ;
#17147=CARTESIAN_POINT ( 'NONE',  ( -128.4459734468149179, 0.000000000000000000, 165.0000000000000000 ) ) ;
#17148=CARTESIAN_POINT ( 'NONE',  ( 35.05402655318504657, -1.025126265847089657, -80.93171244307201562 ) ) ;
#17157=VERTEX_POINT ( 'NONE', #16827 ) ;
#17164=ORIENTED_EDGE ( 'NONE', *, *, #21501, .T. ) ;
#17167=ORIENTED_EDGE ( 'NONE', *, *, #6401, .F. ) ;
#17169=CARTESIAN_POINT ( 'NONE',  ( 210.0000000000000568, 0.000000000000000000, 42.56828755692799149 ) ) ;
#17172=DIRECTION ( 'NONE',  ( -1.000000000000000000, -0.000000000000000000, -0.000000000000000000 ) ) ;
#17177=DIRECTION ( 'NONE',  ( 1.000000000000000000, 0.000000000000000000, 0.000000000000000000 ) ) ;
#17178=( BOUNDED_CURVE ( )  B_SPLINE_CURVE ( 3, ( #31235, #49892, #46570, #14802 ),
 .UNSPECIFIED., .F., .F. ) 
 B_SPLINE_CURVE_WITH_KNOTS ( ( 4, 4 ),
 ( 3.141592653589793116, 4.712388980384689674 ),
 .UNSPECIFIED. ) 
 CURVE ( )  GEOMETRIC_REPRESENTATION_ITEM ( )  RATIONAL_B_SPLINE_CURVE ( ( 1.000000000000000000, 0.8047378541243649375, 0.8047378541243649375, 1.000000000000000000 ) ) 
 REPRESENTATION_ITEM ( '' )  );
#17180=CARTESIAN_POINT ( 'NONE',  ( 210.0000000000000568, 0.000000000000000000, 2.568287556927987048 ) ) ;
#17182=ORIENTED_EDGE ( 'NONE', *, *, #12727, .T. ) ;
#17186=( BOUNDED_CURVE ( )  B_SPLINE_CURVE ( 3, ( #2242, #49890, #45571, #18386 ),
 .UNSPECIFIED., .F., .F. ) 
 B_SPLINE_CURVE_WITH_KNOTS ( ( 4, 4 ),
 ( 4.712388980384689674, 6.283185307179586232 ),
 .UNSPECIFIED. ) 
 CURVE ( )  GEOMETRIC_REPRESENTATION_ITEM ( )  RATIONAL_B_SPLINE_CURVE ( ( 1.000000000000000000, 0.8047378541243649375, 0.8047378541243649375, 1.000000000000000000 ) ) 
 REPRESENTATION_ITEM ( '' )  );
#17187=CARTESIAN_POINT ( 'NONE',  ( 71.55402655318505367, 0.000000000000000000, -0.9317124430720524764 ) ) ;
#17194=EDGE_CURVE ( 'NONE', #8176, #29055, #42628, .T. ) ;
#17197=VERTEX_POINT ( 'NONE', #18822 ) ;
#17198=FACE_OUTER_BOUND ( 'NONE', #14106, .T. ) ;
#17199=FACE_OUTER_BOUND ( 'NONE', #49114, .T. ) ;
#17207=EDGE_CURVE ( 'NONE', #38997, #11761, #34504, .T. ) ;
#17214=CARTESIAN_POINT ( 'NONE',  ( 113.3040265531850537, 1.749999999999997335, -79.18171244307201562 ) ) ;
#17215=ADVANCED_FACE ( 'NONE', ( #3430 ), #26797, .T. ) ;
#17217=DIRECTION ( 'NONE',  ( 0.000000000000000000, 0.000000000000000000, 1.000000000000000000 ) ) ;
#17220=CARTESIAN_POINT ( 'NONE',  ( -167.7210997126620384, 1.750000000000009326, 1.843413822775066269 ) ) ;
#17223=ORIENTED_EDGE ( 'NONE', *, *, #18160, .F. ) ;
#17224=CARTESIAN_POINT ( 'NONE',  ( 193.3040265531851105, -1.750000000000010658, -79.18171244307201562 ) ) ;
#17227=AXIS2_PLACEMENT_3D ( 'NONE', #30937, #3447, #35297 ) ;
#17229=CARTESIAN_POINT ( 'NONE',  ( -204.9459734468149463, 2.143131898507880377E-16, -80.93171244307201562 ) ) ;
#17231=VECTOR ( 'NONE', #38358, 1000.000000000000000 ) ;
#17232=CARTESIAN_POINT ( 'NONE',  ( 210.0000000000000568, 0.000000000000000000, -79.18171244307201562 ) ) ;
#17233=LINE ( 'NONE', #32899, #34743 ) ;
#17235=CYLINDRICAL_SURFACE ( 'NONE', #5730, 1.750000000000001554 ) ;
#17241=ORIENTED_EDGE ( 'NONE', *, *, #21949, .F. ) ;
#17245=CARTESIAN_POINT ( 'NONE',  ( 113.3040265531850537, -1.749999999999997335, 80.81828755692798438 ) ) ;
#17247=EDGE_LOOP ( 'NONE', ( #10263, #11730, #48254, #2782, #43801, #36395 ) ) ;
#17250=ORIENTED_EDGE ( 'NONE', *, *, #30204, .F. ) ;
#17256=VERTEX_POINT ( 'NONE', #37857 ) ;
#17263=CARTESIAN_POINT ( 'NONE',  ( 210.0000000000000568, 0.000000000000000000, -157.4317124430720298 ) ) ;
#17267=CARTESIAN_POINT ( 'NONE',  ( 210.0000000000000568, 0.000000000000000000, 40.81828755692798438 ) ) ;
#17269=VECTOR ( 'NONE', #1896, 1000.000000000000000 ) ;
#17270=DIRECTION ( 'NONE',  ( -1.000000000000000000, -0.000000000000000000, -0.000000000000000000 ) ) ;
#17271=FACE_OUTER_BOUND ( 'NONE', #7589, .T. ) ;
#17282=ORIENTED_EDGE ( 'NONE', *, *, #15864, .T. ) ;
#17283=CARTESIAN_POINT ( 'NONE',  ( 72.27890028733797578, 1.750000000000010436, -80.20683870891910772 ) ) ;
#17285=CYLINDRICAL_SURFACE ( 'NONE', #39330, 1.749999999999987566 ) ;
#17297=AXIS2_PLACEMENT_3D ( 'NONE', #50111, #47037, #42213 ) ;
#17301=CARTESIAN_POINT ( 'NONE',  ( -86.69597344681494633, 1.750000000000010658, 80.81828755692798438 ) ) ;
#17303=CARTESIAN_POINT ( 'NONE',  ( 112.2789002873379758, -1.749999999999996891, 79.79316129108087807 ) ) ;
#17310=VERTEX_POINT ( 'NONE', #45246 ) ;
#17311=VERTEX_POINT ( 'NONE', #22937 ) ;
#17312=CARTESIAN_POINT ( 'NONE',  ( 35.05402655318504657, 2.143131898507880377E-16, -0.9317124430720247208 ) ) ;
#17313=DIRECTION ( 'NONE',  ( -1.000000000000000000, -0.000000000000000000, -0.000000000000000000 ) ) ;
#17320=( BOUNDED_CURVE ( )  B_SPLINE_CURVE ( 3, ( #13106, #44392, #9267, #24927 ),
 .UNSPECIFIED., .F., .F. ) 
 B_SPLINE_CURVE_WITH_KNOTS ( ( 4, 4 ),
 ( 1.570796326794896558, 3.141592653589793116 ),
 .UNSPECIFIED. ) 
 CURVE ( )  GEOMETRIC_REPRESENTATION_ITEM ( )  RATIONAL_B_SPLINE_CURVE ( ( 1.000000000000000000, 0.8047378541243649375, 0.8047378541243649375, 1.000000000000000000 ) ) 
 REPRESENTATION_ITEM ( '' )  );
#17323=CARTESIAN_POINT ( 'NONE',  ( 113.3040265531850537, -1.749999999999996891, -159.1817124430720298 ) ) ;
#17324=CARTESIAN_POINT ( 'NONE',  ( -204.9459734468149463, 2.143131898507880377E-16, 165.0000000000000000 ) ) ;
#17326=EDGE_CURVE ( 'NONE', #936, #48234, #21936, .T. ) ;
#17327=CARTESIAN_POINT ( 'NONE',  ( -6.695973446814940111, 1.750000000000023315, 160.8182875569279702 ) ) ;
#17328=( BOUNDED_CURVE ( )  B_SPLINE_CURVE ( 3, ( #14157, #33443, #21114, #21884 ),
 .UNSPECIFIED., .F., .F. ) 
 B_SPLINE_CURVE_WITH_KNOTS ( ( 4, 4 ),
 ( 3.141592653589793116, 4.712388980384689674 ),
 .UNSPECIFIED. ) 
 CURVE ( )  GEOMETRIC_REPRESENTATION_ITEM ( )  RATIONAL_B_SPLINE_CURVE ( ( 1.000000000000000000, 0.8047378541243649375, 0.8047378541243649375, 1.000000000000000000 ) ) 
 REPRESENTATION_ITEM ( '' )  );
#17335=CARTESIAN_POINT ( 'NONE',  ( 31.55402655318503236, -1.025126265847089879, 122.5682875569280128 ) ) ;
#17337=EDGE_CURVE ( 'NONE', #44970, #34157, #41294, .T. ) ;
#17338=( BOUNDED_CURVE ( )  B_SPLINE_CURVE ( 3, ( #32746, #12471, #1452, #35856 ),
 .UNSPECIFIED., .F., .F. ) 
 B_SPLINE_CURVE_WITH_KNOTS ( ( 4, 4 ),
 ( 3.141592653589793116, 4.712388980384689674 ),
 .UNSPECIFIED. ) 
 CURVE ( )  GEOMETRIC_REPRESENTATION_ITEM ( )  RATIONAL_B_SPLINE_CURVE ( ( 1.000000000000000000, 0.8047378541243649375, 0.8047378541243649375, 1.000000000000000000 ) ) 
 REPRESENTATION_ITEM ( '' )  );
#17342=CARTESIAN_POINT ( 'NONE',  ( 112.2789002873379758, 1.749999999999996669, 121.8434138227750481 ) ) ;
#17344=CYLINDRICAL_SURFACE ( 'NONE', #46644, 1.750000000000008438 ) ;
#17346=CARTESIAN_POINT ( 'NONE',  ( 210.0000000000000568, 0.000000000000000000, -117.4317124430720298 ) ) ;
#17353=CARTESIAN_POINT ( 'NONE',  ( 111.5540265531850679, 0.000000000000000000, 119.0682875569279844 ) ) ;
#17356=ORIENTED_EDGE ( 'NONE', *, *, #32906, .T. ) ;
#17357=CARTESIAN_POINT ( 'NONE',  ( 33.30402655318503946, 1.750000000000010658, 80.81828755692798438 ) ) ;
#17364=CARTESIAN_POINT ( 'NONE',  ( -124.9459734468149321, -1.025126265847081442, -160.9317124430720014 ) ) ;
#17365=CARTESIAN_POINT ( 'NONE',  ( 210.0000000000000568, 0.000000000000000000, 80.81828755692798438 ) ) ;
#17366=ORIENTED_EDGE ( 'NONE', *, *, #5322, .F. ) ;
#17370=LINE ( 'NONE', #13005, #796 ) ;
#17377=CARTESIAN_POINT ( 'NONE',  ( 210.0000000000000568, 0.000000000000000000, -117.4317124430720298 ) ) ;
#17378=DIRECTION ( 'NONE',  ( -1.000000000000000000, -0.000000000000000000, -0.000000000000000000 ) ) ;
#17380=DIRECTION ( 'NONE',  ( -1.000000000000000000, -0.000000000000000000, -0.000000000000000000 ) ) ;
#17382=EDGE_CURVE ( 'NONE', #49918, #24712, #31162, .T. ) ;
#17383=CARTESIAN_POINT ( 'NONE',  ( -204.9459734468149463, 2.143131898507880377E-16, 42.56828755692798438 ) ) ;
#17388=DIRECTION ( 'NONE',  ( 0.000000000000000000, 0.000000000000000000, 1.000000000000000000 ) ) ;
#17389=DIRECTION ( 'NONE',  ( -0.000000000000000000, -0.000000000000000000, -1.000000000000000000 ) ) ;
#17390=EDGE_CURVE ( 'NONE', #40762, #10372, #23305, .T. ) ;
#17392=CARTESIAN_POINT ( 'NONE',  ( 192.2789002873380184, -1.750000000000009548, 159.7931612910809065 ) ) ;
#17395=CARTESIAN_POINT ( 'NONE',  ( -204.9459734468149463, 2.143131898507880377E-16, 82.56828755692798438 ) ) ;
#17401=ORIENTED_EDGE ( 'NONE', *, *, #16557, .T. ) ;
#17402=CYLINDRICAL_SURFACE ( 'NONE', #33055, 1.750000000000001554 ) ;
#17404=CARTESIAN_POINT ( 'NONE',  ( -47.72109971266203132, 1.750000000000009548, 161.8434138227750907 ) ) ;
#17414=CARTESIAN_POINT ( 'NONE',  ( 153.3040265531850537, 0.000000000000000000, 165.0000000000000000 ) ) ;
#17417=ORIENTED_EDGE ( 'NONE', *, *, #26161, .T. ) ;
#17418=CARTESIAN_POINT ( 'NONE',  ( 191.5540265531851105, 0.000000000000000000, 79.06828755692797017 ) ) ;
#17420=EDGE_LOOP ( 'NONE', ( #45228, #39412, #24729, #37967, #3080 ) ) ;
#17421=CARTESIAN_POINT ( 'NONE',  ( 153.3040265531850537, -1.750000000000010658, 80.81828755692798438 ) ) ;
#17426=EDGE_CURVE ( 'NONE', #45594, #28550, #8070, .T. ) ;
#17430=EDGE_LOOP ( 'NONE', ( #1030, #7963, #9916, #13006, #13568, #28415 ) ) ;
#17434=AXIS2_PLACEMENT_3D ( 'NONE', #26036, #27755, #571 ) ;
#17436=VERTEX_POINT ( 'NONE', #39125 ) ;
#17438=AXIS2_PLACEMENT_3D ( 'NONE', #43574, #40001, #20234 ) ;
#17439=CARTESIAN_POINT ( 'NONE',  ( -166.6959734468149463, -1.750000000000010658, 120.8182875569279702 ) ) ;
#17441=VECTOR ( 'NONE', #7953, 1000.000000000000000 ) ;
#17444=CARTESIAN_POINT ( 'NONE',  ( 193.3040265531851105, 1.750000000000009992, 160.8182875569279702 ) ) ;
#17445=EDGE_CURVE ( 'NONE', #38893, #8676, #36071, .T. ) ;
#17450=CARTESIAN_POINT ( 'NONE',  ( 75.05402655318509630, 1.025126265847089879, -117.4317124430720156 ) ) ;
#17453=DIRECTION ( 'NONE',  ( 1.000000000000000000, 0.000000000000000000, 0.000000000000000000 ) ) ;
#17456=FACE_OUTER_BOUND ( 'NONE', #45392, .T. ) ;
#17458=CARTESIAN_POINT ( 'NONE',  ( -166.6959734468149463, 0.000000000000000000, 165.0000000000000000 ) ) ;
#17461=FACE_OUTER_BOUND ( 'NONE', #44318, .T. ) ;
#17464=ORIENTED_EDGE ( 'NONE', *, *, #41775, .F. ) ;
#17474=EDGE_CURVE ( 'NONE', #46647, #40582, #46497, .T. ) ;
#17477=VECTOR ( 'NONE', #39063, 1000.000000000000000 ) ;
#17479=CARTESIAN_POINT ( 'NONE',  ( -86.69597344681494633, 1.750000000000009992, 0.8182875569279768335 ) ) ;
#17484=( BOUNDED_CURVE ( )  B_SPLINE_CURVE ( 3, ( #38865, #27305, #3689, #12402 ),
 .UNSPECIFIED., .F., .F. ) 
 B_SPLINE_CURVE_WITH_KNOTS ( ( 4, 4 ),
 ( 4.712388980384689674, 6.283185307179586232 ),
 .UNSPECIFIED. ) 
 CURVE ( )  GEOMETRIC_REPRESENTATION_ITEM ( )  RATIONAL_B_SPLINE_CURVE ( ( 1.000000000000000000, 0.8047378541243649375, 0.8047378541243649375, 1.000000000000000000 ) ) 
 REPRESENTATION_ITEM ( '' )  );
#17485=EDGE_LOOP ( 'NONE', ( #5929, #3503, #12201, #46522, #2936, #979 ) ) ;
#17490=EDGE_CURVE ( 'NONE', #36250, #34589, #995, .T. ) ;
#17492=CARTESIAN_POINT ( 'NONE',  ( 115.0540265531850395, 2.143131898507847836E-16, 165.0000000000000000 ) ) ;
#17495=DIRECTION ( 'NONE',  ( 0.000000000000000000, 0.000000000000000000, 1.000000000000000000 ) ) ;
#17498=ORIENTED_EDGE ( 'NONE', *, *, #19984, .F. ) ;
#17501=CARTESIAN_POINT ( 'NONE',  ( 31.55402655318503236, -1.025126265847089213, -0.9317124430720324924 ) ) ;
#17505=AXIS2_PLACEMENT_3D ( 'NONE', #40333, #78, #16483 ) ;
#17506=ORIENTED_EDGE ( 'NONE', *, *, #45038, .T. ) ;
#17514=ORIENTED_EDGE ( 'NONE', *, *, #15062, .F. ) ;
#17521=DIRECTION ( 'NONE',  ( -1.000000000000000000, 0.000000000000000000, 0.000000000000000000 ) ) ;
#17522=ORIENTED_EDGE ( 'NONE', *, *, #37753, .F. ) ;
#17525=DIRECTION ( 'NONE',  ( 0.000000000000000000, 0.000000000000000000, 1.000000000000000000 ) ) ;
#17533=CARTESIAN_POINT ( 'NONE',  ( 71.55402655318505367, 0.000000000000000000, -77.43171244307198720 ) ) ;
#17538=EDGE_CURVE ( 'NONE', #24424, #2781, #6241, .T. ) ;
#17545=CARTESIAN_POINT ( 'NONE',  ( -207.7210997126620384, -1.750000000000009548, -40.20683870891912193 ) ) ;
#17546=VECTOR ( 'NONE', #26996, 1000.000000000000000 ) ;
#17548=ORIENTED_EDGE ( 'NONE', *, *, #49281, .T. ) ;
#17552=EDGE_CURVE ( 'NONE', #31866, #6992, #39070, .T. ) ;
#17554=ORIENTED_EDGE ( 'NONE', *, *, #17390, .T. ) ;
#17557=CARTESIAN_POINT ( 'NONE',  ( -204.9459734468149463, 2.143131898507880377E-16, 79.06828755692797017 ) ) ;
#17558=CARTESIAN_POINT ( 'NONE',  ( 210.0000000000000568, 0.000000000000000000, 82.56828755692799859 ) ) ;
#17563=CARTESIAN_POINT ( 'NONE',  ( 195.0540265531851105, 1.025126265847089657, 119.0682875569279560 ) ) ;
#17569=ORIENTED_EDGE ( 'NONE', *, *, #27525, .T. ) ;
#17576=DIRECTION ( 'NONE',  ( -1.000000000000000000, -0.000000000000000000, -0.000000000000000000 ) ) ;
#17578=CARTESIAN_POINT ( 'NONE',  ( -44.94597344681493922, -1.025126265847089657, -120.9317124430720440 ) ) ;
#17579=ORIENTED_EDGE ( 'NONE', *, *, #35008, .F. ) ;
#17580=AXIS2_PLACEMENT_3D ( 'NONE', #9399, #40456, #25058 ) ;
#17581=CARTESIAN_POINT ( 'NONE',  ( 113.3040265531850537, -1.749999999999997113, 40.81828755692798438 ) ) ;
#17588=CARTESIAN_POINT ( 'NONE',  ( 73.30402655318508209, -1.750000000000010658, 120.8182875569279702 ) ) ;
#17593=CARTESIAN_POINT ( 'NONE',  ( -166.6959734468149463, 0.000000000000000000, 165.0000000000000000 ) ) ;
#17594=VECTOR ( 'NONE', #38043, 1000.000000000000000 ) ;
#17595=CARTESIAN_POINT ( 'NONE',  ( -166.6959734468149463, -1.750000000000009992, -159.1817124430720298 ) ) ;
#17597=FACE_OUTER_BOUND ( 'NONE', #8574, .T. ) ;
#17607=CARTESIAN_POINT ( 'NONE',  ( -44.94597344681493922, 1.025126265847088991, 162.5682875569279133 ) ) ;
#17608=FACE_OUTER_BOUND ( 'NONE', #46973, .T. ) ;
#17610=ORIENTED_EDGE ( 'NONE', *, *, #5933, .F. ) ;
#17611=ORIENTED_EDGE ( 'NONE', *, *, #37198, .F. ) ;
#17615=CYLINDRICAL_SURFACE ( 'NONE', #3799, 1.750000000000001554 ) ;
#17616=( BOUNDED_CURVE ( )  B_SPLINE_CURVE ( 3, ( #12356, #39839, #22766, #26104 ),
 .UNSPECIFIED., .F., .F. ) 
 B_SPLINE_CURVE_WITH_KNOTS ( ( 4, 4 ),
 ( 3.141592653589793116, 4.712388980384689674 ),
 .UNSPECIFIED. ) 
 CURVE ( )  GEOMETRIC_REPRESENTATION_ITEM ( )  RATIONAL_B_SPLINE_CURVE ( ( 1.000000000000000000, 0.8047378541243649375, 0.8047378541243649375, 1.000000000000000000 ) ) 
 REPRESENTATION_ITEM ( '' )  );
#17619=CYLINDRICAL_SURFACE ( 'NONE', #32913, 1.750000000000001554 ) ;
#17620=LINE ( 'NONE', #44293, #9783 ) ;
#17621=ORIENTED_EDGE ( 'NONE', *, *, #39119, .T. ) ;
#17624=CYLINDRICAL_SURFACE ( 'NONE', #38569, 1.750000000000008438 ) ;
#17625=( BOUNDED_CURVE ( )  B_SPLINE_CURVE ( 3, ( #23859, #27956, #31821, #20501 ),
 .UNSPECIFIED., .F., .F. ) 
 B_SPLINE_CURVE_WITH_KNOTS ( ( 4, 4 ),
 ( 4.712388980384689674, 6.283185307179586232 ),
 .UNSPECIFIED. ) 
 CURVE ( )  GEOMETRIC_REPRESENTATION_ITEM ( )  RATIONAL_B_SPLINE_CURVE ( ( 1.000000000000000000, 0.8047378541243649375, 0.8047378541243649375, 1.000000000000000000 ) ) 
 REPRESENTATION_ITEM ( '' )  );
#17627=EDGE_LOOP ( 'NONE', ( #10411, #47365, #13749, #6859, #29432, #12945 ) ) ;
#17629=CARTESIAN_POINT ( 'NONE',  ( -4.945973446814917018, -1.025126265847096985, -37.43171244307200851 ) ) ;
#17633=CARTESIAN_POINT ( 'NONE',  ( -8.445973446814976526, 0.000000000000000000, 79.06828755692795596 ) ) ;
#17635=AXIS2_PLACEMENT_3D ( 'NONE', #42747, #35356, #43010 ) ;
#17638=DIRECTION ( 'NONE',  ( -0.000000000000000000, -0.000000000000000000, -1.000000000000000000 ) ) ;
#17639=VECTOR ( 'NONE', #4715, 1000.000000000000000 ) ;
#17643=VECTOR ( 'NONE', #44440, 1000.000000000000000 ) ;
#17645=VECTOR ( 'NONE', #6391, 1000.000000000000000 ) ;
#17646=VERTEX_POINT ( 'NONE', #50020 ) ;
#17652=EDGE_LOOP ( 'NONE', ( #30314, #37096, #11509, #12810, #33118 ) ) ;
#17653=CARTESIAN_POINT ( 'NONE',  ( -88.44597344681494633, 1.025126265847089657, -120.9317124430720440 ) ) ;
#17657=CARTESIAN_POINT ( 'NONE',  ( 153.3040265531850537, 0.000000000000000000, 165.0000000000000000 ) ) ;
#17658=CARTESIAN_POINT ( 'NONE',  ( 151.5540265531850537, 1.025126265847089435, -117.4317124430720156 ) ) ;
#17662=VERTEX_POINT ( 'NONE', #45938 ) ;
#17664=DIRECTION ( 'NONE',  ( -1.000000000000000000, -0.000000000000000000, -0.000000000000000000 ) ) ;
#17666=EDGE_CURVE ( 'NONE', #19994, #19154, #45480, .T. ) ;
#17669=DIRECTION ( 'NONE',  ( -1.000000000000000000, -0.000000000000000000, -0.000000000000000000 ) ) ;
#17674=CARTESIAN_POINT ( 'NONE',  ( -4.945973446814903696, 2.143131898507912917E-16, -77.43171244307198720 ) ) ;
#17675=VECTOR ( 'NONE', #23190, 1000.000000000000000 ) ;
#17680=EDGE_CURVE ( 'NONE', #50107, #39980, #33813, .T. ) ;
#17685=ORIENTED_EDGE ( 'NONE', *, *, #43099, .F. ) ;
#17692=AXIS2_PLACEMENT_3D ( 'NONE', #21234, #1744, #45569 ) ;
#17694=CARTESIAN_POINT ( 'NONE',  ( 210.0000000000000568, 0.000000000000000000, 82.56828755692799859 ) ) ;
#17695=FACE_OUTER_BOUND ( 'NONE', #2571, .T. ) ;
#17696=CYLINDRICAL_SURFACE ( 'NONE', #32559, 1.750000000000015543 ) ;
#17697=ORIENTED_EDGE ( 'NONE', *, *, #18897, .T. ) ;
#17701=EDGE_CURVE ( 'NONE', #31600, #28309, #41622, .T. ) ;
#17707=EDGE_CURVE ( 'NONE', #18077, #5399, #44265, .T. ) ;
#17710=AXIS2_PLACEMENT_3D ( 'NONE', #37529, #20843, #21593 ) ;
#17714=CARTESIAN_POINT ( 'NONE',  ( 112.2789002873379758, 1.749999999999997113, -80.20683870891909351 ) ) ;
#17721=ORIENTED_EDGE ( 'NONE', *, *, #4825, .F. ) ;
#17727=LINE ( 'NONE', #30286, #45861 ) ;
#17728=DIRECTION ( 'NONE',  ( -1.000000000000000000, -0.000000000000000000, -0.000000000000000000 ) ) ;
#17731=VERTEX_POINT ( 'NONE', #46945 ) ;
#17732=VECTOR ( 'NONE', #23926, 1000.000000000000000 ) ;
#17744=DIRECTION ( 'NONE',  ( 1.000000000000000000, 0.000000000000000000, 0.000000000000000000 ) ) ;
#17747=CARTESIAN_POINT ( 'NONE',  ( 115.0540265531850395, 2.143131898507847836E-16, 82.56828755692797017 ) ) ;
#17753=FACE_OUTER_BOUND ( 'NONE', #12262, .T. ) ;
#17754=ORIENTED_EDGE ( 'NONE', *, *, #20381, .T. ) ;
#17757=CARTESIAN_POINT ( 'NONE',  ( 33.30402655318503946, -1.750000000000009992, 0.8182875569279768335 ) ) ;
#17760=ORIENTED_EDGE ( 'NONE', *, *, #39498, .F. ) ;
#17764=CARTESIAN_POINT ( 'NONE',  ( -128.4459734468149463, -1.025126265847081442, -0.9317124430720195027 ) ) ;
#17765=CARTESIAN_POINT ( 'NONE',  ( -44.94597344681493922, 1.025126265847089657, -80.93171244307201562 ) ) ;
#17771=CARTESIAN_POINT ( 'NONE',  ( 113.3040265531850537, 1.749999999999997335, 80.81828755692798438 ) ) ;
#17778=EDGE_CURVE ( 'NONE', #12842, #40787, #3974, .T. ) ;
#17787=CARTESIAN_POINT ( 'NONE',  ( 71.55402655318505367, -1.025126265847089879, -77.43171244307200141 ) ) ;
#17790=( BOUNDED_CURVE ( )  B_SPLINE_CURVE ( 3, ( #27138, #31500, #6872, #50682 ),
 .UNSPECIFIED., .F., .F. ) 
 B_SPLINE_CURVE_WITH_KNOTS ( ( 4, 4 ),
 ( 3.141592653589793116, 4.712388980384689674 ),
 .UNSPECIFIED. ) 
 CURVE ( )  GEOMETRIC_REPRESENTATION_ITEM ( )  RATIONAL_B_SPLINE_CURVE ( ( 1.000000000000000000, 0.8047378541243649375, 0.8047378541243649375, 1.000000000000000000 ) ) 
 REPRESENTATION_ITEM ( '' )  );
#17794=ORIENTED_EDGE ( 'NONE', *, *, #40659, .F. ) ;
#17803=CYLINDRICAL_SURFACE ( 'NONE', #26409, 1.750000000000015543 ) ;
#17805=LINE ( 'NONE', #45474, #49625 ) ;
#17807=ORIENTED_EDGE ( 'NONE', *, *, #16002, .T. ) ;
#17823=CARTESIAN_POINT ( 'NONE',  ( -86.69597344681494633, -1.750000000000010658, -79.18171244307201562 ) ) ;
#17828=CARTESIAN_POINT ( 'NONE',  ( -206.6959734468149463, -1.750000000000010658, -79.18171244307201562 ) ) ;
#17829=CARTESIAN_POINT ( 'NONE',  ( 71.55402655318505367, 0.000000000000000000, -40.93171244307205825 ) ) ;
#17834=EDGE_CURVE ( 'NONE', #16395, #16392, #9222, .T. ) ;
#17844=LINE ( 'NONE', #33270, #2459 ) ;
#17845=CARTESIAN_POINT ( 'NONE',  ( 153.3040265531850537, -1.750000000000010214, 40.81828755692798438 ) ) ;
#17846=CARTESIAN_POINT ( 'NONE',  ( -124.9459734468149321, -1.025126265847081664, 42.56828755692797017 ) ) ;
#17851=CARTESIAN_POINT ( 'NONE',  ( -46.69597344681494633, 1.750000000000009992, 0.8182875569279768335 ) ) ;
#17855=( BOUNDED_CURVE ( )  B_SPLINE_CURVE ( 3, ( #37889, #30686, #45780, #6566 ),
 .UNSPECIFIED., .F., .F. ) 
 B_SPLINE_CURVE_WITH_KNOTS ( ( 4, 4 ),
 ( 3.141592653589793116, 4.712388980384689674 ),
 .UNSPECIFIED. ) 
 CURVE ( )  GEOMETRIC_REPRESENTATION_ITEM ( )  RATIONAL_B_SPLINE_CURVE ( ( 1.000000000000000000, 0.8047378541243649375, 0.8047378541243649375, 1.000000000000000000 ) ) 
 REPRESENTATION_ITEM ( '' )  );
#17856=ORIENTED_EDGE ( 'NONE', *, *, #32773, .T. ) ;
#17859=ORIENTED_EDGE ( 'NONE', *, *, #33389, .F. ) ;
#17861=DIRECTION ( 'NONE',  ( -1.000000000000000000, -0.000000000000000000, -0.000000000000000000 ) ) ;
#17867=DIRECTION ( 'NONE',  ( -0.000000000000000000, -0.000000000000000000, -1.000000000000000000 ) ) ;
#17869=CARTESIAN_POINT ( 'NONE',  ( -204.9459734468148895, 1.025126265847089213, -160.9317124430720014 ) ) ;
#17871=DIRECTION ( 'NONE',  ( 0.000000000000000000, 0.000000000000000000, 1.000000000000000000 ) ) ;
#17872=CARTESIAN_POINT ( 'NONE',  ( -208.4459734468148611, -1.025126265847089435, 39.06828755692797728 ) ) ;
#17873=FACE_OUTER_BOUND ( 'NONE', #1168, .T. ) ;
#17878=CARTESIAN_POINT ( 'NONE',  ( 115.0540265531850395, 2.143131898507847836E-16, 2.568287556927950632 ) ) ;
#17881=CARTESIAN_POINT ( 'NONE',  ( 113.3040265531850537, 1.749999999999996891, -159.1817124430720298 ) ) ;
#17882=CARTESIAN_POINT ( 'NONE',  ( 191.5540265531850537, -1.025126265847089213, 159.0682875569279418 ) ) ;
#17889=ORIENTED_EDGE ( 'NONE', *, *, #35477, .F. ) ;
#17891=FACE_OUTER_BOUND ( 'NONE', #36780, .T. ) ;
#17892=ORIENTED_EDGE ( 'NONE', *, *, #440, .F. ) ;
#17894=CARTESIAN_POINT ( 'NONE',  ( -164.9459734468149463, 1.025126265847089657, 79.06828755692797017 ) ) ;
#17895=DIRECTION ( 'NONE',  ( -1.000000000000000000, -0.000000000000000000, -0.000000000000000000 ) ) ;
#17896=FACE_OUTER_BOUND ( 'NONE', #37498, .T. ) ;
#17897=ORIENTED_EDGE ( 'NONE', *, *, #30250, .T. ) ;
#17898=ORIENTED_EDGE ( 'NONE', *, *, #431, .T. ) ;
#17899=ORIENTED_EDGE ( 'NONE', *, *, #50388, .F. ) ;
#17900=CARTESIAN_POINT ( 'NONE',  ( 210.0000000000000568, 0.000000000000000000, 80.81828755692798438 ) ) ;
#17901=( BOUNDED_CURVE ( )  B_SPLINE_CURVE ( 3, ( #32366, #1324, #33137, #5909 ),
 .UNSPECIFIED., .F., .F. ) 
 B_SPLINE_CURVE_WITH_KNOTS ( ( 4, 4 ),
 ( 4.712388980384689674, 6.283185307179586232 ),
 .UNSPECIFIED. ) 
 CURVE ( )  GEOMETRIC_REPRESENTATION_ITEM ( )  RATIONAL_B_SPLINE_CURVE ( ( 1.000000000000000000, 0.8047378541243649375, 0.8047378541243649375, 1.000000000000000000 ) ) 
 REPRESENTATION_ITEM ( '' )  );
#17903=ORIENTED_EDGE ( 'NONE', *, *, #23288, .F. ) ;
#17908=CARTESIAN_POINT ( 'NONE',  ( -165.6708471809677974, 1.750000000000010214, 81.84341382277507648 ) ) ;
#17909=( BOUNDED_CURVE ( )  B_SPLINE_CURVE ( 3, ( #7448, #30531, #18966, #6665 ),
 .UNSPECIFIED., .F., .F. ) 
 B_SPLINE_CURVE_WITH_KNOTS ( ( 4, 4 ),
 ( 3.141592653589793116, 4.712388980384689674 ),
 .UNSPECIFIED. ) 
 CURVE ( )  GEOMETRIC_REPRESENTATION_ITEM ( )  RATIONAL_B_SPLINE_CURVE ( ( 1.000000000000000000, 0.8047378541243649375, 0.8047378541243649375, 1.000000000000000000 ) ) 
 REPRESENTATION_ITEM ( '' )  );
#17915=CARTESIAN_POINT ( 'NONE',  ( 210.0000000000000568, 2.143131898507880377E-16, -160.9317124430720298 ) ) ;
#17917=CARTESIAN_POINT ( 'NONE',  ( 111.5540265531850537, 1.025126265847081442, -160.9317124430720014 ) ) ;
#17919=EDGE_LOOP ( 'NONE', ( #16456, #46429, #31431, #1419, #5362, #12831 ) ) ;
#17921=ORIENTED_EDGE ( 'NONE', *, *, #33068, .F. ) ;
#17926=DIRECTION ( 'NONE',  ( -1.000000000000000000, -0.000000000000000000, -0.000000000000000000 ) ) ;
#17927=DIRECTION ( 'NONE',  ( -1.000000000000000000, 0.000000000000000000, 0.000000000000000000 ) ) ;
#17929=CARTESIAN_POINT ( 'NONE',  ( -84.94597344681494633, 2.143131898507880377E-16, 165.0000000000000000 ) ) ;
#17932=CARTESIAN_POINT ( 'NONE',  ( -87.72109971266203843, 1.750000000000010436, -80.20683870891910772 ) ) ;
#17934=ORIENTED_EDGE ( 'NONE', *, *, #36206, .T. ) ;
#17943=DIRECTION ( 'NONE',  ( -0.000000000000000000, -0.000000000000000000, -1.000000000000000000 ) ) ;
#17949=ADVANCED_FACE ( 'NONE', ( #9005 ), #24659, .T. ) ;
#17950=CARTESIAN_POINT ( 'NONE',  ( 71.55402655318505367, 0.000000000000000000, 2.568287556928006143 ) ) ;
#17954=CARTESIAN_POINT ( 'NONE',  ( 210.0000000000000568, 2.143131898507880377E-16, 159.0682875569279702 ) ) ;
#17961=EDGE_CURVE ( 'NONE', #7778, #9118, #39987, .T. ) ;
#17963=ORIENTED_EDGE ( 'NONE', *, *, #37769, .T. ) ;
#17969=DIRECTION ( 'NONE',  ( -1.000000000000000000, -0.000000000000000000, -0.000000000000000000 ) ) ;
#17971=VERTEX_POINT ( 'NONE', #9249 ) ;
#17976=CIRCLE ( 'NONE', #32758, 1.749999999999987566 ) ;
#17984=CARTESIAN_POINT ( 'NONE',  ( -166.6959734468149463, -1.750000000000010214, -39.18171244307202983 ) ) ;
#17988=ORIENTED_EDGE ( 'NONE', *, *, #6401, .T. ) ;
#17991=FACE_OUTER_BOUND ( 'NONE', #5312, .T. ) ;
#17993=AXIS2_PLACEMENT_3D ( 'NONE', #13686, #6746, #29850 ) ;
#17994=LINE ( 'NONE', #37532, #1803 ) ;
#17997=CARTESIAN_POINT ( 'NONE',  ( -86.69597344681494633, 1.750000000000010658, 80.81828755692798438 ) ) ;
#18011=CARTESIAN_POINT ( 'NONE',  ( -44.94597344681493922, 2.143131898507880377E-16, -120.9317124430720725 ) ) ;
#18013=CARTESIAN_POINT ( 'NONE',  ( 194.3291528190321742, -1.750000000000009548, -40.20683870891912193 ) ) ;
#18018=EDGE_CURVE ( 'NONE', #7014, #43847, #22053, .T. ) ;
#18021=DIRECTION ( 'NONE',  ( -0.000000000000000000, -0.000000000000000000, -1.000000000000000000 ) ) ;
#18024=VERTEX_POINT ( 'NONE', #26160 ) ;
#18025=VECTOR ( 'NONE', #50714, 1000.000000000000000 ) ;
#18034=EDGE_LOOP ( 'NONE', ( #39584, #4149, #43426, #1017, #48351 ) ) ;
#18035=DIRECTION ( 'NONE',  ( -1.000000000000000000, 0.000000000000000000, 0.000000000000000000 ) ) ;
#18036=EDGE_CURVE ( 'NONE', #12513, #9595, #8812, .T. ) ;
#18048=CARTESIAN_POINT ( 'NONE',  ( -206.6959734468149463, 1.750000000000010658, 120.8182875569279702 ) ) ;
#18050=ORIENTED_EDGE ( 'NONE', *, *, #29937, .F. ) ;
#18054=EDGE_CURVE ( 'NONE', #16946, #18861, #27431, .T. ) ;
#18057=( BOUNDED_CURVE ( )  B_SPLINE_CURVE ( 3, ( #30713, #50141, #42244, #34299 ),
 .UNSPECIFIED., .F., .F. ) 
 B_SPLINE_CURVE_WITH_KNOTS ( ( 4, 4 ),
 ( 3.141592653589793116, 4.712388980384689674 ),
 .UNSPECIFIED. ) 
 CURVE ( )  GEOMETRIC_REPRESENTATION_ITEM ( )  RATIONAL_B_SPLINE_CURVE ( ( 1.000000000000000000, 0.8047378541243649375, 0.8047378541243649375, 1.000000000000000000 ) ) 
 REPRESENTATION_ITEM ( '' )  );
#18058=CARTESIAN_POINT ( 'NONE',  ( 210.0000000000000568, 0.000000000000000000, 0.8182875569279768335 ) ) ;
#18060=VERTEX_POINT ( 'NONE', #249 ) ;
#18075=EDGE_CURVE ( 'NONE', #47399, #9715, #12392, .T. ) ;
#18076=LINE ( 'NONE', #6787, #30722 ) ;
#18077=VERTEX_POINT ( 'NONE', #8193 ) ;
#18079=CARTESIAN_POINT ( 'NONE',  ( 73.30402655318508209, -1.750000000000009992, 160.8182875569279702 ) ) ;
#18080=( BOUNDED_CURVE ( )  B_SPLINE_CURVE ( 3, ( #16551, #16298, #47552, #16048 ),
 .UNSPECIFIED., .F., .F. ) 
 B_SPLINE_CURVE_WITH_KNOTS ( ( 4, 4 ),
 ( 4.712388980384689674, 6.283185307179586232 ),
 .UNSPECIFIED. ) 
 CURVE ( )  GEOMETRIC_REPRESENTATION_ITEM ( )  RATIONAL_B_SPLINE_CURVE ( ( 1.000000000000000000, 0.8047378541243649375, 0.8047378541243649375, 1.000000000000000000 ) ) 
 REPRESENTATION_ITEM ( '' )  );
#18082=CARTESIAN_POINT ( 'NONE',  ( 73.30402655318508209, 1.750000000000010214, -39.18171244307202983 ) ) ;
#18083=DIRECTION ( 'NONE',  ( -1.000000000000000000, 0.000000000000000000, 0.000000000000000000 ) ) ;
#18085=CARTESIAN_POINT ( 'NONE',  ( 111.5540265531850679, 0.000000000000000000, 119.0682875569279844 ) ) ;
#18090=VERTEX_POINT ( 'NONE', #34896 ) ;
#18093=CARTESIAN_POINT ( 'NONE',  ( -126.6959734468149321, 1.749999999999997335, 80.81828755692798438 ) ) ;
#18100=EDGE_LOOP ( 'NONE', ( #7576, #15484, #8157, #25003, #7472, #12154 ) ) ;
#18102=CARTESIAN_POINT ( 'NONE',  ( -47.72109971266203132, 1.750000000000009548, -0.2068387089191121020 ) ) ;
#18112=CARTESIAN_POINT ( 'NONE',  ( 210.0000000000000568, 2.143131898507880377E-16, -160.9317124430720298 ) ) ;
#18113=EDGE_CURVE ( 'NONE', #39055, #36017, #18951, .T. ) ;
#18114=CARTESIAN_POINT ( 'NONE',  ( -207.7210997126620384, 1.750000000000010436, -120.2068387089191219 ) ) ;
#18118=CARTESIAN_POINT ( 'NONE',  ( 75.05402655318509630, 2.143131898507880377E-16, 119.0682875569279560 ) ) ;
#18119=DIRECTION ( 'NONE',  ( -1.000000000000000000, -0.000000000000000000, -0.000000000000000000 ) ) ;
#18122=ORIENTED_EDGE ( 'NONE', *, *, #15701, .F. ) ;
#18129=DIRECTION ( 'NONE',  ( -1.000000000000000000, -0.000000000000000000, -0.000000000000000000 ) ) ;
#18131=LINE ( 'NONE', #41995, #19678 ) ;
#18136=AXIS2_PLACEMENT_3D ( 'NONE', #34211, #6485, #2627 ) ;
#18140=CARTESIAN_POINT ( 'NONE',  ( -44.94597344681497475, 0.000000000000000000, 162.5682875569279702 ) ) ;
#18142=CARTESIAN_POINT ( 'NONE',  ( -206.6959734468149463, 0.000000000000000000, 165.0000000000000000 ) ) ;
#18145=EDGE_CURVE ( 'NONE', #6771, #16019, #21235, .T. ) ;
#18147=DIRECTION ( 'NONE',  ( -1.000000000000000000, 0.000000000000000000, 0.000000000000000000 ) ) ;
#18153=CYLINDRICAL_SURFACE ( 'NONE', #33048, 1.750000000000015543 ) ;
#18156=ORIENTED_EDGE ( 'NONE', *, *, #33987, .F. ) ;
#18157=CYLINDRICAL_SURFACE ( 'NONE', #28182, 1.750000000000008438 ) ;
#18159=ORIENTED_EDGE ( 'NONE', *, *, #8185, .T. ) ;
#18160=EDGE_CURVE ( 'NONE', #37586, #9366, #15119, .T. ) ;
#18161=ORIENTED_EDGE ( 'NONE', *, *, #12112, .F. ) ;
#18166=CARTESIAN_POINT ( 'NONE',  ( 74.32915281903215998, -1.750000000000009548, -0.2068387089191121020 ) ) ;
#18168=EDGE_LOOP ( 'NONE', ( #27393, #16300 ) ) ;
#18172=EDGE_CURVE ( 'NONE', #1473, #22181, #23841, .T. ) ;
#18173=DIRECTION ( 'NONE',  ( 1.000000000000000000, 0.000000000000000000, 0.000000000000000000 ) ) ;
#18175=CARTESIAN_POINT ( 'NONE',  ( 73.30402655318508209, 1.750000000000010214, -39.18171244307202983 ) ) ;
#18178=ORIENTED_EDGE ( 'NONE', *, *, #21838, .F. ) ;
#18179=ORIENTED_EDGE ( 'NONE', *, *, #36620, .T. ) ;
#18180=LINE ( 'NONE', #45851, #34424 ) ;
#18183=EDGE_LOOP ( 'NONE', ( #49518, #16196, #5510, #13317, #31465, #14381 ) ) ;
#18184=FACE_OUTER_BOUND ( 'NONE', #27669, .T. ) ;
#18190=VECTOR ( 'NONE', #13332, 1000.000000000000000 ) ;
#18201=DIRECTION ( 'NONE',  ( 0.000000000000000000, 0.000000000000000000, 1.000000000000000000 ) ) ;
#18203=CARTESIAN_POINT ( 'NONE',  ( -4.945973446814903696, 2.143131898507912917E-16, 165.0000000000000000 ) ) ;
#18205=( BOUNDED_CURVE ( )  B_SPLINE_CURVE ( 3, ( #447, #47088, #35612, #7898 ),
 .UNSPECIFIED., .F., .F. ) 
 B_SPLINE_CURVE_WITH_KNOTS ( ( 4, 4 ),
 ( 3.141592653589793116, 4.712388980384689674 ),
 .UNSPECIFIED. ) 
 CURVE ( )  GEOMETRIC_REPRESENTATION_ITEM ( )  RATIONAL_B_SPLINE_CURVE ( ( 1.000000000000000000, 0.8047378541243649375, 0.8047378541243649375, 1.000000000000000000 ) ) 
 REPRESENTATION_ITEM ( '' )  );
#18207=FACE_OUTER_BOUND ( 'NONE', #17059, .T. ) ;
#18210=ORIENTED_EDGE ( 'NONE', *, *, #34701, .T. ) ;
#18211=DIRECTION ( 'NONE',  ( 0.000000000000000000, 0.000000000000000000, 1.000000000000000000 ) ) ;
#18213=( BOUNDED_CURVE ( )  B_SPLINE_CURVE ( 3, ( #19745, #31569, #43336, #38509 ),
 .UNSPECIFIED., .F., .F. ) 
 B_SPLINE_CURVE_WITH_KNOTS ( ( 4, 4 ),
 ( 4.712388980384689674, 6.283185307179586232 ),
 .UNSPECIFIED. ) 
 CURVE ( )  GEOMETRIC_REPRESENTATION_ITEM ( )  RATIONAL_B_SPLINE_CURVE ( ( 1.000000000000000000, 0.8047378541243649375, 0.8047378541243649375, 1.000000000000000000 ) ) 
 REPRESENTATION_ITEM ( '' )  );
#18215=CARTESIAN_POINT ( 'NONE',  ( 35.05402655318504657, 1.025126265847089657, 79.06828755692797017 ) ) ;
#18226=ORIENTED_EDGE ( 'NONE', *, *, #5823, .F. ) ;
#18235=CARTESIAN_POINT ( 'NONE',  ( -46.69597344681494633, -1.750000000000009992, -159.1817124430720298 ) ) ;
#18237=CARTESIAN_POINT ( 'NONE',  ( -168.4459734468149747, 1.025126265847089657, 79.06828755692797017 ) ) ;
#18239=ORIENTED_EDGE ( 'NONE', *, *, #31292, .T. ) ;
#18241=CARTESIAN_POINT ( 'NONE',  ( 33.30402655318503946, 1.750000000000010658, -119.1817124430720440 ) ) ;
#18243=DIRECTION ( 'NONE',  ( -1.000000000000000000, -0.000000000000000000, -0.000000000000000000 ) ) ;
#18246=CARTESIAN_POINT ( 'NONE',  ( -86.69597344681494633, -1.750000000000010214, -39.18171244307202983 ) ) ;
#18256=CARTESIAN_POINT ( 'NONE',  ( -6.695973446814940111, -1.750000000000024203, -119.1817124430720440 ) ) ;
#18261=CARTESIAN_POINT ( 'NONE',  ( 34.32915281903212446, -1.750000000000009548, -40.20683870891912193 ) ) ;
#18264=VECTOR ( 'NONE', #43523, 1000.000000000000000 ) ;
#18267=ORIENTED_EDGE ( 'NONE', *, *, #27406, .F. ) ;
#18269=CARTESIAN_POINT ( 'NONE',  ( 115.0540265531850395, 2.143131898507847836E-16, 82.56828755692797017 ) ) ;
#18270=ORIENTED_EDGE ( 'NONE', *, *, #32849, .F. ) ;
#18274=ORIENTED_EDGE ( 'NONE', *, *, #440, .T. ) ;
#18275=CARTESIAN_POINT ( 'NONE',  ( 191.5540265531851105, 0.000000000000000000, 165.0000000000000000 ) ) ;
#18278=CARTESIAN_POINT ( 'NONE',  ( -88.44597344681494633, -1.025126265847089879, 122.5682875569280128 ) ) ;
#18279=EDGE_LOOP ( 'NONE', ( #27661, #1893, #11564, #11, #45107, #31263 ) ) ;
#18283=CARTESIAN_POINT ( 'NONE',  ( -8.445973446814976526, 0.000000000000000000, -37.43171244307200141 ) ) ;
#18287=ORIENTED_EDGE ( 'NONE', *, *, #23972, .F. ) ;
#18290=AXIS2_PLACEMENT_3D ( 'NONE', #33404, #45147, #28781 ) ;
#18302=VERTEX_POINT ( 'NONE', #29141 ) ;
#18306=ORIENTED_EDGE ( 'NONE', *, *, #23846, .T. ) ;
#18308=VERTEX_POINT ( 'NONE', #5783 ) ;
#18309=CARTESIAN_POINT ( 'NONE',  ( -6.695973446814940111, 0.000000000000000000, 165.0000000000000000 ) ) ;
#18310=LINE ( 'NONE', #41932, #24000 ) ;
#18311=ORIENTED_EDGE ( 'NONE', *, *, #50627, .F. ) ;
#18312=CARTESIAN_POINT ( 'NONE',  ( -46.69597344681494633, -1.750000000000010658, -79.18171244307201562 ) ) ;
#18313=CARTESIAN_POINT ( 'NONE',  ( 114.3291528190321173, -1.749999999999997113, 119.7931612910809065 ) ) ;
#18316=VECTOR ( 'NONE', #37593, 1000.000000000000000 ) ;
#18323=EDGE_CURVE ( 'NONE', #8111, #48485, #14491, .T. ) ;
#18325=EDGE_CURVE ( 'NONE', #12576, #36969, #45404, .T. ) ;
#18326=DIRECTION ( 'NONE',  ( -1.000000000000000000, -0.000000000000000000, -0.000000000000000000 ) ) ;
#18331=EDGE_CURVE ( 'NONE', #38661, #7012, #20865, .T. ) ;
#18339=DIRECTION ( 'NONE',  ( -1.000000000000000000, -0.000000000000000000, -0.000000000000000000 ) ) ;
#18342=ORIENTED_EDGE ( 'NONE', *, *, #15787, .F. ) ;
#18346=( BOUNDED_CURVE ( )  B_SPLINE_CURVE ( 3, ( #16292, #31709, #47546, #48044 ),
 .UNSPECIFIED., .F., .F. ) 
 B_SPLINE_CURVE_WITH_KNOTS ( ( 4, 4 ),
 ( 0.000000000000000000, 1.570796326794896558 ),
 .UNSPECIFIED. ) 
 CURVE ( )  GEOMETRIC_REPRESENTATION_ITEM ( )  RATIONAL_B_SPLINE_CURVE ( ( 1.000000000000000000, 0.8047378541243649375, 0.8047378541243649375, 1.000000000000000000 ) ) 
 REPRESENTATION_ITEM ( '' )  );
#18348=EDGE_CURVE ( 'NONE', #40036, #17662, #6540, .T. ) ;
#18350=EDGE_CURVE ( 'NONE', #35947, #13085, #50715, .T. ) ;
#18351=DIRECTION ( 'NONE',  ( -0.000000000000000000, -0.000000000000000000, -1.000000000000000000 ) ) ;
#18352=CARTESIAN_POINT ( 'NONE',  ( 192.2789002873380184, -1.750000000000009548, 1.843413822775065825 ) ) ;
#18356=( BOUNDED_CURVE ( )  B_SPLINE_CURVE ( 3, ( #2476, #48621, #45792, #49380 ),
 .UNSPECIFIED., .F., .F. ) 
 B_SPLINE_CURVE_WITH_KNOTS ( ( 4, 4 ),
 ( 3.141592653589793116, 4.712388980384689674 ),
 .UNSPECIFIED. ) 
 CURVE ( )  GEOMETRIC_REPRESENTATION_ITEM ( )  RATIONAL_B_SPLINE_CURVE ( ( 1.000000000000000000, 0.8047378541243649375, 0.8047378541243649375, 1.000000000000000000 ) ) 
 REPRESENTATION_ITEM ( '' )  );
#18359=DIRECTION ( 'NONE',  ( 0.000000000000000000, 0.000000000000000000, 1.000000000000000000 ) ) ;
#18361=EDGE_LOOP ( 'NONE', ( #9632, #6107 ) ) ;
#18362=CARTESIAN_POINT ( 'NONE',  ( -208.4459734468148611, -1.025126265847089879, 82.56828755692798438 ) ) ;
#18366=VERTEX_POINT ( 'NONE', #33755 ) ;
#18371=CARTESIAN_POINT ( 'NONE',  ( -6.695973446814940111, -1.750000000000023759, -39.18171244307202983 ) ) ;
#18372=( BOUNDED_CURVE ( )  B_SPLINE_CURVE ( 3, ( #5067, #1741, #6087, #16628 ),
 .UNSPECIFIED., .F., .F. ) 
 B_SPLINE_CURVE_WITH_KNOTS ( ( 4, 4 ),
 ( 4.712388980384689674, 6.283185307179586232 ),
 .UNSPECIFIED. ) 
 CURVE ( )  GEOMETRIC_REPRESENTATION_ITEM ( )  RATIONAL_B_SPLINE_CURVE ( ( 1.000000000000000000, 0.8047378541243649375, 0.8047378541243649375, 1.000000000000000000 ) ) 
 REPRESENTATION_ITEM ( '' )  );
#18376=LINE ( 'NONE', #10436, #23332 ) ;
#18378=CARTESIAN_POINT ( 'NONE',  ( -124.9459734468149463, 2.143131898507842906E-16, -165.0000000000000000 ) ) ;
#18382=EDGE_LOOP ( 'NONE', ( #28224, #20442, #16921, #19203, #30320, #26377 ) ) ;
#18384=CARTESIAN_POINT ( 'NONE',  ( -84.94597344681494633, 2.143131898507880377E-16, 42.56828755692798438 ) ) ;
#18386=CARTESIAN_POINT ( 'NONE',  ( -164.9459734468149463, 2.143131898507880377E-16, -160.9317124430720014 ) ) ;
#18391=FACE_OUTER_BOUND ( 'NONE', #37850, .T. ) ;
#18392=AXIS2_PLACEMENT_3D ( 'NONE', #34778, #50352, #30146 ) ;
#18395=ADVANCED_FACE ( 'NONE', ( #3437 ), #19087, .T. ) ;
#18408=DIRECTION ( 'NONE',  ( 0.000000000000000000, 0.000000000000000000, 1.000000000000000000 ) ) ;
#18409=ADVANCED_FACE ( 'NONE', ( #12169 ), #39386, .T. ) ;
#18410=ORIENTED_EDGE ( 'NONE', *, *, #4360, .T. ) ;
#18411=LINE ( 'NONE', #46588, #33136 ) ;
#18414=AXIS2_PLACEMENT_3D ( 'NONE', #49576, #48574, #48823 ) ;
#18415=CARTESIAN_POINT ( 'NONE',  ( -4.945973446814916130, -1.025126265847097429, -120.9317124430720440 ) ) ;
#18420=LINE ( 'NONE', #41772, #4322 ) ;
#18421=DIRECTION ( 'NONE',  ( -0.000000000000000000, -0.000000000000000000, -1.000000000000000000 ) ) ;
#18431=EDGE_LOOP ( 'NONE', ( #17721, #48812 ) ) ;
#18436=EDGE_CURVE ( 'NONE', #8682, #42453, #48766, .T. ) ;
#18437=CYLINDRICAL_SURFACE ( 'NONE', #50353, 1.750000000000001554 ) ;
#18441=CARTESIAN_POINT ( 'NONE',  ( -128.4459734468149463, -1.025126265847082108, 42.56828755692797017 ) ) ;
#18449=ORIENTED_EDGE ( 'NONE', *, *, #20507, .T. ) ;
#18453=ADVANCED_FACE ( 'NONE', ( #31936 ), #35039, .T. ) ;
#18454=( BOUNDED_CURVE ( )  B_SPLINE_CURVE ( 3, ( #12119, #20565, #23910, #47221 ),
 .UNSPECIFIED., .F., .F. ) 
 B_SPLINE_CURVE_WITH_KNOTS ( ( 4, 4 ),
 ( 0.000000000000000000, 1.570796326794896558 ),
 .UNSPECIFIED. ) 
 CURVE ( )  GEOMETRIC_REPRESENTATION_ITEM ( )  RATIONAL_B_SPLINE_CURVE ( ( 1.000000000000000000, 0.8047378541243649375, 0.8047378541243649375, 1.000000000000000000 ) ) 
 REPRESENTATION_ITEM ( '' )  );
#18456=CARTESIAN_POINT ( 'NONE',  ( -44.94597344681493922, -1.025126265847089435, 39.06828755692797728 ) ) ;
#18459=CARTESIAN_POINT ( 'NONE',  ( 210.0000000000000568, 0.000000000000000000, 40.81828755692798438 ) ) ;
#18464=ADVANCED_FACE ( 'NONE', ( #4219 ), #15755, .T. ) ;
#18467=CARTESIAN_POINT ( 'NONE',  ( -46.69597344681494633, -1.750000000000010658, 120.8182875569279702 ) ) ;
#18469=CARTESIAN_POINT ( 'NONE',  ( -86.69597344681494633, 1.750000000000010214, 40.81828755692798438 ) ) ;
#18472=EDGE_CURVE ( 'NONE', #18302, #25384, #7155, .T. ) ;
#18476=FACE_OUTER_BOUND ( 'NONE', #39803, .T. ) ;
#18478=AXIS2_PLACEMENT_3D ( 'NONE', #42869, #31093, #6721 ) ;
#18479=CARTESIAN_POINT ( 'NONE',  ( -84.94597344681493212, -1.025126265847089213, -0.9317124430720324924 ) ) ;
#18480=ORIENTED_EDGE ( 'NONE', *, *, #6034, .F. ) ;
#18485=DIRECTION ( 'NONE',  ( 0.000000000000000000, 0.000000000000000000, 1.000000000000000000 ) ) ;
#18492=EDGE_LOOP ( 'NONE', ( #16560, #41039, #10040, #37727, #45294, #45449 ) ) ;
#18494=ORIENTED_EDGE ( 'NONE', *, *, #27024, .T. ) ;
#18496=ADVANCED_FACE ( 'NONE', ( #379 ), #36037, .T. ) ;
#18498=ORIENTED_EDGE ( 'NONE', *, *, #44681, .F. ) ;
#18499=ADVANCED_FACE ( 'NONE', ( #19600 ), #16024, .T. ) ;
#18505=VERTEX_POINT ( 'NONE', #43957 ) ;
#18509=CARTESIAN_POINT ( 'NONE',  ( -128.4459734468149463, -1.025126265847081442, -160.9317124430720014 ) ) ;
#18513=( BOUNDED_CURVE ( )  B_SPLINE_CURVE ( 3, ( #30116, #45219, #40665, #5499 ),
 .UNSPECIFIED., .F., .F. ) 
 B_SPLINE_CURVE_WITH_KNOTS ( ( 4, 4 ),
 ( 0.000000000000000000, 1.570796326794896558 ),
 .UNSPECIFIED. ) 
 CURVE ( )  GEOMETRIC_REPRESENTATION_ITEM ( )  RATIONAL_B_SPLINE_CURVE ( ( 1.000000000000000000, 0.8047378541243649375, 0.8047378541243649375, 1.000000000000000000 ) ) 
 REPRESENTATION_ITEM ( '' )  );
#18520=ORIENTED_EDGE ( 'NONE', *, *, #1141, .F. ) ;
#18521=( BOUNDED_CURVE ( )  B_SPLINE_CURVE ( 3, ( #271, #46908, #11812, #27460 ),
 .UNSPECIFIED., .F., .F. ) 
 B_SPLINE_CURVE_WITH_KNOTS ( ( 4, 4 ),
 ( 0.000000000000000000, 1.570796326794896558 ),
 .UNSPECIFIED. ) 
 CURVE ( )  GEOMETRIC_REPRESENTATION_ITEM ( )  RATIONAL_B_SPLINE_CURVE ( ( 1.000000000000000000, 0.8047378541243649375, 0.8047378541243649375, 1.000000000000000000 ) ) 
 REPRESENTATION_ITEM ( '' )  );
#18522=FACE_OUTER_BOUND ( 'NONE', #1094, .T. ) ;
#18525=ORIENTED_EDGE ( 'NONE', *, *, #19048, .F. ) ;
#18526=CARTESIAN_POINT ( 'NONE',  ( 114.3291528190321173, 1.749999999999996891, 81.84341382277506227 ) ) ;
#18536=FACE_OUTER_BOUND ( 'NONE', #28427, .T. ) ;
#18539=CARTESIAN_POINT ( 'NONE',  ( -48.44597344681495343, 0.000000000000000000, -37.43171244307200141 ) ) ;
#18547=ORIENTED_EDGE ( 'NONE', *, *, #22703, .T. ) ;
#18549=FACE_OUTER_BOUND ( 'NONE', #45642, .T. ) ;
#18551=AXIS2_PLACEMENT_3D ( 'NONE', #40177, #5012, #1681 ) ;
#18565=ORIENTED_EDGE ( 'NONE', *, *, #18075, .T. ) ;
#18570=LINE ( 'NONE', #49080, #23586 ) ;
#18577=FACE_OUTER_BOUND ( 'NONE', #25989, .T. ) ;
#18586=ADVANCED_FACE ( 'NONE', ( #21623 ), #17021, .T. ) ;
#18594=ORIENTED_EDGE ( 'NONE', *, *, #25665, .T. ) ;
#18600=VERTEX_POINT ( 'NONE', #49024 ) ;
#18601=FACE_OUTER_BOUND ( 'NONE', #31488, .T. ) ;
#18602=CARTESIAN_POINT ( 'NONE',  ( -204.9459734468149747, 0.000000000000000000, 162.5682875569279702 ) ) ;
#18603=CARTESIAN_POINT ( 'NONE',  ( -86.69597344681496054, 0.000000000000000000, 165.0000000000000000 ) ) ;
#18612=ADVANCED_FACE ( 'NONE', ( #40634 ), #9326, .T. ) ;
#18614=EDGE_CURVE ( 'NONE', #17157, #32209, #11898, .T. ) ;
#18615=CARTESIAN_POINT ( 'NONE',  ( -208.4459734468149463, 0.000000000000000000, 82.56828755692798438 ) ) ;
#18620=DIRECTION ( 'NONE',  ( -0.000000000000000000, -0.000000000000000000, -1.000000000000000000 ) ) ;
#18622=CARTESIAN_POINT ( 'NONE',  ( -126.6959734468149321, -1.749999999999997335, -119.1817124430720440 ) ) ;
#18624=ORIENTED_EDGE ( 'NONE', *, *, #27807, .T. ) ;
#18626=CYLINDRICAL_SURFACE ( 'NONE', #6961, 1.750000000000015543 ) ;
#18637=LINE ( 'NONE', #42743, #49227 ) ;
#18638=EDGE_CURVE ( 'NONE', #16975, #16858, #37056, .T. ) ;
#18639=AXIS2_PLACEMENT_3D ( 'NONE', #5833, #17380, #30186 ) ;
#18645=CARTESIAN_POINT ( 'NONE',  ( -124.9459734468149463, 2.143131898507847836E-16, 165.0000000000000000 ) ) ;
#18647=( BOUNDED_CURVE ( )  B_SPLINE_CURVE ( 3, ( #37445, #49427, #42023, #14313 ),
 .UNSPECIFIED., .F., .F. ) 
 B_SPLINE_CURVE_WITH_KNOTS ( ( 4, 4 ),
 ( 1.570796326794896558, 3.141592653589793116 ),
 .UNSPECIFIED. ) 
 CURVE ( )  GEOMETRIC_REPRESENTATION_ITEM ( )  RATIONAL_B_SPLINE_CURVE ( ( 1.000000000000000000, 0.8047378541243649375, 0.8047378541243649375, 1.000000000000000000 ) ) 
 REPRESENTATION_ITEM ( '' )  );
#18648=ORIENTED_EDGE ( 'NONE', *, *, #47288, .T. ) ;
#18656=( BOUNDED_CURVE ( )  B_SPLINE_CURVE ( 3, ( #14740, #25790, #49087, #41941 ),
 .UNSPECIFIED., .F., .F. ) 
 B_SPLINE_CURVE_WITH_KNOTS ( ( 4, 4 ),
 ( 3.141592653589793116, 4.712388980384689674 ),
 .UNSPECIFIED. ) 
 CURVE ( )  GEOMETRIC_REPRESENTATION_ITEM ( )  RATIONAL_B_SPLINE_CURVE ( ( 1.000000000000000000, 0.8047378541243649375, 0.8047378541243649375, 1.000000000000000000 ) ) 
 REPRESENTATION_ITEM ( '' )  );
#18658=ORIENTED_EDGE ( 'NONE', *, *, #35190, .F. ) ;
#18663=CARTESIAN_POINT ( 'NONE',  ( -210.0000000000000568, 0.000000000000000000, -37.43171244307202272 ) ) ;
#18669=( BOUNDED_CURVE ( )  B_SPLINE_CURVE ( 3, ( #22785, #38462, #46604, #27152 ),
 .UNSPECIFIED., .F., .F. ) 
 B_SPLINE_CURVE_WITH_KNOTS ( ( 4, 4 ),
 ( 4.712388980384689674, 6.283185307179586232 ),
 .UNSPECIFIED. ) 
 CURVE ( )  GEOMETRIC_REPRESENTATION_ITEM ( )  RATIONAL_B_SPLINE_CURVE ( ( 1.000000000000000000, 0.8047378541243649375, 0.8047378541243649375, 1.000000000000000000 ) ) 
 REPRESENTATION_ITEM ( '' )  );
#18679=AXIS2_PLACEMENT_3D ( 'NONE', #41237, #45061, #33811 ) ;
#18682=ORIENTED_EDGE ( 'NONE', *, *, #23609, .T. ) ;
#18689=EDGE_CURVE ( 'NONE', #29366, #47482, #8515, .T. ) ;
#18690=CARTESIAN_POINT ( 'NONE',  ( 111.5540265531850679, 0.000000000000000000, 79.06828755692798438 ) ) ;
#18696=EDGE_LOOP ( 'NONE', ( #27776, #16706, #26604, #30803, #11569, #47783 ) ) ;
#18709=ORIENTED_EDGE ( 'NONE', *, *, #27069, .F. ) ;
#18712=CARTESIAN_POINT ( 'NONE',  ( -85.67084718096784002, -1.750000000000009548, -38.15658617722494483 ) ) ;
#18713=DIRECTION ( 'NONE',  ( -1.000000000000000000, -0.000000000000000000, -0.000000000000000000 ) ) ;
#18714=ORIENTED_EDGE ( 'NONE', *, *, #44095, .F. ) ;
#18715=DIRECTION ( 'NONE',  ( 0.000000000000000000, 0.000000000000000000, 1.000000000000000000 ) ) ;
#18717=CARTESIAN_POINT ( 'NONE',  ( -8.445973446814976526, 0.000000000000000000, -157.4317124430720014 ) ) ;
#18718=ORIENTED_EDGE ( 'NONE', *, *, #3120, .F. ) ;
#18719=CARTESIAN_POINT ( 'NONE',  ( 73.30402655318508209, 1.750000000000010658, -79.18171244307201562 ) ) ;
#18723=CARTESIAN_POINT ( 'NONE',  ( -6.695973446814940111, 1.750000000000023759, -39.18171244307202983 ) ) ;
#18732=EDGE_CURVE ( 'NONE', #46541, #48958, #29782, .T. ) ;
#18743=DIRECTION ( 'NONE',  ( -0.000000000000000000, -0.000000000000000000, -1.000000000000000000 ) ) ;
#18744=CARTESIAN_POINT ( 'NONE',  ( 155.0540265531850537, 2.143131898507880377E-16, -117.4317124430720725 ) ) ;
#18745=EDGE_CURVE ( 'NONE', #9366, #24608, #34204, .T. ) ;
#18750=FACE_OUTER_BOUND ( 'NONE', #6355, .T. ) ;
#18751=CIRCLE ( 'NONE', #38457, 1.750000000000008438 ) ;
#18760=LINE ( 'NONE', #10330, #17125 ) ;
#18775=CYLINDRICAL_SURFACE ( 'NONE', #8194, 1.750000000000001554 ) ;
#18777=FACE_OUTER_BOUND ( 'NONE', #23858, .T. ) ;
#18782=CARTESIAN_POINT ( 'NONE',  ( 151.5540265531850537, 1.025126265847089213, -0.9317124430720324924 ) ) ;
#18796=LINE ( 'NONE', #34480, #38243 ) ;
#18798=ORIENTED_EDGE ( 'NONE', *, *, #22749, .F. ) ;
#18803=( BOUNDED_CURVE ( )  B_SPLINE_CURVE ( 3, ( #43265, #36100, #39442, #24535 ),
 .UNSPECIFIED., .F., .F. ) 
 B_SPLINE_CURVE_WITH_KNOTS ( ( 4, 4 ),
 ( 3.141592653589793116, 4.712388980384689674 ),
 .UNSPECIFIED. ) 
 CURVE ( )  GEOMETRIC_REPRESENTATION_ITEM ( )  RATIONAL_B_SPLINE_CURVE ( ( 1.000000000000000000, 0.8047378541243649375, 0.8047378541243649375, 1.000000000000000000 ) ) 
 REPRESENTATION_ITEM ( '' )  );
#18807=VERTEX_POINT ( 'NONE', #42626 ) ;
#18809=( BOUNDED_CURVE ( )  B_SPLINE_CURVE ( 3, ( #13253, #21213, #28918, #1727 ),
 .UNSPECIFIED., .F., .F. ) 
 B_SPLINE_CURVE_WITH_KNOTS ( ( 4, 4 ),
 ( 4.712388980384689674, 6.283185307179586232 ),
 .UNSPECIFIED. ) 
 CURVE ( )  GEOMETRIC_REPRESENTATION_ITEM ( )  RATIONAL_B_SPLINE_CURVE ( ( 1.000000000000000000, 0.8047378541243649375, 0.8047378541243649375, 1.000000000000000000 ) ) 
 REPRESENTATION_ITEM ( '' )  );
#18810=CARTESIAN_POINT ( 'NONE',  ( -168.4459734468149463, 0.000000000000000000, -120.9317124430720156 ) ) ;
#18815=CARTESIAN_POINT ( 'NONE',  ( -44.94597344681493922, 2.143131898507880377E-16, -157.4317124430720014 ) ) ;
#18822=CARTESIAN_POINT ( 'NONE',  ( -4.945973446814903696, 2.143131898507912917E-16, 79.06828755692795596 ) ) ;
#18828=CARTESIAN_POINT ( 'NONE',  ( -46.69597344681494633, 0.000000000000000000, 165.0000000000000000 ) ) ;
#18831=AXIS2_PLACEMENT_3D ( 'NONE', #38326, #10358, #3135 ) ;
#18836=EDGE_CURVE ( 'NONE', #40222, #21159, #5205, .T. ) ;
#18837=EDGE_LOOP ( 'NONE', ( #2409, #35066, #18410, #49634, #22596, #39867 ) ) ;
#18839=CARTESIAN_POINT ( 'NONE',  ( 151.5540265531850537, 0.000000000000000000, 42.56828755692798438 ) ) ;
#18841=EDGE_LOOP ( 'NONE', ( #39643, #21962, #28396, #42865, #30363, #38225 ) ) ;
#18846=AXIS2_PLACEMENT_3D ( 'NONE', #44022, #36364, #8886 ) ;
#18848=EDGE_LOOP ( 'NONE', ( #28893, #45077, #49841, #34553, #12957, #30670 ) ) ;
#18852=CARTESIAN_POINT ( 'NONE',  ( 210.0000000000000568, 0.000000000000000000, -157.4317124430720298 ) ) ;
#18853=ORIENTED_EDGE ( 'NONE', *, *, #10198, .T. ) ;
#18861=VERTEX_POINT ( 'NONE', #46449 ) ;
#18863=CARTESIAN_POINT ( 'NONE',  ( 75.05402655318509630, 1.025126265847089435, -40.93171244307204404 ) ) ;
#18869=CARTESIAN_POINT ( 'NONE',  ( -48.44597344681495343, 0.000000000000000000, 159.0682875569279702 ) ) ;
#18881=EDGE_CURVE ( 'NONE', #22379, #48473, #31138, .T. ) ;
#18888=EDGE_CURVE ( 'NONE', #1022, #40841, #20051, .T. ) ;
#18892=ORIENTED_EDGE ( 'NONE', *, *, #12, .T. ) ;
#18896=ADVANCED_FACE ( 'NONE', ( #27505 ), #19282, .T. ) ;
#18897=EDGE_CURVE ( 'NONE', #7763, #18861, #11043, .T. ) ;
#18902=ADVANCED_FACE ( 'NONE', ( #8012 ), #12110, .T. ) ;
#18903=CARTESIAN_POINT ( 'NONE',  ( -164.9459734468149463, 2.143131898507880377E-16, 122.5682875569279702 ) ) ;
#18911=DIRECTION ( 'NONE',  ( -1.000000000000000000, -0.000000000000000000, -0.000000000000000000 ) ) ;
#18914=CARTESIAN_POINT ( 'NONE',  ( -88.44597344681494633, -1.025126265847089435, -40.93171244307204404 ) ) ;
#18915=VERTEX_POINT ( 'NONE', #9261 ) ;
#18918=CARTESIAN_POINT ( 'NONE',  ( -210.0000000000000568, 2.143131898507884075E-16, 39.06828755692797728 ) ) ;
#18919=CARTESIAN_POINT ( 'NONE',  ( 74.32915281903215998, -1.750000000000010436, 79.79316129108087807 ) ) ;
#18920=ADVANCED_FACE ( 'NONE', ( #37249 ), #1819, .T. ) ;
#18921=ORIENTED_EDGE ( 'NONE', *, *, #7076, .T. ) ;
#18928=DIRECTION ( 'NONE',  ( 0.000000000000000000, 0.000000000000000000, 1.000000000000000000 ) ) ;
#18934=EDGE_CURVE ( 'NONE', #20319, #49361, #47120, .T. ) ;
#18937=ORIENTED_EDGE ( 'NONE', *, *, #31719, .F. ) ;
#18943=CARTESIAN_POINT ( 'NONE',  ( 153.3040265531850537, -1.750000000000010658, -79.18171244307201562 ) ) ;
#18950=( BOUNDED_CURVE ( )  B_SPLINE_CURVE ( 3, ( #38258, #45137, #44888, #30283 ),
 .UNSPECIFIED., .F., .F. ) 
 B_SPLINE_CURVE_WITH_KNOTS ( ( 4, 4 ),
 ( 1.570796326794896558, 3.141592653589793116 ),
 .UNSPECIFIED. ) 
 CURVE ( )  GEOMETRIC_REPRESENTATION_ITEM ( )  RATIONAL_B_SPLINE_CURVE ( ( 1.000000000000000000, 0.8047378541243649375, 0.8047378541243649375, 1.000000000000000000 ) ) 
 REPRESENTATION_ITEM ( '' )  );
#18951=LINE ( 'NONE', #50474, #41444 ) ;
#18952=EDGE_CURVE ( 'NONE', #48473, #8241, #36480, .T. ) ;
#18955=ORIENTED_EDGE ( 'NONE', *, *, #47606, .T. ) ;
#18957=DIRECTION ( 'NONE',  ( -1.000000000000000000, -0.000000000000000000, -0.000000000000000000 ) ) ;
#18958=( BOUNDED_CURVE ( )  B_SPLINE_CURVE ( 3, ( #6393, #26144, #6904, #41791 ),
 .UNSPECIFIED., .F., .F. ) 
 B_SPLINE_CURVE_WITH_KNOTS ( ( 4, 4 ),
 ( 3.141592653589793116, 4.712388980384689674 ),
 .UNSPECIFIED. ) 
 CURVE ( )  GEOMETRIC_REPRESENTATION_ITEM ( )  RATIONAL_B_SPLINE_CURVE ( ( 1.000000000000000000, 0.8047378541243649375, 0.8047378541243649375, 1.000000000000000000 ) ) 
 REPRESENTATION_ITEM ( '' )  );
#18961=CARTESIAN_POINT ( 'NONE',  ( 195.0540265531851105, 2.143131898507880377E-16, -120.9317124430720156 ) ) ;
#18962=ADVANCED_FACE ( 'NONE', ( #48713 ), #47963, .T. ) ;
#18965=ORIENTED_EDGE ( 'NONE', *, *, #35302, .F. ) ;
#18966=CARTESIAN_POINT ( 'NONE',  ( 34.32915281903212446, -1.750000000000009548, 81.84341382277507648 ) ) ;
#18970=CARTESIAN_POINT ( 'NONE',  ( 193.3040265531851105, -1.750000000000010214, 40.81828755692798438 ) ) ;
#18971=ORIENTED_EDGE ( 'NONE', *, *, #1470, .F. ) ;
#18973=CARTESIAN_POINT ( 'NONE',  ( -86.69597344681494633, 1.750000000000009992, 0.8182875569279768335 ) ) ;
#18975=EDGE_CURVE ( 'NONE', #30427, #23545, #10243, .T. ) ;
#18976=( BOUNDED_CURVE ( )  B_SPLINE_CURVE ( 3, ( #48085, #16332, #24301, #5284 ),
 .UNSPECIFIED., .F., .F. ) 
 B_SPLINE_CURVE_WITH_KNOTS ( ( 4, 4 ),
 ( 1.570796326794896558, 3.141592653589793116 ),
 .UNSPECIFIED. ) 
 CURVE ( )  GEOMETRIC_REPRESENTATION_ITEM ( )  RATIONAL_B_SPLINE_CURVE ( ( 1.000000000000000000, 0.8047378541243649375, 0.8047378541243649375, 1.000000000000000000 ) ) 
 REPRESENTATION_ITEM ( '' )  );
#18980=ORIENTED_EDGE ( 'NONE', *, *, #43808, .T. ) ;
#18981=CARTESIAN_POINT ( 'NONE',  ( 210.0000000000000568, 0.000000000000000000, 80.81828755692798438 ) ) ;
#18982=EDGE_LOOP ( 'NONE', ( #8752, #27047, #16209, #28166, #48123, #41083 ) ) ;
#18984=CARTESIAN_POINT ( 'NONE',  ( 195.0540265531851105, 2.143131898507880377E-16, -40.93171244307202983 ) ) ;
#18985=CARTESIAN_POINT ( 'NONE',  ( -46.69597344681494633, -1.750000000000010658, -79.18171244307201562 ) ) ;
#18990=EDGE_LOOP ( 'NONE', ( #30796, #20039, #40016, #38350, #15460, #47466 ) ) ;
#19000=CYLINDRICAL_SURFACE ( 'NONE', #34790, 1.750000000000001554 ) ;
#19002=CARTESIAN_POINT ( 'NONE',  ( -88.44597344681494633, 1.025126265847089435, 39.06828755692797728 ) ) ;
#19004=ORIENTED_EDGE ( 'NONE', *, *, #28164, .T. ) ;
#19009=ORIENTED_EDGE ( 'NONE', *, *, #6200, .T. ) ;
#19010=EDGE_LOOP ( 'NONE', ( #26034, #48808 ) ) ;
#19011=CARTESIAN_POINT ( 'NONE',  ( 115.0540265531850395, -1.025126265847081664, 122.5682875569279702 ) ) ;
#19017=CARTESIAN_POINT ( 'NONE',  ( 113.3040265531850537, 0.000000000000000000, 165.0000000000000000 ) ) ;
#19020=AXIS2_PLACEMENT_3D ( 'NONE', #34481, #23167, #42401 ) ;
#19022=CARTESIAN_POINT ( 'NONE',  ( -166.6959734468149463, -1.750000000000010658, -79.18171244307201562 ) ) ;
#19024=CARTESIAN_POINT ( 'NONE',  ( -168.4459734468149463, 0.000000000000000000, 82.56828755692798438 ) ) ;
#19031=ORIENTED_EDGE ( 'NONE', *, *, #34465, .F. ) ;
#19036=CARTESIAN_POINT ( 'NONE',  ( -44.94597344681493922, 1.025126265847089435, 159.0682875569279418 ) ) ;
#19039=ADVANCED_FACE ( 'NONE', ( #10763 ), #25932, .T. ) ;
#19045=CARTESIAN_POINT ( 'NONE',  ( 210.0000000000000568, 0.000000000000000000, -37.43171244307202272 ) ) ;
#19048=EDGE_CURVE ( 'NONE', #18915, #9595, #13736, .T. ) ;
#19052=CARTESIAN_POINT ( 'NONE',  ( -124.9459734468149463, 2.143131898507847836E-16, -80.93171244307201562 ) ) ;
#19055=CARTESIAN_POINT ( 'NONE',  ( -204.9459734468149463, 2.143131898507880377E-16, 119.0682875569279702 ) ) ;
#19056=DIRECTION ( 'NONE',  ( -0.000000000000000000, -0.000000000000000000, -1.000000000000000000 ) ) ;
#19057=CARTESIAN_POINT ( 'NONE',  ( -166.6959734468149463, -1.750000000000009992, -159.1817124430720298 ) ) ;
#19062=CARTESIAN_POINT ( 'NONE',  ( 71.55402655318506788, 0.000000000000000000, 162.5682875569279702 ) ) ;
#19072=CARTESIAN_POINT ( 'NONE',  ( 193.3040265531851105, 1.750000000000010214, 40.81828755692798438 ) ) ;
#19075=EDGE_CURVE ( 'NONE', #40327, #38220, #30035, .T. ) ;
#19077=ORIENTED_EDGE ( 'NONE', *, *, #23146, .F. ) ;
#19080=CARTESIAN_POINT ( 'NONE',  ( -87.72109971266203843, 1.750000000000009548, -38.15658617722494483 ) ) ;
#19086=PLANE ( 'NONE',  #48165 ) ;
#19087=CYLINDRICAL_SURFACE ( 'NONE', #18392, 1.749999999999987566 ) ;
#19093=CARTESIAN_POINT ( 'NONE',  ( -4.945973446814903696, 2.143131898507912917E-16, -120.9317124430720725 ) ) ;
#19095=EDGE_CURVE ( 'NONE', #44210, #2259, #1915, .T. ) ;
#19100=CARTESIAN_POINT ( 'NONE',  ( 155.0540265531850537, 2.143131898507880377E-16, 122.5682875569279702 ) ) ;
#19106=CARTESIAN_POINT ( 'NONE',  ( 73.30402655318508209, 1.750000000000010214, 40.81828755692798438 ) ) ;
#19109=( BOUNDED_CURVE ( )  B_SPLINE_CURVE ( 3, ( #22364, #22623, #29565, #41370 ),
 .UNSPECIFIED., .F., .F. ) 
 B_SPLINE_CURVE_WITH_KNOTS ( ( 4, 4 ),
 ( 3.141592653589793116, 4.712388980384689674 ),
 .UNSPECIFIED. ) 
 CURVE ( )  GEOMETRIC_REPRESENTATION_ITEM ( )  RATIONAL_B_SPLINE_CURVE ( ( 1.000000000000000000, 0.8047378541243649375, 0.8047378541243649375, 1.000000000000000000 ) ) 
 REPRESENTATION_ITEM ( '' )  );
#19110=VERTEX_POINT ( 'NONE', #27438 ) ;
#19116=ORIENTED_EDGE ( 'NONE', *, *, #19075, .T. ) ;
#19118=( BOUNDED_CURVE ( )  B_SPLINE_CURVE ( 3, ( #49147, #10693, #14032, #22252 ),
 .UNSPECIFIED., .F., .F. ) 
 B_SPLINE_CURVE_WITH_KNOTS ( ( 4, 4 ),
 ( 4.712388980384689674, 6.283185307179586232 ),
 .UNSPECIFIED. ) 
 CURVE ( )  GEOMETRIC_REPRESENTATION_ITEM ( )  RATIONAL_B_SPLINE_CURVE ( ( 1.000000000000000000, 0.8047378541243649375, 0.8047378541243649375, 1.000000000000000000 ) ) 
 REPRESENTATION_ITEM ( '' )  );
#19119=DIRECTION ( 'NONE',  ( -0.000000000000000000, -0.000000000000000000, -1.000000000000000000 ) ) ;
#19120=CARTESIAN_POINT ( 'NONE',  ( -124.9459734468149463, 2.143131898507847836E-16, 165.0000000000000000 ) ) ;
#19123=AXIS2_PLACEMENT_3D ( 'NONE', #31409, #7281, #22927 ) ;
#19125=CARTESIAN_POINT ( 'NONE',  ( 113.3040265531850537, 0.000000000000000000, 165.0000000000000000 ) ) ;
#19128=ORIENTED_EDGE ( 'NONE', *, *, #7987, .T. ) ;
#19129=CARTESIAN_POINT ( 'NONE',  ( 34.32915281903212446, 1.750000000000009548, -38.15658617722494483 ) ) ;
#19130=CARTESIAN_POINT ( 'NONE',  ( -128.4459734468149179, 0.000000000000000000, 162.5682875569279702 ) ) ;
#19131=CARTESIAN_POINT ( 'NONE',  ( 210.0000000000000568, 0.000000000000000000, 0.8182875569279768335 ) ) ;
#19132=EDGE_LOOP ( 'NONE', ( #27644, #24467, #41922, #50593, #34918, #10232 ) ) ;
#19135=CARTESIAN_POINT ( 'NONE',  ( -210.0000000000000568, 0.000000000000000000, -119.1817124430720440 ) ) ;
#19137=CARTESIAN_POINT ( 'NONE',  ( 73.30402655318508209, -1.750000000000009992, -159.1817124430720298 ) ) ;
#19138=DIRECTION ( 'NONE',  ( -0.000000000000000000, -0.000000000000000000, -1.000000000000000000 ) ) ;
#19142=DIRECTION ( 'NONE',  ( -1.000000000000000000, -0.000000000000000000, -0.000000000000000000 ) ) ;
#19143=VECTOR ( 'NONE', #25104, 1000.000000000000000 ) ;
#19154=VERTEX_POINT ( 'NONE', #23331 ) ;
#19155=CARTESIAN_POINT ( 'NONE',  ( 112.2789002873379758, 1.749999999999996669, -78.15658617722492352 ) ) ;
#19156=AXIS2_PLACEMENT_3D ( 'NONE', #13724, #40180, #8868 ) ;
#19160=EDGE_CURVE ( 'NONE', #16392, #49806, #28136, .T. ) ;
#19168=ORIENTED_EDGE ( 'NONE', *, *, #38399, .F. ) ;
#19171=DIRECTION ( 'NONE',  ( -1.000000000000000000, -0.000000000000000000, -0.000000000000000000 ) ) ;
#19172=AXIS2_PLACEMENT_3D ( 'NONE', #29660, #38389, #50115 ) ;
#19177=VERTEX_POINT ( 'NONE', #3831 ) ;
#19178=AXIS2_PLACEMENT_3D ( 'NONE', #8990, #5630, #13080 ) ;
#19181=CARTESIAN_POINT ( 'NONE',  ( -207.7210997126620384, -1.750000000000010214, 79.79316129108087807 ) ) ;
#19184=LINE ( 'NONE', #45612, #13043 ) ;
#19191=CARTESIAN_POINT ( 'NONE',  ( 33.30402655318503946, -1.750000000000009992, 160.8182875569279702 ) ) ;
#19196=CARTESIAN_POINT ( 'NONE',  ( -168.4459734468149747, -1.025126265847089657, 79.06828755692797017 ) ) ;
#19197=( BOUNDED_CURVE ( )  B_SPLINE_CURVE ( 3, ( #8182, #5519, #29129, #44752 ),
 .UNSPECIFIED., .F., .F. ) 
 B_SPLINE_CURVE_WITH_KNOTS ( ( 4, 4 ),
 ( 1.570796326794896558, 3.141592653589793116 ),
 .UNSPECIFIED. ) 
 CURVE ( )  GEOMETRIC_REPRESENTATION_ITEM ( )  RATIONAL_B_SPLINE_CURVE ( ( 1.000000000000000000, 0.8047378541243649375, 0.8047378541243649375, 1.000000000000000000 ) ) 
 REPRESENTATION_ITEM ( '' )  );
#19199=VECTOR ( 'NONE', #22944, 1000.000000000000000 ) ;
#19201=CARTESIAN_POINT ( 'NONE',  ( -4.945973446814903696, 2.143131898507912917E-16, -0.9317124430720524764 ) ) ;
#19202=DIRECTION ( 'NONE',  ( -1.000000000000000000, -0.000000000000000000, -0.000000000000000000 ) ) ;
#19203=ORIENTED_EDGE ( 'NONE', *, *, #44542, .T. ) ;
#19204=CARTESIAN_POINT ( 'NONE',  ( -8.445973446814976526, 0.000000000000000000, 82.56828755692801280 ) ) ;
#19209=ORIENTED_EDGE ( 'NONE', *, *, #6410, .F. ) ;
#19211=CARTESIAN_POINT ( 'NONE',  ( -128.4459734468149179, 0.000000000000000000, -80.93171244307201562 ) ) ;
#19213=DIRECTION ( 'NONE',  ( -1.000000000000000000, -0.000000000000000000, -0.000000000000000000 ) ) ;
#19214=VECTOR ( 'NONE', #18129, 1000.000000000000000 ) ;
#19219=EDGE_CURVE ( 'NONE', #38220, #9715, #31306, .T. ) ;
#19223=EDGE_CURVE ( 'NONE', #38145, #31704, #23588, .T. ) ;
#19227=ORIENTED_EDGE ( 'NONE', *, *, #11590, .T. ) ;
#19228=EDGE_CURVE ( 'NONE', #9206, #34485, #35053, .T. ) ;
#19229=ADVANCED_FACE ( 'NONE', ( #11543 ), #47389, .T. ) ;
#19232=DIRECTION ( 'NONE',  ( -0.000000000000000000, -0.000000000000000000, -1.000000000000000000 ) ) ;
#19240=ORIENTED_EDGE ( 'NONE', *, *, #44214, .T. ) ;
#19245=AXIS2_PLACEMENT_3D ( 'NONE', #19443, #35124, #20447 ) ;
#19246=CARTESIAN_POINT ( 'NONE',  ( -128.4459734468149179, 2.143131898507880377E-16, -160.9317124430720298 ) ) ;
#19247=ORIENTED_EDGE ( 'NONE', *, *, #20175, .F. ) ;
#19254=DIRECTION ( 'NONE',  ( -1.000000000000000000, -0.000000000000000000, -0.000000000000000000 ) ) ;
#19257=( BOUNDED_CURVE ( )  B_SPLINE_CURVE ( 3, ( #17395, #25348, #9947, #36935 ),
 .UNSPECIFIED., .F., .F. ) 
 B_SPLINE_CURVE_WITH_KNOTS ( ( 4, 4 ),
 ( 3.141592653589793116, 4.712388980384689674 ),
 .UNSPECIFIED. ) 
 CURVE ( )  GEOMETRIC_REPRESENTATION_ITEM ( )  RATIONAL_B_SPLINE_CURVE ( ( 1.000000000000000000, 0.8047378541243649375, 0.8047378541243649375, 1.000000000000000000 ) ) 
 REPRESENTATION_ITEM ( '' )  );
#19258=CARTESIAN_POINT ( 'NONE',  ( -84.94597344681494633, 2.143131898507880377E-16, 2.568287556927978166 ) ) ;
#19261=ORIENTED_EDGE ( 'NONE', *, *, #12659, .F. ) ;
#19263=ADVANCED_FACE ( 'NONE', ( #19737 ), #7444, .T. ) ;
#19265=( BOUNDED_CURVE ( )  B_SPLINE_CURVE ( 3, ( #19433, #39458, #23546, #8403 ),
 .UNSPECIFIED., .F., .F. ) 
 B_SPLINE_CURVE_WITH_KNOTS ( ( 4, 4 ),
 ( 3.141592653589793116, 4.712388980384689674 ),
 .UNSPECIFIED. ) 
 CURVE ( )  GEOMETRIC_REPRESENTATION_ITEM ( )  RATIONAL_B_SPLINE_CURVE ( ( 1.000000000000000000, 0.8047378541243649375, 0.8047378541243649375, 1.000000000000000000 ) ) 
 REPRESENTATION_ITEM ( '' )  );
#19269=VERTEX_POINT ( 'NONE', #7950 ) ;
#19273=CARTESIAN_POINT ( 'NONE',  ( -6.695973446814940111, 1.750000000000023315, 0.8182875569279768335 ) ) ;
#19276=FACE_OUTER_BOUND ( 'NONE', #25683, .T. ) ;
#19280=( BOUNDED_CURVE ( )  B_SPLINE_CURVE ( 3, ( #22854, #30829, #42601, #11318 ),
 .UNSPECIFIED., .F., .F. ) 
 B_SPLINE_CURVE_WITH_KNOTS ( ( 4, 4 ),
 ( 4.712388980384689674, 6.283185307179586232 ),
 .UNSPECIFIED. ) 
 CURVE ( )  GEOMETRIC_REPRESENTATION_ITEM ( )  RATIONAL_B_SPLINE_CURVE ( ( 1.000000000000000000, 0.8047378541243649375, 0.8047378541243649375, 1.000000000000000000 ) ) 
 REPRESENTATION_ITEM ( '' )  );
#19282=CYLINDRICAL_SURFACE ( 'NONE', #44596, 1.750000000000001554 ) ;
#19283=EDGE_CURVE ( 'NONE', #47848, #18060, #47646, .T. ) ;
#19284=CARTESIAN_POINT ( 'NONE',  ( -88.44597344681497475, 0.000000000000000000, 2.568287556928006143 ) ) ;
#19286=EDGE_CURVE ( 'NONE', #10859, #23653, #37011, .T. ) ;
#19294=CARTESIAN_POINT ( 'NONE',  ( 210.0000000000000568, 0.000000000000000000, 0.8182875569279768335 ) ) ;
#19295=CARTESIAN_POINT ( 'NONE',  ( 210.0000000000000568, 0.000000000000000000, -157.4317124430720298 ) ) ;
#19296=FACE_OUTER_BOUND ( 'NONE', #14210, .T. ) ;
#19298=ORIENTED_EDGE ( 'NONE', *, *, #15818, .T. ) ;
#19300=CARTESIAN_POINT ( 'NONE',  ( -48.44597344681495343, 0.000000000000000000, 82.56828755692798438 ) ) ;
#19303=CARTESIAN_POINT ( 'NONE',  ( 33.30402655318503946, 0.000000000000000000, 165.0000000000000000 ) ) ;
#19305=DIRECTION ( 'NONE',  ( -1.000000000000000000, -0.000000000000000000, -0.000000000000000000 ) ) ;
#19311=AXIS2_PLACEMENT_3D ( 'NONE', #25694, #41336, #48737 ) ;
#19312=ORIENTED_EDGE ( 'NONE', *, *, #18472, .F. ) ;
#19317=EDGE_CURVE ( 'NONE', #48914, #21408, #36421, .T. ) ;
#19318=AXIS2_PLACEMENT_3D ( 'NONE', #32776, #31774, #23812 ) ;
#19319=ORIENTED_EDGE ( 'NONE', *, *, #33414, .F. ) ;
#19321=ORIENTED_EDGE ( 'NONE', *, *, #24513, .F. ) ;
#19322=AXIS2_PLACEMENT_3D ( 'NONE', #47773, #3956, #886 ) ;
#19330=ORIENTED_EDGE ( 'NONE', *, *, #18689, .T. ) ;
#19333=CARTESIAN_POINT ( 'NONE',  ( -208.4459734468149463, 0.000000000000000000, 119.0682875569279702 ) ) ;
#19339=AXIS2_PLACEMENT_3D ( 'NONE', #33400, #25431, #41331 ) ;
#19343=EDGE_CURVE ( 'NONE', #23653, #37708, #48400, .T. ) ;
#19351=CARTESIAN_POINT ( 'NONE',  ( 193.3040265531851105, -1.750000000000010214, 40.81828755692798438 ) ) ;
#19354=CARTESIAN_POINT ( 'NONE',  ( 113.3040265531850537, -1.749999999999997113, 40.81828755692798438 ) ) ;
#19364=ORIENTED_EDGE ( 'NONE', *, *, #7454, .T. ) ;
#19367=AXIS2_PLACEMENT_3D ( 'NONE', #38236, #6911, #26667 ) ;
#19377=DIRECTION ( 'NONE',  ( -0.000000000000000000, -0.000000000000000000, -1.000000000000000000 ) ) ;
#19384=CARTESIAN_POINT ( 'NONE',  ( -84.94597344681493212, 1.025126265847089435, 159.0682875569279418 ) ) ;
#19387=CARTESIAN_POINT ( 'NONE',  ( 210.0000000000000568, 0.000000000000000000, -79.18171244307201562 ) ) ;
#19389=AXIS2_PLACEMENT_3D ( 'NONE', #22477, #11196, #30174 ) ;
#19390=CARTESIAN_POINT ( 'NONE',  ( -205.6708471809678827, 1.750000000000009548, 1.843413822775065825 ) ) ;
#19391=DIRECTION ( 'NONE',  ( -1.000000000000000000, -0.000000000000000000, -0.000000000000000000 ) ) ;
#19395=CARTESIAN_POINT ( 'NONE',  ( -124.9459734468149321, -1.025126265847081886, -120.9317124430720440 ) ) ;
#19396=CARTESIAN_POINT ( 'NONE',  ( -84.94597344681494633, 2.143131898507880377E-16, 119.0682875569279702 ) ) ;
#19401=ADVANCED_FACE ( 'NONE', ( #5079 ), #35911, .T. ) ;
#19404=ORIENTED_EDGE ( 'NONE', *, *, #45385, .F. ) ;
#19406=PLANE ( 'NONE',  #45162 ) ;
#19409=DIRECTION ( 'NONE',  ( -0.000000000000000000, -0.000000000000000000, -1.000000000000000000 ) ) ;
#19411=ADVANCED_FACE ( 'NONE', ( #41246 ), #10454, .T. ) ;
#19413=CARTESIAN_POINT ( 'NONE',  ( 210.0000000000000568, 2.143131898507880377E-16, -0.9317124430720331585 ) ) ;
#19419=EDGE_LOOP ( 'NONE', ( #46240, #13578, #14889, #11389, #23212, #35723 ) ) ;
#19422=CARTESIAN_POINT ( 'NONE',  ( -167.7210997126620384, -1.750000000000009548, -160.2068387089191219 ) ) ;
#19424=CARTESIAN_POINT ( 'NONE',  ( -6.695973446814940111, -1.750000000000023315, 160.8182875569279702 ) ) ;
#19431=( BOUNDED_CURVE ( )  B_SPLINE_CURVE ( 3, ( #18723, #4369, #4111, #43602 ),
 .UNSPECIFIED., .F., .F. ) 
 B_SPLINE_CURVE_WITH_KNOTS ( ( 4, 4 ),
 ( 1.570796326794896558, 3.141592653589793116 ),
 .UNSPECIFIED. ) 
 CURVE ( )  GEOMETRIC_REPRESENTATION_ITEM ( )  RATIONAL_B_SPLINE_CURVE ( ( 1.000000000000000000, 0.8047378541243649375, 0.8047378541243649375, 1.000000000000000000 ) ) 
 REPRESENTATION_ITEM ( '' )  );
#19433=CARTESIAN_POINT ( 'NONE',  ( -124.9459734468149463, 2.143131898507847836E-16, -37.43171244307205825 ) ) ;
#19434=ORIENTED_EDGE ( 'NONE', *, *, #27768, .T. ) ;
#19437=CARTESIAN_POINT ( 'NONE',  ( 195.0540265531851105, -1.025126265847089435, 122.5682875569280128 ) ) ;
#19443=CARTESIAN_POINT ( 'NONE',  ( -86.69597344681496054, 0.000000000000000000, 165.0000000000000000 ) ) ;
#19444=CARTESIAN_POINT ( 'NONE',  ( -7.721099712662037540, 1.750000000000023981, 119.7931612910808781 ) ) ;
#19446=DIRECTION ( 'NONE',  ( 0.000000000000000000, 0.000000000000000000, 1.000000000000000000 ) ) ;
#19447=CARTESIAN_POINT ( 'NONE',  ( -86.69597344681494633, 1.750000000000009992, 0.8182875569279768335 ) ) ;
#19450=ORIENTED_EDGE ( 'NONE', *, *, #31186, .F. ) ;
#19457=CARTESIAN_POINT ( 'NONE',  ( -126.6959734468149321, 0.000000000000000000, 165.0000000000000000 ) ) ;
#19464=CARTESIAN_POINT ( 'NONE',  ( -206.6959734468149463, 0.000000000000000000, 165.0000000000000000 ) ) ;
#19475=ORIENTED_EDGE ( 'NONE', *, *, #23641, .F. ) ;
#19478=CARTESIAN_POINT ( 'NONE',  ( 195.0540265531851105, 2.143131898507880377E-16, 39.06828755692798438 ) ) ;
#19481=LINE ( 'NONE', #27953, #31516 ) ;
#19490=ORIENTED_EDGE ( 'NONE', *, *, #44739, .F. ) ;
#19499=CARTESIAN_POINT ( 'NONE',  ( -126.6959734468149321, -1.749999999999997335, -79.18171244307201562 ) ) ;
#19500=( BOUNDED_CURVE ( )  B_SPLINE_CURVE ( 3, ( #46652, #27200, #15644, #757 ),
 .UNSPECIFIED., .F., .F. ) 
 B_SPLINE_CURVE_WITH_KNOTS ( ( 4, 4 ),
 ( 1.570796326794896558, 3.141592653589793116 ),
 .UNSPECIFIED. ) 
 CURVE ( )  GEOMETRIC_REPRESENTATION_ITEM ( )  RATIONAL_B_SPLINE_CURVE ( ( 1.000000000000000000, 0.8047378541243649375, 0.8047378541243649375, 1.000000000000000000 ) ) 
 REPRESENTATION_ITEM ( '' )  );
#19501=EDGE_LOOP ( 'NONE', ( #27417, #43401, #31658, #5536, #37153, #49265 ) ) ;
#19505=VERTEX_POINT ( 'NONE', #37930 ) ;
#19508=CARTESIAN_POINT ( 'NONE',  ( 153.3040265531850537, -1.750000000000010658, -119.1817124430720440 ) ) ;
#19510=ORIENTED_EDGE ( 'NONE', *, *, #6672, .T. ) ;
#19511=CARTESIAN_POINT ( 'NONE',  ( -84.94597344681493212, 1.025126265847089213, -160.9317124430720014 ) ) ;
#19513=EDGE_CURVE ( 'NONE', #50669, #24507, #38171, .T. ) ;
#19516=EDGE_CURVE ( 'NONE', #42490, #13632, #45070, .T. ) ;
#19519=CARTESIAN_POINT ( 'NONE',  ( -208.4459734468149463, 0.000000000000000000, -80.93171244307201562 ) ) ;
#19530=CARTESIAN_POINT ( 'NONE',  ( -124.9459734468149463, 2.143131898507847836E-16, 165.0000000000000000 ) ) ;
#19531=CARTESIAN_POINT ( 'NONE',  ( 193.3040265531851105, 0.000000000000000000, 165.0000000000000000 ) ) ;
#19533=ORIENTED_EDGE ( 'NONE', *, *, #48630, .T. ) ;
#19537=ORIENTED_EDGE ( 'NONE', *, *, #41293, .F. ) ;
#19538=CARTESIAN_POINT ( 'NONE',  ( -6.695973446814940111, 1.750000000000023759, 40.81828755692798438 ) ) ;
#19544=ORIENTED_EDGE ( 'NONE', *, *, #40912, .F. ) ;
#19545=ADVANCED_FACE ( 'NONE', ( #42502 ), #23535, .T. ) ;
#19547=DIRECTION ( 'NONE',  ( -1.000000000000000000, -0.000000000000000000, -0.000000000000000000 ) ) ;
#19548=VERTEX_POINT ( 'NONE', #8140 ) ;
#19551=DIRECTION ( 'NONE',  ( -1.000000000000000000, 0.000000000000000000, 0.000000000000000000 ) ) ;
#19556=AXIS2_PLACEMENT_3D ( 'NONE', #7290, #10126, #41432 ) ;
#19557=( BOUNDED_CURVE ( )  B_SPLINE_CURVE ( 3, ( #28084, #48037, #20374, #24243 ),
 .UNSPECIFIED., .F., .F. ) 
 B_SPLINE_CURVE_WITH_KNOTS ( ( 4, 4 ),
 ( 4.712388980384689674, 6.283185307179586232 ),
 .UNSPECIFIED. ) 
 CURVE ( )  GEOMETRIC_REPRESENTATION_ITEM ( )  RATIONAL_B_SPLINE_CURVE ( ( 1.000000000000000000, 0.8047378541243649375, 0.8047378541243649375, 1.000000000000000000 ) ) 
 REPRESENTATION_ITEM ( '' )  );
#19559=ORIENTED_EDGE ( 'NONE', *, *, #20191, .T. ) ;
#19560=CARTESIAN_POINT ( 'NONE',  ( 210.0000000000000568, 0.000000000000000000, -37.43171244307202272 ) ) ;
#19568=( BOUNDED_CURVE ( )  B_SPLINE_CURVE ( 3, ( #2007, #37185, #17653, #33320 ),
 .UNSPECIFIED., .F., .F. ) 
 B_SPLINE_CURVE_WITH_KNOTS ( ( 4, 4 ),
 ( 4.712388980384689674, 6.283185307179586232 ),
 .UNSPECIFIED. ) 
 CURVE ( )  GEOMETRIC_REPRESENTATION_ITEM ( )  RATIONAL_B_SPLINE_CURVE ( ( 1.000000000000000000, 0.8047378541243649375, 0.8047378541243649375, 1.000000000000000000 ) ) 
 REPRESENTATION_ITEM ( '' )  );
#19572=DIRECTION ( 'NONE',  ( -0.000000000000000000, -0.000000000000000000, -1.000000000000000000 ) ) ;
#19573=VECTOR ( 'NONE', #26381, 1000.000000000000000 ) ;
#19575=ADVANCED_FACE ( 'NONE', ( #34574 ), #7118, .T. ) ;
#19577=EDGE_CURVE ( 'NONE', #37650, #45334, #10143, .T. ) ;
#19579=ORIENTED_EDGE ( 'NONE', *, *, #29601, .F. ) ;
#19582=CARTESIAN_POINT ( 'NONE',  ( 191.5540265531851105, 0.000000000000000000, 162.5682875569279702 ) ) ;
#19583=EDGE_CURVE ( 'NONE', #27396, #2997, #30727, .T. ) ;
#19585=ORIENTED_EDGE ( 'NONE', *, *, #44379, .T. ) ;
#19587=ORIENTED_EDGE ( 'NONE', *, *, #19228, .T. ) ;
#19595=DIRECTION ( 'NONE',  ( -1.000000000000000000, 0.000000000000000000, 0.000000000000000000 ) ) ;
#19600=FACE_OUTER_BOUND ( 'NONE', #18279, .T. ) ;
#19613=VECTOR ( 'NONE', #5733, 1000.000000000000000 ) ;
#19614=EDGE_CURVE ( 'NONE', #19783, #22379, #17338, .T. ) ;
#19615=EDGE_CURVE ( 'NONE', #33842, #14142, #947, .T. ) ;
#19617=CARTESIAN_POINT ( 'NONE',  ( -127.7210997126620242, 1.749999999999996669, 41.84341382277508359 ) ) ;
#19619=DIRECTION ( 'NONE',  ( -1.000000000000000000, 0.000000000000000000, 0.000000000000000000 ) ) ;
#19623=ORIENTED_EDGE ( 'NONE', *, *, #19343, .T. ) ;
#19629=CARTESIAN_POINT ( 'NONE',  ( 193.3040265531851105, -1.750000000000009992, -159.1817124430720298 ) ) ;
#19637=DIRECTION ( 'NONE',  ( -1.000000000000000000, -0.000000000000000000, -0.000000000000000000 ) ) ;
#19640=EDGE_LOOP ( 'NONE', ( #19840, #4267, #44167, #34189, #26204, #27762 ) ) ;
#19643=EDGE_CURVE ( 'NONE', #43762, #7812, #18976, .T. ) ;
#19646=EDGE_LOOP ( 'NONE', ( #32659, #41642, #47548, #33546, #10772 ) ) ;
#19650=FACE_OUTER_BOUND ( 'NONE', #15364, .T. ) ;
#19651=CARTESIAN_POINT ( 'NONE',  ( 113.3040265531850537, -1.749999999999996891, 0.8182875569279768335 ) ) ;
#19652=ORIENTED_EDGE ( 'NONE', *, *, #2894, .T. ) ;
#19656=VERTEX_POINT ( 'NONE', #36358 ) ;
#19657=AXIS2_PLACEMENT_3D ( 'NONE', #50240, #27464, #35179 ) ;
#19659=CARTESIAN_POINT ( 'NONE',  ( 71.55402655318505367, -1.025126265847089435, -157.4317124430720582 ) ) ;
#19666=CYLINDRICAL_SURFACE ( 'NONE', #3933, 1.750000000000008438 ) ;
#19672=CARTESIAN_POINT ( 'NONE',  ( 194.3291528190321742, 1.750000000000009548, -160.2068387089191219 ) ) ;
#19676=EDGE_CURVE ( 'NONE', #11666, #30190, #43854, .T. ) ;
#19678=VECTOR ( 'NONE', #30187, 1000.000000000000000 ) ;
#19684=CARTESIAN_POINT ( 'NONE',  ( -45.67084718096785423, 1.750000000000010214, 121.8434138227750623 ) ) ;
#19688=CARTESIAN_POINT ( 'NONE',  ( 115.0540265531850395, 1.025126265847081886, -80.93171244307201562 ) ) ;
#19690=ORIENTED_EDGE ( 'NONE', *, *, #20507, .F. ) ;
#19695=AXIS2_PLACEMENT_3D ( 'NONE', #39778, #23866, #1529 ) ;
#19698=CARTESIAN_POINT ( 'NONE',  ( -8.445973446814962315, -1.025126265847096985, 162.5682875569279986 ) ) ;
#19705=VERTEX_POINT ( 'NONE', #28392 ) ;
#19709=ORIENTED_EDGE ( 'NONE', *, *, #6753, .F. ) ;
#19712=CARTESIAN_POINT ( 'NONE',  ( 34.32915281903212446, -1.750000000000010436, 119.7931612910808781 ) ) ;
#19717=CARTESIAN_POINT ( 'NONE',  ( -208.4459734468149463, 0.000000000000000000, 165.0000000000000000 ) ) ;
#19718=AXIS2_PLACEMENT_3D ( 'NONE', #47401, #11800, #42329 ) ;
#19721=CARTESIAN_POINT ( 'NONE',  ( -167.7210997126620384, -1.750000000000010214, 79.79316129108087807 ) ) ;
#19722=CARTESIAN_POINT ( 'NONE',  ( -84.94597344681494633, 2.143131898507880377E-16, 39.06828755692798438 ) ) ;
#19726=FACE_OUTER_BOUND ( 'NONE', #3876, .T. ) ;
#19727=VECTOR ( 'NONE', #12288, 1000.000000000000000 ) ;
#19733=ORIENTED_EDGE ( 'NONE', *, *, #22712, .F. ) ;
#19737=FACE_OUTER_BOUND ( 'NONE', #16252, .T. ) ;
#19740=LINE ( 'NONE', #35419, #17441 ) ;
#19742=EDGE_CURVE ( 'NONE', #27161, #2812, #33094, .T. ) ;
#19745=CARTESIAN_POINT ( 'NONE',  ( 153.3040265531850537, -1.750000000000009992, -159.1817124430720298 ) ) ;
#19746=CARTESIAN_POINT ( 'NONE',  ( 195.0540265531851105, 2.143131898507880377E-16, 122.5682875569279702 ) ) ;
#19747=EDGE_LOOP ( 'NONE', ( #9018, #5880, #40166, #38739, #7278 ) ) ;
#19754=CARTESIAN_POINT ( 'NONE',  ( 191.5540265531851105, 0.000000000000000000, 165.0000000000000000 ) ) ;
#19756=EDGE_LOOP ( 'NONE', ( #8896, #42749, #15368, #18594, #11904, #25352 ) ) ;
#19758=EDGE_CURVE ( 'NONE', #8521, #5706, #10446, .T. ) ;
#19767=EDGE_LOOP ( 'NONE', ( #27554, #12607, #39772, #49675, #21968, #3035 ) ) ;
#19768=CARTESIAN_POINT ( 'NONE',  ( -88.44597344681497475, 0.000000000000000000, -0.9317124430720524764 ) ) ;
#19769=CARTESIAN_POINT ( 'NONE',  ( -86.69597344681494633, 1.750000000000010658, 120.8182875569279702 ) ) ;
#19770=EDGE_LOOP ( 'NONE', ( #27310, #3667, #5318, #10826, #28101 ) ) ;
#19774=CARTESIAN_POINT ( 'NONE',  ( 72.27890028733797578, -1.750000000000010214, -120.2068387089191219 ) ) ;
#19778=AXIS2_PLACEMENT_3D ( 'NONE', #13840, #17943, #33628 ) ;
#19779=CARTESIAN_POINT ( 'NONE',  ( 210.0000000000000568, 2.143131898507880377E-16, 159.0682875569279702 ) ) ;
#19780=ORIENTED_EDGE ( 'NONE', *, *, #35600, .T. ) ;
#19781=ADVANCED_FACE ( 'NONE', ( #17113 ), #16611, .T. ) ;
#19783=VERTEX_POINT ( 'NONE', #28169 ) ;
#19785=CARTESIAN_POINT ( 'NONE',  ( 111.5540265531850537, -1.025126265847081886, -80.93171244307201562 ) ) ;
#19787=CARTESIAN_POINT ( 'NONE',  ( -206.6959734468149463, 1.750000000000010214, -39.18171244307202983 ) ) ;
#19789=VERTEX_POINT ( 'NONE', #16109 ) ;
#19793=DIRECTION ( 'NONE',  ( -1.000000000000000000, -0.000000000000000000, -0.000000000000000000 ) ) ;
#19794=CYLINDRICAL_SURFACE ( 'NONE', #41190, 1.750000000000001554 ) ;
#19797=ORIENTED_EDGE ( 'NONE', *, *, #11131, .T. ) ;
#19800=DIRECTION ( 'NONE',  ( -0.000000000000000000, -0.000000000000000000, -1.000000000000000000 ) ) ;
#19802=DIRECTION ( 'NONE',  ( -0.000000000000000000, -0.000000000000000000, -1.000000000000000000 ) ) ;
#19804=ORIENTED_EDGE ( 'NONE', *, *, #534, .T. ) ;
#19809=CARTESIAN_POINT ( 'NONE',  ( -126.6959734468149321, 1.749999999999996891, 160.8182875569279702 ) ) ;
#19810=( BOUNDED_CURVE ( )  B_SPLINE_CURVE ( 3, ( #6123, #13306, #24624, #1279 ),
 .UNSPECIFIED., .F., .F. ) 
 B_SPLINE_CURVE_WITH_KNOTS ( ( 4, 4 ),
 ( 0.000000000000000000, 1.570796326794896558 ),
 .UNSPECIFIED. ) 
 CURVE ( )  GEOMETRIC_REPRESENTATION_ITEM ( )  RATIONAL_B_SPLINE_CURVE ( ( 1.000000000000000000, 0.8047378541243649375, 0.8047378541243649375, 1.000000000000000000 ) ) 
 REPRESENTATION_ITEM ( '' )  );
#19815=ORIENTED_EDGE ( 'NONE', *, *, #2920, .T. ) ;
#19816=CARTESIAN_POINT ( 'NONE',  ( 155.0540265531850537, 2.143131898507880377E-16, -40.93171244307202983 ) ) ;
#19821=DIRECTION ( 'NONE',  ( -0.000000000000000000, -0.000000000000000000, -1.000000000000000000 ) ) ;
#19823=CARTESIAN_POINT ( 'NONE',  ( 191.5540265531851105, 0.000000000000000000, 165.0000000000000000 ) ) ;
#19832=ORIENTED_EDGE ( 'NONE', *, *, #10325, .F. ) ;
#19837=ADVANCED_FACE ( 'NONE', ( #20210 ), #24070, .T. ) ;
#19839=DIRECTION ( 'NONE',  ( -1.000000000000000000, -0.000000000000000000, -0.000000000000000000 ) ) ;
#19840=ORIENTED_EDGE ( 'NONE', *, *, #46011, .T. ) ;
#19845=CARTESIAN_POINT ( 'NONE',  ( -168.4459734468149747, 1.025126265847089435, -117.4317124430720156 ) ) ;
#19849=ORIENTED_EDGE ( 'NONE', *, *, #39357, .T. ) ;
#19858=ORIENTED_EDGE ( 'NONE', *, *, #10236, .F. ) ;
#19862=( BOUNDED_CURVE ( )  B_SPLINE_CURVE ( 3, ( #43504, #8375, #24021, #31979 ),
 .UNSPECIFIED., .F., .F. ) 
 B_SPLINE_CURVE_WITH_KNOTS ( ( 4, 4 ),
 ( 1.570796326794896558, 3.141592653589793116 ),
 .UNSPECIFIED. ) 
 CURVE ( )  GEOMETRIC_REPRESENTATION_ITEM ( )  RATIONAL_B_SPLINE_CURVE ( ( 1.000000000000000000, 0.8047378541243649375, 0.8047378541243649375, 1.000000000000000000 ) ) 
 REPRESENTATION_ITEM ( '' )  );
#19863=EDGE_CURVE ( 'NONE', #45661, #7807, #24247, .T. ) ;
#19869=( BOUNDED_CURVE ( )  B_SPLINE_CURVE ( 3, ( #45130, #44879, #2559, #33882 ),
 .UNSPECIFIED., .F., .F. ) 
 B_SPLINE_CURVE_WITH_KNOTS ( ( 4, 4 ),
 ( 1.570796326794896558, 3.141592653589793116 ),
 .UNSPECIFIED. ) 
 CURVE ( )  GEOMETRIC_REPRESENTATION_ITEM ( )  RATIONAL_B_SPLINE_CURVE ( ( 1.000000000000000000, 0.8047378541243649375, 0.8047378541243649375, 1.000000000000000000 ) ) 
 REPRESENTATION_ITEM ( '' )  );
#19875=CARTESIAN_POINT ( 'NONE',  ( 153.3040265531850537, -1.750000000000009992, 0.8182875569279768335 ) ) ;
#19876=ADVANCED_FACE ( 'NONE', ( #41211 ), #36902, .T. ) ;
#19878=ORIENTED_EDGE ( 'NONE', *, *, #47586, .F. ) ;
#19879=LINE ( 'NONE', #8096, #48308 ) ;
#19881=CARTESIAN_POINT ( 'NONE',  ( 73.30402655318508209, 1.750000000000010658, 120.8182875569279702 ) ) ;
#19887=CARTESIAN_POINT ( 'NONE',  ( -4.945973446814917018, -1.025126265847096985, 42.56828755692800570 ) ) ;
#19888=VERTEX_POINT ( 'NONE', #25572 ) ;
#19890=VECTOR ( 'NONE', #27247, 1000.000000000000000 ) ;
#19895=DIRECTION ( 'NONE',  ( -1.000000000000000000, -0.000000000000000000, -0.000000000000000000 ) ) ;
#19898=EDGE_CURVE ( 'NONE', #37204, #42077, #36711, .T. ) ;
#19900=CARTESIAN_POINT ( 'NONE',  ( 75.05402655318509630, 2.143131898507880377E-16, -160.9317124430720582 ) ) ;
#19901=CARTESIAN_POINT ( 'NONE',  ( -4.945973446814903696, 2.143131898507912917E-16, -160.9317124430720582 ) ) ;
#19903=EDGE_CURVE ( 'NONE', #50334, #9206, #15398, .T. ) ;
#19909=EDGE_CURVE ( 'NONE', #9194, #9127, #16004, .T. ) ;
#19913=CARTESIAN_POINT ( 'NONE',  ( -4.945973446814903696, 2.143131898507913410E-16, -165.0000000000000000 ) ) ;
#19926=CARTESIAN_POINT ( 'NONE',  ( 194.3291528190321742, -1.750000000000009548, 161.8434138227750907 ) ) ;
#19927=ORIENTED_EDGE ( 'NONE', *, *, #12431, .F. ) ;
#19930=CARTESIAN_POINT ( 'NONE',  ( 32.27890028733795447, -1.750000000000009548, 1.843413822775065825 ) ) ;
#19932=CARTESIAN_POINT ( 'NONE',  ( 114.3291528190321173, 1.749999999999996891, -80.20683870891909351 ) ) ;
#19938=ORIENTED_EDGE ( 'NONE', *, *, #10513, .F. ) ;
#19939=CARTESIAN_POINT ( 'NONE',  ( 193.3040265531851105, 0.000000000000000000, 165.0000000000000000 ) ) ;
#19941=EDGE_CURVE ( 'NONE', #24424, #21250, #20637, .T. ) ;
#19943=VERTEX_POINT ( 'NONE', #9914 ) ;
#19955=DIRECTION ( 'NONE',  ( -1.000000000000000000, -0.000000000000000000, -0.000000000000000000 ) ) ;
#19963=CARTESIAN_POINT ( 'NONE',  ( 111.5540265531850679, 0.000000000000000000, -80.93171244307201562 ) ) ;
#19964=EDGE_CURVE ( 'NONE', #25110, #10906, #25891, .T. ) ;
#19967=EDGE_CURVE ( 'NONE', #2131, #34244, #34750, .T. ) ;
#19974=FACE_OUTER_BOUND ( 'NONE', #6324, .T. ) ;
#19982=ORIENTED_EDGE ( 'NONE', *, *, #19742, .F. ) ;
#19984=EDGE_CURVE ( 'NONE', #16730, #49806, #3736, .T. ) ;
#19988=ORIENTED_EDGE ( 'NONE', *, *, #27216, .F. ) ;
#19994=VERTEX_POINT ( 'NONE', #27342 ) ;
#19998=CARTESIAN_POINT ( 'NONE',  ( -48.44597344681495343, 0.000000000000000000, 2.568287556927978166 ) ) ;
#20002=AXIS2_PLACEMENT_3D ( 'NONE', #32066, #47657, #12547 ) ;
#20003=ORIENTED_EDGE ( 'NONE', *, *, #48189, .F. ) ;
#20005=CARTESIAN_POINT ( 'NONE',  ( 71.55402655318505367, 0.000000000000000000, 165.0000000000000000 ) ) ;
#20010=FACE_OUTER_BOUND ( 'NONE', #38751, .T. ) ;
#20013=( BOUNDED_CURVE ( )  B_SPLINE_CURVE ( 3, ( #39995, #35398, #4813, #20469 ),
 .UNSPECIFIED., .F., .F. ) 
 B_SPLINE_CURVE_WITH_KNOTS ( ( 4, 4 ),
 ( 0.000000000000000000, 1.570796326794896558 ),
 .UNSPECIFIED. ) 
 CURVE ( )  GEOMETRIC_REPRESENTATION_ITEM ( )  RATIONAL_B_SPLINE_CURVE ( ( 1.000000000000000000, 0.8047378541243649375, 0.8047378541243649375, 1.000000000000000000 ) ) 
 REPRESENTATION_ITEM ( '' )  );
#20015=ORIENTED_EDGE ( 'NONE', *, *, #40714, .T. ) ;
#20017=CARTESIAN_POINT ( 'NONE',  ( -210.0000000000000568, 0.000000000000000000, 40.81828755692798438 ) ) ;
#20019=CARTESIAN_POINT ( 'NONE',  ( 193.3040265531851105, 1.750000000000009992, -159.1817124430720298 ) ) ;
#20020=( BOUNDED_CURVE ( )  B_SPLINE_CURVE ( 3, ( #27551, #36016, #855, #20591 ),
 .UNSPECIFIED., .F., .F. ) 
 B_SPLINE_CURVE_WITH_KNOTS ( ( 4, 4 ),
 ( 4.712388980384689674, 6.283185307179586232 ),
 .UNSPECIFIED. ) 
 CURVE ( )  GEOMETRIC_REPRESENTATION_ITEM ( )  RATIONAL_B_SPLINE_CURVE ( ( 1.000000000000000000, 0.8047378541243649375, 0.8047378541243649375, 1.000000000000000000 ) ) 
 REPRESENTATION_ITEM ( '' )  );
#20027=EDGE_CURVE ( 'NONE', #27168, #47806, #6827, .T. ) ;
#20035=ADVANCED_FACE ( 'NONE', ( #14778 ), #30431, .T. ) ;
#20039=ORIENTED_EDGE ( 'NONE', *, *, #32906, .F. ) ;
#20051=LINE ( 'NONE', #19530, #29905 ) ;
#20052=FACE_OUTER_BOUND ( 'NONE', #15044, .T. ) ;
#20055=CARTESIAN_POINT ( 'NONE',  ( 191.5540265531850537, -1.025126265847089657, 119.0682875569279560 ) ) ;
#20058=VECTOR ( 'NONE', #38252, 1000.000000000000000 ) ;
#20060=DIRECTION ( 'NONE',  ( -1.000000000000000000, -0.000000000000000000, -0.000000000000000000 ) ) ;
#20062=CARTESIAN_POINT ( 'NONE',  ( -206.6959734468149463, -1.750000000000010214, -39.18171244307202983 ) ) ;
#20063=VERTEX_POINT ( 'NONE', #16808 ) ;
#20066=ORIENTED_EDGE ( 'NONE', *, *, #49509, .T. ) ;
#20069=CARTESIAN_POINT ( 'NONE',  ( -128.4459734468149179, 0.000000000000000000, -165.0000000000000000 ) ) ;
#20070=DIRECTION ( 'NONE',  ( -0.000000000000000000, -0.000000000000000000, -1.000000000000000000 ) ) ;
#20071=LINE ( 'NONE', #47235, #36522 ) ;
#20078=CARTESIAN_POINT ( 'NONE',  ( -126.6959734468149321, -1.749999999999997335, -119.1817124430720440 ) ) ;
#20080=CARTESIAN_POINT ( 'NONE',  ( -126.6959734468149321, 0.000000000000000000, 165.0000000000000000 ) ) ;
#20084=DIRECTION ( 'NONE',  ( -1.000000000000000000, 0.000000000000000000, 0.000000000000000000 ) ) ;
#20093=CARTESIAN_POINT ( 'NONE',  ( -204.9459734468149463, 2.143131898507880377E-16, -157.4317124430720582 ) ) ;
#20096=LINE ( 'NONE', #16007, #50120 ) ;
#20113=VECTOR ( 'NONE', #35707, 1000.000000000000000 ) ;
#20119=CARTESIAN_POINT ( 'NONE',  ( 210.0000000000000568, 0.000000000000000000, -159.1817124430720298 ) ) ;
#20121=AXIS2_PLACEMENT_3D ( 'NONE', #49043, #1403, #13929 ) ;
#20124=CARTESIAN_POINT ( 'NONE',  ( -166.6959734468149463, 1.750000000000010214, 40.81828755692798438 ) ) ;
#20127=ORIENTED_EDGE ( 'NONE', *, *, #2980, .F. ) ;
#20128=ORIENTED_EDGE ( 'NONE', *, *, #13650, .T. ) ;
#20137=CARTESIAN_POINT ( 'NONE',  ( -204.9459734468148895, -1.025126265847089213, 42.56828755692799149 ) ) ;
#20138=CARTESIAN_POINT ( 'NONE',  ( -86.69597344681496054, 0.000000000000000000, -165.0000000000000000 ) ) ;
#20139=AXIS2_PLACEMENT_3D ( 'NONE', #13709, #25515, #6009 ) ;
#20141=VERTEX_POINT ( 'NONE', #918 ) ;
#20143=VECTOR ( 'NONE', #16832, 1000.000000000000000 ) ;
#20145=CARTESIAN_POINT ( 'NONE',  ( 210.0000000000000568, 2.143131898507881856E-16, 119.0682875569279560 ) ) ;
#20155=DIRECTION ( 'NONE',  ( -1.000000000000000000, -0.000000000000000000, -0.000000000000000000 ) ) ;
#20167=CARTESIAN_POINT ( 'NONE',  ( -48.44597344681496054, 1.025126265847089657, -80.93171244307201562 ) ) ;
#20171=EDGE_CURVE ( 'NONE', #7456, #36951, #32475, .T. ) ;
#20172=( BOUNDED_CURVE ( )  B_SPLINE_CURVE ( 3, ( #18744, #31341, #15424, #19508 ),
 .UNSPECIFIED., .F., .F. ) 
 B_SPLINE_CURVE_WITH_KNOTS ( ( 4, 4 ),
 ( 3.141592653589793116, 4.712388980384689674 ),
 .UNSPECIFIED. ) 
 CURVE ( )  GEOMETRIC_REPRESENTATION_ITEM ( )  RATIONAL_B_SPLINE_CURVE ( ( 1.000000000000000000, 0.8047378541243649375, 0.8047378541243649375, 1.000000000000000000 ) ) 
 REPRESENTATION_ITEM ( '' )  );
#20175=EDGE_CURVE ( 'NONE', #26183, #45274, #43238, .T. ) ;
#20176=( BOUNDED_CURVE ( )  B_SPLINE_CURVE ( 3, ( #26371, #37437, #13546, #29460 ),
 .UNSPECIFIED., .F., .F. ) 
 B_SPLINE_CURVE_WITH_KNOTS ( ( 4, 4 ),
 ( 0.000000000000000000, 1.570796326794896558 ),
 .UNSPECIFIED. ) 
 CURVE ( )  GEOMETRIC_REPRESENTATION_ITEM ( )  RATIONAL_B_SPLINE_CURVE ( ( 1.000000000000000000, 0.8047378541243649375, 0.8047378541243649375, 1.000000000000000000 ) ) 
 REPRESENTATION_ITEM ( '' )  );
#20177=ADVANCED_FACE ( 'NONE', ( #39417 ), #47809, .F. ) ;
#20181=EDGE_CURVE ( 'NONE', #14015, #14684, #14030, .T. ) ;
#20182=ORIENTED_EDGE ( 'NONE', *, *, #10622, .T. ) ;
#20187=CARTESIAN_POINT ( 'NONE',  ( 73.30402655318508209, -1.750000000000010658, -79.18171244307201562 ) ) ;
#20190=CARTESIAN_POINT ( 'NONE',  ( 111.5540265531850679, 0.000000000000000000, 122.5682875569279560 ) ) ;
#20191=EDGE_CURVE ( 'NONE', #24864, #14077, #15690, .T. ) ;
#20196=CARTESIAN_POINT ( 'NONE',  ( -8.445973446814964092, 1.025126265847097429, 79.06828755692792754 ) ) ;
#20204=ORIENTED_EDGE ( 'NONE', *, *, #28961, .T. ) ;
#20207=CYLINDRICAL_SURFACE ( 'NONE', #41531, 1.750000000000001554 ) ;
#20208=ORIENTED_EDGE ( 'NONE', *, *, #8704, .F. ) ;
#20209=DIRECTION ( 'NONE',  ( -1.000000000000000000, -0.000000000000000000, -0.000000000000000000 ) ) ;
#20210=FACE_OUTER_BOUND ( 'NONE', #25214, .T. ) ;
#20220=ORIENTED_EDGE ( 'NONE', *, *, #45836, .T. ) ;
#20221=EDGE_CURVE ( 'NONE', #7107, #6771, #5503, .T. ) ;
#20230=CARTESIAN_POINT ( 'NONE',  ( 151.5540265531850537, 0.000000000000000000, 159.0682875569279702 ) ) ;
#20231=CARTESIAN_POINT ( 'NONE',  ( -168.4459734468149463, 0.000000000000000000, 165.0000000000000000 ) ) ;
#20233=CARTESIAN_POINT ( 'NONE',  ( 151.5540265531850537, 0.000000000000000000, 42.56828755692798438 ) ) ;
#20234=DIRECTION ( 'NONE',  ( 1.000000000000000000, 0.000000000000000000, -0.000000000000000000 ) ) ;
#20237=CARTESIAN_POINT ( 'NONE',  ( 210.0000000000000568, 0.000000000000000000, 0.8182875569279768335 ) ) ;
#20240=ORIENTED_EDGE ( 'NONE', *, *, #16472, .T. ) ;
#20242=CARTESIAN_POINT ( 'NONE',  ( 115.0540265531850395, 2.143131898507847836E-16, 165.0000000000000000 ) ) ;
#20245=EDGE_CURVE ( 'NONE', #12842, #13365, #42208, .T. ) ;
#20247=FACE_OUTER_BOUND ( 'NONE', #19767, .T. ) ;
#20250=ADVANCED_FACE ( 'NONE', ( #36837 ), #29614, .T. ) ;
#20255=ORIENTED_EDGE ( 'NONE', *, *, #15140, .F. ) ;
#20257=ORIENTED_EDGE ( 'NONE', *, *, #40000, .T. ) ;
#20262=CARTESIAN_POINT ( 'NONE',  ( 72.27890028733797578, 1.750000000000010436, 79.79316129108087807 ) ) ;
#20263=CARTESIAN_POINT ( 'NONE',  ( -205.6708471809678827, 1.750000000000010214, 121.8434138227750623 ) ) ;
#20274=ORIENTED_EDGE ( 'NONE', *, *, #48358, .F. ) ;
#20279=LINE ( 'NONE', #3866, #29223 ) ;
#20280=ORIENTED_EDGE ( 'NONE', *, *, #6052, .T. ) ;
#20281=CARTESIAN_POINT ( 'NONE',  ( -46.69597344681494633, 1.750000000000010658, 80.81828755692798438 ) ) ;
#20283=DIRECTION ( 'NONE',  ( -0.000000000000000000, -0.000000000000000000, -1.000000000000000000 ) ) ;
#20284=CARTESIAN_POINT ( 'NONE',  ( -86.69597344681494633, -1.750000000000009992, 0.8182875569279768335 ) ) ;
#20295=FACE_OUTER_BOUND ( 'NONE', #7270, .T. ) ;
#20297=CARTESIAN_POINT ( 'NONE',  ( -84.94597344681494633, 2.143131898507880377E-16, -117.4317124430720725 ) ) ;
#20298=VERTEX_POINT ( 'NONE', #25259 ) ;
#20299=LINE ( 'NONE', #1059, #10810 ) ;
#20301=DIRECTION ( 'NONE',  ( -1.000000000000000000, 0.000000000000000000, 0.000000000000000000 ) ) ;
#20303=CYLINDRICAL_SURFACE ( 'NONE', #237, 1.750000000000036193 ) ;
#20309=CARTESIAN_POINT ( 'NONE',  ( 155.0540265531850537, 2.143131898507880377E-16, 119.0682875569279702 ) ) ;
#20310=CARTESIAN_POINT ( 'NONE',  ( -6.695973446814940111, 1.750000000000023759, -39.18171244307202983 ) ) ;
#20312=CYLINDRICAL_SURFACE ( 'NONE', #10776, 1.750000000000001554 ) ;
#20314=( BOUNDED_CURVE ( )  B_SPLINE_CURVE ( 3, ( #9874, #9125, #1437, #25276 ),
 .UNSPECIFIED., .F., .F. ) 
 B_SPLINE_CURVE_WITH_KNOTS ( ( 4, 4 ),
 ( 1.570796326794896558, 3.141592653589793116 ),
 .UNSPECIFIED. ) 
 CURVE ( )  GEOMETRIC_REPRESENTATION_ITEM ( )  RATIONAL_B_SPLINE_CURVE ( ( 1.000000000000000000, 0.8047378541243649375, 0.8047378541243649375, 1.000000000000000000 ) ) 
 REPRESENTATION_ITEM ( '' )  );
#20319=VERTEX_POINT ( 'NONE', #3672 ) ;
#20320=CARTESIAN_POINT ( 'NONE',  ( -6.695973446814940111, 1.750000000000023315, 0.8182875569279768335 ) ) ;
#20321=CYLINDRICAL_SURFACE ( 'NONE', #17505, 1.750000000000008438 ) ;
#20329=EDGE_CURVE ( 'NONE', #25250, #37586, #22580, .T. ) ;
#20338=( BOUNDED_CURVE ( )  B_SPLINE_CURVE ( 3, ( #26718, #49250, #18237, #34427 ),
 .UNSPECIFIED., .F., .F. ) 
 B_SPLINE_CURVE_WITH_KNOTS ( ( 4, 4 ),
 ( 4.712388980384689674, 6.283185307179586232 ),
 .UNSPECIFIED. ) 
 CURVE ( )  GEOMETRIC_REPRESENTATION_ITEM ( )  RATIONAL_B_SPLINE_CURVE ( ( 1.000000000000000000, 0.8047378541243649375, 0.8047378541243649375, 1.000000000000000000 ) ) 
 REPRESENTATION_ITEM ( '' )  );
#20339=DIRECTION ( 'NONE',  ( -0.000000000000000000, -0.000000000000000000, -1.000000000000000000 ) ) ;
#20340=ORIENTED_EDGE ( 'NONE', *, *, #5835, .F. ) ;
#20341=AXIS2_PLACEMENT_3D ( 'NONE', #32801, #48393, #8938 ) ;
#20343=ORIENTED_EDGE ( 'NONE', *, *, #16863, .F. ) ;
#20361=CARTESIAN_POINT ( 'NONE',  ( -46.69597344681494633, -1.750000000000010658, 80.81828755692798438 ) ) ;
#20374=CARTESIAN_POINT ( 'NONE',  ( -168.4459734468149747, 1.025126265847089213, -160.9317124430720014 ) ) ;
#20379=CARTESIAN_POINT ( 'NONE',  ( 154.3291528190321458, 1.750000000000010214, 81.84341382277507648 ) ) ;
#20380=CARTESIAN_POINT ( 'NONE',  ( -48.44597344681496054, 1.025126265847088991, -157.4317124430720582 ) ) ;
#20381=EDGE_CURVE ( 'NONE', #13763, #10372, #42663, .T. ) ;
#20387=CARTESIAN_POINT ( 'NONE',  ( -206.6959734468149463, 0.000000000000000000, 165.0000000000000000 ) ) ;
#20405=DIRECTION ( 'NONE',  ( -0.000000000000000000, -0.000000000000000000, -1.000000000000000000 ) ) ;
#20406=CARTESIAN_POINT ( 'NONE',  ( -48.44597344681492501, 0.000000000000000000, 162.5682875569279702 ) ) ;
#20408=VECTOR ( 'NONE', #23132, 1000.000000000000000 ) ;
#20409=( BOUNDED_CURVE ( )  B_SPLINE_CURVE ( 3, ( #22560, #34139, #7174, #3825 ),
 .UNSPECIFIED., .F., .F. ) 
 B_SPLINE_CURVE_WITH_KNOTS ( ( 4, 4 ),
 ( 3.141592653589793116, 4.712388980384689674 ),
 .UNSPECIFIED. ) 
 CURVE ( )  GEOMETRIC_REPRESENTATION_ITEM ( )  RATIONAL_B_SPLINE_CURVE ( ( 1.000000000000000000, 0.8047378541243649375, 0.8047378541243649375, 1.000000000000000000 ) ) 
 REPRESENTATION_ITEM ( '' )  );
#20412=VERTEX_POINT ( 'NONE', #22920 ) ;
#20420=CYLINDRICAL_SURFACE ( 'NONE', #49077, 1.750000000000001554 ) ;
#20422=CARTESIAN_POINT ( 'NONE',  ( -166.6959734468149463, 0.000000000000000000, 165.0000000000000000 ) ) ;
#20423=ORIENTED_EDGE ( 'NONE', *, *, #43987, .F. ) ;
#20427=FACE_OUTER_BOUND ( 'NONE', #25979, .T. ) ;
#20429=CARTESIAN_POINT ( 'NONE',  ( 31.55402655318503236, 0.000000000000000000, -77.43171244307198720 ) ) ;
#20439=ORIENTED_EDGE ( 'NONE', *, *, #42119, .T. ) ;
#20440=CYLINDRICAL_SURFACE ( 'NONE', #13111, 1.749999999999987566 ) ;
#20442=ORIENTED_EDGE ( 'NONE', *, *, #25315, .T. ) ;
#20447=DIRECTION ( 'NONE',  ( -1.000000000000000000, 0.000000000000000000, 0.000000000000000000 ) ) ;
#20448=CARTESIAN_POINT ( 'NONE',  ( -7.721099712662037540, -1.750000000000022871, -158.1565861772249093 ) ) ;
#20450=AXIS2_PLACEMENT_3D ( 'NONE', #40953, #1460, #48347 ) ;
#20451=ORIENTED_EDGE ( 'NONE', *, *, #11821, .T. ) ;
#20454=ORIENTED_EDGE ( 'NONE', *, *, #35416, .T. ) ;
#20457=CARTESIAN_POINT ( 'NONE',  ( -206.6959734468149463, -1.750000000000010658, 120.8182875569279702 ) ) ;
#20459=EDGE_CURVE ( 'NONE', #49775, #12842, #45175, .T. ) ;
#20462=EDGE_CURVE ( 'NONE', #38939, #30056, #1618, .T. ) ;
#20464=FACE_OUTER_BOUND ( 'NONE', #35981, .T. ) ;
#20467=( BOUNDED_CURVE ( )  B_SPLINE_CURVE ( 3, ( #15925, #39790, #27723, #31841 ),
 .UNSPECIFIED., .F., .F. ) 
 B_SPLINE_CURVE_WITH_KNOTS ( ( 4, 4 ),
 ( 4.712388980384689674, 6.283185307179586232 ),
 .UNSPECIFIED. ) 
 CURVE ( )  GEOMETRIC_REPRESENTATION_ITEM ( )  RATIONAL_B_SPLINE_CURVE ( ( 1.000000000000000000, 0.8047378541243649375, 0.8047378541243649375, 1.000000000000000000 ) ) 
 REPRESENTATION_ITEM ( '' )  );
#20469=CARTESIAN_POINT ( 'NONE',  ( 33.30402655318503946, 1.750000000000009992, -159.1817124430720298 ) ) ;
#20473=( BOUNDED_CURVE ( )  B_SPLINE_CURVE ( 3, ( #49643, #14533, #29945, #26086 ),
 .UNSPECIFIED., .F., .F. ) 
 B_SPLINE_CURVE_WITH_KNOTS ( ( 4, 4 ),
 ( 1.570796326794896558, 3.141592653589793116 ),
 .UNSPECIFIED. ) 
 CURVE ( )  GEOMETRIC_REPRESENTATION_ITEM ( )  RATIONAL_B_SPLINE_CURVE ( ( 1.000000000000000000, 0.8047378541243649375, 0.8047378541243649375, 1.000000000000000000 ) ) 
 REPRESENTATION_ITEM ( '' )  );
#20475=ADVANCED_FACE ( 'NONE', ( #14974 ), #20588, .T. ) ;
#20478=AXIS2_PLACEMENT_3D ( 'NONE', #18981, #6681, #34659 ) ;
#20479=AXIS2_PLACEMENT_3D ( 'NONE', #2318, #2813, #37996 ) ;
#20480=CYLINDRICAL_SURFACE ( 'NONE', #33100, 1.750000000000036193 ) ;
#20481=EDGE_CURVE ( 'NONE', #3971, #47427, #16243, .T. ) ;
#20486=ORIENTED_EDGE ( 'NONE', *, *, #4837, .T. ) ;
#20487=LINE ( 'NONE', #17147, #758 ) ;
#20501=CARTESIAN_POINT ( 'NONE',  ( -208.4459734468149463, 0.000000000000000000, 159.0682875569279702 ) ) ;
#20502=ADVANCED_FACE ( 'NONE', ( #4696 ), #43670, .T. ) ;
#20503=ORIENTED_EDGE ( 'NONE', *, *, #48476, .T. ) ;
#20507=EDGE_CURVE ( 'NONE', #25771, #40611, #46992, .T. ) ;
#20510=CARTESIAN_POINT ( 'NONE',  ( -5.670847180967843570, -1.750000000000022871, 161.8434138227750907 ) ) ;
#20511=ORIENTED_EDGE ( 'NONE', *, *, #32433, .F. ) ;
#20517=ORIENTED_EDGE ( 'NONE', *, *, #39854, .T. ) ;
#20522=ORIENTED_EDGE ( 'NONE', *, *, #7013, .F. ) ;
#20525=VERTEX_POINT ( 'NONE', #95 ) ;
#20534=CARTESIAN_POINT ( 'NONE',  ( -46.69597344681494633, -1.750000000000010658, -79.18171244307201562 ) ) ;
#20537=EDGE_CURVE ( 'NONE', #11343, #16858, #4934, .T. ) ;
#20541=EDGE_LOOP ( 'NONE', ( #18050, #2265, #24663, #36244, #26820, #18122 ) ) ;
#20545=CARTESIAN_POINT ( 'NONE',  ( -8.445973446814976526, 0.000000000000000000, -37.43171244307200141 ) ) ;
#20549=CARTESIAN_POINT ( 'NONE',  ( 210.0000000000000568, 2.143131898507881856E-16, -120.9317124430720582 ) ) ;
#20554=LINE ( 'NONE', #30032, #46806 ) ;
#20556=CARTESIAN_POINT ( 'NONE',  ( -205.6708471809678827, -1.750000000000009326, 161.8434138227750907 ) ) ;
#20559=VERTEX_POINT ( 'NONE', #8298 ) ;
#20562=ORIENTED_EDGE ( 'NONE', *, *, #39401, .F. ) ;
#20563=EDGE_LOOP ( 'NONE', ( #21104, #4411, #37786, #41091, #37711, #34994 ) ) ;
#20564=CYLINDRICAL_SURFACE ( 'NONE', #6599, 1.750000000000001554 ) ;
#20565=CARTESIAN_POINT ( 'NONE',  ( -208.4459734468148611, -1.025126265847089213, 159.0682875569279418 ) ) ;
#20567=CARTESIAN_POINT ( 'NONE',  ( -85.67084718096784002, 1.750000000000010214, -80.20683870891910772 ) ) ;
#20568=DIRECTION ( 'NONE',  ( 0.000000000000000000, 0.000000000000000000, 1.000000000000000000 ) ) ;
#20571=ADVANCED_FACE ( 'NONE', ( #32653 ), #29052, .T. ) ;
#20572=EDGE_LOOP ( 'NONE', ( #35961, #15823 ) ) ;
#20573=CARTESIAN_POINT ( 'NONE',  ( -164.9459734468149463, 1.025126265847089435, 39.06828755692797728 ) ) ;
#20574=CARTESIAN_POINT ( 'NONE',  ( -166.6959734468149463, 0.000000000000000000, 165.0000000000000000 ) ) ;
#20576=CYLINDRICAL_SURFACE ( 'NONE', #50405, 1.750000000000015543 ) ;
#20580=VERTEX_POINT ( 'NONE', #48501 ) ;
#20581=CARTESIAN_POINT ( 'NONE',  ( -4.945973446814903696, 2.143131898507912917E-16, 165.0000000000000000 ) ) ;
#20582=CARTESIAN_POINT ( 'NONE',  ( -164.9459734468149463, -1.025126265847089435, 39.06828755692797728 ) ) ;
#20584=VERTEX_POINT ( 'NONE', #33662 ) ;
#20588=CYLINDRICAL_SURFACE ( 'NONE', #24288, 1.750000000000015543 ) ;
#20591=CARTESIAN_POINT ( 'NONE',  ( -204.9459734468149463, 2.143131898507880377E-16, 119.0682875569279702 ) ) ;
#20592=ORIENTED_EDGE ( 'NONE', *, *, #50621, .F. ) ;
#20593=ORIENTED_EDGE ( 'NONE', *, *, #49638, .T. ) ;
#20594=ADVANCED_FACE ( 'NONE', ( #41353 ), #44423, .T. ) ;
#20599=ORIENTED_EDGE ( 'NONE', *, *, #18745, .T. ) ;
#20604=ORIENTED_EDGE ( 'NONE', *, *, #4805, .F. ) ;
#20608=CARTESIAN_POINT ( 'NONE',  ( 151.5540265531850537, 0.000000000000000000, 39.06828755692798438 ) ) ;
#20610=EDGE_CURVE ( 'NONE', #10906, #12365, #29549, .T. ) ;
#20612=CARTESIAN_POINT ( 'NONE',  ( 151.5540265531850537, 0.000000000000000000, -77.43171244307204404 ) ) ;
#20615=CARTESIAN_POINT ( 'NONE',  ( -204.9459734468148895, -1.025126265847089213, 159.0682875569279418 ) ) ;
#20620=EDGE_CURVE ( 'NONE', #40787, #14561, #50416, .T. ) ;
#20621=( BOUNDED_CURVE ( )  B_SPLINE_CURVE ( 3, ( #47183, #31843, #4126, #19768 ),
 .UNSPECIFIED., .F., .F. ) 
 B_SPLINE_CURVE_WITH_KNOTS ( ( 4, 4 ),
 ( 4.712388980384689674, 6.283185307179586232 ),
 .UNSPECIFIED. ) 
 CURVE ( )  GEOMETRIC_REPRESENTATION_ITEM ( )  RATIONAL_B_SPLINE_CURVE ( ( 1.000000000000000000, 0.8047378541243649375, 0.8047378541243649375, 1.000000000000000000 ) ) 
 REPRESENTATION_ITEM ( '' )  );
#20623=ORIENTED_EDGE ( 'NONE', *, *, #30204, .T. ) ;
#20625=ORIENTED_EDGE ( 'NONE', *, *, #46351, .T. ) ;
#20627=( BOUNDED_CURVE ( )  B_SPLINE_CURVE ( 3, ( #37244, #2066, #3311, #26168 ),
 .UNSPECIFIED., .F., .F. ) 
 B_SPLINE_CURVE_WITH_KNOTS ( ( 4, 4 ),
 ( 3.141592653589793116, 4.712388980384689674 ),
 .UNSPECIFIED. ) 
 CURVE ( )  GEOMETRIC_REPRESENTATION_ITEM ( )  RATIONAL_B_SPLINE_CURVE ( ( 1.000000000000000000, 0.8047378541243649375, 0.8047378541243649375, 1.000000000000000000 ) ) 
 REPRESENTATION_ITEM ( '' )  );
#20637=( BOUNDED_CURVE ( )  B_SPLINE_CURVE ( 3, ( #50384, #35321, #7086, #39158 ),
 .UNSPECIFIED., .F., .F. ) 
 B_SPLINE_CURVE_WITH_KNOTS ( ( 4, 4 ),
 ( 1.570796326794896558, 3.141592653589793116 ),
 .UNSPECIFIED. ) 
 CURVE ( )  GEOMETRIC_REPRESENTATION_ITEM ( )  RATIONAL_B_SPLINE_CURVE ( ( 1.000000000000000000, 0.8047378541243649375, 0.8047378541243649375, 1.000000000000000000 ) ) 
 REPRESENTATION_ITEM ( '' )  );
#20639=ORIENTED_EDGE ( 'NONE', *, *, #42742, .F. ) ;
#20641=DIRECTION ( 'NONE',  ( -0.000000000000000000, -0.000000000000000000, -1.000000000000000000 ) ) ;
#20643=ORIENTED_EDGE ( 'NONE', *, *, #21107, .F. ) ;
#20645=DIRECTION ( 'NONE',  ( -1.000000000000000000, -0.000000000000000000, -0.000000000000000000 ) ) ;
#20652=CARTESIAN_POINT ( 'NONE',  ( -4.945973446814903696, 2.143131898507912917E-16, 42.56828755692802702 ) ) ;
#20654=VERTEX_POINT ( 'NONE', #1856 ) ;
#20655=ORIENTED_EDGE ( 'NONE', *, *, #49136, .F. ) ;
#20656=CARTESIAN_POINT ( 'NONE',  ( -6.695973446814940111, -1.750000000000024203, -79.18171244307201562 ) ) ;
#20668=EDGE_CURVE ( 'NONE', #41009, #13781, #26458, .T. ) ;
#20671=CARTESIAN_POINT ( 'NONE',  ( -208.4459734468149463, 0.000000000000000000, -40.93171244307202983 ) ) ;
#20675=CARTESIAN_POINT ( 'NONE',  ( -6.695973446814940111, 0.000000000000000000, 165.0000000000000000 ) ) ;
#20677=CARTESIAN_POINT ( 'NONE',  ( 210.0000000000000568, 2.143131898507881856E-16, -120.9317124430720582 ) ) ;
#20678=EDGE_CURVE ( 'NONE', #7390, #14002, #27839, .T. ) ;
#20687=CARTESIAN_POINT ( 'NONE',  ( 71.55402655318505367, -1.025126265847089213, -160.9317124430720014 ) ) ;
#20693=DIRECTION ( 'NONE',  ( 0.000000000000000000, 0.000000000000000000, 1.000000000000000000 ) ) ;
#20694=ORIENTED_EDGE ( 'NONE', *, *, #33211, .F. ) ;
#20696=ORIENTED_EDGE ( 'NONE', *, *, #22860, .T. ) ;
#20699=AXIS2_PLACEMENT_3D ( 'NONE', #14881, #50486, #38749 ) ;
#20705=ORIENTED_EDGE ( 'NONE', *, *, #7627, .T. ) ;
#20706=ORIENTED_EDGE ( 'NONE', *, *, #22593, .F. ) ;
#20713=ORIENTED_EDGE ( 'NONE', *, *, #39119, .F. ) ;
#20723=CARTESIAN_POINT ( 'NONE',  ( 35.05402655318504657, 2.143131898507880377E-16, -77.43171244307198720 ) ) ;
#20724=CARTESIAN_POINT ( 'NONE',  ( -4.945973446814903696, 2.143131898507912917E-16, -117.4317124430720156 ) ) ;
#20725=CARTESIAN_POINT ( 'NONE',  ( 73.30402655318508209, -1.750000000000010658, 120.8182875569279702 ) ) ;
#20732=DIRECTION ( 'NONE',  ( 0.000000000000000000, 0.000000000000000000, 1.000000000000000000 ) ) ;
#20743=LINE ( 'NONE', #36684, #14808 ) ;
#20744=ORIENTED_EDGE ( 'NONE', *, *, #31058, .F. ) ;
#20747=EDGE_LOOP ( 'NONE', ( #21966, #30444, #8573, #32350, #41610, #268 ) ) ;
#20751=ORIENTED_EDGE ( 'NONE', *, *, #42917, .T. ) ;
#20754=ORIENTED_EDGE ( 'NONE', *, *, #28681, .F. ) ;
#20760=CARTESIAN_POINT ( 'NONE',  ( -204.9459734468149463, 2.143131898507880377E-16, -77.43171244307204404 ) ) ;
#20769=CARTESIAN_POINT ( 'NONE',  ( 112.2789002873379758, 1.749999999999996669, -160.2068387089191219 ) ) ;
#20778=FACE_OUTER_BOUND ( 'NONE', #7795, .T. ) ;
#20783=DIRECTION ( 'NONE',  ( -1.000000000000000000, 0.000000000000000000, 0.000000000000000000 ) ) ;
#20785=CARTESIAN_POINT ( 'NONE',  ( 152.2789002873379900, 1.750000000000009548, 161.8434138227750907 ) ) ;
#20789=CARTESIAN_POINT ( 'NONE',  ( 35.05402655318504657, -1.025126265847089213, -160.9317124430720014 ) ) ;
#20791=ADVANCED_FACE ( 'NONE', ( #50007 ), #22349, .T. ) ;
#20793=CARTESIAN_POINT ( 'NONE',  ( 33.30402655318503946, 1.750000000000010214, -39.18171244307202983 ) ) ;
#20795=ORIENTED_EDGE ( 'NONE', *, *, #2101, .T. ) ;
#20797=EDGE_CURVE ( 'NONE', #28550, #29366, #6854, .T. ) ;
#20798=LINE ( 'NONE', #40068, #4011 ) ;
#20799=DIRECTION ( 'NONE',  ( 1.000000000000000000, 0.000000000000000000, 0.000000000000000000 ) ) ;
#20801=EDGE_CURVE ( 'NONE', #11997, #49578, #19280, .T. ) ;
#20802=DIRECTION ( 'NONE',  ( 0.000000000000000000, 0.000000000000000000, -1.000000000000000000 ) ) ;
#20805=CARTESIAN_POINT ( 'NONE',  ( 115.0540265531850395, 1.025126265847081886, -120.9317124430720440 ) ) ;
#20810=CARTESIAN_POINT ( 'NONE',  ( -206.6959734468149463, 1.750000000000010658, -119.1817124430720440 ) ) ;
#20813=CARTESIAN_POINT ( 'NONE',  ( 210.0000000000000568, 0.000000000000000000, 160.8182875569279702 ) ) ;
#20815=AXIS2_PLACEMENT_3D ( 'NONE', #4012, #19409, #43761 ) ;
#20817=EDGE_LOOP ( 'NONE', ( #19227, #25640, #28606, #33123, #15243, #49697 ) ) ;
#20818=DIRECTION ( 'NONE',  ( -1.000000000000000000, -0.000000000000000000, -0.000000000000000000 ) ) ;
#20820=CYLINDRICAL_SURFACE ( 'NONE', #22147, 1.750000000000015543 ) ;
#20825=EDGE_LOOP ( 'NONE', ( #12925, #42535, #12135, #31215, #46589, #45333 ) ) ;
#20827=EDGE_CURVE ( 'NONE', #33640, #7390, #31076, .T. ) ;
#20830=ORIENTED_EDGE ( 'NONE', *, *, #30899, .F. ) ;
#20833=AXIS2_PLACEMENT_3D ( 'NONE', #11188, #6061, #2218 ) ;
#20834=LINE ( 'NONE', #11885, #45261 ) ;
#20835=VERTEX_POINT ( 'NONE', #23624 ) ;
#20841=VECTOR ( 'NONE', #17926, 1000.000000000000000 ) ;
#20843=DIRECTION ( 'NONE',  ( -1.000000000000000000, -0.000000000000000000, -0.000000000000000000 ) ) ;
#20846=ORIENTED_EDGE ( 'NONE', *, *, #3635, .T. ) ;
#20848=ORIENTED_EDGE ( 'NONE', *, *, #12488, .F. ) ;
#20853=ADVANCED_FACE ( 'NONE', ( #31847 ), #39545, .T. ) ;
#20858=CARTESIAN_POINT ( 'NONE',  ( -166.6959734468149463, 1.750000000000010658, -119.1817124430720440 ) ) ;
#20863=( BOUNDED_CURVE ( )  B_SPLINE_CURVE ( 3, ( #3167, #45499, #22682, #7287 ),
 .UNSPECIFIED., .F., .F. ) 
 B_SPLINE_CURVE_WITH_KNOTS ( ( 4, 4 ),
 ( 3.141592653589793116, 4.712388980384689674 ),
 .UNSPECIFIED. ) 
 CURVE ( )  GEOMETRIC_REPRESENTATION_ITEM ( )  RATIONAL_B_SPLINE_CURVE ( ( 1.000000000000000000, 0.8047378541243649375, 0.8047378541243649375, 1.000000000000000000 ) ) 
 REPRESENTATION_ITEM ( '' )  );
#20865=CIRCLE ( 'NONE', #43893, 1.750000000000015543 ) ;
#20866=CARTESIAN_POINT ( 'NONE',  ( -128.4459734468149179, 0.000000000000000000, 79.06828755692799859 ) ) ;
#20867=ORIENTED_EDGE ( 'NONE', *, *, #38385, .F. ) ;
#20868=CARTESIAN_POINT ( 'NONE',  ( -46.69597344681494633, -1.750000000000009992, 0.8182875569279768335 ) ) ;
#20877=CARTESIAN_POINT ( 'NONE',  ( -86.69597344681494633, -1.750000000000009992, 0.8182875569279768335 ) ) ;
#20884=EDGE_CURVE ( 'NONE', #5777, #21583, #4892, .T. ) ;
#20886=FACE_OUTER_BOUND ( 'NONE', #36908, .T. ) ;
#20887=ORIENTED_EDGE ( 'NONE', *, *, #26455, .F. ) ;
#20895=EDGE_LOOP ( 'NONE', ( #26443, #23655, #18714, #25204, #27955 ) ) ;
#20897=CARTESIAN_POINT ( 'NONE',  ( -206.6959734468149463, -1.750000000000010658, 80.81828755692798438 ) ) ;
#20898=CARTESIAN_POINT ( 'NONE',  ( 75.05402655318509630, 2.143131898507880377E-16, -160.9317124430720582 ) ) ;
#20899=ORIENTED_EDGE ( 'NONE', *, *, #40874, .F. ) ;
#20902=ORIENTED_EDGE ( 'NONE', *, *, #32619, .F. ) ;
#20903=EDGE_CURVE ( 'NONE', #34748, #39727, #548, .T. ) ;
#20908=LINE ( 'NONE', #41607, #13956 ) ;
#20915=ORIENTED_EDGE ( 'NONE', *, *, #8552, .T. ) ;
#20917=ORIENTED_EDGE ( 'NONE', *, *, #10442, .T. ) ;
#20922=( BOUNDED_CURVE ( )  B_SPLINE_CURVE ( 3, ( #13842, #6412, #10510, #33133 ),
 .UNSPECIFIED., .F., .F. ) 
 B_SPLINE_CURVE_WITH_KNOTS ( ( 4, 4 ),
 ( 1.570796326794896558, 3.141592653589793116 ),
 .UNSPECIFIED. ) 
 CURVE ( )  GEOMETRIC_REPRESENTATION_ITEM ( )  RATIONAL_B_SPLINE_CURVE ( ( 1.000000000000000000, 0.8047378541243649375, 0.8047378541243649375, 1.000000000000000000 ) ) 
 REPRESENTATION_ITEM ( '' )  );
#20923=LINE ( 'NONE', #37102, #23789 ) ;
#20925=DIRECTION ( 'NONE',  ( 0.000000000000000000, 0.000000000000000000, 1.000000000000000000 ) ) ;
#20938=AXIS2_PLACEMENT_3D ( 'NONE', #37305, #22626, #37793 ) ;
#20939=( BOUNDED_CURVE ( )  B_SPLINE_CURVE ( 3, ( #18622, #38657, #19395, #163 ),
 .UNSPECIFIED., .F., .F. ) 
 B_SPLINE_CURVE_WITH_KNOTS ( ( 4, 4 ),
 ( 4.712388980384689674, 6.283185307179586232 ),
 .UNSPECIFIED. ) 
 CURVE ( )  GEOMETRIC_REPRESENTATION_ITEM ( )  RATIONAL_B_SPLINE_CURVE ( ( 1.000000000000000000, 0.8047378541243649375, 0.8047378541243649375, 1.000000000000000000 ) ) 
 REPRESENTATION_ITEM ( '' )  );
#20948=FACE_OUTER_BOUND ( 'NONE', #28598, .T. ) ;
#20953=ORIENTED_EDGE ( 'NONE', *, *, #48405, .F. ) ;
#20959=EDGE_CURVE ( 'NONE', #6771, #43286, #22882, .T. ) ;
#20960=ORIENTED_EDGE ( 'NONE', *, *, #32808, .F. ) ;
#20965=ADVANCED_FACE ( 'NONE', ( #22235 ), #45799, .T. ) ;
#20967=ORIENTED_EDGE ( 'NONE', *, *, #50436, .T. ) ;
#20973=VECTOR ( 'NONE', #7851, 1000.000000000000000 ) ;
#20980=VERTEX_POINT ( 'NONE', #40292 ) ;
#20984=ORIENTED_EDGE ( 'NONE', *, *, #50038, .T. ) ;
#20986=CARTESIAN_POINT ( 'NONE',  ( -5.670847180967843570, -1.750000000000023315, -0.2068387089191201234 ) ) ;
#20987=VECTOR ( 'NONE', #37644, 1000.000000000000000 ) ;
#20988=CARTESIAN_POINT ( 'NONE',  ( -45.67084718096785423, 1.750000000000009548, 41.84341382277508359 ) ) ;
#20992=CARTESIAN_POINT ( 'NONE',  ( -86.69597344681494633, 1.750000000000010658, -119.1817124430720440 ) ) ;
#20993=CARTESIAN_POINT ( 'NONE',  ( -206.6959734468149463, 1.750000000000009992, -159.1817124430720298 ) ) ;
#20994=LINE ( 'NONE', #24845, #1495 ) ;
#20995=VECTOR ( 'NONE', #30421, 1000.000000000000000 ) ;
#20999=CARTESIAN_POINT ( 'NONE',  ( -6.695973446814940111, 1.750000000000024203, -119.1817124430720440 ) ) ;
#21000=CARTESIAN_POINT ( 'NONE',  ( 210.0000000000000568, 2.143131898507880377E-16, 159.0682875569279702 ) ) ;
#21001=DIRECTION ( 'NONE',  ( -0.000000000000000000, -0.000000000000000000, -1.000000000000000000 ) ) ;
#21002=ADVANCED_FACE ( 'NONE', ( #20778 ), #36458, .T. ) ;
#21008=ORIENTED_EDGE ( 'NONE', *, *, #29580, .T. ) ;
#21012=CARTESIAN_POINT ( 'NONE',  ( -48.44597344681496054, 1.025126265847088991, 2.568287556927986159 ) ) ;
#21017=AXIS2_PLACEMENT_3D ( 'NONE', #49754, #14652, #30313 ) ;
#21020=CARTESIAN_POINT ( 'NONE',  ( -86.69597344681494633, 1.750000000000010658, 120.8182875569279702 ) ) ;
#21026=ORIENTED_EDGE ( 'NONE', *, *, #50584, .T. ) ;
#21028=DIRECTION ( 'NONE',  ( 0.000000000000000000, 0.000000000000000000, -1.000000000000000000 ) ) ;
#21029=ORIENTED_EDGE ( 'NONE', *, *, #39037, .F. ) ;
#21032=ORIENTED_EDGE ( 'NONE', *, *, #37452, .T. ) ;
#21033=APPLICATION_CONTEXT ( 'automotive_design' ) ;
#21034=ORIENTED_EDGE ( 'NONE', *, *, #14239, .F. ) ;
#21037=EDGE_CURVE ( 'NONE', #23031, #39985, #47422, .T. ) ;
#21039=ORIENTED_EDGE ( 'NONE', *, *, #25309, .T. ) ;
#21040=CARTESIAN_POINT ( 'NONE',  ( 153.3040265531850537, -1.750000000000009992, -159.1817124430720298 ) ) ;
#21045=FACE_OUTER_BOUND ( 'NONE', #29811, .T. ) ;
#21051=CARTESIAN_POINT ( 'NONE',  ( 33.30402655318503946, 0.000000000000000000, -165.0000000000000000 ) ) ;
#21057=DIRECTION ( 'NONE',  ( 0.000000000000000000, 0.000000000000000000, 1.000000000000000000 ) ) ;
#21060=ADVANCED_FACE ( 'NONE', ( #45050 ), #33543, .T. ) ;
#21062=CARTESIAN_POINT ( 'NONE',  ( -86.69597344681494633, -1.750000000000010658, 80.81828755692798438 ) ) ;
#21063=ORIENTED_EDGE ( 'NONE', *, *, #35359, .T. ) ;
#21072=EDGE_LOOP ( 'NONE', ( #5758, #15253, #25172, #30273, #47260, #7802 ) ) ;
#21075=CARTESIAN_POINT ( 'NONE',  ( -48.44597344681496054, -1.025126265847089435, -40.93171244307204404 ) ) ;
#21076=LINE ( 'NONE', #14125, #37009 ) ;
#21077=( BOUNDED_CURVE ( )  B_SPLINE_CURVE ( 3, ( #36504, #5173, #45149, #6192 ),
 .UNSPECIFIED., .F., .F. ) 
 B_SPLINE_CURVE_WITH_KNOTS ( ( 4, 4 ),
 ( 3.141592653589793116, 4.712388980384689674 ),
 .UNSPECIFIED. ) 
 CURVE ( )  GEOMETRIC_REPRESENTATION_ITEM ( )  RATIONAL_B_SPLINE_CURVE ( ( 1.000000000000000000, 0.8047378541243649375, 0.8047378541243649375, 1.000000000000000000 ) ) 
 REPRESENTATION_ITEM ( '' )  );
#21079=EDGE_LOOP ( 'NONE', ( #41563, #13299 ) ) ;
#21082=CYLINDRICAL_SURFACE ( 'NONE', #24286, 1.750000000000015543 ) ;
#21083=DIRECTION ( 'NONE',  ( -1.000000000000000000, -0.000000000000000000, -0.000000000000000000 ) ) ;
#21092=DIRECTION ( 'NONE',  ( 0.000000000000000000, 0.000000000000000000, 1.000000000000000000 ) ) ;
#21093=DIRECTION ( 'NONE',  ( -1.000000000000000000, 0.000000000000000000, 0.000000000000000000 ) ) ;
#21096=ORIENTED_EDGE ( 'NONE', *, *, #28205, .T. ) ;
#21100=EDGE_CURVE ( 'NONE', #14002, #9039, #20939, .T. ) ;
#21102=EDGE_CURVE ( 'NONE', #7456, #18807, #40278, .T. ) ;
#21104=ORIENTED_EDGE ( 'NONE', *, *, #39511, .T. ) ;
#21107=EDGE_CURVE ( 'NONE', #47806, #6245, #26484, .T. ) ;
#21111=AXIS2_PLACEMENT_3D ( 'NONE', #12650, #28058, #24724 ) ;
#21112=CYLINDRICAL_SURFACE ( 'NONE', #48727, 1.750000000000015543 ) ;
#21113=DIRECTION ( 'NONE',  ( -1.000000000000000000, 0.000000000000000000, 0.000000000000000000 ) ) ;
#21114=CARTESIAN_POINT ( 'NONE',  ( 32.27890028733795447, 1.750000000000009548, 81.84341382277507648 ) ) ;
#21116=CARTESIAN_POINT ( 'NONE',  ( 73.30402655318508209, 1.750000000000009992, 0.8182875569279768335 ) ) ;
#21117=CARTESIAN_POINT ( 'NONE',  ( 35.05402655318504657, 2.143131898507880377E-16, -40.93171244307205825 ) ) ;
#21119=ADVANCED_FACE ( 'NONE', ( #19650 ), #22735, .T. ) ;
#21126=ORIENTED_EDGE ( 'NONE', *, *, #29025, .T. ) ;
#21127=CARTESIAN_POINT ( 'NONE',  ( -5.670847180967843570, 1.750000000000023537, -78.15658617722490931 ) ) ;
#21128=CARTESIAN_POINT ( 'NONE',  ( 75.05402655318509630, 2.143131898507880377E-16, 2.568287556928006143 ) ) ;
#21139=EDGE_CURVE ( 'NONE', #4734, #24760, #38341, .T. ) ;
#21140=CYLINDRICAL_SURFACE ( 'NONE', #6240, 1.750000000000001554 ) ;
#21144=EDGE_CURVE ( 'NONE', #11740, #45663, #31749, .T. ) ;
#21148=CARTESIAN_POINT ( 'NONE',  ( -167.7210997126620384, 1.750000000000009548, 159.7931612910809065 ) ) ;
#21151=VERTEX_POINT ( 'NONE', #47815 ) ;
#21152=ORIENTED_EDGE ( 'NONE', *, *, #48039, .T. ) ;
#21158=ORIENTED_EDGE ( 'NONE', *, *, #32264, .T. ) ;
#21159=VERTEX_POINT ( 'NONE', #28113 ) ;
#21160=CARTESIAN_POINT ( 'NONE',  ( 34.32915281903212446, -1.750000000000009548, -0.2068387089191121020 ) ) ;
#21161=LINE ( 'NONE', #1674, #46970 ) ;
#21171=EDGE_CURVE ( 'NONE', #387, #40469, #24538, .T. ) ;
#21172=DIRECTION ( 'NONE',  ( 0.000000000000000000, 0.000000000000000000, 1.000000000000000000 ) ) ;
#21173=ORIENTED_EDGE ( 'NONE', *, *, #3266, .F. ) ;
#21175=CYLINDRICAL_SURFACE ( 'NONE', #35547, 1.750000000000001554 ) ;
#21178=ADVANCED_FACE ( 'NONE', ( #923 ), #44488, .T. ) ;
#21187=CARTESIAN_POINT ( 'NONE',  ( -124.9459734468149463, 2.143131898507847836E-16, 165.0000000000000000 ) ) ;
#21188=EDGE_CURVE ( 'NONE', #9702, #27396, #38634, .T. ) ;
#21190=DIRECTION ( 'NONE',  ( -1.000000000000000000, 0.000000000000000000, 0.000000000000000000 ) ) ;
#21192=DIRECTION ( 'NONE',  ( 0.000000000000000000, 0.000000000000000000, 1.000000000000000000 ) ) ;
#21194=FACE_OUTER_BOUND ( 'NONE', #13103, .T. ) ;
#21200=CYLINDRICAL_SURFACE ( 'NONE', #40229, 1.750000000000008438 ) ;
#21202=EDGE_CURVE ( 'NONE', #34395, #34063, #43859, .T. ) ;
#21203=CARTESIAN_POINT ( 'NONE',  ( -165.6708471809677974, 1.750000000000009548, -160.2068387089191219 ) ) ;
#21206=ORIENTED_EDGE ( 'NONE', *, *, #40246, .F. ) ;
#21207=CARTESIAN_POINT ( 'NONE',  ( 210.0000000000000568, 0.000000000000000000, 0.8182875569279768335 ) ) ;
#21209=FACE_OUTER_BOUND ( 'NONE', #40731, .T. ) ;
#21210=( BOUNDED_CURVE ( )  B_SPLINE_CURVE ( 3, ( #22258, #22001, #34317, #41247 ),
 .UNSPECIFIED., .F., .F. ) 
 B_SPLINE_CURVE_WITH_KNOTS ( ( 4, 4 ),
 ( 4.712388980384689674, 6.283185307179586232 ),
 .UNSPECIFIED. ) 
 CURVE ( )  GEOMETRIC_REPRESENTATION_ITEM ( )  RATIONAL_B_SPLINE_CURVE ( ( 1.000000000000000000, 0.8047378541243649375, 0.8047378541243649375, 1.000000000000000000 ) ) 
 REPRESENTATION_ITEM ( '' )  );
#21211=ORIENTED_EDGE ( 'NONE', *, *, #13583, .T. ) ;
#21213=CARTESIAN_POINT ( 'NONE',  ( 114.3291528190321173, -1.749999999999997113, 79.79316129108087807 ) ) ;
#21214=CARTESIAN_POINT ( 'NONE',  ( -84.94597344681493212, 1.025126265847089435, -40.93171244307204404 ) ) ;
#21215=CARTESIAN_POINT ( 'NONE',  ( -87.72109971266203843, -1.750000000000010214, -78.15658617722490931 ) ) ;
#21218=ORIENTED_EDGE ( 'NONE', *, *, #26130, .T. ) ;
#21219=CARTESIAN_POINT ( 'NONE',  ( -88.44597344681494633, 1.025126265847089657, 79.06828755692797017 ) ) ;
#21220=AXIS2_PLACEMENT_3D ( 'NONE', #15683, #35463, #15949 ) ;
#21222=EDGE_CURVE ( 'NONE', #27700, #4361, #29477, .T. ) ;
#21223=( BOUNDED_CURVE ( )  B_SPLINE_CURVE ( 3, ( #32376, #47974, #39838, #20062 ),
 .UNSPECIFIED., .F., .F. ) 
 B_SPLINE_CURVE_WITH_KNOTS ( ( 4, 4 ),
 ( 3.141592653589793116, 4.712388980384689674 ),
 .UNSPECIFIED. ) 
 CURVE ( )  GEOMETRIC_REPRESENTATION_ITEM ( )  RATIONAL_B_SPLINE_CURVE ( ( 1.000000000000000000, 0.8047378541243649375, 0.8047378541243649375, 1.000000000000000000 ) ) 
 REPRESENTATION_ITEM ( '' )  );
#21227=CARTESIAN_POINT ( 'NONE',  ( -44.94597344681493922, 2.143131898507880377E-16, 122.5682875569279702 ) ) ;
#21228=DIRECTION ( 'NONE',  ( 1.000000000000000000, 0.000000000000000000, 0.000000000000000000 ) ) ;
#21229=VECTOR ( 'NONE', #37867, 1000.000000000000000 ) ;
#21232=CARTESIAN_POINT ( 'NONE',  ( -204.9459734468148895, 1.025126265847089657, 42.56828755692799149 ) ) ;
#21234=CARTESIAN_POINT ( 'NONE',  ( -166.6959734468149463, 0.000000000000000000, 165.0000000000000000 ) ) ;
#21235=( BOUNDED_CURVE ( )  B_SPLINE_CURVE ( 3, ( #46119, #42314, #30784, #38994 ),
 .UNSPECIFIED., .F., .F. ) 
 B_SPLINE_CURVE_WITH_KNOTS ( ( 4, 4 ),
 ( 1.570796326794896558, 3.141592653589793116 ),
 .UNSPECIFIED. ) 
 CURVE ( )  GEOMETRIC_REPRESENTATION_ITEM ( )  RATIONAL_B_SPLINE_CURVE ( ( 1.000000000000000000, 0.8047378541243649375, 0.8047378541243649375, 1.000000000000000000 ) ) 
 REPRESENTATION_ITEM ( '' )  );
#21237=CARTESIAN_POINT ( 'NONE',  ( -4.945973446814917018, 1.025126265847097207, 2.568287556927999926 ) ) ;
#21239=EDGE_CURVE ( 'NONE', #10859, #14506, #43561, .T. ) ;
#21241=ORIENTED_EDGE ( 'NONE', *, *, #7513, .T. ) ;
#21242=CARTESIAN_POINT ( 'NONE',  ( -126.6959734468149321, 0.000000000000000000, 165.0000000000000000 ) ) ;
#21246=FACE_OUTER_BOUND ( 'NONE', #17485, .T. ) ;
#21247=EDGE_CURVE ( 'NONE', #4914, #39755, #49569, .T. ) ;
#21250=VERTEX_POINT ( 'NONE', #41421 ) ;
#21252=CIRCLE ( 'NONE', #49083, 1.750000000000001554 ) ;
#21257=CARTESIAN_POINT ( 'NONE',  ( -126.6959734468149321, 0.000000000000000000, 165.0000000000000000 ) ) ;
#21258=CARTESIAN_POINT ( 'NONE',  ( -46.69597344681494633, -1.750000000000010214, -39.18171244307202983 ) ) ;
#21262=VERTEX_POINT ( 'NONE', #29618 ) ;
#21264=FACE_OUTER_BOUND ( 'NONE', #15523, .T. ) ;
#21266=ORIENTED_EDGE ( 'NONE', *, *, #41129, .F. ) ;
#21271=CARTESIAN_POINT ( 'NONE',  ( -5.670847180967843570, -1.750000000000023315, -78.15658617722490931 ) ) ;
#21274=DIRECTION ( 'NONE',  ( 0.000000000000000000, 0.000000000000000000, 1.000000000000000000 ) ) ;
#21275=ORIENTED_EDGE ( 'NONE', *, *, #19228, .F. ) ;
#21276=CARTESIAN_POINT ( 'NONE',  ( -86.69597344681494633, 1.750000000000010214, -39.18171244307202983 ) ) ;
#21279=EDGE_LOOP ( 'NONE', ( #8144, #20454, #21096, #15674, #42355, #2072 ) ) ;
#21282=CARTESIAN_POINT ( 'NONE',  ( 210.0000000000000568, 0.000000000000000000, -79.18171244307201562 ) ) ;
#21304=VERTEX_POINT ( 'NONE', #29872 ) ;
#21305=CARTESIAN_POINT ( 'NONE',  ( 194.3291528190321742, -1.750000000000009548, 41.84341382277508359 ) ) ;
#21307=DIRECTION ( 'NONE',  ( -0.000000000000000000, -0.000000000000000000, -1.000000000000000000 ) ) ;
#21311=ADVANCED_FACE ( 'NONE', ( #48819 ), #9863, .T. ) ;
#21318=FACE_OUTER_BOUND ( 'NONE', #17627, .T. ) ;
#21320=CARTESIAN_POINT ( 'NONE',  ( -4.945973446814903696, 2.143131898507912917E-16, -80.93171244307204404 ) ) ;
#21325=CARTESIAN_POINT ( 'NONE',  ( -86.69597344681494633, -1.750000000000009992, 0.8182875569279768335 ) ) ;
#21327=DIRECTION ( 'NONE',  ( -1.000000000000000000, -0.000000000000000000, -0.000000000000000000 ) ) ;
#21329=LINE ( 'NONE', #37513, #30318 ) ;
#21334=ORIENTED_EDGE ( 'NONE', *, *, #40382, .F. ) ;
#21335=VERTEX_POINT ( 'NONE', #23449 ) ;
#21340=DIRECTION ( 'NONE',  ( -1.000000000000000000, 0.000000000000000000, 0.000000000000000000 ) ) ;
#21350=CARTESIAN_POINT ( 'NONE',  ( -168.4459734468149747, -1.025126265847089879, -117.4317124430720156 ) ) ;
#21358=DIRECTION ( 'NONE',  ( -1.000000000000000000, -0.000000000000000000, -0.000000000000000000 ) ) ;
#21361=DIRECTION ( 'NONE',  ( -1.000000000000000000, 0.000000000000000000, 0.000000000000000000 ) ) ;
#21362=LINE ( 'NONE', #10335, #2820 ) ;
#21374=FACE_OUTER_BOUND ( 'NONE', #10166, .T. ) ;
#21375=CARTESIAN_POINT ( 'NONE',  ( -206.6959734468149463, 0.000000000000000000, -165.0000000000000000 ) ) ;
#21376=( BOUNDED_CURVE ( )  B_SPLINE_CURVE ( 3, ( #5544, #21696, #25810, #9649 ),
 .UNSPECIFIED., .F., .F. ) 
 B_SPLINE_CURVE_WITH_KNOTS ( ( 4, 4 ),
 ( 3.141592653589793116, 4.712388980384689674 ),
 .UNSPECIFIED. ) 
 CURVE ( )  GEOMETRIC_REPRESENTATION_ITEM ( )  RATIONAL_B_SPLINE_CURVE ( ( 1.000000000000000000, 0.8047378541243649375, 0.8047378541243649375, 1.000000000000000000 ) ) 
 REPRESENTATION_ITEM ( '' )  );
#21383=CARTESIAN_POINT ( 'NONE',  ( -164.9459734468149463, -1.025126265847089435, 82.56828755692798438 ) ) ;
#21386=CARTESIAN_POINT ( 'NONE',  ( 152.2789002873379900, -1.750000000000010214, -118.1565861772249519 ) ) ;
#21388=CARTESIAN_POINT ( 'NONE',  ( -128.4459734468149179, 0.000000000000000000, -157.4317124430720582 ) ) ;
#21389=AXIS2_PLACEMENT_3D ( 'NONE', #9349, #20641, #32700 ) ;
#21393=CARTESIAN_POINT ( 'NONE',  ( -204.9459734468149463, 2.143131898507880377E-16, 79.06828755692797017 ) ) ;
#21394=CARTESIAN_POINT ( 'NONE',  ( 35.05402655318504657, 2.143131898507880377E-16, 159.0682875569279702 ) ) ;
#21407=CARTESIAN_POINT ( 'NONE',  ( -208.4459734468148611, 1.025126265847088991, -157.4317124430720582 ) ) ;
#21408=VERTEX_POINT ( 'NONE', #50588 ) ;
#21410=CARTESIAN_POINT ( 'NONE',  ( -168.4459734468149463, 0.000000000000000000, 165.0000000000000000 ) ) ;
#21411=CARTESIAN_POINT ( 'NONE',  ( -6.695973446814940111, 0.000000000000000000, 165.0000000000000000 ) ) ;
#21412=ORIENTED_EDGE ( 'NONE', *, *, #43149, .T. ) ;
#21415=CARTESIAN_POINT ( 'NONE',  ( 114.3291528190321173, -1.749999999999997113, -80.20683870891909351 ) ) ;
#21418=VERTEX_POINT ( 'NONE', #30905 ) ;
#21421=CARTESIAN_POINT ( 'NONE',  ( 210.0000000000000568, 0.000000000000000000, 120.8182875569279702 ) ) ;
#21425=DIRECTION ( 'NONE',  ( -0.000000000000000000, -0.000000000000000000, -1.000000000000000000 ) ) ;
#21426=CARTESIAN_POINT ( 'NONE',  ( 192.2789002873380184, -1.750000000000010214, -118.1565861772249519 ) ) ;
#21428=CARTESIAN_POINT ( 'NONE',  ( 33.30402655318503946, -1.750000000000010658, 120.8182875569279702 ) ) ;
#21433=EDGE_CURVE ( 'NONE', #48435, #42421, #3538, .T. ) ;
#21438=CARTESIAN_POINT ( 'NONE',  ( -8.445973446814976526, 0.000000000000000000, -117.4317124430720156 ) ) ;
#21440=CARTESIAN_POINT ( 'NONE',  ( 33.30402655318503946, 1.750000000000010214, 40.81828755692798438 ) ) ;
#21443=ORIENTED_EDGE ( 'NONE', *, *, #43046, .T. ) ;
#21449=( BOUNDED_CURVE ( )  B_SPLINE_CURVE ( 3, ( #1890, #45454, #24741, #5727 ),
 .UNSPECIFIED., .F., .F. ) 
 B_SPLINE_CURVE_WITH_KNOTS ( ( 4, 4 ),
 ( 1.570796326794896558, 3.141592653589793116 ),
 .UNSPECIFIED. ) 
 CURVE ( )  GEOMETRIC_REPRESENTATION_ITEM ( )  RATIONAL_B_SPLINE_CURVE ( ( 1.000000000000000000, 0.8047378541243649375, 0.8047378541243649375, 1.000000000000000000 ) ) 
 REPRESENTATION_ITEM ( '' )  );
#21455=DIRECTION ( 'NONE',  ( -1.000000000000000000, -0.000000000000000000, -0.000000000000000000 ) ) ;
#21456=CARTESIAN_POINT ( 'NONE',  ( -86.69597344681494633, -1.750000000000009992, 0.8182875569279768335 ) ) ;
#21460=EDGE_CURVE ( 'NONE', #7318, #24424, #26182, .T. ) ;
#21466=VERTEX_POINT ( 'NONE', #27557 ) ;
#21472=EDGE_LOOP ( 'NONE', ( #49867, #20522, #29845, #4125, #17579 ) ) ;
#21479=CARTESIAN_POINT ( 'NONE',  ( -48.44597344681495343, 0.000000000000000000, -0.9317124430720247208 ) ) ;
#21484=EDGE_CURVE ( 'NONE', #30864, #22009, #31440, .T. ) ;
#21487=ADVANCED_FACE ( 'NONE', ( #8810 ), #27799, .T. ) ;
#21489=CIRCLE ( 'NONE', #25603, 1.750000000000001554 ) ;
#21494=ORIENTED_EDGE ( 'NONE', *, *, #113, .F. ) ;
#21495=DIRECTION ( 'NONE',  ( -0.000000000000000000, -0.000000000000000000, -1.000000000000000000 ) ) ;
#21497=DIRECTION ( 'NONE',  ( -0.000000000000000000, -0.000000000000000000, -1.000000000000000000 ) ) ;
#21501=EDGE_CURVE ( 'NONE', #48877, #25305, #3237, .T. ) ;
#21506=EDGE_LOOP ( 'NONE', ( #40574, #191, #3848, #20795, #28641, #2804 ) ) ;
#21507=ORIENTED_EDGE ( 'NONE', *, *, #30899, .T. ) ;
#21509=( BOUNDED_CURVE ( )  B_SPLINE_CURVE ( 3, ( #17588, #2197, #41180, #2687 ),
 .UNSPECIFIED., .F., .F. ) 
 B_SPLINE_CURVE_WITH_KNOTS ( ( 4, 4 ),
 ( 1.570796326794896558, 3.141592653589793116 ),
 .UNSPECIFIED. ) 
 CURVE ( )  GEOMETRIC_REPRESENTATION_ITEM ( )  RATIONAL_B_SPLINE_CURVE ( ( 1.000000000000000000, 0.8047378541243649375, 0.8047378541243649375, 1.000000000000000000 ) ) 
 REPRESENTATION_ITEM ( '' )  );
#21512=CARTESIAN_POINT ( 'NONE',  ( -87.72109971266203843, 1.750000000000009548, 121.8434138227750623 ) ) ;
#21518=( BOUNDED_CURVE ( )  B_SPLINE_CURVE ( 3, ( #28583, #6256, #36308, #24751 ),
 .UNSPECIFIED., .F., .F. ) 
 B_SPLINE_CURVE_WITH_KNOTS ( ( 4, 4 ),
 ( 1.570796326794896558, 3.141592653589793116 ),
 .UNSPECIFIED. ) 
 CURVE ( )  GEOMETRIC_REPRESENTATION_ITEM ( )  RATIONAL_B_SPLINE_CURVE ( ( 1.000000000000000000, 0.8047378541243649375, 0.8047378541243649375, 1.000000000000000000 ) ) 
 REPRESENTATION_ITEM ( '' )  );
#21531=CARTESIAN_POINT ( 'NONE',  ( -6.695973446814940111, 1.750000000000023315, -159.1817124430720298 ) ) ;
#21536=FACE_OUTER_BOUND ( 'NONE', #6694, .T. ) ;
#21543=CARTESIAN_POINT ( 'NONE',  ( 75.05402655318509630, 2.143131898507880377E-16, 165.0000000000000000 ) ) ;
#21553=ORIENTED_EDGE ( 'NONE', *, *, #30935, .T. ) ;
#21555=DIRECTION ( 'NONE',  ( -1.000000000000000000, -0.000000000000000000, -0.000000000000000000 ) ) ;
#21558=DIRECTION ( 'NONE',  ( 1.000000000000000000, 0.000000000000000000, 0.000000000000000000 ) ) ;
#21565=CARTESIAN_POINT ( 'NONE',  ( -86.69597344681494633, 1.750000000000010658, 120.8182875569279702 ) ) ;
#21568=CARTESIAN_POINT ( 'NONE',  ( -164.9459734468149463, -1.025126265847089435, 162.5682875569279133 ) ) ;
#21575=DIRECTION ( 'NONE',  ( -1.000000000000000000, -0.000000000000000000, -0.000000000000000000 ) ) ;
#21576=CARTESIAN_POINT ( 'NONE',  ( -166.6959734468149463, 1.750000000000010658, -79.18171244307201562 ) ) ;
#21583=VERTEX_POINT ( 'NONE', #37296 ) ;
#21589=EDGE_CURVE ( 'NONE', #16313, #24770, #41916, .T. ) ;
#21593=DIRECTION ( 'NONE',  ( 0.000000000000000000, 0.000000000000000000, 1.000000000000000000 ) ) ;
#21594=EDGE_CURVE ( 'NONE', #48103, #41850, #12108, .T. ) ;
#21596=EDGE_CURVE ( 'NONE', #5763, #10383, #46520, .T. ) ;
#21597=CARTESIAN_POINT ( 'NONE',  ( -204.9459734468149463, 2.143131898507880377E-16, 42.56828755692798438 ) ) ;
#21599=ORIENTED_EDGE ( 'NONE', *, *, #16565, .F. ) ;
#21600=AXIS2_PLACEMENT_3D ( 'NONE', #10532, #14387, #31061 ) ;
#21614=DIRECTION ( 'NONE',  ( -1.000000000000000000, -0.000000000000000000, -0.000000000000000000 ) ) ;
#21616=DIRECTION ( 'NONE',  ( 1.000000000000000000, 0.000000000000000000, 0.000000000000000000 ) ) ;
#21619=ORIENTED_EDGE ( 'NONE', *, *, #10479, .T. ) ;
#21623=FACE_OUTER_BOUND ( 'NONE', #50629, .T. ) ;
#21624=VECTOR ( 'NONE', #31289, 1000.000000000000000 ) ;
#21629=CARTESIAN_POINT ( 'NONE',  ( 35.05402655318504657, 2.143131898507880377E-16, 165.0000000000000000 ) ) ;
#21636=AXIS2_PLACEMENT_3D ( 'NONE', #28971, #40527, #5615 ) ;
#21643=VERTEX_POINT ( 'NONE', #18246 ) ;
#21647=ORIENTED_EDGE ( 'NONE', *, *, #2406, .F. ) ;
#21649=CARTESIAN_POINT ( 'NONE',  ( 153.3040265531850537, 1.750000000000010658, -79.18171244307201562 ) ) ;
#21654=VERTEX_POINT ( 'NONE', #50521 ) ;
#21655=ORIENTED_EDGE ( 'NONE', *, *, #19614, .F. ) ;
#21657=( BOUNDED_CURVE ( )  B_SPLINE_CURVE ( 3, ( #24061, #4549, #20196, #35870 ),
 .UNSPECIFIED., .F., .F. ) 
 B_SPLINE_CURVE_WITH_KNOTS ( ( 4, 4 ),
 ( 4.712388980384689674, 6.283185307179586232 ),
 .UNSPECIFIED. ) 
 CURVE ( )  GEOMETRIC_REPRESENTATION_ITEM ( )  RATIONAL_B_SPLINE_CURVE ( ( 1.000000000000000000, 0.8047378541243649375, 0.8047378541243649375, 1.000000000000000000 ) ) 
 REPRESENTATION_ITEM ( '' )  );
#21658=LINE ( 'NONE', #48311, #13397 ) ;
#21659=VECTOR ( 'NONE', #35032, 1000.000000000000000 ) ;
#21663=CARTESIAN_POINT ( 'NONE',  ( -165.6708471809677974, -1.750000000000009548, -0.2068387089191121020 ) ) ;
#21668=DIRECTION ( 'NONE',  ( -0.000000000000000000, -0.000000000000000000, -1.000000000000000000 ) ) ;
#21670=CARTESIAN_POINT ( 'NONE',  ( -168.4459734468149463, 0.000000000000000000, 165.0000000000000000 ) ) ;
#21671=DIRECTION ( 'NONE',  ( -0.000000000000000000, -0.000000000000000000, -1.000000000000000000 ) ) ;
#21675=CARTESIAN_POINT ( 'NONE',  ( -166.6959734468149463, -1.750000000000010658, 80.81828755692798438 ) ) ;
#21676=ORIENTED_EDGE ( 'NONE', *, *, #40268, .T. ) ;
#21677=CARTESIAN_POINT ( 'NONE',  ( 193.3040265531851105, -1.750000000000009992, 160.8182875569279702 ) ) ;
#21678=CARTESIAN_POINT ( 'NONE',  ( 155.0540265531850537, 0.000000000000000000, 162.5682875569279702 ) ) ;
#21679=( BOUNDED_CURVE ( )  B_SPLINE_CURVE ( 3, ( #21440, #33016, #1706, #48601 ),
 .UNSPECIFIED., .F., .F. ) 
 B_SPLINE_CURVE_WITH_KNOTS ( ( 4, 4 ),
 ( 4.712388980384689674, 6.283185307179586232 ),
 .UNSPECIFIED. ) 
 CURVE ( )  GEOMETRIC_REPRESENTATION_ITEM ( )  RATIONAL_B_SPLINE_CURVE ( ( 1.000000000000000000, 0.8047378541243649375, 0.8047378541243649375, 1.000000000000000000 ) ) 
 REPRESENTATION_ITEM ( '' )  );
#21695=CARTESIAN_POINT ( 'NONE',  ( -204.9459734468149463, 2.143131898507880377E-16, -160.9317124430720014 ) ) ;
#21696=CARTESIAN_POINT ( 'NONE',  ( -44.94597344681493922, -1.025126265847089213, -37.43171244307202272 ) ) ;
#21701=CARTESIAN_POINT ( 'NONE',  ( -164.9459734468149463, 2.143131898507880377E-16, -120.9317124430720156 ) ) ;
#21704=CARTESIAN_POINT ( 'NONE',  ( -46.69597344681494633, 1.750000000000009992, 160.8182875569279702 ) ) ;
#21709=EDGE_LOOP ( 'NONE', ( #21126, #23371, #11943, #1926, #46747, #37337 ) ) ;
#21716=CARTESIAN_POINT ( 'NONE',  ( -84.94597344681494633, 2.143131898507880377E-16, -40.93171244307202983 ) ) ;
#21720=CARTESIAN_POINT ( 'NONE',  ( 193.3040265531851105, 0.000000000000000000, 165.0000000000000000 ) ) ;
#21726=CARTESIAN_POINT ( 'NONE',  ( 112.2789002873379758, -1.749999999999996669, 41.84341382277508359 ) ) ;
#21732=CARTESIAN_POINT ( 'NONE',  ( -168.4459734468149463, 0.000000000000000000, 165.0000000000000000 ) ) ;
#21737=DIRECTION ( 'NONE',  ( 0.000000000000000000, 0.000000000000000000, 1.000000000000000000 ) ) ;
#21753=CARTESIAN_POINT ( 'NONE',  ( 155.0540265531850537, 2.143131898507880377E-16, -120.9317124430720156 ) ) ;
#21755=ORIENTED_EDGE ( 'NONE', *, *, #15729, .F. ) ;
#21759=( BOUNDED_CURVE ( )  B_SPLINE_CURVE ( 3, ( #14637, #33900, #49493, #22837 ),
 .UNSPECIFIED., .F., .F. ) 
 B_SPLINE_CURVE_WITH_KNOTS ( ( 4, 4 ),
 ( 4.712388980384689674, 6.283185307179586232 ),
 .UNSPECIFIED. ) 
 CURVE ( )  GEOMETRIC_REPRESENTATION_ITEM ( )  RATIONAL_B_SPLINE_CURVE ( ( 1.000000000000000000, 0.8047378541243649375, 0.8047378541243649375, 1.000000000000000000 ) ) 
 REPRESENTATION_ITEM ( '' )  );
#21760=ORIENTED_EDGE ( 'NONE', *, *, #29292, .F. ) ;
#21763=CARTESIAN_POINT ( 'NONE',  ( 33.30402655318503946, 1.750000000000010214, -39.18171244307202983 ) ) ;
#21767=ORIENTED_EDGE ( 'NONE', *, *, #35566, .F. ) ;
#21768=ORIENTED_EDGE ( 'NONE', *, *, #36183, .F. ) ;
#21772=FACE_OUTER_BOUND ( 'NONE', #12188, .T. ) ;
#21774=ORIENTED_EDGE ( 'NONE', *, *, #9846, .T. ) ;
#21797=EDGE_CURVE ( 'NONE', #1049, #46904, #23631, .T. ) ;
#21798=AXIS2_PLACEMENT_3D ( 'NONE', #4240, #36059, #16291 ) ;
#21799=CARTESIAN_POINT ( 'NONE',  ( -124.9459734468149463, 2.143131898507847836E-16, -40.93171244307202983 ) ) ;
#21801=DIRECTION ( 'NONE',  ( 1.000000000000000000, 0.000000000000000000, -0.000000000000000000 ) ) ;
#21807=EDGE_CURVE ( 'NONE', #31511, #47298, #29754, .T. ) ;
#21816=AXIS2_PLACEMENT_3D ( 'NONE', #33798, #41985, #2726 ) ;
#21817=CARTESIAN_POINT ( 'NONE',  ( -164.9459734468149463, 2.143131898507880377E-16, -120.9317124430720156 ) ) ;
#21820=DIRECTION ( 'NONE',  ( -1.000000000000000000, -0.000000000000000000, -0.000000000000000000 ) ) ;
#21821=DIRECTION ( 'NONE',  ( -1.000000000000000000, -0.000000000000000000, -0.000000000000000000 ) ) ;
#21824=( BOUNDED_CURVE ( )  B_SPLINE_CURVE ( 3, ( #17051, #4492, #47805, #28596 ),
 .UNSPECIFIED., .F., .F. ) 
 B_SPLINE_CURVE_WITH_KNOTS ( ( 4, 4 ),
 ( 0.000000000000000000, 1.570796326794896558 ),
 .UNSPECIFIED. ) 
 CURVE ( )  GEOMETRIC_REPRESENTATION_ITEM ( )  RATIONAL_B_SPLINE_CURVE ( ( 1.000000000000000000, 0.8047378541243649375, 0.8047378541243649375, 1.000000000000000000 ) ) 
 REPRESENTATION_ITEM ( '' )  );
#21828=DIRECTION ( 'NONE',  ( -1.000000000000000000, -0.000000000000000000, -0.000000000000000000 ) ) ;
#21837=( BOUNDED_CURVE ( )  B_SPLINE_CURVE ( 3, ( #23494, #35311, #11679, #19629 ),
 .UNSPECIFIED., .F., .F. ) 
 B_SPLINE_CURVE_WITH_KNOTS ( ( 4, 4 ),
 ( 3.141592653589793116, 4.712388980384689674 ),
 .UNSPECIFIED. ) 
 CURVE ( )  GEOMETRIC_REPRESENTATION_ITEM ( )  RATIONAL_B_SPLINE_CURVE ( ( 1.000000000000000000, 0.8047378541243649375, 0.8047378541243649375, 1.000000000000000000 ) ) 
 REPRESENTATION_ITEM ( '' )  );
#21838=EDGE_CURVE ( 'NONE', #9213, #16293, #704, .T. ) ;
#21841=ORIENTED_EDGE ( 'NONE', *, *, #9545, .T. ) ;
#21845=ORIENTED_EDGE ( 'NONE', *, *, #39739, .T. ) ;
#21846=CARTESIAN_POINT ( 'NONE',  ( 195.0540265531851105, 1.025126265847088991, 162.5682875569279133 ) ) ;
#21847=DIRECTION ( 'NONE',  ( -1.000000000000000000, -0.000000000000000000, -0.000000000000000000 ) ) ;
#21852=ORIENTED_EDGE ( 'NONE', *, *, #26447, .T. ) ;
#21855=VECTOR ( 'NONE', #47618, 1000.000000000000000 ) ;
#21856=ADVANCED_FACE ( 'NONE', ( #17199 ), #10258, .T. ) ;
#21857=FACE_OUTER_BOUND ( 'NONE', #7449, .T. ) ;
#21861=CARTESIAN_POINT ( 'NONE',  ( -167.7210997126620384, -1.750000000000009548, -38.15658617722494483 ) ) ;
#21863=ORIENTED_EDGE ( 'NONE', *, *, #47288, .F. ) ;
#21864=CARTESIAN_POINT ( 'NONE',  ( 193.3040265531851105, 1.750000000000010658, -79.18171244307201562 ) ) ;
#21866=LINE ( 'NONE', #29808, #6926 ) ;
#21867=CARTESIAN_POINT ( 'NONE',  ( -126.6959734468149321, -1.749999999999996891, 160.8182875569279702 ) ) ;
#21879=CARTESIAN_POINT ( 'NONE',  ( 75.05402655318509630, -1.025126265847089213, -160.9317124430720014 ) ) ;
#21882=DIRECTION ( 'NONE',  ( -1.000000000000000000, -0.000000000000000000, -0.000000000000000000 ) ) ;
#21884=CARTESIAN_POINT ( 'NONE',  ( 33.30402655318503946, 1.750000000000010658, 80.81828755692798438 ) ) ;
#21888=CARTESIAN_POINT ( 'NONE',  ( -168.4459734468149747, -1.025126265847089879, -77.43171244307200141 ) ) ;
#21891=EDGE_CURVE ( 'NONE', #15960, #42459, #33615, .T. ) ;
#21895=ORIENTED_EDGE ( 'NONE', *, *, #18036, .T. ) ;
#21898=EDGE_CURVE ( 'NONE', #29622, #5743, #32867, .T. ) ;
#21900=ADVANCED_FACE ( 'NONE', ( #2054 ), #13828, .T. ) ;
#21901=EDGE_CURVE ( 'NONE', #5114, #7869, #48004, .T. ) ;
#21902=CYLINDRICAL_SURFACE ( 'NONE', #36105, 1.750000000000015543 ) ;
#21904=CARTESIAN_POINT ( 'NONE',  ( 71.55402655318505367, 0.000000000000000000, 165.0000000000000000 ) ) ;
#21919=EDGE_LOOP ( 'NONE', ( #49318, #46459, #27070, #41369, #1620, #41400 ) ) ;
#21929=ORIENTED_EDGE ( 'NONE', *, *, #47227, .T. ) ;
#21933=ORIENTED_EDGE ( 'NONE', *, *, #43046, .F. ) ;
#21934=CARTESIAN_POINT ( 'NONE',  ( -6.695973446814940111, 0.000000000000000000, 165.0000000000000000 ) ) ;
#21936=LINE ( 'NONE', #37601, #39252 ) ;
#21944=CARTESIAN_POINT ( 'NONE',  ( 153.3040265531850537, 0.000000000000000000, 165.0000000000000000 ) ) ;
#21949=EDGE_CURVE ( 'NONE', #829, #960, #7915, .T. ) ;
#21962=ORIENTED_EDGE ( 'NONE', *, *, #23738, .T. ) ;
#21965=VERTEX_POINT ( 'NONE', #22048 ) ;
#21966=ORIENTED_EDGE ( 'NONE', *, *, #50537, .F. ) ;
#21967=( BOUNDED_CURVE ( )  B_SPLINE_CURVE ( 3, ( #31796, #39746, #12035, #46385 ),
 .UNSPECIFIED., .F., .F. ) 
 B_SPLINE_CURVE_WITH_KNOTS ( ( 4, 4 ),
 ( 3.141592653589793116, 4.712388980384689674 ),
 .UNSPECIFIED. ) 
 CURVE ( )  GEOMETRIC_REPRESENTATION_ITEM ( )  RATIONAL_B_SPLINE_CURVE ( ( 1.000000000000000000, 0.8047378541243649375, 0.8047378541243649375, 1.000000000000000000 ) ) 
 REPRESENTATION_ITEM ( '' )  );
#21968=ORIENTED_EDGE ( 'NONE', *, *, #16489, .F. ) ;
#21971=LINE ( 'NONE', #22225, #35775 ) ;
#21975=CARTESIAN_POINT ( 'NONE',  ( -48.44597344681495343, 0.000000000000000000, -117.4317124430720156 ) ) ;
#21980=( BOUNDED_CURVE ( )  B_SPLINE_CURVE ( 3, ( #19769, #46679, #35949, #27977 ),
 .UNSPECIFIED., .F., .F. ) 
 B_SPLINE_CURVE_WITH_KNOTS ( ( 4, 4 ),
 ( 4.712388980384689674, 6.283185307179586232 ),
 .UNSPECIFIED. ) 
 CURVE ( )  GEOMETRIC_REPRESENTATION_ITEM ( )  RATIONAL_B_SPLINE_CURVE ( ( 1.000000000000000000, 0.8047378541243649375, 0.8047378541243649375, 1.000000000000000000 ) ) 
 REPRESENTATION_ITEM ( '' )  );
#21983=EDGE_CURVE ( 'NONE', #16166, #7390, #46384, .T. ) ;
#21985=CARTESIAN_POINT ( 'NONE',  ( -168.4459734468149463, 0.000000000000000000, 122.5682875569279702 ) ) ;
#21986=DIRECTION ( 'NONE',  ( -1.000000000000000000, -0.000000000000000000, -0.000000000000000000 ) ) ;
#21995=CARTESIAN_POINT ( 'NONE',  ( 111.5540265531850679, 0.000000000000000000, -120.9317124430720156 ) ) ;
#21997=CARTESIAN_POINT ( 'NONE',  ( 115.0540265531850395, -1.025126265847081664, 162.5682875569279133 ) ) ;
#22001=CARTESIAN_POINT ( 'NONE',  ( -5.670847180967843570, -1.750000000000023315, 39.79316129108089228 ) ) ;
#22002=ORIENTED_EDGE ( 'NONE', *, *, #11198, .T. ) ;
#22003=DIRECTION ( 'NONE',  ( -1.000000000000000000, -0.000000000000000000, -0.000000000000000000 ) ) ;
#22006=ADVANCED_FACE ( 'NONE', ( #4076 ), #30776, .T. ) ;
#22009=VERTEX_POINT ( 'NONE', #8184 ) ;
#22010=ORIENTED_EDGE ( 'NONE', *, *, #26455, .T. ) ;
#22011=ORIENTED_EDGE ( 'NONE', *, *, #21797, .F. ) ;
#22015=ORIENTED_EDGE ( 'NONE', *, *, #26230, .F. ) ;
#22018=( BOUNDED_CURVE ( )  B_SPLINE_CURVE ( 3, ( #8996, #16953, #44121, #13086 ),
 .UNSPECIFIED., .F., .F. ) 
 B_SPLINE_CURVE_WITH_KNOTS ( ( 4, 4 ),
 ( 0.000000000000000000, 1.570796326794896558 ),
 .UNSPECIFIED. ) 
 CURVE ( )  GEOMETRIC_REPRESENTATION_ITEM ( )  RATIONAL_B_SPLINE_CURVE ( ( 1.000000000000000000, 0.8047378541243649375, 0.8047378541243649375, 1.000000000000000000 ) ) 
 REPRESENTATION_ITEM ( '' )  );
#22026=CARTESIAN_POINT ( 'NONE',  ( 195.0540265531851105, 2.143131898507880377E-16, -120.9317124430720156 ) ) ;
#22029=ORIENTED_EDGE ( 'NONE', *, *, #31352, .T. ) ;
#22030=CARTESIAN_POINT ( 'NONE',  ( -8.445973446814976526, 0.000000000000000000, 79.06828755692795596 ) ) ;
#22032=VERTEX_POINT ( 'NONE', #15878 ) ;
#22036=DIRECTION ( 'NONE',  ( 0.000000000000000000, 0.000000000000000000, -1.000000000000000000 ) ) ;
#22041=CARTESIAN_POINT ( 'NONE',  ( 210.0000000000000568, 0.000000000000000000, -37.43171244307202272 ) ) ;
#22044=ADVANCED_FACE ( 'NONE', ( #23313 ), #36550, .T. ) ;
#22046=EDGE_LOOP ( 'NONE', ( #8286, #41329, #50055, #33486, #43529, #39350 ) ) ;
#22047=CARTESIAN_POINT ( 'NONE',  ( 35.05402655318504657, 2.143131898507880377E-16, -0.9317124430720247208 ) ) ;
#22048=CARTESIAN_POINT ( 'NONE',  ( 195.0540265531851105, 2.143131898507880377E-16, 2.568287556927978166 ) ) ;
#22052=CARTESIAN_POINT ( 'NONE',  ( 191.5540265531850537, -1.025126265847089435, -40.93171244307204404 ) ) ;
#22053=LINE ( 'NONE', #22306, #33981 ) ;
#22054=( BOUNDED_CURVE ( )  B_SPLINE_CURVE ( 3, ( #40673, #17563, #29116, #44737 ),
 .UNSPECIFIED., .F., .F. ) 
 B_SPLINE_CURVE_WITH_KNOTS ( ( 4, 4 ),
 ( 0.000000000000000000, 1.570796326794896558 ),
 .UNSPECIFIED. ) 
 CURVE ( )  GEOMETRIC_REPRESENTATION_ITEM ( )  RATIONAL_B_SPLINE_CURVE ( ( 1.000000000000000000, 0.8047378541243649375, 0.8047378541243649375, 1.000000000000000000 ) ) 
 REPRESENTATION_ITEM ( '' )  );
#22056=CARTESIAN_POINT ( 'NONE',  ( -124.9459734468149463, 2.143131898507847836E-16, -117.4317124430720725 ) ) ;
#22059=FACE_OUTER_BOUND ( 'NONE', #1110, .T. ) ;
#22066=ORIENTED_EDGE ( 'NONE', *, *, #8410, .T. ) ;
#22067=EDGE_CURVE ( 'NONE', #41009, #40604, #11524, .T. ) ;
#22068=LINE ( 'NONE', #28767, #40385 ) ;
#22071=CARTESIAN_POINT ( 'NONE',  ( 75.05402655318509630, -1.025126265847089435, -40.93171244307204404 ) ) ;
#22073=ORIENTED_EDGE ( 'NONE', *, *, #30216, .F. ) ;
#22076=CYLINDRICAL_SURFACE ( 'NONE', #24120, 1.750000000000015543 ) ;
#22078=CARTESIAN_POINT ( 'NONE',  ( 75.05402655318509630, 1.025126265847089657, 119.0682875569279560 ) ) ;
#22080=EDGE_CURVE ( 'NONE', #20319, #18505, #8441, .T. ) ;
#22091=AXIS2_PLACEMENT_3D ( 'NONE', #35687, #31060, #27711 ) ;
#22098=CARTESIAN_POINT ( 'NONE',  ( -6.695973446814940111, 1.750000000000024203, -119.1817124430720440 ) ) ;
#22100=CARTESIAN_POINT ( 'NONE',  ( 155.0540265531850537, 1.025126265847089657, -80.93171244307201562 ) ) ;
#22101=EDGE_CURVE ( 'NONE', #30683, #45850, #44878, .T. ) ;
#22103=EDGE_CURVE ( 'NONE', #33964, #21965, #4613, .T. ) ;
#22115=EDGE_CURVE ( 'NONE', #23986, #9366, #25584, .T. ) ;
#22120=DIRECTION ( 'NONE',  ( -1.000000000000000000, -0.000000000000000000, -0.000000000000000000 ) ) ;
#22121=( BOUNDED_CURVE ( )  B_SPLINE_CURVE ( 3, ( #23875, #8982, #43866, #39280 ),
 .UNSPECIFIED., .F., .F. ) 
 B_SPLINE_CURVE_WITH_KNOTS ( ( 4, 4 ),
 ( 3.141592653589793116, 4.712388980384689674 ),
 .UNSPECIFIED. ) 
 CURVE ( )  GEOMETRIC_REPRESENTATION_ITEM ( )  RATIONAL_B_SPLINE_CURVE ( ( 1.000000000000000000, 0.8047378541243649375, 0.8047378541243649375, 1.000000000000000000 ) ) 
 REPRESENTATION_ITEM ( '' )  );
#22129=( BOUNDED_CURVE ( )  B_SPLINE_CURVE ( 3, ( #19998, #21012, #28711, #27954 ),
 .UNSPECIFIED., .F., .F. ) 
 B_SPLINE_CURVE_WITH_KNOTS ( ( 4, 4 ),
 ( 3.141592653589793116, 4.712388980384689674 ),
 .UNSPECIFIED. ) 
 CURVE ( )  GEOMETRIC_REPRESENTATION_ITEM ( )  RATIONAL_B_SPLINE_CURVE ( ( 1.000000000000000000, 0.8047378541243649375, 0.8047378541243649375, 1.000000000000000000 ) ) 
 REPRESENTATION_ITEM ( '' )  );
#22130=CARTESIAN_POINT ( 'NONE',  ( 35.05402655318504657, -1.025126265847089435, -40.93171244307204404 ) ) ;
#22132=EDGE_CURVE ( 'NONE', #30495, #5180, #6259, .T. ) ;
#22139=DIRECTION ( 'NONE',  ( -0.000000000000000000, -0.000000000000000000, -1.000000000000000000 ) ) ;
#22143=DIRECTION ( 'NONE',  ( -0.000000000000000000, -0.000000000000000000, -1.000000000000000000 ) ) ;
#22145=CARTESIAN_POINT ( 'NONE',  ( -206.6959734468149463, -1.750000000000010658, -79.18171244307201562 ) ) ;
#22146=EDGE_LOOP ( 'NONE', ( #24913, #32768, #40911, #46587, #41195, #48445 ) ) ;
#22147=AXIS2_PLACEMENT_3D ( 'NONE', #25183, #40828, #1340 ) ;
#22149=ORIENTED_EDGE ( 'NONE', *, *, #24333, .F. ) ;
#22150=LINE ( 'NONE', #21904, #4157 ) ;
#22152=DIRECTION ( 'NONE',  ( -1.000000000000000000, -0.000000000000000000, -0.000000000000000000 ) ) ;
#22155=EDGE_LOOP ( 'NONE', ( #10011, #35193, #5244, #47555, #41050 ) ) ;
#22159=ORIENTED_EDGE ( 'NONE', *, *, #50266, .F. ) ;
#22161=CARTESIAN_POINT ( 'NONE',  ( 111.5540265531850537, -1.025126265847081886, 79.06828755692797017 ) ) ;
#22166=CARTESIAN_POINT ( 'NONE',  ( -128.4459734468149179, 0.000000000000000000, -37.43171244307205825 ) ) ;
#22176=CARTESIAN_POINT ( 'NONE',  ( 155.0540265531850537, 1.025126265847089213, -0.9317124430720324924 ) ) ;
#22179=FACE_OUTER_BOUND ( 'NONE', #10329, .T. ) ;
#22181=VERTEX_POINT ( 'NONE', #41998 ) ;
#22194=CARTESIAN_POINT ( 'NONE',  ( 72.27890028733797578, -1.750000000000009548, -40.20683870891912193 ) ) ;
#22205=ORIENTED_EDGE ( 'NONE', *, *, #21102, .F. ) ;
#22211=LINE ( 'NONE', #25554, #35685 ) ;
#22212=VERTEX_POINT ( 'NONE', #6344 ) ;
#22214=ORIENTED_EDGE ( 'NONE', *, *, #41930, .F. ) ;
#22218=CARTESIAN_POINT ( 'NONE',  ( 111.5540265531850679, 0.000000000000000000, 165.0000000000000000 ) ) ;
#22223=CARTESIAN_POINT ( 'NONE',  ( -204.9459734468148895, 1.025126265847089657, -37.43171244307202272 ) ) ;
#22225=CARTESIAN_POINT ( 'NONE',  ( 115.0540265531850395, 2.143131898507847836E-16, 165.0000000000000000 ) ) ;
#22230=DIRECTION ( 'NONE',  ( 0.000000000000000000, 0.000000000000000000, 1.000000000000000000 ) ) ;
#22232=ORIENTED_EDGE ( 'NONE', *, *, #24401, .F. ) ;
#22233=ORIENTED_EDGE ( 'NONE', *, *, #19676, .T. ) ;
#22235=FACE_OUTER_BOUND ( 'NONE', #1184, .T. ) ;
#22237=CARTESIAN_POINT ( 'NONE',  ( 153.3040265531850537, -1.750000000000010658, 120.8182875569279702 ) ) ;
#22238=ORIENTED_EDGE ( 'NONE', *, *, #6057, .T. ) ;
#22241=CARTESIAN_POINT ( 'NONE',  ( 191.5540265531850537, 1.025126265847089213, 42.56828755692799149 ) ) ;
#22242=EDGE_CURVE ( 'NONE', #17311, #22032, #7361, .T. ) ;
#22245=CARTESIAN_POINT ( 'NONE',  ( -46.69597344681494633, -1.750000000000009992, 160.8182875569279702 ) ) ;
#22247=CARTESIAN_POINT ( 'NONE',  ( 210.0000000000000568, 2.143131898507880377E-16, 159.0682875569279702 ) ) ;
#22248=EDGE_CURVE ( 'NONE', #46611, #23935, #41743, .T. ) ;
#22249=DIRECTION ( 'NONE',  ( -1.000000000000000000, -0.000000000000000000, -0.000000000000000000 ) ) ;
#22252=CARTESIAN_POINT ( 'NONE',  ( -168.4459734468149463, 0.000000000000000000, -0.9317124430720247208 ) ) ;
#22253=CARTESIAN_POINT ( 'NONE',  ( 111.5540265531850537, 1.025126265847081219, -157.4317124430720582 ) ) ;
#22258=CARTESIAN_POINT ( 'NONE',  ( -6.695973446814940111, -1.750000000000023759, 40.81828755692798438 ) ) ;
#22259=( BOUNDED_CURVE ( )  B_SPLINE_CURVE ( 3, ( #1584, #28528, #40824, #44154 ),
 .UNSPECIFIED., .F., .F. ) 
 B_SPLINE_CURVE_WITH_KNOTS ( ( 4, 4 ),
 ( 3.141592653589793116, 4.712388980384689674 ),
 .UNSPECIFIED. ) 
 CURVE ( )  GEOMETRIC_REPRESENTATION_ITEM ( )  RATIONAL_B_SPLINE_CURVE ( ( 1.000000000000000000, 0.8047378541243649375, 0.8047378541243649375, 1.000000000000000000 ) ) 
 REPRESENTATION_ITEM ( '' )  );
#22261=CARTESIAN_POINT ( 'NONE',  ( 111.5540265531850537, 1.025126265847081664, -77.43171244307201562 ) ) ;
#22262=CARTESIAN_POINT ( 'NONE',  ( 210.0000000000000568, 0.000000000000000000, 80.81828755692798438 ) ) ;
#22266=CARTESIAN_POINT ( 'NONE',  ( -128.4459734468149463, 1.025126265847081664, -77.43171244307201562 ) ) ;
#22268=( BOUNDED_CURVE ( )  B_SPLINE_CURVE ( 3, ( #40991, #1498, #8697, #9180 ),
 .UNSPECIFIED., .F., .F. ) 
 B_SPLINE_CURVE_WITH_KNOTS ( ( 4, 4 ),
 ( 3.141592653589793116, 4.712388980384689674 ),
 .UNSPECIFIED. ) 
 CURVE ( )  GEOMETRIC_REPRESENTATION_ITEM ( )  RATIONAL_B_SPLINE_CURVE ( ( 1.000000000000000000, 0.8047378541243649375, 0.8047378541243649375, 1.000000000000000000 ) ) 
 REPRESENTATION_ITEM ( '' )  );
#22269=VECTOR ( 'NONE', #39993, 1000.000000000000000 ) ;
#22270=ORIENTED_EDGE ( 'NONE', *, *, #17707, .T. ) ;
#22279=CARTESIAN_POINT ( 'NONE',  ( 154.3291528190321458, -1.750000000000010436, 79.79316129108087807 ) ) ;
#22280=DIRECTION ( 'NONE',  ( -1.000000000000000000, -0.000000000000000000, -0.000000000000000000 ) ) ;
#22281=( BOUNDED_CURVE ( )  B_SPLINE_CURVE ( 3, ( #2838, #22100, #30565, #10545 ),
 .UNSPECIFIED., .F., .F. ) 
 B_SPLINE_CURVE_WITH_KNOTS ( ( 4, 4 ),
 ( 0.000000000000000000, 1.570796326794896558 ),
 .UNSPECIFIED. ) 
 CURVE ( )  GEOMETRIC_REPRESENTATION_ITEM ( )  RATIONAL_B_SPLINE_CURVE ( ( 1.000000000000000000, 0.8047378541243649375, 0.8047378541243649375, 1.000000000000000000 ) ) 
 REPRESENTATION_ITEM ( '' )  );
#22284=DIRECTION ( 'NONE',  ( -1.000000000000000000, -0.000000000000000000, -0.000000000000000000 ) ) ;
#22287=LINE ( 'NONE', #34108, #27612 ) ;
#22288=LINE ( 'NONE', #23038, #31084 ) ;
#22290=ORIENTED_EDGE ( 'NONE', *, *, #50621, .T. ) ;
#22298=CARTESIAN_POINT ( 'NONE',  ( -127.7210997126620242, -1.749999999999996669, 41.84341382277508359 ) ) ;
#22299=ORIENTED_EDGE ( 'NONE', *, *, #8392, .F. ) ;
#22301=AXIS2_PLACEMENT_3D ( 'NONE', #29127, #44749, #5768 ) ;
#22306=CARTESIAN_POINT ( 'NONE',  ( 210.0000000000000568, 0.000000000000000000, 82.56828755692799859 ) ) ;
#22307=CIRCLE ( 'NONE', #6741, 1.750000000000008438 ) ;
#22314=CARTESIAN_POINT ( 'NONE',  ( 72.27890028733797578, 1.750000000000009548, 161.8434138227750907 ) ) ;
#22319=LINE ( 'NONE', #49727, #44203 ) ;
#22321=( BOUNDED_CURVE ( )  B_SPLINE_CURVE ( 3, ( #3365, #19011, #40553, #1558 ),
 .UNSPECIFIED., .F., .F. ) 
 B_SPLINE_CURVE_WITH_KNOTS ( ( 4, 4 ),
 ( 3.141592653589793116, 4.712388980384689674 ),
 .UNSPECIFIED. ) 
 CURVE ( )  GEOMETRIC_REPRESENTATION_ITEM ( )  RATIONAL_B_SPLINE_CURVE ( ( 1.000000000000000000, 0.8047378541243649375, 0.8047378541243649375, 1.000000000000000000 ) ) 
 REPRESENTATION_ITEM ( '' )  );
#22324=FACE_OUTER_BOUND ( 'NONE', #48618, .T. ) ;
#22330=CARTESIAN_POINT ( 'NONE',  ( 73.30402655318508209, -1.750000000000010214, -39.18171244307202983 ) ) ;
#22332=CARTESIAN_POINT ( 'NONE',  ( -44.94597344681493922, 2.143131898507880377E-16, 2.568287556927978166 ) ) ;
#22333=CARTESIAN_POINT ( 'NONE',  ( -87.72109971266203843, -1.750000000000010214, -118.1565861772249519 ) ) ;
#22334=CIRCLE ( 'NONE', #201, 1.750000000000008438 ) ;
#22336=ORIENTED_EDGE ( 'NONE', *, *, #37492, .T. ) ;
#22344=ORIENTED_EDGE ( 'NONE', *, *, #15529, .T. ) ;
#22346=DIRECTION ( 'NONE',  ( -1.000000000000000000, -0.000000000000000000, -0.000000000000000000 ) ) ;
#22349=CYLINDRICAL_SURFACE ( 'NONE', #4607, 1.750000000000015543 ) ;
#22355=( BOUNDED_CURVE ( )  B_SPLINE_CURVE ( 3, ( #16327, #8133, #20167, #35595 ),
 .UNSPECIFIED., .F., .F. ) 
 B_SPLINE_CURVE_WITH_KNOTS ( ( 4, 4 ),
 ( 4.712388980384689674, 6.283185307179586232 ),
 .UNSPECIFIED. ) 
 CURVE ( )  GEOMETRIC_REPRESENTATION_ITEM ( )  RATIONAL_B_SPLINE_CURVE ( ( 1.000000000000000000, 0.8047378541243649375, 0.8047378541243649375, 1.000000000000000000 ) ) 
 REPRESENTATION_ITEM ( '' )  );
#22356=ORIENTED_EDGE ( 'NONE', *, *, #40715, .F. ) ;
#22360=EDGE_CURVE ( 'NONE', #15143, #21583, #8212, .T. ) ;
#22364=CARTESIAN_POINT ( 'NONE',  ( -124.9459734468149463, 2.143131898507847836E-16, 159.0682875569279702 ) ) ;
#22367=DIRECTION ( 'NONE',  ( 0.000000000000000000, 0.000000000000000000, 1.000000000000000000 ) ) ;
#22372=CARTESIAN_POINT ( 'NONE',  ( 75.05402655318509630, -1.025126265847089435, 39.06828755692797728 ) ) ;
#22373=VECTOR ( 'NONE', #1253, 1000.000000000000000 ) ;
#22377=AXIS2_PLACEMENT_3D ( 'NONE', #48650, #24609, #40255 ) ;
#22379=VERTEX_POINT ( 'NONE', #40375 ) ;
#22385=EDGE_CURVE ( 'NONE', #33144, #3012, #47525, .T. ) ;
#22387=EDGE_CURVE ( 'NONE', #29044, #7807, #24979, .T. ) ;
#22390=EDGE_CURVE ( 'NONE', #42553, #23855, #14788, .T. ) ;
#22394=CARTESIAN_POINT ( 'NONE',  ( -164.9459734468149463, 2.143131898507880377E-16, 122.5682875569279702 ) ) ;
#22396=CARTESIAN_POINT ( 'NONE',  ( -4.945973446814938335, 0.000000000000000000, 162.5682875569279702 ) ) ;
#22397=ADVANCED_FACE ( 'NONE', ( #5462 ), #21112, .T. ) ;
#22405=FACE_OUTER_BOUND ( 'NONE', #13042, .T. ) ;
#22407=ORIENTED_EDGE ( 'NONE', *, *, #28379, .F. ) ;
#22409=ORIENTED_EDGE ( 'NONE', *, *, #21239, .F. ) ;
#22411=AXIS2_PLACEMENT_3D ( 'NONE', #8526, #27765, #36239 ) ;
#22413=( BOUNDED_CURVE ( )  B_SPLINE_CURVE ( 3, ( #44171, #24702, #23931, #40347 ),
 .UNSPECIFIED., .F., .F. ) 
 B_SPLINE_CURVE_WITH_KNOTS ( ( 4, 4 ),
 ( 4.712388980384689674, 6.283185307179586232 ),
 .UNSPECIFIED. ) 
 CURVE ( )  GEOMETRIC_REPRESENTATION_ITEM ( )  RATIONAL_B_SPLINE_CURVE ( ( 1.000000000000000000, 0.8047378541243649375, 0.8047378541243649375, 1.000000000000000000 ) ) 
 REPRESENTATION_ITEM ( '' )  );
#22417=ADVANCED_FACE ( 'NONE', ( #13901 ), #29072, .T. ) ;
#22419=ORIENTED_EDGE ( 'NONE', *, *, #5158, .F. ) ;
#22420=( BOUNDED_CURVE ( )  B_SPLINE_CURVE ( 3, ( #49337, #29888, #37864, #14490 ),
 .UNSPECIFIED., .F., .F. ) 
 B_SPLINE_CURVE_WITH_KNOTS ( ( 4, 4 ),
 ( 3.141592653589793116, 4.712388980384689674 ),
 .UNSPECIFIED. ) 
 CURVE ( )  GEOMETRIC_REPRESENTATION_ITEM ( )  RATIONAL_B_SPLINE_CURVE ( ( 1.000000000000000000, 0.8047378541243649375, 0.8047378541243649375, 1.000000000000000000 ) ) 
 REPRESENTATION_ITEM ( '' )  );
#22421=CARTESIAN_POINT ( 'NONE',  ( 154.3291528190321458, 1.750000000000009548, -0.2068387089191121020 ) ) ;
#22422=ORIENTED_EDGE ( 'NONE', *, *, #45901, .T. ) ;
#22425=EDGE_CURVE ( 'NONE', #24712, #28277, #25854, .T. ) ;
#22426=DIRECTION ( 'NONE',  ( -1.000000000000000000, 0.000000000000000000, 0.000000000000000000 ) ) ;
#22429=CARTESIAN_POINT ( 'NONE',  ( -168.4459734468149747, -1.025126265847089435, -40.93171244307204404 ) ) ;
#22438=CARTESIAN_POINT ( 'NONE',  ( 71.55402655318505367, 1.025126265847089213, -37.43171244307202272 ) ) ;
#22439=EDGE_CURVE ( 'NONE', #1904, #4802, #30088, .T. ) ;
#22442=VECTOR ( 'NONE', #25564, 1000.000000000000000 ) ;
#22452=ADVANCED_FACE ( 'NONE', ( #9572 ), #5964, .T. ) ;
#22453=CARTESIAN_POINT ( 'NONE',  ( -165.6708471809677974, -1.750000000000009548, 41.84341382277508359 ) ) ;
#22454=LINE ( 'NONE', #2207, #30277 ) ;
#22456=CARTESIAN_POINT ( 'NONE',  ( -8.445973446814964092, 1.025126265847097207, -40.93171244307204404 ) ) ;
#22457=ADVANCED_FACE ( 'NONE', ( #33686 ), #37049, .T. ) ;
#22465=AXIS2_PLACEMENT_3D ( 'NONE', #31739, #47327, #27880 ) ;
#22467=LINE ( 'NONE', #38140, #35266 ) ;
#22470=ORIENTED_EDGE ( 'NONE', *, *, #42843, .F. ) ;
#22471=ORIENTED_EDGE ( 'NONE', *, *, #24322, .F. ) ;
#22477=CARTESIAN_POINT ( 'NONE',  ( 210.0000000000000568, 0.000000000000000000, -79.18171244307201562 ) ) ;
#22478=ADVANCED_FACE ( 'NONE', ( #13668 ), #44934, .T. ) ;
#22482=ORIENTED_EDGE ( 'NONE', *, *, #30061, .F. ) ;
#22485=LINE ( 'NONE', #9926, #32427 ) ;
#22489=CARTESIAN_POINT ( 'NONE',  ( -4.945973446814903696, 2.143131898507912917E-16, -37.43171244307200141 ) ) ;
#22491=DIRECTION ( 'NONE',  ( 1.000000000000000000, 0.000000000000000000, 0.000000000000000000 ) ) ;
#22497=CARTESIAN_POINT ( 'NONE',  ( -124.9459734468149463, 2.143131898507847836E-16, -160.9317124430720014 ) ) ;
#22498=CARTESIAN_POINT ( 'NONE',  ( -48.44597344681495343, 0.000000000000000000, -80.93171244307204404 ) ) ;
#22499=CYLINDRICAL_SURFACE ( 'NONE', #29611, 1.750000000000015543 ) ;
#22500=CYLINDRICAL_SURFACE ( 'NONE', #49433, 1.750000000000036193 ) ;
#22507=EDGE_CURVE ( 'NONE', #42464, #29500, #27548, .T. ) ;
#22511=CARTESIAN_POINT ( 'NONE',  ( -47.72109971266203132, -1.750000000000009548, 39.79316129108089228 ) ) ;
#22513=CARTESIAN_POINT ( 'NONE',  ( 31.55402655318503236, 1.025126265847089213, -37.43171244307202272 ) ) ;
#22514=CYLINDRICAL_SURFACE ( 'NONE', #8638, 1.750000000000008438 ) ;
#22517=VERTEX_POINT ( 'NONE', #19273 ) ;
#22519=VECTOR ( 'NONE', #2671, 1000.000000000000000 ) ;
#22522=ADVANCED_FACE ( 'NONE', ( #50531 ), #10823, .T. ) ;
#22523=EDGE_LOOP ( 'NONE', ( #14618, #31493, #29084, #22214, #23981, #49138 ) ) ;
#22530=LINE ( 'NONE', #6131, #3471 ) ;
#22531=DIRECTION ( 'NONE',  ( -1.000000000000000000, 0.000000000000000000, 0.000000000000000000 ) ) ;
#22536=DIRECTION ( 'NONE',  ( -1.000000000000000000, -0.000000000000000000, -0.000000000000000000 ) ) ;
#22539=VECTOR ( 'NONE', #38502, 1000.000000000000000 ) ;
#22558=( BOUNDED_CURVE ( )  B_SPLINE_CURVE ( 3, ( #9768, #10031, #10782, #26432 ),
 .UNSPECIFIED., .F., .F. ) 
 B_SPLINE_CURVE_WITH_KNOTS ( ( 4, 4 ),
 ( 1.570796326794896558, 3.141592653589793116 ),
 .UNSPECIFIED. ) 
 CURVE ( )  GEOMETRIC_REPRESENTATION_ITEM ( )  RATIONAL_B_SPLINE_CURVE ( ( 1.000000000000000000, 0.8047378541243649375, 0.8047378541243649375, 1.000000000000000000 ) ) 
 REPRESENTATION_ITEM ( '' )  );
#22560=CARTESIAN_POINT ( 'NONE',  ( 111.5540265531850679, 0.000000000000000000, 2.568287556927950632 ) ) ;
#22563=CARTESIAN_POINT ( 'NONE',  ( -164.9459734468149463, 2.143131898507880377E-16, 119.0682875569279702 ) ) ;
#22570=AXIS2_PLACEMENT_3D ( 'NONE', #50563, #34733, #26761 ) ;
#22572=VERTEX_POINT ( 'NONE', #50021 ) ;
#22580=( BOUNDED_CURVE ( )  B_SPLINE_CURVE ( 3, ( #2656, #35013, #26525, #42159 ),
 .UNSPECIFIED., .F., .F. ) 
 B_SPLINE_CURVE_WITH_KNOTS ( ( 4, 4 ),
 ( 4.712388980384689674, 6.283185307179586232 ),
 .UNSPECIFIED. ) 
 CURVE ( )  GEOMETRIC_REPRESENTATION_ITEM ( )  RATIONAL_B_SPLINE_CURVE ( ( 1.000000000000000000, 0.8047378541243649375, 0.8047378541243649375, 1.000000000000000000 ) ) 
 REPRESENTATION_ITEM ( '' )  );
#22586=EDGE_LOOP ( 'NONE', ( #14814, #46692, #14962, #19364, #9615 ) ) ;
#22587=CARTESIAN_POINT ( 'NONE',  ( 72.27890028733797578, -1.750000000000009548, -38.15658617722494483 ) ) ;
#22593=EDGE_CURVE ( 'NONE', #44023, #25029, #36097, .T. ) ;
#22596=ORIENTED_EDGE ( 'NONE', *, *, #36676, .T. ) ;
#22598=CARTESIAN_POINT ( 'NONE',  ( -46.69597344681494633, 1.750000000000010658, -79.18171244307201562 ) ) ;
#22599=VECTOR ( 'NONE', #49887, 1000.000000000000000 ) ;
#22600=VECTOR ( 'NONE', #12185, 1000.000000000000000 ) ;
#22606=CARTESIAN_POINT ( 'NONE',  ( -5.670847180967843570, 1.750000000000023537, -120.2068387089191219 ) ) ;
#22623=CARTESIAN_POINT ( 'NONE',  ( -124.9459734468149321, -1.025126265847081219, 159.0682875569279418 ) ) ;
#22625=CARTESIAN_POINT ( 'NONE',  ( -45.67084718096785423, -1.750000000000009548, 161.8434138227750907 ) ) ;
#22626=DIRECTION ( 'NONE',  ( 0.000000000000000000, 0.000000000000000000, 1.000000000000000000 ) ) ;
#22628=CARTESIAN_POINT ( 'NONE',  ( -5.670847180967843570, -1.750000000000023315, -118.1565861772249519 ) ) ;
#22631=ORIENTED_EDGE ( 'NONE', *, *, #21139, .T. ) ;
#22643=AXIS2_PLACEMENT_3D ( 'NONE', #47933, #47428, #39788 ) ;
#22645=ORIENTED_EDGE ( 'NONE', *, *, #34837, .F. ) ;
#22649=CARTESIAN_POINT ( 'NONE',  ( -128.4459734468149179, 0.000000000000000000, 2.568287556927950632 ) ) ;
#22650=EDGE_CURVE ( 'NONE', #17310, #46387, #41316, .T. ) ;
#22652=ORIENTED_EDGE ( 'NONE', *, *, #41883, .T. ) ;
#22654=CARTESIAN_POINT ( 'NONE',  ( 33.30402655318503946, 1.750000000000009992, -159.1817124430720298 ) ) ;
#22655=ORIENTED_EDGE ( 'NONE', *, *, #10685, .F. ) ;
#22656=ORIENTED_EDGE ( 'NONE', *, *, #46155, .F. ) ;
#22658=CARTESIAN_POINT ( 'NONE',  ( -84.94597344681494633, 2.143131898507880377E-16, -120.9317124430720156 ) ) ;
#22668=ADVANCED_FACE ( 'NONE', ( #20295 ), #27497, .T. ) ;
#22669=CARTESIAN_POINT ( 'NONE',  ( 151.5540265531850537, 1.025126265847089657, -80.93171244307201562 ) ) ;
#22670=EDGE_LOOP ( 'NONE', ( #44428, #43360, #645, #9667, #46788 ) ) ;
#22677=EDGE_CURVE ( 'NONE', #9127, #38661, #24416, .T. ) ;
#22680=DIRECTION ( 'NONE',  ( -1.000000000000000000, -0.000000000000000000, -0.000000000000000000 ) ) ;
#22681=EDGE_LOOP ( 'NONE', ( #30374, #43216, #7185, #8366, #37584 ) ) ;
#22682=CARTESIAN_POINT ( 'NONE',  ( -207.7210997126620384, 1.750000000000009326, 1.843413822775066269 ) ) ;
#22689=CARTESIAN_POINT ( 'NONE',  ( -4.945973446814903696, 2.143131898507912917E-16, 79.06828755692795596 ) ) ;
#22693=DIRECTION ( 'NONE',  ( 0.000000000000000000, 0.000000000000000000, -1.000000000000000000 ) ) ;
#22699=LINE ( 'NONE', #42196, #32891 ) ;
#22703=EDGE_CURVE ( 'NONE', #5041, #47564, #18669, .T. ) ;
#22705=FACE_OUTER_BOUND ( 'NONE', #35387, .T. ) ;
#22707=ADVANCED_FACE ( 'NONE', ( #3277 ), #26644, .T. ) ;
#22710=DIRECTION ( 'NONE',  ( 0.000000000000000000, 0.000000000000000000, 1.000000000000000000 ) ) ;
#22712=EDGE_CURVE ( 'NONE', #25305, #41166, #1015, .T. ) ;
#22713=CARTESIAN_POINT ( 'NONE',  ( -164.9459734468149463, 2.143131898507880377E-16, 42.56828755692798438 ) ) ;
#22715=ORIENTED_EDGE ( 'NONE', *, *, #4611, .T. ) ;
#22719=DIRECTION ( 'NONE',  ( -0.000000000000000000, -0.000000000000000000, -1.000000000000000000 ) ) ;
#22720=ORIENTED_EDGE ( 'NONE', *, *, #20175, .T. ) ;
#22724=( BOUNDED_CURVE ( )  B_SPLINE_CURVE ( 3, ( #4714, #4456, #27568, #17012 ),
 .UNSPECIFIED., .F., .F. ) 
 B_SPLINE_CURVE_WITH_KNOTS ( ( 4, 4 ),
 ( 3.141592653589793116, 4.712388980384689674 ),
 .UNSPECIFIED. ) 
 CURVE ( )  GEOMETRIC_REPRESENTATION_ITEM ( )  RATIONAL_B_SPLINE_CURVE ( ( 1.000000000000000000, 0.8047378541243649375, 0.8047378541243649375, 1.000000000000000000 ) ) 
 REPRESENTATION_ITEM ( '' )  );
#22725=CARTESIAN_POINT ( 'NONE',  ( 74.32915281903215998, -1.750000000000010436, 119.7931612910808781 ) ) ;
#22727=DIRECTION ( 'NONE',  ( -0.000000000000000000, -0.000000000000000000, -1.000000000000000000 ) ) ;
#22730=CARTESIAN_POINT ( 'NONE',  ( -206.6959734468149463, 1.750000000000009992, 0.8182875569279768335 ) ) ;
#22734=CARTESIAN_POINT ( 'NONE',  ( 112.2789002873379758, 1.749999999999996669, 159.7931612910809065 ) ) ;
#22735=CYLINDRICAL_SURFACE ( 'NONE', #45550, 1.750000000000036193 ) ;
#22736=CARTESIAN_POINT ( 'NONE',  ( -48.44597344681495343, 0.000000000000000000, -40.93171244307205825 ) ) ;
#22743=FACE_OUTER_BOUND ( 'NONE', #11028, .T. ) ;
#22744=CARTESIAN_POINT ( 'NONE',  ( -207.7210997126620384, 1.750000000000010436, 79.79316129108087807 ) ) ;
#22749=EDGE_CURVE ( 'NONE', #50360, #30887, #9838, .T. ) ;
#22750=CARTESIAN_POINT ( 'NONE',  ( 210.0000000000000568, 2.143131898507880377E-16, -160.9317124430720298 ) ) ;
#22754=CYLINDRICAL_SURFACE ( 'NONE', #31276, 1.750000000000015543 ) ;
#22759=CARTESIAN_POINT ( 'NONE',  ( 193.3040265531851105, 0.000000000000000000, 165.0000000000000000 ) ) ;
#22762=CYLINDRICAL_SURFACE ( 'NONE', #24044, 1.750000000000001554 ) ;
#22766=CARTESIAN_POINT ( 'NONE',  ( -125.6708471809678542, -1.749999999999996669, -78.15658617722492352 ) ) ;
#22770=AXIS2_PLACEMENT_3D ( 'NONE', #41936, #21671, #6783 ) ;
#22772=CARTESIAN_POINT ( 'NONE',  ( 210.0000000000000568, 0.000000000000000000, 162.5682875569279702 ) ) ;
#22776=FACE_OUTER_BOUND ( 'NONE', #44665, .T. ) ;
#22777=ORIENTED_EDGE ( 'NONE', *, *, #7332, .F. ) ;
#22781=EDGE_CURVE ( 'NONE', #23545, #30427, #48773, .T. ) ;
#22785=CARTESIAN_POINT ( 'NONE',  ( 33.30402655318503946, 1.750000000000009992, 160.8182875569279702 ) ) ;
#22788=VECTOR ( 'NONE', #21614, 1000.000000000000000 ) ;
#22797=ORIENTED_EDGE ( 'NONE', *, *, #29580, .F. ) ;
#22802=CARTESIAN_POINT ( 'NONE',  ( 113.3040265531850537, 0.000000000000000000, 165.0000000000000000 ) ) ;
#22810=ORIENTED_EDGE ( 'NONE', *, *, #31994, .F. ) ;
#22819=CARTESIAN_POINT ( 'NONE',  ( 113.3040265531850537, 0.000000000000000000, 165.0000000000000000 ) ) ;
#22822=CARTESIAN_POINT ( 'NONE',  ( -127.7210997126620242, 1.749999999999996669, 121.8434138227750481 ) ) ;
#22829=EDGE_LOOP ( 'NONE', ( #20887, #30706, #1637, #841, #25781, #18270 ) ) ;
#22837=CARTESIAN_POINT ( 'NONE',  ( -164.9459734468149463, 2.143131898507880377E-16, 119.0682875569279702 ) ) ;
#22838=ORIENTED_EDGE ( 'NONE', *, *, #22242, .T. ) ;
#22841=DIRECTION ( 'NONE',  ( -1.000000000000000000, -0.000000000000000000, -0.000000000000000000 ) ) ;
#22846=CARTESIAN_POINT ( 'NONE',  ( 152.2789002873379900, 1.750000000000009326, 1.843413822775066269 ) ) ;
#22851=CARTESIAN_POINT ( 'NONE',  ( -44.94597344681493922, 2.143131898507880377E-16, -157.4317124430720014 ) ) ;
#22854=CARTESIAN_POINT ( 'NONE',  ( 193.3040265531851105, 1.750000000000009992, -159.1817124430720298 ) ) ;
#22857=( BOUNDED_CURVE ( )  B_SPLINE_CURVE ( 3, ( #26080, #2230, #2972, #33299 ),
 .UNSPECIFIED., .F., .F. ) 
 B_SPLINE_CURVE_WITH_KNOTS ( ( 4, 4 ),
 ( 4.712388980384689674, 6.283185307179586232 ),
 .UNSPECIFIED. ) 
 CURVE ( )  GEOMETRIC_REPRESENTATION_ITEM ( )  RATIONAL_B_SPLINE_CURVE ( ( 1.000000000000000000, 0.8047378541243649375, 0.8047378541243649375, 1.000000000000000000 ) ) 
 REPRESENTATION_ITEM ( '' )  );
#22859=AXIS2_PLACEMENT_3D ( 'NONE', #15441, #3637, #46953 ) ;
#22860=EDGE_CURVE ( 'NONE', #3579, #16946, #9979, .T. ) ;
#22863=CIRCLE ( 'NONE', #25329, 1.750000000000008438 ) ;
#22866=( BOUNDED_CURVE ( )  B_SPLINE_CURVE ( 3, ( #44833, #9203, #24863, #45332 ),
 .UNSPECIFIED., .F., .F. ) 
 B_SPLINE_CURVE_WITH_KNOTS ( ( 4, 4 ),
 ( 1.570796326794896558, 3.141592653589793116 ),
 .UNSPECIFIED. ) 
 CURVE ( )  GEOMETRIC_REPRESENTATION_ITEM ( )  RATIONAL_B_SPLINE_CURVE ( ( 1.000000000000000000, 0.8047378541243649375, 0.8047378541243649375, 1.000000000000000000 ) ) 
 REPRESENTATION_ITEM ( '' )  );
#22869=ORIENTED_EDGE ( 'NONE', *, *, #27580, .F. ) ;
#22876=CARTESIAN_POINT ( 'NONE',  ( -124.9459734468149321, 1.025126265847081664, -157.4317124430720582 ) ) ;
#22877=DIRECTION ( 'NONE',  ( -1.000000000000000000, -0.000000000000000000, -0.000000000000000000 ) ) ;
#22879=ORIENTED_EDGE ( 'NONE', *, *, #44782, .T. ) ;
#22882=( BOUNDED_CURVE ( )  B_SPLINE_CURVE ( 3, ( #18371, #41733, #28490, #10433 ),
 .UNSPECIFIED., .F., .F. ) 
 B_SPLINE_CURVE_WITH_KNOTS ( ( 4, 4 ),
 ( 4.712388980384689674, 6.283185307179586232 ),
 .UNSPECIFIED. ) 
 CURVE ( )  GEOMETRIC_REPRESENTATION_ITEM ( )  RATIONAL_B_SPLINE_CURVE ( ( 1.000000000000000000, 0.8047378541243649375, 0.8047378541243649375, 1.000000000000000000 ) ) 
 REPRESENTATION_ITEM ( '' )  );
#22887=CARTESIAN_POINT ( 'NONE',  ( 72.27890028733797578, -1.750000000000009548, 159.7931612910809065 ) ) ;
#22889=ORIENTED_EDGE ( 'NONE', *, *, #37456, .F. ) ;
#22890=CYLINDRICAL_SURFACE ( 'NONE', #14737, 1.750000000000001554 ) ;
#22892=CARTESIAN_POINT ( 'NONE',  ( 210.0000000000000568, 2.143131898507881116E-16, 39.06828755692797728 ) ) ;
#22893=EDGE_LOOP ( 'NONE', ( #1542, #49231, #19312, #4215, #3461, #27553 ) ) ;
#22897=CARTESIAN_POINT ( 'NONE',  ( 33.30402655318503946, 1.750000000000010214, -39.18171244307202983 ) ) ;
#22900=CARTESIAN_POINT ( 'NONE',  ( -46.69597344681494633, 1.750000000000009992, -159.1817124430720298 ) ) ;
#22906=DIRECTION ( 'NONE',  ( 0.000000000000000000, 0.000000000000000000, 1.000000000000000000 ) ) ;
#22908=EDGE_CURVE ( 'NONE', #40358, #3643, #36399, .T. ) ;
#22912=CARTESIAN_POINT ( 'NONE',  ( 73.30402655318508209, 1.750000000000009992, 0.8182875569279768335 ) ) ;
#22919=FACE_OUTER_BOUND ( 'NONE', #44894, .T. ) ;
#22920=CARTESIAN_POINT ( 'NONE',  ( -128.4459734468149179, 0.000000000000000000, 82.56828755692795596 ) ) ;
#22927=DIRECTION ( 'NONE',  ( -1.000000000000000000, 0.000000000000000000, 0.000000000000000000 ) ) ;
#22935=CARTESIAN_POINT ( 'NONE',  ( -46.69597344681494633, -1.750000000000010658, 80.81828755692798438 ) ) ;
#22937=CARTESIAN_POINT ( 'NONE',  ( 191.5540265531851105, 0.000000000000000000, -117.4317124430720725 ) ) ;
#22940=EDGE_CURVE ( 'NONE', #42417, #40803, #32500, .T. ) ;
#22942=CARTESIAN_POINT ( 'NONE',  ( -87.72109971266203843, -1.750000000000010214, -80.20683870891910772 ) ) ;
#22944=DIRECTION ( 'NONE',  ( -0.000000000000000000, -0.000000000000000000, -1.000000000000000000 ) ) ;
#22948=EDGE_LOOP ( 'NONE', ( #23664, #37455, #43542, #44373, #43295, #3843 ) ) ;
#22951=ORIENTED_EDGE ( 'NONE', *, *, #13132, .T. ) ;
#22955=EDGE_LOOP ( 'NONE', ( #31253, #30220, #37065, #19982, #30893, #40113 ) ) ;
#22956=ORIENTED_EDGE ( 'NONE', *, *, #19615, .T. ) ;
#22965=CYLINDRICAL_SURFACE ( 'NONE', #3752, 1.750000000000015543 ) ;
#22982=DIRECTION ( 'NONE',  ( 0.000000000000000000, 0.000000000000000000, 1.000000000000000000 ) ) ;
#22990=ORIENTED_EDGE ( 'NONE', *, *, #19742, .T. ) ;
#22996=VECTOR ( 'NONE', #25560, 1000.000000000000000 ) ;
#23007=CYLINDRICAL_SURFACE ( 'NONE', #29745, 1.750000000000015543 ) ;
#23009=ORIENTED_EDGE ( 'NONE', *, *, #15729, .T. ) ;
#23010=CARTESIAN_POINT ( 'NONE',  ( -208.4459734468149179, 2.143131898507880377E-16, -160.9317124430720298 ) ) ;
#23013=DIRECTION ( 'NONE',  ( -1.000000000000000000, -0.000000000000000000, -0.000000000000000000 ) ) ;
#23014=( BOUNDED_CURVE ( )  B_SPLINE_CURVE ( 3, ( #50509, #3602, #42348, #42848 ),
 .UNSPECIFIED., .F., .F. ) 
 B_SPLINE_CURVE_WITH_KNOTS ( ( 4, 4 ),
 ( 1.570796326794896558, 3.141592653589793116 ),
 .UNSPECIFIED. ) 
 CURVE ( )  GEOMETRIC_REPRESENTATION_ITEM ( )  RATIONAL_B_SPLINE_CURVE ( ( 1.000000000000000000, 0.8047378541243649375, 0.8047378541243649375, 1.000000000000000000 ) ) 
 REPRESENTATION_ITEM ( '' )  );
#23018=EDGE_CURVE ( 'NONE', #38997, #49549, #16110, .T. ) ;
#23024=ORIENTED_EDGE ( 'NONE', *, *, #6367, .T. ) ;
#23031=VERTEX_POINT ( 'NONE', #23814 ) ;
#23033=CARTESIAN_POINT ( 'NONE',  ( 33.30402655318503946, 0.000000000000000000, 165.0000000000000000 ) ) ;
#23037=CARTESIAN_POINT ( 'NONE',  ( -126.6959734468149321, -1.749999999999997335, -79.18171244307201562 ) ) ;
#23038=CARTESIAN_POINT ( 'NONE',  ( 210.0000000000000568, 0.000000000000000000, 42.56828755692799149 ) ) ;
#23040=ORIENTED_EDGE ( 'NONE', *, *, #45901, .F. ) ;
#23043=AXIS2_PLACEMENT_3D ( 'NONE', #26778, #7536, #3671 ) ;
#23047=ADVANCED_FACE ( 'NONE', ( #25075 ), #16612, .T. ) ;
#23049=CARTESIAN_POINT ( 'NONE',  ( 73.30402655318508209, 1.750000000000009992, 160.8182875569279702 ) ) ;
#23053=CARTESIAN_POINT ( 'NONE',  ( 152.2789002873379900, -1.750000000000010214, -78.15658617722490931 ) ) ;
#23055=CARTESIAN_POINT ( 'NONE',  ( 210.0000000000000568, 0.000000000000000000, 122.5682875569279844 ) ) ;
#23056=CARTESIAN_POINT ( 'NONE',  ( 32.27890028733795447, -1.750000000000010214, 119.7931612910808781 ) ) ;
#23057=CARTESIAN_POINT ( 'NONE',  ( 31.55402655318506788, 2.143131898507880377E-16, -160.9317124430720298 ) ) ;
#23059=ORIENTED_EDGE ( 'NONE', *, *, #45434, .T. ) ;
#23061=CARTESIAN_POINT ( 'NONE',  ( 210.0000000000000568, 2.143131898507881856E-16, -80.93171244307202983 ) ) ;
#23063=CARTESIAN_POINT ( 'NONE',  ( -204.9459734468149463, 2.143131898507880377E-16, 2.568287556927978166 ) ) ;
#23066=ADVANCED_FACE ( 'NONE', ( #21209 ), #40727, .T. ) ;
#23070=CARTESIAN_POINT ( 'NONE',  ( 33.30402655318503946, 1.750000000000010658, 80.81828755692798438 ) ) ;
#23071=CARTESIAN_POINT ( 'NONE',  ( 210.0000000000000568, 0.000000000000000000, -79.18171244307201562 ) ) ;
#23072=CARTESIAN_POINT ( 'NONE',  ( 71.55402655318505367, 1.025126265847088991, 2.568287556927986159 ) ) ;
#23078=EDGE_CURVE ( 'NONE', #42417, #40485, #9161, .T. ) ;
#23084=CARTESIAN_POINT ( 'NONE',  ( 210.0000000000000568, 0.000000000000000000, 120.8182875569279702 ) ) ;
#23085=ORIENTED_EDGE ( 'NONE', *, *, #40032, .F. ) ;
#23086=ADVANCED_FACE ( 'NONE', ( #1480 ), #36903, .T. ) ;
#23104=( BOUNDED_CURVE ( )  B_SPLINE_CURVE ( 3, ( #49688, #3276, #14580, #30237 ),
 .UNSPECIFIED., .F., .F. ) 
 B_SPLINE_CURVE_WITH_KNOTS ( ( 4, 4 ),
 ( 1.570796326794896558, 3.141592653589793116 ),
 .UNSPECIFIED. ) 
 CURVE ( )  GEOMETRIC_REPRESENTATION_ITEM ( )  RATIONAL_B_SPLINE_CURVE ( ( 1.000000000000000000, 0.8047378541243649375, 0.8047378541243649375, 1.000000000000000000 ) ) 
 REPRESENTATION_ITEM ( '' )  );
#23111=AXIS2_PLACEMENT_3D ( 'NONE', #37615, #18326, #9638 ) ;
#23112=CARTESIAN_POINT ( 'NONE',  ( -124.9459734468149463, 2.143131898507847836E-16, -117.4317124430720725 ) ) ;
#23113=FACE_OUTER_BOUND ( 'NONE', #1850, .T. ) ;
#23114=LINE ( 'NONE', #38787, #46712 ) ;
#23118=ORIENTED_EDGE ( 'NONE', *, *, #10249, .F. ) ;
#23125=CARTESIAN_POINT ( 'NONE',  ( -207.7210997126620384, 1.750000000000010436, -80.20683870891910772 ) ) ;
#23132=DIRECTION ( 'NONE',  ( -0.000000000000000000, -0.000000000000000000, -1.000000000000000000 ) ) ;
#23134=ORIENTED_EDGE ( 'NONE', *, *, #16785, .F. ) ;
#23135=CARTESIAN_POINT ( 'NONE',  ( 113.3040265531850537, 1.749999999999996891, -159.1817124430720298 ) ) ;
#23136=AXIS2_PLACEMENT_3D ( 'NONE', #16623, #32293, #12774 ) ;
#23139=CARTESIAN_POINT ( 'NONE',  ( 210.0000000000000568, 0.000000000000000000, -39.18171244307202983 ) ) ;
#23142=CARTESIAN_POINT ( 'NONE',  ( 113.3040265531850537, 1.749999999999996891, 0.8182875569279768335 ) ) ;
#23145=VECTOR ( 'NONE', #21828, 1000.000000000000000 ) ;
#23146=EDGE_CURVE ( 'NONE', #48817, #11294, #44045, .T. ) ;
#23152=CARTESIAN_POINT ( 'NONE',  ( -8.445973446814962315, 1.025126265847096985, -0.9317124430720461481 ) ) ;
#23154=DIRECTION ( 'NONE',  ( 0.000000000000000000, 0.000000000000000000, 1.000000000000000000 ) ) ;
#23156=ADVANCED_FACE ( 'NONE', ( #6067 ), #17615, .T. ) ;
#23161=EDGE_CURVE ( 'NONE', #5437, #3794, #49377, .T. ) ;
#23162=( BOUNDED_CURVE ( )  B_SPLINE_CURVE ( 3, ( #41951, #25800, #49839, #26558 ),
 .UNSPECIFIED., .F., .F. ) 
 B_SPLINE_CURVE_WITH_KNOTS ( ( 4, 4 ),
 ( 3.141592653589793116, 4.712388980384689674 ),
 .UNSPECIFIED. ) 
 CURVE ( )  GEOMETRIC_REPRESENTATION_ITEM ( )  RATIONAL_B_SPLINE_CURVE ( ( 1.000000000000000000, 0.8047378541243649375, 0.8047378541243649375, 1.000000000000000000 ) ) 
 REPRESENTATION_ITEM ( '' )  );
#23165=CARTESIAN_POINT ( 'NONE',  ( 210.0000000000000568, 2.143131898507881856E-16, 79.06828755692797017 ) ) ;
#23167=DIRECTION ( 'NONE',  ( -0.000000000000000000, -0.000000000000000000, -1.000000000000000000 ) ) ;
#23172=( BOUNDED_CURVE ( )  B_SPLINE_CURVE ( 3, ( #26741, #33936, #15189, #38557 ),
 .UNSPECIFIED., .F., .F. ) 
 B_SPLINE_CURVE_WITH_KNOTS ( ( 4, 4 ),
 ( 0.000000000000000000, 1.570796326794896558 ),
 .UNSPECIFIED. ) 
 CURVE ( )  GEOMETRIC_REPRESENTATION_ITEM ( )  RATIONAL_B_SPLINE_CURVE ( ( 1.000000000000000000, 0.8047378541243649375, 0.8047378541243649375, 1.000000000000000000 ) ) 
 REPRESENTATION_ITEM ( '' )  );
#23179=EDGE_LOOP ( 'NONE', ( #527, #46535, #47306, #1081, #4131, #26572 ) ) ;
#23185=CARTESIAN_POINT ( 'NONE',  ( -86.69597344681494633, -1.750000000000010214, 40.81828755692798438 ) ) ;
#23190=DIRECTION ( 'NONE',  ( -1.000000000000000000, -0.000000000000000000, -0.000000000000000000 ) ) ;
#23192=FACE_OUTER_BOUND ( 'NONE', #39928, .T. ) ;
#23193=ORIENTED_EDGE ( 'NONE', *, *, #1519, .F. ) ;
#23200=CARTESIAN_POINT ( 'NONE',  ( 32.27890028733795447, -1.750000000000009548, -40.20683870891912193 ) ) ;
#23201=EDGE_CURVE ( 'NONE', #42197, #43746, #40657, .T. ) ;
#23212=ORIENTED_EDGE ( 'NONE', *, *, #40939, .T. ) ;
#23213=DIRECTION ( 'NONE',  ( -1.000000000000000000, 0.000000000000000000, 0.000000000000000000 ) ) ;
#23218=ORIENTED_EDGE ( 'NONE', *, *, #11835, .T. ) ;
#23223=ORIENTED_EDGE ( 'NONE', *, *, #22360, .F. ) ;
#23228=EDGE_LOOP ( 'NONE', ( #35642, #2958, #19510, #27205, #43533, #16807 ) ) ;
#23229=VECTOR ( 'NONE', #41160, 1000.000000000000000 ) ;
#23232=ORIENTED_EDGE ( 'NONE', *, *, #20481, .T. ) ;
#23234=CARTESIAN_POINT ( 'NONE',  ( -6.695973446814940111, 0.000000000000000000, 165.0000000000000000 ) ) ;
#23236=CARTESIAN_POINT ( 'NONE',  ( 191.5540265531851105, 0.000000000000000000, -117.4317124430720725 ) ) ;
#23238=ORIENTED_EDGE ( 'NONE', *, *, #48813, .T. ) ;
#23243=CYLINDRICAL_SURFACE ( 'NONE', #34235, 1.750000000000001554 ) ;
#23247=ORIENTED_EDGE ( 'NONE', *, *, #24617, .T. ) ;
#23249=CARTESIAN_POINT ( 'NONE',  ( 193.3040265531851105, -1.750000000000009992, -159.1817124430720298 ) ) ;
#23250=CARTESIAN_POINT ( 'NONE',  ( -6.695973446814940111, 1.750000000000023759, 40.81828755692798438 ) ) ;
#23255=FACE_OUTER_BOUND ( 'NONE', #48985, .T. ) ;
#23260=ORIENTED_EDGE ( 'NONE', *, *, #31803, .T. ) ;
#23263=DIRECTION ( 'NONE',  ( 1.000000000000000000, 0.000000000000000000, 0.000000000000000000 ) ) ;
#23265=CARTESIAN_POINT ( 'NONE',  ( -86.69597344681494633, -1.750000000000010658, -79.18171244307201562 ) ) ;
#23268=CARTESIAN_POINT ( 'NONE',  ( -44.94597344681493922, 2.143131898507880377E-16, 122.5682875569279702 ) ) ;
#23270=FACE_OUTER_BOUND ( 'NONE', #37691, .T. ) ;
#23271=VERTEX_POINT ( 'NONE', #41723 ) ;
#23273=CARTESIAN_POINT ( 'NONE',  ( -88.44597344681497475, 0.000000000000000000, -40.93171244307205825 ) ) ;
#23274=ORIENTED_EDGE ( 'NONE', *, *, #7416, .F. ) ;
#23285=EDGE_CURVE ( 'NONE', #40502, #40611, #49126, .T. ) ;
#23288=EDGE_CURVE ( 'NONE', #47457, #32283, #21971, .T. ) ;
#23289=CARTESIAN_POINT ( 'NONE',  ( -208.4459734468149463, 0.000000000000000000, 79.06828755692797017 ) ) ;
#23292=CYLINDRICAL_SURFACE ( 'NONE', #39293, 1.750000000000036193 ) ;
#23297=EDGE_CURVE ( 'NONE', #15732, #20063, #28883, .T. ) ;
#23301=ORIENTED_EDGE ( 'NONE', *, *, #25881, .F. ) ;
#23305=( BOUNDED_CURVE ( )  B_SPLINE_CURVE ( 3, ( #27813, #43448, #50600, #15747 ),
 .UNSPECIFIED., .F., .F. ) 
 B_SPLINE_CURVE_WITH_KNOTS ( ( 4, 4 ),
 ( 1.570796326794896558, 3.141592653589793116 ),
 .UNSPECIFIED. ) 
 CURVE ( )  GEOMETRIC_REPRESENTATION_ITEM ( )  RATIONAL_B_SPLINE_CURVE ( ( 1.000000000000000000, 0.8047378541243649375, 0.8047378541243649375, 1.000000000000000000 ) ) 
 REPRESENTATION_ITEM ( '' )  );
#23308=CARTESIAN_POINT ( 'NONE',  ( -128.4459734468149179, 0.000000000000000000, -157.4317124430720582 ) ) ;
#23309=CARTESIAN_POINT ( 'NONE',  ( 210.0000000000000568, 0.000000000000000000, 160.8182875569279702 ) ) ;
#23313=FACE_OUTER_BOUND ( 'NONE', #18183, .T. ) ;
#23314=CARTESIAN_POINT ( 'NONE',  ( 31.55402655318503236, -1.025126265847089213, -160.9317124430720014 ) ) ;
#23315=CARTESIAN_POINT ( 'NONE',  ( -168.4459734468149463, 0.000000000000000000, 119.0682875569279702 ) ) ;
#23318=VERTEX_POINT ( 'NONE', #1103 ) ;
#23319=CARTESIAN_POINT ( 'NONE',  ( -8.445973446814964092, 1.025126265847097207, 82.56828755692798438 ) ) ;
#23320=DIRECTION ( 'NONE',  ( -1.000000000000000000, -0.000000000000000000, -0.000000000000000000 ) ) ;
#23324=CARTESIAN_POINT ( 'NONE',  ( -128.4459734468149179, 0.000000000000000000, -120.9317124430720156 ) ) ;
#23329=( BOUNDED_CURVE ( )  B_SPLINE_CURVE ( 3, ( #956, #16853, #5033, #32754 ),
 .UNSPECIFIED., .F., .F. ) 
 B_SPLINE_CURVE_WITH_KNOTS ( ( 4, 4 ),
 ( 3.141592653589793116, 4.712388980384689674 ),
 .UNSPECIFIED. ) 
 CURVE ( )  GEOMETRIC_REPRESENTATION_ITEM ( )  RATIONAL_B_SPLINE_CURVE ( ( 1.000000000000000000, 0.8047378541243649375, 0.8047378541243649375, 1.000000000000000000 ) ) 
 REPRESENTATION_ITEM ( '' )  );
#23331=CARTESIAN_POINT ( 'NONE',  ( 191.5540265531851105, 0.000000000000000000, 165.0000000000000000 ) ) ;
#23332=VECTOR ( 'NONE', #9929, 1000.000000000000000 ) ;
#23333=CARTESIAN_POINT ( 'NONE',  ( 152.2789002873379900, -1.750000000000009548, 161.8434138227750907 ) ) ;
#23334=ORIENTED_EDGE ( 'NONE', *, *, #49905, .F. ) ;
#23337=EDGE_LOOP ( 'NONE', ( #7978, #19240, #44588, #13515, #47528, #18239 ) ) ;
#23342=ADVANCED_FACE ( 'NONE', ( #36263 ), #8804, .T. ) ;
#23344=AXIS2_PLACEMENT_3D ( 'NONE', #40765, #34088, #18408 ) ;
#23345=EDGE_CURVE ( 'NONE', #16751, #5777, #50124, .T. ) ;
#23360=EDGE_CURVE ( 'NONE', #4790, #30864, #15089, .T. ) ;
#23364=DIRECTION ( 'NONE',  ( 1.000000000000000000, 0.000000000000000000, 0.000000000000000000 ) ) ;
#23365=VECTOR ( 'NONE', #30508, 1000.000000000000000 ) ;
#23371=ORIENTED_EDGE ( 'NONE', *, *, #36689, .T. ) ;
#23373=CARTESIAN_POINT ( 'NONE',  ( 210.0000000000000568, 0.000000000000000000, 120.8182875569279702 ) ) ;
#23376=CARTESIAN_POINT ( 'NONE',  ( 71.55402655318505367, 0.000000000000000000, -120.9317124430720725 ) ) ;
#23378=EDGE_CURVE ( 'NONE', #9039, #29500, #27343, .T. ) ;
#23383=VERTEX_POINT ( 'NONE', #23503 ) ;
#23386=ADVANCED_FACE ( 'NONE', ( #47995 ), #44664, .T. ) ;
#23392=CARTESIAN_POINT ( 'NONE',  ( 155.0540265531850537, -1.025126265847089657, -120.9317124430720440 ) ) ;
#23394=EDGE_CURVE ( 'NONE', #35332, #5910, #34147, .T. ) ;
#23407=CARTESIAN_POINT ( 'NONE',  ( -88.44597344681497475, 0.000000000000000000, -40.93171244307205825 ) ) ;
#23410=EDGE_LOOP ( 'NONE', ( #7, #50711, #36751, #3108, #4863, #38280 ) ) ;
#23411=DIRECTION ( 'NONE',  ( -0.000000000000000000, -0.000000000000000000, -1.000000000000000000 ) ) ;
#23415=CARTESIAN_POINT ( 'NONE',  ( -168.4459734468149463, 0.000000000000000000, 159.0682875569279702 ) ) ;
#23424=( BOUNDED_CURVE ( )  B_SPLINE_CURVE ( 3, ( #47551, #38643, #3458, #11680 ),
 .UNSPECIFIED., .F., .F. ) 
 B_SPLINE_CURVE_WITH_KNOTS ( ( 4, 4 ),
 ( 3.141592653589793116, 4.712388980384689674 ),
 .UNSPECIFIED. ) 
 CURVE ( )  GEOMETRIC_REPRESENTATION_ITEM ( )  RATIONAL_B_SPLINE_CURVE ( ( 1.000000000000000000, 0.8047378541243649375, 0.8047378541243649375, 1.000000000000000000 ) ) 
 REPRESENTATION_ITEM ( '' )  );
#23425=CARTESIAN_POINT ( 'NONE',  ( -207.7210997126620384, -1.750000000000009548, -0.2068387089191121020 ) ) ;
#23428=ORIENTED_EDGE ( 'NONE', *, *, #42917, .F. ) ;
#23432=CARTESIAN_POINT ( 'NONE',  ( 191.5540265531851105, 0.000000000000000000, -77.43171244307204404 ) ) ;
#23436=ORIENTED_EDGE ( 'NONE', *, *, #43808, .F. ) ;
#23439=ADVANCED_FACE ( 'NONE', ( #13139 ), #25705, .T. ) ;
#23442=DIRECTION ( 'NONE',  ( -0.000000000000000000, -0.000000000000000000, -1.000000000000000000 ) ) ;
#23447=VERTEX_POINT ( 'NONE', #44908 ) ;
#23449=CARTESIAN_POINT ( 'NONE',  ( -46.69597344681494633, 1.750000000000010214, 40.81828755692798438 ) ) ;
#23454=CARTESIAN_POINT ( 'NONE',  ( -8.445973446814962315, 1.025126265847096985, -160.9317124430720014 ) ) ;
#23460=ADVANCED_FACE ( 'NONE', ( #17753 ), #44420, .T. ) ;
#23467=CARTESIAN_POINT ( 'NONE',  ( -166.6959734468149463, -1.750000000000009992, 160.8182875569279702 ) ) ;
#23468=DIRECTION ( 'NONE',  ( -1.000000000000000000, 0.000000000000000000, 0.000000000000000000 ) ) ;
#23469=EDGE_CURVE ( 'NONE', #6842, #11488, #44572, .T. ) ;
#23472=CARTESIAN_POINT ( 'NONE',  ( -126.6959734468149321, 1.749999999999997335, -79.18171244307201562 ) ) ;
#23481=( BOUNDED_CURVE ( )  B_SPLINE_CURVE ( 3, ( #35047, #4230, #50615, #47026 ),
 .UNSPECIFIED., .F., .F. ) 
 B_SPLINE_CURVE_WITH_KNOTS ( ( 4, 4 ),
 ( 1.570796326794896558, 3.141592653589793116 ),
 .UNSPECIFIED. ) 
 CURVE ( )  GEOMETRIC_REPRESENTATION_ITEM ( )  RATIONAL_B_SPLINE_CURVE ( ( 1.000000000000000000, 0.8047378541243649375, 0.8047378541243649375, 1.000000000000000000 ) ) 
 REPRESENTATION_ITEM ( '' )  );
#23483=FACE_OUTER_BOUND ( 'NONE', #45189, .T. ) ;
#23485=CARTESIAN_POINT ( 'NONE',  ( -6.695973446814940111, 1.750000000000023759, -39.18171244307202983 ) ) ;
#23486=( BOUNDED_CURVE ( )  B_SPLINE_CURVE ( 3, ( #5088, #47908, #28954, #9452 ),
 .UNSPECIFIED., .F., .F. ) 
 B_SPLINE_CURVE_WITH_KNOTS ( ( 4, 4 ),
 ( 3.141592653589793116, 4.712388980384689674 ),
 .UNSPECIFIED. ) 
 CURVE ( )  GEOMETRIC_REPRESENTATION_ITEM ( )  RATIONAL_B_SPLINE_CURVE ( ( 1.000000000000000000, 0.8047378541243649375, 0.8047378541243649375, 1.000000000000000000 ) ) 
 REPRESENTATION_ITEM ( '' )  );
#23488=ORIENTED_EDGE ( 'NONE', *, *, #1241, .T. ) ;
#23494=CARTESIAN_POINT ( 'NONE',  ( 195.0540265531851105, 2.143131898507880377E-16, -157.4317124430720582 ) ) ;
#23497=CARTESIAN_POINT ( 'NONE',  ( 153.3040265531850537, 1.750000000000009992, 160.8182875569279702 ) ) ;
#23503=CARTESIAN_POINT ( 'NONE',  ( -168.4459734468149463, 0.000000000000000000, 39.06828755692798438 ) ) ;
#23508=DIRECTION ( 'NONE',  ( -0.000000000000000000, -0.000000000000000000, -1.000000000000000000 ) ) ;
#23511=DIRECTION ( 'NONE',  ( -1.000000000000000000, -0.000000000000000000, -0.000000000000000000 ) ) ;
#23516=ORIENTED_EDGE ( 'NONE', *, *, #25535, .T. ) ;
#23519=CYLINDRICAL_SURFACE ( 'NONE', #46086, 1.750000000000036193 ) ;
#23522=EDGE_CURVE ( 'NONE', #6202, #35055, #22281, .T. ) ;
#23526=LINE ( 'NONE', #39186, #3535 ) ;
#23529=EDGE_CURVE ( 'NONE', #43783, #21151, #39690, .T. ) ;
#23535=CYLINDRICAL_SURFACE ( 'NONE', #17635, 1.750000000000001554 ) ;
#23539=AXIS2_PLACEMENT_3D ( 'NONE', #19457, #35144, #50721 ) ;
#23541=ORIENTED_EDGE ( 'NONE', *, *, #24513, .T. ) ;
#23544=CARTESIAN_POINT ( 'NONE',  ( -88.44597344681494633, 1.025126265847089435, -40.93171244307204404 ) ) ;
#23545=VERTEX_POINT ( 'NONE', #29803 ) ;
#23546=CARTESIAN_POINT ( 'NONE',  ( -125.6708471809678542, -1.749999999999996669, -38.15658617722495194 ) ) ;
#23547=ORIENTED_EDGE ( 'NONE', *, *, #40394, .T. ) ;
#23548=EDGE_LOOP ( 'NONE', ( #18682, #46107, #3310, #29205, #30464, #41742 ) ) ;
#23556=EDGE_CURVE ( 'NONE', #13632, #14882, #34681, .T. ) ;
#23564=ORIENTED_EDGE ( 'NONE', *, *, #1607, .T. ) ;
#23568=ORIENTED_EDGE ( 'NONE', *, *, #44095, .T. ) ;
#23569=CARTESIAN_POINT ( 'NONE',  ( -124.9459734468149463, 2.143131898507847836E-16, 2.568287556927950632 ) ) ;
#23570=CARTESIAN_POINT ( 'NONE',  ( 195.0540265531851105, 2.143131898507880377E-16, -80.93171244307201562 ) ) ;
#23571=CARTESIAN_POINT ( 'NONE',  ( -48.44597344681495343, 0.000000000000000000, 159.0682875569279702 ) ) ;
#23573=DIRECTION ( 'NONE',  ( -1.000000000000000000, -0.000000000000000000, -0.000000000000000000 ) ) ;
#23582=DIRECTION ( 'NONE',  ( 0.000000000000000000, 0.000000000000000000, -1.000000000000000000 ) ) ;
#23586=VECTOR ( 'NONE', #11651, 1000.000000000000000 ) ;
#23588=LINE ( 'NONE', #27191, #22539 ) ;
#23590=EDGE_LOOP ( 'NONE', ( #15290, #19261, #43024, #27340, #9279, #41609 ) ) ;
#23598=LINE ( 'NONE', #16163, #3583 ) ;
#23600=VECTOR ( 'NONE', #37544, 1000.000000000000000 ) ;
#23602=LINE ( 'NONE', #19754, #49073 ) ;
#23608=ORIENTED_EDGE ( 'NONE', *, *, #5264, .T. ) ;
#23609=EDGE_CURVE ( 'NONE', #35393, #18024, #20338, .T. ) ;
#23612=( BOUNDED_CURVE ( )  B_SPLINE_CURVE ( 3, ( #33180, #48507, #11267, #42798 ),
 .UNSPECIFIED., .F., .F. ) 
 B_SPLINE_CURVE_WITH_KNOTS ( ( 4, 4 ),
 ( 4.712388980384689674, 6.283185307179586232 ),
 .UNSPECIFIED. ) 
 CURVE ( )  GEOMETRIC_REPRESENTATION_ITEM ( )  RATIONAL_B_SPLINE_CURVE ( ( 1.000000000000000000, 0.8047378541243649375, 0.8047378541243649375, 1.000000000000000000 ) ) 
 REPRESENTATION_ITEM ( '' )  );
#23614=EDGE_LOOP ( 'NONE', ( #8600, #43023, #28460, #39509, #25211, #6012 ) ) ;
#23616=DIRECTION ( 'NONE',  ( -1.000000000000000000, 0.000000000000000000, 0.000000000000000000 ) ) ;
#23619=( BOUNDED_CURVE ( )  B_SPLINE_CURVE ( 3, ( #28882, #16579, #12720, #25536 ),
 .UNSPECIFIED., .F., .F. ) 
 B_SPLINE_CURVE_WITH_KNOTS ( ( 4, 4 ),
 ( 3.141592653589793116, 4.712388980384689674 ),
 .UNSPECIFIED. ) 
 CURVE ( )  GEOMETRIC_REPRESENTATION_ITEM ( )  RATIONAL_B_SPLINE_CURVE ( ( 1.000000000000000000, 0.8047378541243649375, 0.8047378541243649375, 1.000000000000000000 ) ) 
 REPRESENTATION_ITEM ( '' )  );
#23624=CARTESIAN_POINT ( 'NONE',  ( -204.9459734468149463, 2.143131898507880377E-16, -37.43171244307205825 ) ) ;
#23631=( BOUNDED_CURVE ( )  B_SPLINE_CURVE ( 3, ( #37478, #17932, #36465, #28751 ),
 .UNSPECIFIED., .F., .F. ) 
 B_SPLINE_CURVE_WITH_KNOTS ( ( 4, 4 ),
 ( 4.712388980384689674, 6.283185307179586232 ),
 .UNSPECIFIED. ) 
 CURVE ( )  GEOMETRIC_REPRESENTATION_ITEM ( )  RATIONAL_B_SPLINE_CURVE ( ( 1.000000000000000000, 0.8047378541243649375, 0.8047378541243649375, 1.000000000000000000 ) ) 
 REPRESENTATION_ITEM ( '' )  );
#23634=EDGE_CURVE ( 'NONE', #8918, #4845, #45673, .T. ) ;
#23638=CARTESIAN_POINT ( 'NONE',  ( -124.9459734468149463, 2.143131898507847836E-16, -40.93171244307202983 ) ) ;
#23639=ADVANCED_FACE ( 'NONE', ( #6959 ), #38024, .T. ) ;
#23641=EDGE_CURVE ( 'NONE', #41219, #25957, #32790, .T. ) ;
#23642=CARTESIAN_POINT ( 'NONE',  ( -204.9459734468149463, 2.143131898507880377E-16, -40.93171244307202983 ) ) ;
#23644=CARTESIAN_POINT ( 'NONE',  ( 210.0000000000000568, 0.000000000000000000, 2.568287556927987048 ) ) ;
#23646=CARTESIAN_POINT ( 'NONE',  ( -48.44597344681496054, 1.025126265847089435, -77.43171244307200141 ) ) ;
#23653=VERTEX_POINT ( 'NONE', #288 ) ;
#23655=ORIENTED_EDGE ( 'NONE', *, *, #36978, .T. ) ;
#23663=DIRECTION ( 'NONE',  ( 0.000000000000000000, 0.000000000000000000, 1.000000000000000000 ) ) ;
#23664=ORIENTED_EDGE ( 'NONE', *, *, #25841, .T. ) ;
#23667=CARTESIAN_POINT ( 'NONE',  ( -208.4459734468148611, -1.025126265847089213, -0.9317124430720324924 ) ) ;
#23672=CARTESIAN_POINT ( 'NONE',  ( 111.5540265531850679, 0.000000000000000000, 2.568287556927950632 ) ) ;
#23679=DIRECTION ( 'NONE',  ( -1.000000000000000000, 0.000000000000000000, 0.000000000000000000 ) ) ;
#23680=CARTESIAN_POINT ( 'NONE',  ( -208.4459734468149463, 0.000000000000000000, 119.0682875569279702 ) ) ;
#23683=CARTESIAN_POINT ( 'NONE',  ( 35.05402655318504657, 2.143131898507880377E-16, -37.43171244307200141 ) ) ;
#23684=AXIS2_PLACEMENT_3D ( 'NONE', #10565, #45435, #3112 ) ;
#23697=CARTESIAN_POINT ( 'NONE',  ( -207.7210997126620384, 1.750000000000010436, 119.7931612910808781 ) ) ;
#23701=CARTESIAN_POINT ( 'NONE',  ( 114.3291528190321173, 1.749999999999996225, 161.8434138227750907 ) ) ;
#23702=ORIENTED_EDGE ( 'NONE', *, *, #31474, .F. ) ;
#23704=CARTESIAN_POINT ( 'NONE',  ( -45.67084718096785423, -1.750000000000009548, 81.84341382277507648 ) ) ;
#23708=CARTESIAN_POINT ( 'NONE',  ( 35.05402655318504657, 2.143131898507880377E-16, 165.0000000000000000 ) ) ;
#23709=ADVANCED_FACE ( 'NONE', ( #546 ), #40044, .T. ) ;
#23713=ORIENTED_EDGE ( 'NONE', *, *, #43986, .F. ) ;
#23717=CARTESIAN_POINT ( 'NONE',  ( 210.0000000000000568, 0.000000000000000000, 40.81828755692798438 ) ) ;
#23720=( BOUNDED_CURVE ( )  B_SPLINE_CURVE ( 3, ( #25685, #32890, #44149, #20810 ),
 .UNSPECIFIED., .F., .F. ) 
 B_SPLINE_CURVE_WITH_KNOTS ( ( 4, 4 ),
 ( 0.000000000000000000, 1.570796326794896558 ),
 .UNSPECIFIED. ) 
 CURVE ( )  GEOMETRIC_REPRESENTATION_ITEM ( )  RATIONAL_B_SPLINE_CURVE ( ( 1.000000000000000000, 0.8047378541243649375, 0.8047378541243649375, 1.000000000000000000 ) ) 
 REPRESENTATION_ITEM ( '' )  );
#23723=EDGE_CURVE ( 'NONE', #19705, #28470, #21980, .T. ) ;
#23728=AXIS2_PLACEMENT_3D ( 'NONE', #28638, #40706, #21192 ) ;
#23730=EDGE_CURVE ( 'NONE', #41145, #41350, #5440, .T. ) ;
#23731=CARTESIAN_POINT ( 'NONE',  ( -128.4459734468149463, 1.025126265847081664, 42.56828755692797017 ) ) ;
#23738=EDGE_CURVE ( 'NONE', #11190, #37195, #20279, .T. ) ;
#23742=CYLINDRICAL_SURFACE ( 'NONE', #2801, 1.750000000000001554 ) ;
#23743=CARTESIAN_POINT ( 'NONE',  ( -204.9459734468149463, 2.143131898507880377E-16, 42.56828755692798438 ) ) ;
#23746=ORIENTED_EDGE ( 'NONE', *, *, #4628, .T. ) ;
#23754=ORIENTED_EDGE ( 'NONE', *, *, #22390, .T. ) ;
#23757=CARTESIAN_POINT ( 'NONE',  ( 34.32915281903212446, -1.750000000000009326, 159.7931612910809065 ) ) ;
#23770=DIRECTION ( 'NONE',  ( -0.000000000000000000, -0.000000000000000000, -1.000000000000000000 ) ) ;
#23773=CARTESIAN_POINT ( 'NONE',  ( -168.4459734468149747, -1.025126265847089879, 82.56828755692798438 ) ) ;
#23778=LINE ( 'NONE', #5020, #45140 ) ;
#23781=( BOUNDED_CURVE ( )  B_SPLINE_CURVE ( 3, ( #32583, #48167, #5360, #40027 ),
 .UNSPECIFIED., .F., .F. ) 
 B_SPLINE_CURVE_WITH_KNOTS ( ( 4, 4 ),
 ( 0.000000000000000000, 1.570796326794896558 ),
 .UNSPECIFIED. ) 
 CURVE ( )  GEOMETRIC_REPRESENTATION_ITEM ( )  RATIONAL_B_SPLINE_CURVE ( ( 1.000000000000000000, 0.8047378541243649375, 0.8047378541243649375, 1.000000000000000000 ) ) 
 REPRESENTATION_ITEM ( '' )  );
#23789=VECTOR ( 'NONE', #32490, 1000.000000000000000 ) ;
#23796=VERTEX_POINT ( 'NONE', #17187 ) ;
#23803=EDGE_CURVE ( 'NONE', #21335, #26878, #30839, .T. ) ;
#23805=FACE_OUTER_BOUND ( 'NONE', #41508, .T. ) ;
#23806=CARTESIAN_POINT ( 'NONE',  ( 115.0540265531850395, 2.143131898507847836E-16, -117.4317124430720725 ) ) ;
#23808=LINE ( 'NONE', #969, #33344 ) ;
#23812=DIRECTION ( 'NONE',  ( 0.000000000000000000, 0.000000000000000000, 1.000000000000000000 ) ) ;
#23814=CARTESIAN_POINT ( 'NONE',  ( 113.3040265531850537, -1.749999999999997335, 120.8182875569279702 ) ) ;
#23816=DIRECTION ( 'NONE',  ( -1.000000000000000000, -0.000000000000000000, -0.000000000000000000 ) ) ;
#23818=ORIENTED_EDGE ( 'NONE', *, *, #30216, .T. ) ;
#23824=ORIENTED_EDGE ( 'NONE', *, *, #30895, .F. ) ;
#23831=CARTESIAN_POINT ( 'NONE',  ( -168.4459734468149463, 0.000000000000000000, -157.4317124430720582 ) ) ;
#23840=DIRECTION ( 'NONE',  ( 0.000000000000000000, 0.000000000000000000, 1.000000000000000000 ) ) ;
#23841=LINE ( 'NONE', #19295, #34915 ) ;
#23844=VERTEX_POINT ( 'NONE', #17439 ) ;
#23846=EDGE_CURVE ( 'NONE', #920, #32767, #33354, .T. ) ;
#23849=LINE ( 'NONE', #258, #7433 ) ;
#23852=DIRECTION ( 'NONE',  ( -1.000000000000000000, -0.000000000000000000, -0.000000000000000000 ) ) ;
#23855=VERTEX_POINT ( 'NONE', #13819 ) ;
#23858=EDGE_LOOP ( 'NONE', ( #44382, #46239, #7994, #8330, #17611, #27648 ) ) ;
#23859=CARTESIAN_POINT ( 'NONE',  ( -206.6959734468149463, 1.750000000000009992, 160.8182875569279702 ) ) ;
#23863=FACE_OUTER_BOUND ( 'NONE', #27555, .T. ) ;
#23864=CARTESIAN_POINT ( 'NONE',  ( 155.0540265531850537, 2.143131898507880377E-16, 122.5682875569279702 ) ) ;
#23866=DIRECTION ( 'NONE',  ( 1.000000000000000000, 0.000000000000000000, 0.000000000000000000 ) ) ;
#23867=CARTESIAN_POINT ( 'NONE',  ( 111.5540265531850537, 1.025126265847081442, -0.9317124430720195027 ) ) ;
#23869=CARTESIAN_POINT ( 'NONE',  ( 191.5540265531850537, 1.025126265847089213, 162.5682875569279133 ) ) ;
#23871=CARTESIAN_POINT ( 'NONE',  ( 210.0000000000000568, 0.000000000000000000, -159.1817124430720298 ) ) ;
#23875=CARTESIAN_POINT ( 'NONE',  ( 155.0540265531850537, 2.143131898507880377E-16, 42.56828755692798438 ) ) ;
#23876=ORIENTED_EDGE ( 'NONE', *, *, #41883, .F. ) ;
#23883=CARTESIAN_POINT ( 'NONE',  ( 152.2789002873379900, 1.750000000000009326, -158.1565861772249377 ) ) ;
#23894=CARTESIAN_POINT ( 'NONE',  ( -208.4459734468148611, 1.025126265847089657, -80.93171244307201562 ) ) ;
#23897=CARTESIAN_POINT ( 'NONE',  ( 111.5540265531850679, 0.000000000000000000, -0.9317124430719969652 ) ) ;
#23901=CIRCLE ( 'NONE', #5873, 1.750000000000001554 ) ;
#23910=CARTESIAN_POINT ( 'NONE',  ( -207.7210997126620384, -1.750000000000009548, 159.7931612910809065 ) ) ;
#23912=CARTESIAN_POINT ( 'NONE',  ( 195.0540265531851105, 1.025126265847089657, 42.56828755692799149 ) ) ;
#23914=( BOUNDED_CURVE ( )  B_SPLINE_CURVE ( 3, ( #17353, #44783, #41200, #33282 ),
 .UNSPECIFIED., .F., .F. ) 
 B_SPLINE_CURVE_WITH_KNOTS ( ( 4, 4 ),
 ( 0.000000000000000000, 1.570796326794896558 ),
 .UNSPECIFIED. ) 
 CURVE ( )  GEOMETRIC_REPRESENTATION_ITEM ( )  RATIONAL_B_SPLINE_CURVE ( ( 1.000000000000000000, 0.8047378541243649375, 0.8047378541243649375, 1.000000000000000000 ) ) 
 REPRESENTATION_ITEM ( '' )  );
#23916=CYLINDRICAL_SURFACE ( 'NONE', #25429, 1.750000000000001554 ) ;
#23918=CARTESIAN_POINT ( 'NONE',  ( -8.445973446814976526, 0.000000000000000000, -0.9317124430720524764 ) ) ;
#23919=CARTESIAN_POINT ( 'NONE',  ( 153.3040265531850537, -1.750000000000010658, 120.8182875569279702 ) ) ;
#23920=CARTESIAN_POINT ( 'NONE',  ( 35.05402655318504657, 1.025126265847089879, 82.56828755692798438 ) ) ;
#23922=( BOUNDED_CURVE ( )  B_SPLINE_CURVE ( 3, ( #41991, #22241, #37913, #49641 ),
 .UNSPECIFIED., .F., .F. ) 
 B_SPLINE_CURVE_WITH_KNOTS ( ( 4, 4 ),
 ( 3.141592653589793116, 4.712388980384689674 ),
 .UNSPECIFIED. ) 
 CURVE ( )  GEOMETRIC_REPRESENTATION_ITEM ( )  RATIONAL_B_SPLINE_CURVE ( ( 1.000000000000000000, 0.8047378541243649375, 0.8047378541243649375, 1.000000000000000000 ) ) 
 REPRESENTATION_ITEM ( '' )  );
#23924=ORIENTED_EDGE ( 'NONE', *, *, #31152, .F. ) ;
#23926=DIRECTION ( 'NONE',  ( -0.000000000000000000, -0.000000000000000000, -1.000000000000000000 ) ) ;
#23930=CARTESIAN_POINT ( 'NONE',  ( 154.3291528190321458, -1.750000000000009548, 81.84341382277507648 ) ) ;
#23931=CARTESIAN_POINT ( 'NONE',  ( 35.05402655318504657, -1.025126265847089657, -120.9317124430720440 ) ) ;
#23932=VERTEX_POINT ( 'NONE', #36456 ) ;
#23934=ADVANCED_FACE ( 'NONE', ( #45109 ), #1296, .T. ) ;
#23935=VERTEX_POINT ( 'NONE', #16945 ) ;
#23936=( BOUNDED_CURVE ( )  B_SPLINE_CURVE ( 3, ( #45174, #42548, #23056, #38727 ),
 .UNSPECIFIED., .F., .F. ) 
 B_SPLINE_CURVE_WITH_KNOTS ( ( 4, 4 ),
 ( 0.000000000000000000, 1.570796326794896558 ),
 .UNSPECIFIED. ) 
 CURVE ( )  GEOMETRIC_REPRESENTATION_ITEM ( )  RATIONAL_B_SPLINE_CURVE ( ( 1.000000000000000000, 0.8047378541243649375, 0.8047378541243649375, 1.000000000000000000 ) ) 
 REPRESENTATION_ITEM ( '' )  );
#23942=VERTEX_POINT ( 'NONE', #44600 ) ;
#23943=ORIENTED_EDGE ( 'NONE', *, *, #25726, .T. ) ;
#23946=CARTESIAN_POINT ( 'NONE',  ( 115.0540265531850395, 2.143131898507847836E-16, -117.4317124430720725 ) ) ;
#23948=AXIS2_PLACEMENT_3D ( 'NONE', #10607, #26271, #41911 ) ;
#23949=ADVANCED_FACE ( 'NONE', ( #25147 ), #40791, .T. ) ;
#23950=ORIENTED_EDGE ( 'NONE', *, *, #31352, .F. ) ;
#23964=CARTESIAN_POINT ( 'NONE',  ( -128.4459734468149179, 0.000000000000000000, -120.9317124430720156 ) ) ;
#23967=CARTESIAN_POINT ( 'NONE',  ( 153.3040265531850537, 0.000000000000000000, 165.0000000000000000 ) ) ;
#23972=EDGE_CURVE ( 'NONE', #40787, #11639, #10494, .T. ) ;
#23974=VECTOR ( 'NONE', #7583, 1000.000000000000000 ) ;
#23976=ADVANCED_FACE ( 'NONE', ( #41544 ), #37710, .T. ) ;
#23981=ORIENTED_EDGE ( 'NONE', *, *, #3386, .F. ) ;
#23986=VERTEX_POINT ( 'NONE', #41786 ) ;
#23995=CARTESIAN_POINT ( 'NONE',  ( 31.55402655318503236, 0.000000000000000000, 119.0682875569279702 ) ) ;
#24000=VECTOR ( 'NONE', #33990, 1000.000000000000000 ) ;
#24001=ORIENTED_EDGE ( 'NONE', *, *, #26811, .T. ) ;
#24004=ORIENTED_EDGE ( 'NONE', *, *, #43769, .T. ) ;
#24006=VECTOR ( 'NONE', #14299, 1000.000000000000000 ) ;
#24007=ADVANCED_FACE ( 'NONE', ( #3037 ), #30007, .T. ) ;
#24010=VECTOR ( 'NONE', #24982, 1000.000000000000000 ) ;
#24020=LINE ( 'NONE', #39674, #34824 ) ;
#24021=CARTESIAN_POINT ( 'NONE',  ( 35.05402655318504657, 1.025126265847089435, -157.4317124430720582 ) ) ;
#24025=CARTESIAN_POINT ( 'NONE',  ( 151.5540265531850537, 0.000000000000000000, -157.4317124430720582 ) ) ;
#24026=( BOUNDED_CURVE ( )  B_SPLINE_CURVE ( 3, ( #10260, #20785, #36467, #37235 ),
 .UNSPECIFIED., .F., .F. ) 
 B_SPLINE_CURVE_WITH_KNOTS ( ( 4, 4 ),
 ( 4.712388980384689674, 6.283185307179586232 ),
 .UNSPECIFIED. ) 
 CURVE ( )  GEOMETRIC_REPRESENTATION_ITEM ( )  RATIONAL_B_SPLINE_CURVE ( ( 1.000000000000000000, 0.8047378541243649375, 0.8047378541243649375, 1.000000000000000000 ) ) 
 REPRESENTATION_ITEM ( '' )  );
#24028=DIRECTION ( 'NONE',  ( -0.000000000000000000, -0.000000000000000000, -1.000000000000000000 ) ) ;
#24030=DIRECTION ( 'NONE',  ( -0.000000000000000000, -0.000000000000000000, -1.000000000000000000 ) ) ;
#24034=EDGE_CURVE ( 'NONE', #5399, #13539, #46820, .T. ) ;
#24035=EDGE_CURVE ( 'NONE', #19888, #50159, #25282, .T. ) ;
#24043=CARTESIAN_POINT ( 'NONE',  ( -168.4459734468149747, 2.143131898507880377E-16, -160.9317124430720298 ) ) ;
#24044=AXIS2_PLACEMENT_3D ( 'NONE', #3249, #34577, #34081 ) ;
#24052=CARTESIAN_POINT ( 'NONE',  ( -85.67084718096784002, -1.750000000000009548, -78.15658617722490931 ) ) ;
#24055=ORIENTED_EDGE ( 'NONE', *, *, #49008, .F. ) ;
#24056=CARTESIAN_POINT ( 'NONE',  ( 33.30402655318503946, 0.000000000000000000, 165.0000000000000000 ) ) ;
#24061=CARTESIAN_POINT ( 'NONE',  ( -6.695973446814940111, 1.750000000000024203, 80.81828755692798438 ) ) ;
#24062=ORIENTED_EDGE ( 'NONE', *, *, #11881, .F. ) ;
#24070=CYLINDRICAL_SURFACE ( 'NONE', #19318, 1.750000000000015543 ) ;
#24074=AXIS2_PLACEMENT_3D ( 'NONE', #13215, #20405, #1931 ) ;
#24076=AXIS2_PLACEMENT_3D ( 'NONE', #25951, #21575, #33645 ) ;
#24078=ORIENTED_EDGE ( 'NONE', *, *, #30935, .F. ) ;
#24079=ORIENTED_EDGE ( 'NONE', *, *, #14396, .F. ) ;
#24082=CARTESIAN_POINT ( 'NONE',  ( 155.0540265531850537, -1.025126265847088991, 2.568287556927986159 ) ) ;
#24086=DIRECTION ( 'NONE',  ( 1.000000000000000000, 0.000000000000000000, 0.000000000000000000 ) ) ;
#24089=( BOUNDED_CURVE ( )  B_SPLINE_CURVE ( 3, ( #11305, #26195, #34408, #38519 ),
 .UNSPECIFIED., .F., .F. ) 
 B_SPLINE_CURVE_WITH_KNOTS ( ( 4, 4 ),
 ( 0.000000000000000000, 1.570796326794896558 ),
 .UNSPECIFIED. ) 
 CURVE ( )  GEOMETRIC_REPRESENTATION_ITEM ( )  RATIONAL_B_SPLINE_CURVE ( ( 1.000000000000000000, 0.8047378541243649375, 0.8047378541243649375, 1.000000000000000000 ) ) 
 REPRESENTATION_ITEM ( '' )  );
#24095=( BOUNDED_CURVE ( )  B_SPLINE_CURVE ( 3, ( #21864, #5944, #45165, #25453 ),
 .UNSPECIFIED., .F., .F. ) 
 B_SPLINE_CURVE_WITH_KNOTS ( ( 4, 4 ),
 ( 1.570796326794896558, 3.141592653589793116 ),
 .UNSPECIFIED. ) 
 CURVE ( )  GEOMETRIC_REPRESENTATION_ITEM ( )  RATIONAL_B_SPLINE_CURVE ( ( 1.000000000000000000, 0.8047378541243649375, 0.8047378541243649375, 1.000000000000000000 ) ) 
 REPRESENTATION_ITEM ( '' )  );
#24103=CARTESIAN_POINT ( 'NONE',  ( 152.2789002873379900, 1.750000000000010436, 119.7931612910808781 ) ) ;
#24104=VERTEX_POINT ( 'NONE', #47625 ) ;
#24120=AXIS2_PLACEMENT_3D ( 'NONE', #7192, #2569, #50227 ) ;
#24126=EDGE_LOOP ( 'NONE', ( #5875, #21768 ) ) ;
#24128=EDGE_LOOP ( 'NONE', ( #26834, #38204, #38373, #41404, #39733, #32127 ) ) ;
#24140=CARTESIAN_POINT ( 'NONE',  ( 151.5540265531850537, 0.000000000000000000, 82.56828755692798438 ) ) ;
#24144=CARTESIAN_POINT ( 'NONE',  ( 73.30402655318508209, 0.000000000000000000, 165.0000000000000000 ) ) ;
#24157=ORIENTED_EDGE ( 'NONE', *, *, #22593, .T. ) ;
#24158=VECTOR ( 'NONE', #9551, 1000.000000000000000 ) ;
#24161=DIRECTION ( 'NONE',  ( 0.000000000000000000, 0.000000000000000000, 1.000000000000000000 ) ) ;
#24165=ORIENTED_EDGE ( 'NONE', *, *, #37230, .F. ) ;
#24167=FACE_OUTER_BOUND ( 'NONE', #5548, .T. ) ;
#24168=CARTESIAN_POINT ( 'NONE',  ( 114.3291528190321173, 1.749999999999996669, -40.20683870891911482 ) ) ;
#24169=DIRECTION ( 'NONE',  ( -0.000000000000000000, -0.000000000000000000, -1.000000000000000000 ) ) ;
#24176=ORIENTED_EDGE ( 'NONE', *, *, #15588, .F. ) ;
#24179=CARTESIAN_POINT ( 'NONE',  ( 75.05402655318509630, 2.143131898507880377E-16, 39.06828755692795596 ) ) ;
#24181=CARTESIAN_POINT ( 'NONE',  ( 194.3291528190321742, 1.750000000000009548, 41.84341382277508359 ) ) ;
#24183=CARTESIAN_POINT ( 'NONE',  ( -125.6708471809678542, 1.749999999999996669, -0.2068387089191042749 ) ) ;
#24188=DIRECTION ( 'NONE',  ( -0.000000000000000000, -0.000000000000000000, -1.000000000000000000 ) ) ;
#24193=CARTESIAN_POINT ( 'NONE',  ( 210.0000000000000568, 0.000000000000000000, 42.56828755692799149 ) ) ;
#24198=DIRECTION ( 'NONE',  ( -0.000000000000000000, -0.000000000000000000, -1.000000000000000000 ) ) ;
#24211=PRODUCT_DEFINITION_CONTEXT ( 'detailed design', #40744, 'design' ) ;
#24221=CARTESIAN_POINT ( 'NONE',  ( -48.44597344681495343, 0.000000000000000000, 82.56828755692798438 ) ) ;
#24222=CARTESIAN_POINT ( 'NONE',  ( -44.94597344681493922, 2.143131898507880377E-16, 119.0682875569279702 ) ) ;
#24224=DIRECTION ( 'NONE',  ( -0.000000000000000000, -0.000000000000000000, -1.000000000000000000 ) ) ;
#24226=ORIENTED_EDGE ( 'NONE', *, *, #15155, .T. ) ;
#24229=CARTESIAN_POINT ( 'NONE',  ( -47.72109971266203132, -1.750000000000010214, 79.79316129108087807 ) ) ;
#24230=CARTESIAN_POINT ( 'NONE',  ( 31.55402655318503236, 0.000000000000000000, -40.93171244307205825 ) ) ;
#24232=( BOUNDED_CURVE ( )  B_SPLINE_CURVE ( 3, ( #12292, #44329, #9197, #44564 ),
 .UNSPECIFIED., .F., .F. ) 
 B_SPLINE_CURVE_WITH_KNOTS ( ( 4, 4 ),
 ( 0.000000000000000000, 1.570796326794896558 ),
 .UNSPECIFIED. ) 
 CURVE ( )  GEOMETRIC_REPRESENTATION_ITEM ( )  RATIONAL_B_SPLINE_CURVE ( ( 1.000000000000000000, 0.8047378541243649375, 0.8047378541243649375, 1.000000000000000000 ) ) 
 REPRESENTATION_ITEM ( '' )  );
#24238=( BOUNDED_CURVE ( )  B_SPLINE_CURVE ( 3, ( #17214, #17714, #49215, #1816 ),
 .UNSPECIFIED., .F., .F. ) 
 B_SPLINE_CURVE_WITH_KNOTS ( ( 4, 4 ),
 ( 4.712388980384689674, 6.283185307179586232 ),
 .UNSPECIFIED. ) 
 CURVE ( )  GEOMETRIC_REPRESENTATION_ITEM ( )  RATIONAL_B_SPLINE_CURVE ( ( 1.000000000000000000, 0.8047378541243649375, 0.8047378541243649375, 1.000000000000000000 ) ) 
 REPRESENTATION_ITEM ( '' )  );
#24239=DIRECTION ( 'NONE',  ( 0.000000000000000000, 0.000000000000000000, -1.000000000000000000 ) ) ;
#24241=CARTESIAN_POINT ( 'NONE',  ( 115.0540265531850395, 2.143131898507847836E-16, 82.56828755692797017 ) ) ;
#24243=CARTESIAN_POINT ( 'NONE',  ( -168.4459734468149747, 2.143131898507880377E-16, -160.9317124430720298 ) ) ;
#24247=( BOUNDED_CURVE ( )  B_SPLINE_CURVE ( 3, ( #12759, #47359, #12254, #43550 ),
 .UNSPECIFIED., .F., .F. ) 
 B_SPLINE_CURVE_WITH_KNOTS ( ( 4, 4 ),
 ( 4.712388980384689674, 6.283185307179586232 ),
 .UNSPECIFIED. ) 
 CURVE ( )  GEOMETRIC_REPRESENTATION_ITEM ( )  RATIONAL_B_SPLINE_CURVE ( ( 1.000000000000000000, 0.8047378541243649375, 0.8047378541243649375, 1.000000000000000000 ) ) 
 REPRESENTATION_ITEM ( '' )  );
#24249=EDGE_LOOP ( 'NONE', ( #39356, #31667, #15401, #45783, #10997, #29717 ) ) ;
#24250=CARTESIAN_POINT ( 'NONE',  ( 155.0540265531850537, 2.143131898507890731E-16, -165.0000000000000000 ) ) ;
#24251=CARTESIAN_POINT ( 'NONE',  ( 155.0540265531850537, 2.143131898507880377E-16, -0.9317124430720247208 ) ) ;
#24252=EDGE_CURVE ( 'NONE', #17436, #6557, #11803, .T. ) ;
#24257=CARTESIAN_POINT ( 'NONE',  ( -204.9459734468148895, -1.025126265847089657, 79.06828755692797017 ) ) ;
#24259=DIRECTION ( 'NONE',  ( 0.000000000000000000, 0.000000000000000000, 1.000000000000000000 ) ) ;
#24267=CARTESIAN_POINT ( 'NONE',  ( 73.30402655318508209, -1.750000000000010214, 40.81828755692798438 ) ) ;
#24277=ORIENTED_EDGE ( 'NONE', *, *, #40636, .F. ) ;
#24281=ORIENTED_EDGE ( 'NONE', *, *, #22677, .F. ) ;
#24283=CARTESIAN_POINT ( 'NONE',  ( -84.94597344681494633, 2.143131898507880377E-16, 122.5682875569279702 ) ) ;
#24284=CARTESIAN_POINT ( 'NONE',  ( -48.44597344681495343, 0.000000000000000000, 119.0682875569279702 ) ) ;
#24285=CARTESIAN_POINT ( 'NONE',  ( -44.94597344681493922, 2.143131898507880377E-16, 39.06828755692798438 ) ) ;
#24286=AXIS2_PLACEMENT_3D ( 'NONE', #29540, #9539, #37519 ) ;
#24288=AXIS2_PLACEMENT_3D ( 'NONE', #35771, #23442, #20084 ) ;
#24289=ORIENTED_EDGE ( 'NONE', *, *, #6086, .F. ) ;
#24291=FACE_OUTER_BOUND ( 'NONE', #43282, .T. ) ;
#24293=EDGE_CURVE ( 'NONE', #48817, #21466, #8921, .T. ) ;
#24298=VECTOR ( 'NONE', #1553, 1000.000000000000000 ) ;
#24299=CARTESIAN_POINT ( 'NONE',  ( 33.30402655318503946, 1.750000000000010658, 120.8182875569279702 ) ) ;
#24301=CARTESIAN_POINT ( 'NONE',  ( -8.445973446814964092, -1.025126265847097651, -117.4317124430720014 ) ) ;
#24308=ORIENTED_EDGE ( 'NONE', *, *, #25545, .F. ) ;
#24317=FACE_OUTER_BOUND ( 'NONE', #544, .T. ) ;
#24321=DIRECTION ( 'NONE',  ( 0.000000000000000000, 0.000000000000000000, 1.000000000000000000 ) ) ;
#24322=EDGE_CURVE ( 'NONE', #42490, #48152, #16739, .T. ) ;
#24324=ORIENTED_EDGE ( 'NONE', *, *, #20181, .F. ) ;
#24325=DIRECTION ( 'NONE',  ( -1.000000000000000000, -0.000000000000000000, -0.000000000000000000 ) ) ;
#24328=CARTESIAN_POINT ( 'NONE',  ( 71.55402655318505367, 0.000000000000000000, 122.5682875569279844 ) ) ;
#24330=DIRECTION ( 'NONE',  ( -1.000000000000000000, 0.000000000000000000, 0.000000000000000000 ) ) ;
#24333=EDGE_CURVE ( 'NONE', #39140, #2997, #22485, .T. ) ;
#24340=EDGE_CURVE ( 'NONE', #38537, #14624, #2727, .T. ) ;
#24341=EDGE_CURVE ( 'NONE', #11190, #6144, #17039, .T. ) ;
#24343=ORIENTED_EDGE ( 'NONE', *, *, #44747, .T. ) ;
#24348=CARTESIAN_POINT ( 'NONE',  ( 111.5540265531850679, 0.000000000000000000, -37.43171244307205825 ) ) ;
#24352=FACE_OUTER_BOUND ( 'NONE', #37502, .T. ) ;
#24362=CARTESIAN_POINT ( 'NONE',  ( 210.0000000000000568, 0.000000000000000000, 2.568287556927987048 ) ) ;
#24369=LINE ( 'NONE', #31570, #15942 ) ;
#24370=EDGE_CURVE ( 'NONE', #21159, #32283, #27239, .T. ) ;
#24375=ORIENTED_EDGE ( 'NONE', *, *, #22101, .F. ) ;
#24376=ORIENTED_EDGE ( 'NONE', *, *, #16002, .F. ) ;
#24378=FACE_OUTER_BOUND ( 'NONE', #2957, .T. ) ;
#24380=ORIENTED_EDGE ( 'NONE', *, *, #23394, .T. ) ;
#24389=EDGE_CURVE ( 'NONE', #3971, #38882, #46046, .T. ) ;
#24392=DIRECTION ( 'NONE',  ( 0.000000000000000000, 0.000000000000000000, -1.000000000000000000 ) ) ;
#24395=( BOUNDED_CURVE ( )  B_SPLINE_CURVE ( 3, ( #5279, #16581, #676, #12467 ),
 .UNSPECIFIED., .F., .F. ) 
 B_SPLINE_CURVE_WITH_KNOTS ( ( 4, 4 ),
 ( 1.570796326794896558, 3.141592653589793116 ),
 .UNSPECIFIED. ) 
 CURVE ( )  GEOMETRIC_REPRESENTATION_ITEM ( )  RATIONAL_B_SPLINE_CURVE ( ( 1.000000000000000000, 0.8047378541243649375, 0.8047378541243649375, 1.000000000000000000 ) ) 
 REPRESENTATION_ITEM ( '' )  );
#24400=DIRECTION ( 'NONE',  ( -1.000000000000000000, -0.000000000000000000, -0.000000000000000000 ) ) ;
#24401=EDGE_CURVE ( 'NONE', #18807, #48817, #30525, .T. ) ;
#24404=EDGE_CURVE ( 'NONE', #27650, #47604, #50097, .T. ) ;
#24405=CARTESIAN_POINT ( 'NONE',  ( -4.945973446814917018, 1.025126265847097207, 39.06828755692796307 ) ) ;
#24406=ORIENTED_EDGE ( 'NONE', *, *, #26827, .T. ) ;
#24407=DIRECTION ( 'NONE',  ( 0.000000000000000000, 0.000000000000000000, 1.000000000000000000 ) ) ;
#24411=ORIENTED_EDGE ( 'NONE', *, *, #14563, .T. ) ;
#24414=CARTESIAN_POINT ( 'NONE',  ( 34.32915281903212446, -1.750000000000009548, -160.2068387089191219 ) ) ;
#24416=LINE ( 'NONE', #20549, #45523 ) ;
#24421=CARTESIAN_POINT ( 'NONE',  ( -204.9459734468149747, 0.000000000000000000, 162.5682875569279702 ) ) ;
#24422=DIRECTION ( 'NONE',  ( -1.000000000000000000, -0.000000000000000000, -0.000000000000000000 ) ) ;
#24424=VERTEX_POINT ( 'NONE', #15313 ) ;
#24425=LINE ( 'NONE', #8017, #33021 ) ;
#24426=VERTEX_POINT ( 'NONE', #4510 ) ;
#24431=CARTESIAN_POINT ( 'NONE',  ( -86.69597344681494633, 1.750000000000010214, 40.81828755692798438 ) ) ;
#24439=CARTESIAN_POINT ( 'NONE',  ( -124.9459734468149463, 2.143131898507847836E-16, 159.0682875569279702 ) ) ;
#24442=ORIENTED_EDGE ( 'NONE', *, *, #1446, .T. ) ;
#24444=CARTESIAN_POINT ( 'NONE',  ( 194.3291528190321742, 1.750000000000009548, -158.1565861772249377 ) ) ;
#24445=ADVANCED_FACE ( 'NONE', ( #46308 ), #38659, .T. ) ;
#24450=CARTESIAN_POINT ( 'NONE',  ( -88.44597344681497475, 0.000000000000000000, 42.56828755692799859 ) ) ;
#24452=VERTEX_POINT ( 'NONE', #19396 ) ;
#24453=CARTESIAN_POINT ( 'NONE',  ( -126.6959734468149321, 1.749999999999997335, -119.1817124430720440 ) ) ;
#24456=EDGE_CURVE ( 'NONE', #17311, #13126, #35809, .T. ) ;
#24461=ORIENTED_EDGE ( 'NONE', *, *, #38876, .F. ) ;
#24467=ORIENTED_EDGE ( 'NONE', *, *, #20959, .F. ) ;
#24468=ORIENTED_EDGE ( 'NONE', *, *, #49905, .T. ) ;
#24469=LINE ( 'NONE', #5209, #30781 ) ;
#24474=CARTESIAN_POINT ( 'NONE',  ( -46.69597344681494633, 1.750000000000010658, 80.81828755692798438 ) ) ;
#24485=ORIENTED_EDGE ( 'NONE', *, *, #23803, .T. ) ;
#24487=DIRECTION ( 'NONE',  ( -1.000000000000000000, -0.000000000000000000, -0.000000000000000000 ) ) ;
#24489=CIRCLE ( 'NONE', #4122, 1.749999999999987566 ) ;
#24505=FACE_OUTER_BOUND ( 'NONE', #19646, .T. ) ;
#24506=VERTEX_POINT ( 'NONE', #30704 ) ;
#24507=VERTEX_POINT ( 'NONE', #15804 ) ;
#24508=ORIENTED_EDGE ( 'NONE', *, *, #833, .T. ) ;
#24513=EDGE_CURVE ( 'NONE', #37518, #5763, #39392, .T. ) ;
#24514=CARTESIAN_POINT ( 'NONE',  ( -8.445973446814964092, -1.025126265847097651, -77.43171244307197298 ) ) ;
#24515=CARTESIAN_POINT ( 'NONE',  ( 111.5540265531850679, 0.000000000000000000, -40.93171244307202983 ) ) ;
#24516=ORIENTED_EDGE ( 'NONE', *, *, #39731, .F. ) ;
#24518=CARTESIAN_POINT ( 'NONE',  ( 35.05402655318504657, -1.025126265847089657, 79.06828755692797017 ) ) ;
#24522=( BOUNDED_CURVE ( )  B_SPLINE_CURVE ( 3, ( #45970, #14182, #3139, #33960 ),
 .UNSPECIFIED., .F., .F. ) 
 B_SPLINE_CURVE_WITH_KNOTS ( ( 4, 4 ),
 ( 1.570796326794896558, 3.141592653589793116 ),
 .UNSPECIFIED. ) 
 CURVE ( )  GEOMETRIC_REPRESENTATION_ITEM ( )  RATIONAL_B_SPLINE_CURVE ( ( 1.000000000000000000, 0.8047378541243649375, 0.8047378541243649375, 1.000000000000000000 ) ) 
 REPRESENTATION_ITEM ( '' )  );
#24523=FACE_OUTER_BOUND ( 'NONE', #13107, .T. ) ;
#24524=DIRECTION ( 'NONE',  ( 1.000000000000000000, 0.000000000000000000, 0.000000000000000000 ) ) ;
#24527=CARTESIAN_POINT ( 'NONE',  ( -86.69597344681494633, 1.750000000000010658, -119.1817124430720440 ) ) ;
#24528=AXIS2_PLACEMENT_3D ( 'NONE', #11845, #31614, #47200 ) ;
#24532=( BOUNDED_CURVE ( )  B_SPLINE_CURVE ( 3, ( #4166, #39577, #43398, #35744 ),
 .UNSPECIFIED., .F., .F. ) 
 B_SPLINE_CURVE_WITH_KNOTS ( ( 4, 4 ),
 ( 3.141592653589793116, 4.712388980384689674 ),
 .UNSPECIFIED. ) 
 CURVE ( )  GEOMETRIC_REPRESENTATION_ITEM ( )  RATIONAL_B_SPLINE_CURVE ( ( 1.000000000000000000, 0.8047378541243649375, 0.8047378541243649375, 1.000000000000000000 ) ) 
 REPRESENTATION_ITEM ( '' )  );
#24534=CARTESIAN_POINT ( 'NONE',  ( -164.9459734468149463, 1.025126265847089879, -117.4317124430720156 ) ) ;
#24535=CARTESIAN_POINT ( 'NONE',  ( -6.695973446814940111, 1.750000000000023315, 0.8182875569279768335 ) ) ;
#24537=DIRECTION ( 'NONE',  ( -0.000000000000000000, -0.000000000000000000, -1.000000000000000000 ) ) ;
#24538=( BOUNDED_CURVE ( )  B_SPLINE_CURVE ( 3, ( #20656, #17060, #24514, #28866 ),
 .UNSPECIFIED., .F., .F. ) 
 B_SPLINE_CURVE_WITH_KNOTS ( ( 4, 4 ),
 ( 1.570796326794896558, 3.141592653589793116 ),
 .UNSPECIFIED. ) 
 CURVE ( )  GEOMETRIC_REPRESENTATION_ITEM ( )  RATIONAL_B_SPLINE_CURVE ( ( 1.000000000000000000, 0.8047378541243649375, 0.8047378541243649375, 1.000000000000000000 ) ) 
 REPRESENTATION_ITEM ( '' )  );
#24540=DIRECTION ( 'NONE',  ( -0.000000000000000000, -0.000000000000000000, -1.000000000000000000 ) ) ;
#24541=ORIENTED_EDGE ( 'NONE', *, *, #39646, .F. ) ;
#24542=CARTESIAN_POINT ( 'NONE',  ( 71.55402655318506788, 2.143131898507880377E-16, -160.9317124430720298 ) ) ;
#24544=EDGE_LOOP ( 'NONE', ( #15040, #37398, #13671, #18520, #7331 ) ) ;
#24545=DIRECTION ( 'NONE',  ( 0.000000000000000000, 0.000000000000000000, 1.000000000000000000 ) ) ;
#24546=CARTESIAN_POINT ( 'NONE',  ( -128.4459734468149179, 0.000000000000000000, -40.93171244307202983 ) ) ;
#24551=VECTOR ( 'NONE', #40826, 1000.000000000000000 ) ;
#24554=FACE_OUTER_BOUND ( 'NONE', #38099, .T. ) ;
#24558=CARTESIAN_POINT ( 'NONE',  ( 193.3040265531851105, 0.000000000000000000, -165.0000000000000000 ) ) ;
#24559=CARTESIAN_POINT ( 'NONE',  ( -168.4459734468149747, -1.025126265847089213, -0.9317124430720324924 ) ) ;
#24561=ORIENTED_EDGE ( 'NONE', *, *, #24692, .T. ) ;
#24565=CARTESIAN_POINT ( 'NONE',  ( 192.2789002873380184, -1.750000000000010214, 121.8434138227750623 ) ) ;
#24567=DIRECTION ( 'NONE',  ( -0.000000000000000000, -0.000000000000000000, -1.000000000000000000 ) ) ;
#24569=EDGE_CURVE ( 'NONE', #47251, #38939, #46552, .T. ) ;
#24572=ORIENTED_EDGE ( 'NONE', *, *, #5895, .F. ) ;
#24573=ORIENTED_EDGE ( 'NONE', *, *, #9132, .F. ) ;
#24574=EDGE_LOOP ( 'NONE', ( #44027, #14819, #26272, #4753, #3978, #10714 ) ) ;
#24575=DIRECTION ( 'NONE',  ( 0.000000000000000000, 0.000000000000000000, 1.000000000000000000 ) ) ;
#24580=DIRECTION ( 'NONE',  ( -1.000000000000000000, -0.000000000000000000, -0.000000000000000000 ) ) ;
#24581=CARTESIAN_POINT ( 'NONE',  ( 71.55402655318505367, 0.000000000000000000, 165.0000000000000000 ) ) ;
#24585=CARTESIAN_POINT ( 'NONE',  ( -84.94597344681497475, 0.000000000000000000, 162.5682875569279702 ) ) ;
#24587=CARTESIAN_POINT ( 'NONE',  ( -48.44597344681496054, -1.025126265847089213, -0.9317124430720324924 ) ) ;
#24597=EDGE_LOOP ( 'NONE', ( #21173, #28657, #45630, #38257, #47623, #11616 ) ) ;
#24603=ADVANCED_FACE ( 'NONE', ( #31464 ), #47061, .T. ) ;
#24607=ADVANCED_FACE ( 'NONE', ( #4261 ), #43500, .T. ) ;
#24608=VERTEX_POINT ( 'NONE', #924 ) ;
#24609=DIRECTION ( 'NONE',  ( -0.000000000000000000, -0.000000000000000000, -1.000000000000000000 ) ) ;
#24610=ADVANCED_FACE ( 'NONE', ( #36082 ), #16311, .T. ) ;
#24613=ADVANCED_FACE ( 'NONE', ( #32482 ), #5513, .T. ) ;
#24616=CARTESIAN_POINT ( 'NONE',  ( -128.4459734468149463, 1.025126265847081442, 159.0682875569279418 ) ) ;
#24617=EDGE_CURVE ( 'NONE', #37708, #38609, #5941, .T. ) ;
#24624=CARTESIAN_POINT ( 'NONE',  ( 74.32915281903215998, 1.750000000000010214, -80.20683870891910772 ) ) ;
#24635=EDGE_CURVE ( 'NONE', #21159, #35861, #42952, .T. ) ;
#24640=VERTEX_POINT ( 'NONE', #40425 ) ;
#24645=ORIENTED_EDGE ( 'NONE', *, *, #5314, .F. ) ;
#24649=CARTESIAN_POINT ( 'NONE',  ( 153.3040265531850537, 1.750000000000009992, -159.1817124430720298 ) ) ;
#24650=CARTESIAN_POINT ( 'NONE',  ( 151.5540265531850537, 0.000000000000000000, -165.0000000000000000 ) ) ;
#24659=CYLINDRICAL_SURFACE ( 'NONE', #2893, 1.750000000000008438 ) ;
#24661=CARTESIAN_POINT ( 'NONE',  ( -88.44597344681494633, -1.025126265847089657, -80.93171244307201562 ) ) ;
#24663=ORIENTED_EDGE ( 'NONE', *, *, #36311, .F. ) ;
#24666=CARTESIAN_POINT ( 'NONE',  ( -46.69597344681494633, 0.000000000000000000, -165.0000000000000000 ) ) ;
#24668=EDGE_CURVE ( 'NONE', #45714, #16313, #21161, .T. ) ;
#24671=CARTESIAN_POINT ( 'NONE',  ( -46.69597344681494633, -1.750000000000009992, 0.8182875569279768335 ) ) ;
#24676=CARTESIAN_POINT ( 'NONE',  ( 210.0000000000000568, 0.000000000000000000, -159.1817124430720298 ) ) ;
#24678=EDGE_CURVE ( 'NONE', #38516, #47604, #41614, .T. ) ;
#24680=CARTESIAN_POINT ( 'NONE',  ( -206.6959734468149463, 1.750000000000009992, -159.1817124430720298 ) ) ;
#24681=CARTESIAN_POINT ( 'NONE',  ( -4.945973446814903696, 2.143131898507912917E-16, -157.4317124430720014 ) ) ;
#24684=EDGE_CURVE ( 'NONE', #11965, #34539, #6549, .T. ) ;
#24687=CARTESIAN_POINT ( 'NONE',  ( 151.5540265531850537, 2.143131898507880377E-16, -160.9317124430720298 ) ) ;
#24688=CARTESIAN_POINT ( 'NONE',  ( -124.9459734468149321, 1.025126265847081664, 159.0682875569279418 ) ) ;
#24689=CARTESIAN_POINT ( 'NONE',  ( -6.695973446814940111, -1.750000000000023315, -159.1817124430720298 ) ) ;
#24692=EDGE_CURVE ( 'NONE', #44183, #18077, #43262, .T. ) ;
#24693=( BOUNDED_CURVE ( )  B_SPLINE_CURVE ( 3, ( #30215, #19684, #39201, #23268 ),
 .UNSPECIFIED., .F., .F. ) 
 B_SPLINE_CURVE_WITH_KNOTS ( ( 4, 4 ),
 ( 1.570796326794896558, 3.141592653589793116 ),
 .UNSPECIFIED. ) 
 CURVE ( )  GEOMETRIC_REPRESENTATION_ITEM ( )  RATIONAL_B_SPLINE_CURVE ( ( 1.000000000000000000, 0.8047378541243649375, 0.8047378541243649375, 1.000000000000000000 ) ) 
 REPRESENTATION_ITEM ( '' )  );
#24698=ORIENTED_EDGE ( 'NONE', *, *, #1846, .F. ) ;
#24699=EDGE_CURVE ( 'NONE', #6202, #22032, #26281, .T. ) ;
#24702=CARTESIAN_POINT ( 'NONE',  ( 34.32915281903212446, -1.750000000000010436, -120.2068387089191219 ) ) ;
#24704=CARTESIAN_POINT ( 'NONE',  ( -124.9459734468149463, 2.143131898507847836E-16, -77.43171244307204404 ) ) ;
#24712=VERTEX_POINT ( 'NONE', #2904 ) ;
#24713=ORIENTED_EDGE ( 'NONE', *, *, #44379, .F. ) ;
#24715=DIRECTION ( 'NONE',  ( -0.000000000000000000, -0.000000000000000000, -1.000000000000000000 ) ) ;
#24720=ORIENTED_EDGE ( 'NONE', *, *, #5582, .T. ) ;
#24722=ORIENTED_EDGE ( 'NONE', *, *, #49891, .T. ) ;
#24724=DIRECTION ( 'NONE',  ( 0.000000000000000000, 0.000000000000000000, -1.000000000000000000 ) ) ;
#24729=ORIENTED_EDGE ( 'NONE', *, *, #46847, .T. ) ;
#24736=ORIENTED_EDGE ( 'NONE', *, *, #22781, .T. ) ;
#24741=CARTESIAN_POINT ( 'NONE',  ( 115.0540265531850395, 1.025126265847082108, 122.5682875569279702 ) ) ;
#24747=EDGE_CURVE ( 'NONE', #12693, #16975, #2177, .T. ) ;
#24751=CARTESIAN_POINT ( 'NONE',  ( -208.4459734468149463, 0.000000000000000000, 42.56828755692798438 ) ) ;
#24758=CARTESIAN_POINT ( 'NONE',  ( 154.3291528190321458, -1.750000000000009548, -0.2068387089191121020 ) ) ;
#24760=VERTEX_POINT ( 'NONE', #45988 ) ;
#24770=VERTEX_POINT ( 'NONE', #2665 ) ;
#24777=EDGE_LOOP ( 'NONE', ( #33784, #43547, #18853, #42879, #17164, #42716 ) ) ;
#24779=AXIS2_PLACEMENT_3D ( 'NONE', #36040, #28069, #8578 ) ;
#24784=DIRECTION ( 'NONE',  ( -1.000000000000000000, 0.000000000000000000, 0.000000000000000000 ) ) ;
#24788=DIRECTION ( 'NONE',  ( 1.000000000000000000, 0.000000000000000000, -0.000000000000000000 ) ) ;
#24802=EDGE_CURVE ( 'NONE', #46959, #29991, #1321, .T. ) ;
#24804=CARTESIAN_POINT ( 'NONE',  ( 33.30402655318503946, -1.750000000000009992, 0.8182875569279768335 ) ) ;
#24810=AXIS2_PLACEMENT_3D ( 'NONE', #49479, #14372, #30039 ) ;
#24823=( BOUNDED_CURVE ( )  B_SPLINE_CURVE ( 3, ( #27766, #24181, #23912, #35745 ),
 .UNSPECIFIED., .F., .F. ) 
 B_SPLINE_CURVE_WITH_KNOTS ( ( 4, 4 ),
 ( 1.570796326794896558, 3.141592653589793116 ),
 .UNSPECIFIED. ) 
 CURVE ( )  GEOMETRIC_REPRESENTATION_ITEM ( )  RATIONAL_B_SPLINE_CURVE ( ( 1.000000000000000000, 0.8047378541243649375, 0.8047378541243649375, 1.000000000000000000 ) ) 
 REPRESENTATION_ITEM ( '' )  );
#24828=ORIENTED_EDGE ( 'NONE', *, *, #24859, .T. ) ;
#24830=FACE_OUTER_BOUND ( 'NONE', #49426, .T. ) ;
#24831=( BOUNDED_CURVE ( )  B_SPLINE_CURVE ( 3, ( #39196, #29152, #48851, #44513 ),
 .UNSPECIFIED., .F., .F. ) 
 B_SPLINE_CURVE_WITH_KNOTS ( ( 4, 4 ),
 ( 3.141592653589793116, 4.712388980384689674 ),
 .UNSPECIFIED. ) 
 CURVE ( )  GEOMETRIC_REPRESENTATION_ITEM ( )  RATIONAL_B_SPLINE_CURVE ( ( 1.000000000000000000, 0.8047378541243649375, 0.8047378541243649375, 1.000000000000000000 ) ) 
 REPRESENTATION_ITEM ( '' )  );
#24834=EDGE_CURVE ( 'NONE', #47416, #30683, #4200, .T. ) ;
#24835=LINE ( 'NONE', #17377, #3661 ) ;
#24845=CARTESIAN_POINT ( 'NONE',  ( -8.445973446814976526, 0.000000000000000000, 165.0000000000000000 ) ) ;
#24847=FACE_OUTER_BOUND ( 'NONE', #5685, .T. ) ;
#24852=CARTESIAN_POINT ( 'NONE',  ( -167.7210997126620384, -1.750000000000009548, 1.843413822775065825 ) ) ;
#24859=EDGE_CURVE ( 'NONE', #8676, #20584, #13440, .T. ) ;
#24862=ORIENTED_EDGE ( 'NONE', *, *, #38287, .T. ) ;
#24863=CARTESIAN_POINT ( 'NONE',  ( 31.55402655318503236, -1.025126265847089879, -117.4317124430720156 ) ) ;
#24864=VERTEX_POINT ( 'NONE', #26788 ) ;
#24870=VERTEX_POINT ( 'NONE', #50071 ) ;
#24872=CARTESIAN_POINT ( 'NONE',  ( 210.0000000000000568, 2.143131898507881856E-16, 119.0682875569279560 ) ) ;
#24876=ADVANCED_FACE ( 'NONE', ( #47256 ), #50332, .T. ) ;
#24894=ADVANCED_FACE ( 'NONE', ( #34494 ), #39114, .T. ) ;
#24896=LINE ( 'NONE', #48442, #18190 ) ;
#24900=DIRECTION ( 'NONE',  ( -0.000000000000000000, -0.000000000000000000, -1.000000000000000000 ) ) ;
#24905=ORIENTED_EDGE ( 'NONE', *, *, #49279, .T. ) ;
#24906=VERTEX_POINT ( 'NONE', #46743 ) ;
#24913=ORIENTED_EDGE ( 'NONE', *, *, #49509, .F. ) ;
#24927=CARTESIAN_POINT ( 'NONE',  ( -208.4459734468149463, 0.000000000000000000, -37.43171244307205825 ) ) ;
#24931=CARTESIAN_POINT ( 'NONE',  ( -206.6959734468149463, -1.750000000000009992, -159.1817124430720298 ) ) ;
#24933=ORIENTED_EDGE ( 'NONE', *, *, #37119, .F. ) ;
#24936=CARTESIAN_POINT ( 'NONE',  ( -7.721099712662037540, 1.750000000000023315, 39.79316129108089228 ) ) ;
#24940=DIRECTION ( 'NONE',  ( -0.000000000000000000, -0.000000000000000000, -1.000000000000000000 ) ) ;
#24948=VECTOR ( 'NONE', #3727, 1000.000000000000000 ) ;
#24949=DIRECTION ( 'NONE',  ( -1.000000000000000000, -0.000000000000000000, -0.000000000000000000 ) ) ;
#24952=CYLINDRICAL_SURFACE ( 'NONE', #43410, 1.750000000000008438 ) ;
#24955=VERTEX_POINT ( 'NONE', #20093 ) ;
#24957=CARTESIAN_POINT ( 'NONE',  ( -124.9459734468149321, 1.025126265847081886, -40.93171244307202272 ) ) ;
#24965=CARTESIAN_POINT ( 'NONE',  ( -166.6959734468149463, -1.750000000000010658, -119.1817124430720440 ) ) ;
#24974=ORIENTED_EDGE ( 'NONE', *, *, #1369, .T. ) ;
#24979=LINE ( 'NONE', #44195, #45484 ) ;
#24982=DIRECTION ( 'NONE',  ( -1.000000000000000000, -0.000000000000000000, -0.000000000000000000 ) ) ;
#24987=EDGE_LOOP ( 'NONE', ( #29526, #9247, #20128, #11719, #37579, #33596 ) ) ;
#24989=VECTOR ( 'NONE', #5745, 1000.000000000000000 ) ;
#24992=CARTESIAN_POINT ( 'NONE',  ( 111.5540265531850679, 0.000000000000000000, 159.0682875569279702 ) ) ;
#24994=( BOUNDED_CURVE ( )  B_SPLINE_CURVE ( 3, ( #50431, #43020, #23544, #38199 ),
 .UNSPECIFIED., .F., .F. ) 
 B_SPLINE_CURVE_WITH_KNOTS ( ( 4, 4 ),
 ( 4.712388980384689674, 6.283185307179586232 ),
 .UNSPECIFIED. ) 
 CURVE ( )  GEOMETRIC_REPRESENTATION_ITEM ( )  RATIONAL_B_SPLINE_CURVE ( ( 1.000000000000000000, 0.8047378541243649375, 0.8047378541243649375, 1.000000000000000000 ) ) 
 REPRESENTATION_ITEM ( '' )  );
#24995=CARTESIAN_POINT ( 'NONE',  ( 191.5540265531851105, 0.000000000000000000, 2.568287556927978166 ) ) ;
#24996=AXIS2_PLACEMENT_3D ( 'NONE', #30255, #33864, #49949 ) ;
#25000=CARTESIAN_POINT ( 'NONE',  ( -208.4459734468149463, 0.000000000000000000, 165.0000000000000000 ) ) ;
#25001=EDGE_CURVE ( 'NONE', #21151, #12850, #48463, .T. ) ;
#25003=ORIENTED_EDGE ( 'NONE', *, *, #242, .T. ) ;
#25006=AXIS2_PLACEMENT_3D ( 'NONE', #9705, #29975, #48909 ) ;
#25011=CARTESIAN_POINT ( 'NONE',  ( 35.05402655318504657, -1.025126265847089435, -77.43171244307200141 ) ) ;
#25013=ORIENTED_EDGE ( 'NONE', *, *, #46143, .T. ) ;
#25015=ORIENTED_EDGE ( 'NONE', *, *, #7489, .T. ) ;
#25016=ORIENTED_EDGE ( 'NONE', *, *, #31517, .F. ) ;
#25025=CARTESIAN_POINT ( 'NONE',  ( -164.9459734468149463, -1.025126265847089213, -0.9317124430720324924 ) ) ;
#25026=CARTESIAN_POINT ( 'NONE',  ( 113.3040265531850537, 1.749999999999997113, -39.18171244307202983 ) ) ;
#25029=VERTEX_POINT ( 'NONE', #9307 ) ;
#25032=CARTESIAN_POINT ( 'NONE',  ( 34.32915281903212446, -1.750000000000010436, 79.79316129108087807 ) ) ;
#25034=ORIENTED_EDGE ( 'NONE', *, *, #11131, .F. ) ;
#25040=LINE ( 'NONE', #17324, #371 ) ;
#25041=ORIENTED_EDGE ( 'NONE', *, *, #19909, .F. ) ;
#25043=CARTESIAN_POINT ( 'NONE',  ( -46.69597344681494633, -1.750000000000009992, 160.8182875569279702 ) ) ;
#25047=AXIS2_PLACEMENT_3D ( 'NONE', #22759, #38431, #3245 ) ;
#25049=CARTESIAN_POINT ( 'NONE',  ( -206.6959734468149463, -1.750000000000010658, 120.8182875569279702 ) ) ;
#25051=CARTESIAN_POINT ( 'NONE',  ( 155.0540265531850537, 1.025126265847089213, -160.9317124430720014 ) ) ;
#25053=FACE_OUTER_BOUND ( 'NONE', #8624, .T. ) ;
#25056=AXIS2_PLACEMENT_3D ( 'NONE', #46106, #10999, #26900 ) ;
#25057=CYLINDRICAL_SURFACE ( 'NONE', #23728, 1.750000000000015543 ) ;
#25058=DIRECTION ( 'NONE',  ( 0.000000000000000000, 0.000000000000000000, 1.000000000000000000 ) ) ;
#25062=CARTESIAN_POINT ( 'NONE',  ( 210.0000000000000568, 2.143131898507880377E-16, 159.0682875569279702 ) ) ;
#25064=VECTOR ( 'NONE', #14540, 1000.000000000000000 ) ;
#25065=ADVANCED_FACE ( 'NONE', ( #37538 ), #3299, .T. ) ;
#25066=CARTESIAN_POINT ( 'NONE',  ( 33.30402655318503946, -1.750000000000010658, -119.1817124430720440 ) ) ;
#25070=( BOUNDED_CURVE ( )  B_SPLINE_CURVE ( 3, ( #2016, #17658, #1517, #48908 ),
 .UNSPECIFIED., .F., .F. ) 
 B_SPLINE_CURVE_WITH_KNOTS ( ( 4, 4 ),
 ( 3.141592653589793116, 4.712388980384689674 ),
 .UNSPECIFIED. ) 
 CURVE ( )  GEOMETRIC_REPRESENTATION_ITEM ( )  RATIONAL_B_SPLINE_CURVE ( ( 1.000000000000000000, 0.8047378541243649375, 0.8047378541243649375, 1.000000000000000000 ) ) 
 REPRESENTATION_ITEM ( '' )  );
#25075=FACE_OUTER_BOUND ( 'NONE', #4988, .T. ) ;
#25080=CARTESIAN_POINT ( 'NONE',  ( -84.94597344681494633, 2.143131898507880377E-16, 2.568287556927978166 ) ) ;
#25083=ORIENTED_EDGE ( 'NONE', *, *, #45211, .F. ) ;
#25089=EDGE_CURVE ( 'NONE', #43884, #41782, #49795, .T. ) ;
#25090=CARTESIAN_POINT ( 'NONE',  ( 35.05402655318504657, 2.143131898507880377E-16, 159.0682875569279702 ) ) ;
#25091=CARTESIAN_POINT ( 'NONE',  ( 74.32915281903215998, 1.750000000000009326, 161.8434138227750907 ) ) ;
#25093=VECTOR ( 'NONE', #6329, 1000.000000000000000 ) ;
#25098=CARTESIAN_POINT ( 'NONE',  ( -204.9459734468149463, 2.143131898507880377E-16, -80.93171244307201562 ) ) ;
#25099=ADVANCED_FACE ( 'NONE', ( #50201 ), #34621, .T. ) ;
#25100=DIRECTION ( 'NONE',  ( 0.000000000000000000, 0.000000000000000000, -1.000000000000000000 ) ) ;
#25104=DIRECTION ( 'NONE',  ( -0.000000000000000000, -0.000000000000000000, -1.000000000000000000 ) ) ;
#25109=CARTESIAN_POINT ( 'NONE',  ( -165.6708471809677974, -1.750000000000009326, 159.7931612910809065 ) ) ;
#25110=VERTEX_POINT ( 'NONE', #15113 ) ;
#25113=PLANE ( 'NONE',  #42591 ) ;
#25123=ADVANCED_FACE ( 'NONE', ( #33182 ), #46383, .T. ) ;
#25124=( BOUNDED_CURVE ( )  B_SPLINE_CURVE ( 3, ( #17845, #49356, #45525, #18839 ),
 .UNSPECIFIED., .F., .F. ) 
 B_SPLINE_CURVE_WITH_KNOTS ( ( 4, 4 ),
 ( 1.570796326794896558, 3.141592653589793116 ),
 .UNSPECIFIED. ) 
 CURVE ( )  GEOMETRIC_REPRESENTATION_ITEM ( )  RATIONAL_B_SPLINE_CURVE ( ( 1.000000000000000000, 0.8047378541243649375, 0.8047378541243649375, 1.000000000000000000 ) ) 
 REPRESENTATION_ITEM ( '' )  );
#25128=CARTESIAN_POINT ( 'NONE',  ( -88.44597344681497475, 0.000000000000000000, 122.5682875569279986 ) ) ;
#25131=ORIENTED_EDGE ( 'NONE', *, *, #10352, .T. ) ;
#25141=CARTESIAN_POINT ( 'NONE',  ( -8.445973446814976526, 0.000000000000000000, 2.568287556928034121 ) ) ;
#25144=ORIENTED_EDGE ( 'NONE', *, *, #42546, .T. ) ;
#25146=CARTESIAN_POINT ( 'NONE',  ( -166.6959734468149463, 0.000000000000000000, 165.0000000000000000 ) ) ;
#25147=FACE_OUTER_BOUND ( 'NONE', #10632, .T. ) ;
#25150=DIRECTION ( 'NONE',  ( 1.000000000000000000, 0.000000000000000000, 0.000000000000000000 ) ) ;
#25155=EDGE_CURVE ( 'NONE', #9119, #19888, #23936, .T. ) ;
#25164=VERTEX_POINT ( 'NONE', #14145 ) ;
#25167=CARTESIAN_POINT ( 'NONE',  ( -208.4459734468149463, 0.000000000000000000, 165.0000000000000000 ) ) ;
#25170=ORIENTED_EDGE ( 'NONE', *, *, #22507, .F. ) ;
#25172=ORIENTED_EDGE ( 'NONE', *, *, #21102, .T. ) ;
#25178=CYLINDRICAL_SURFACE ( 'NONE', #765, 1.750000000000015543 ) ;
#25180=ORIENTED_EDGE ( 'NONE', *, *, #50337, .T. ) ;
#25183=CARTESIAN_POINT ( 'NONE',  ( 73.30402655318508209, 0.000000000000000000, 165.0000000000000000 ) ) ;
#25194=CARTESIAN_POINT ( 'NONE',  ( 151.5540265531850537, -1.025126265847089657, 79.06828755692797017 ) ) ;
#25196=ORIENTED_EDGE ( 'NONE', *, *, #48677, .F. ) ;
#25197=DIRECTION ( 'NONE',  ( -1.000000000000000000, 0.000000000000000000, 0.000000000000000000 ) ) ;
#25198=CARTESIAN_POINT ( 'NONE',  ( -125.6708471809678542, 1.749999999999996669, -40.20683870891911482 ) ) ;
#25203=EDGE_CURVE ( 'NONE', #50033, #41657, #48160, .T. ) ;
#25204=ORIENTED_EDGE ( 'NONE', *, *, #35539, .F. ) ;
#25211=ORIENTED_EDGE ( 'NONE', *, *, #28650, .T. ) ;
#25213=CARTESIAN_POINT ( 'NONE',  ( -84.94597344681494633, 2.143131898507880377E-16, 39.06828755692798438 ) ) ;
#25214=EDGE_LOOP ( 'NONE', ( #3151, #1651, #743, #42600, #42172, #40545 ) ) ;
#25218=CARTESIAN_POINT ( 'NONE',  ( -5.670847180967843570, -1.750000000000023981, 119.7931612910808781 ) ) ;
#25225=CARTESIAN_POINT ( 'NONE',  ( -210.0000000000000568, 0.000000000000000000, 80.81828755692798438 ) ) ;
#25230=CARTESIAN_POINT ( 'NONE',  ( -44.94597344681493922, 1.025126265847089879, 82.56828755692798438 ) ) ;
#25231=CARTESIAN_POINT ( 'NONE',  ( 75.05402655318509630, -1.025126265847088991, 2.568287556927986159 ) ) ;
#25244=EDGE_CURVE ( 'NONE', #26079, #7763, #27933, .T. ) ;
#25247=DIRECTION ( 'NONE',  ( -1.000000000000000000, 0.000000000000000000, 0.000000000000000000 ) ) ;
#25248=DIRECTION ( 'NONE',  ( -0.000000000000000000, -0.000000000000000000, -1.000000000000000000 ) ) ;
#25249=ORIENTED_EDGE ( 'NONE', *, *, #26127, .F. ) ;
#25250=VERTEX_POINT ( 'NONE', #35400 ) ;
#25252=DIRECTION ( 'NONE',  ( -0.000000000000000000, -0.000000000000000000, -1.000000000000000000 ) ) ;
#25253=CARTESIAN_POINT ( 'NONE',  ( 34.32915281903212446, 1.750000000000009548, 159.7931612910809065 ) ) ;
#25254=CARTESIAN_POINT ( 'NONE',  ( 113.3040265531850537, -1.749999999999997335, 80.81828755692798438 ) ) ;
#25258=EDGE_CURVE ( 'NONE', #30782, #9269, #11206, .T. ) ;
#25259=CARTESIAN_POINT ( 'NONE',  ( 31.55402655318506788, 2.143131898507880377E-16, -160.9317124430720298 ) ) ;
#25262=EDGE_CURVE ( 'NONE', #9366, #25957, #41017, .T. ) ;
#25263=EDGE_CURVE ( 'NONE', #41151, #28572, #16376, .T. ) ;
#25264=ORIENTED_EDGE ( 'NONE', *, *, #12214, .F. ) ;
#25270=FACE_OUTER_BOUND ( 'NONE', #37406, .T. ) ;
#25271=DIRECTION ( 'NONE',  ( -1.000000000000000000, 0.000000000000000000, 0.000000000000000000 ) ) ;
#25276=CARTESIAN_POINT ( 'NONE',  ( 155.0540265531850537, 2.143131898507880377E-16, -157.4317124430720582 ) ) ;
#25277=CARTESIAN_POINT ( 'NONE',  ( 151.5540265531850537, 0.000000000000000000, 2.568287556927978166 ) ) ;
#25280=DIRECTION ( 'NONE',  ( -1.000000000000000000, -0.000000000000000000, -0.000000000000000000 ) ) ;
#25281=CARTESIAN_POINT ( 'NONE',  ( 210.0000000000000568, 0.000000000000000000, 40.81828755692798438 ) ) ;
#25282=( BOUNDED_CURVE ( )  B_SPLINE_CURVE ( 3, ( #35890, #19712, #35391, #4574 ),
 .UNSPECIFIED., .F., .F. ) 
 B_SPLINE_CURVE_WITH_KNOTS ( ( 4, 4 ),
 ( 4.712388980384689674, 6.283185307179586232 ),
 .UNSPECIFIED. ) 
 CURVE ( )  GEOMETRIC_REPRESENTATION_ITEM ( )  RATIONAL_B_SPLINE_CURVE ( ( 1.000000000000000000, 0.8047378541243649375, 0.8047378541243649375, 1.000000000000000000 ) ) 
 REPRESENTATION_ITEM ( '' )  );
#25287=CARTESIAN_POINT ( 'NONE',  ( -4.945973446814903696, 2.143131898507912917E-16, 165.0000000000000000 ) ) ;
#25293=ORIENTED_EDGE ( 'NONE', *, *, #42556, .T. ) ;
#25305=VERTEX_POINT ( 'NONE', #44065 ) ;
#25309=EDGE_CURVE ( 'NONE', #2518, #29162, #18372, .T. ) ;
#25312=DIRECTION ( 'NONE',  ( -1.000000000000000000, -0.000000000000000000, -0.000000000000000000 ) ) ;
#25315=EDGE_CURVE ( 'NONE', #40327, #38568, #29188, .T. ) ;
#25316=CARTESIAN_POINT ( 'NONE',  ( 191.5540265531850537, -1.025126265847089879, 122.5682875569280128 ) ) ;
#25326=ORIENTED_EDGE ( 'NONE', *, *, #17326, .T. ) ;
#25328=CARTESIAN_POINT ( 'NONE',  ( -6.695973446814940111, 0.000000000000000000, 165.0000000000000000 ) ) ;
#25329=AXIS2_PLACEMENT_3D ( 'NONE', #9004, #48455, #29000 ) ;
#25333=AXIS2_PLACEMENT_3D ( 'NONE', #50520, #7488, #46174 ) ;
#25342=CARTESIAN_POINT ( 'NONE',  ( -164.9459734468149463, 2.143131898507880377E-16, 165.0000000000000000 ) ) ;
#25347=EDGE_LOOP ( 'NONE', ( #4707, #8323, #42085, #49812, #44270, #47014 ) ) ;
#25348=CARTESIAN_POINT ( 'NONE',  ( -204.9459734468148895, -1.025126265847089435, 82.56828755692798438 ) ) ;
#25349=CARTESIAN_POINT ( 'NONE',  ( 210.0000000000000568, 0.000000000000000000, -159.1817124430720298 ) ) ;
#25351=AXIS2_PLACEMENT_3D ( 'NONE', #21242, #2247, #9695 ) ;
#25352=ORIENTED_EDGE ( 'NONE', *, *, #28077, .F. ) ;
#25363=EDGE_CURVE ( 'NONE', #41350, #1434, #13021, .T. ) ;
#25365=DIRECTION ( 'NONE',  ( -1.000000000000000000, -0.000000000000000000, -0.000000000000000000 ) ) ;
#25370=EDGE_CURVE ( 'NONE', #30782, #43794, #4308, .T. ) ;
#25374=DIRECTION ( 'NONE',  ( -1.000000000000000000, -0.000000000000000000, -0.000000000000000000 ) ) ;
#25375=ORIENTED_EDGE ( 'NONE', *, *, #37108, .T. ) ;
#25377=CARTESIAN_POINT ( 'NONE',  ( 31.55402655318503236, 0.000000000000000000, -0.9317124430720247208 ) ) ;
#25384=VERTEX_POINT ( 'NONE', #9685 ) ;
#25389=ORIENTED_EDGE ( 'NONE', *, *, #38703, .T. ) ;
#25395=CARTESIAN_POINT ( 'NONE',  ( 35.05402655318504657, 2.143131898507880377E-16, -77.43171244307198720 ) ) ;
#25396=PLANE ( 'NONE',  #8234 ) ;
#25412=CARTESIAN_POINT ( 'NONE',  ( 210.0000000000000568, 0.000000000000000000, -39.18171244307202983 ) ) ;
#25414=DIRECTION ( 'NONE',  ( -1.000000000000000000, 0.000000000000000000, 0.000000000000000000 ) ) ;
#25415=CYLINDRICAL_SURFACE ( 'NONE', #9785, 1.750000000000008438 ) ;
#25419=( BOUNDED_CURVE ( )  B_SPLINE_CURVE ( 3, ( #23570, #8926, #28184, #43813 ),
 .UNSPECIFIED., .F., .F. ) 
 B_SPLINE_CURVE_WITH_KNOTS ( ( 4, 4 ),
 ( 0.000000000000000000, 1.570796326794896558 ),
 .UNSPECIFIED. ) 
 CURVE ( )  GEOMETRIC_REPRESENTATION_ITEM ( )  RATIONAL_B_SPLINE_CURVE ( ( 1.000000000000000000, 0.8047378541243649375, 0.8047378541243649375, 1.000000000000000000 ) ) 
 REPRESENTATION_ITEM ( '' )  );
#25420=ORIENTED_EDGE ( 'NONE', *, *, #41182, .F. ) ;
#25424=DIRECTION ( 'NONE',  ( -1.000000000000000000, 0.000000000000000000, 0.000000000000000000 ) ) ;
#25426=( BOUNDED_CURVE ( )  B_SPLINE_CURVE ( 3, ( #6870, #17894, #29215, #45079 ),
 .UNSPECIFIED., .F., .F. ) 
 B_SPLINE_CURVE_WITH_KNOTS ( ( 4, 4 ),
 ( 0.000000000000000000, 1.570796326794896558 ),
 .UNSPECIFIED. ) 
 CURVE ( )  GEOMETRIC_REPRESENTATION_ITEM ( )  RATIONAL_B_SPLINE_CURVE ( ( 1.000000000000000000, 0.8047378541243649375, 0.8047378541243649375, 1.000000000000000000 ) ) 
 REPRESENTATION_ITEM ( '' )  );
#25429=AXIS2_PLACEMENT_3D ( 'NONE', #17414, #28276, #585 ) ;
#25431=DIRECTION ( 'NONE',  ( -0.000000000000000000, -0.000000000000000000, -1.000000000000000000 ) ) ;
#25432=ORIENTED_EDGE ( 'NONE', *, *, #29025, .F. ) ;
#25435=CARTESIAN_POINT ( 'NONE',  ( -166.6959734468149463, 1.750000000000010658, -119.1817124430720440 ) ) ;
#25437=EDGE_CURVE ( 'NONE', #9119, #2781, #7106, .T. ) ;
#25439=CYLINDRICAL_SURFACE ( 'NONE', #14847, 1.749999999999987566 ) ;
#25444=DIRECTION ( 'NONE',  ( 0.000000000000000000, 0.000000000000000000, 1.000000000000000000 ) ) ;
#25453=CARTESIAN_POINT ( 'NONE',  ( 195.0540265531851105, 2.143131898507880377E-16, -77.43171244307204404 ) ) ;
#25456=CARTESIAN_POINT ( 'NONE',  ( 114.3291528190321173, -1.749999999999996891, 39.79316129108089228 ) ) ;
#25459=FACE_OUTER_BOUND ( 'NONE', #41908, .T. ) ;
#25462=DIRECTION ( 'NONE',  ( -0.000000000000000000, -0.000000000000000000, -1.000000000000000000 ) ) ;
#25464=EDGE_LOOP ( 'NONE', ( #47345, #29607, #16756, #18480, #30521, #7873 ) ) ;
#25467=VECTOR ( 'NONE', #37884, 1000.000000000000000 ) ;
#25472=CARTESIAN_POINT ( 'NONE',  ( 210.0000000000000568, 0.000000000000000000, -119.1817124430720440 ) ) ;
#25476=CARTESIAN_POINT ( 'NONE',  ( 72.27890028733797578, -1.750000000000009548, 39.79316129108089228 ) ) ;
#25483=ORIENTED_EDGE ( 'NONE', *, *, #42791, .T. ) ;
#25493=ORIENTED_EDGE ( 'NONE', *, *, #47145, .T. ) ;
#25494=CYLINDRICAL_SURFACE ( 'NONE', #26709, 1.750000000000008438 ) ;
#25498=EDGE_CURVE ( 'NONE', #25957, #8816, #34437, .T. ) ;
#25499=ORIENTED_EDGE ( 'NONE', *, *, #6040, .F. ) ;
#25500=ORIENTED_EDGE ( 'NONE', *, *, #11533, .F. ) ;
#25502=DIRECTION ( 'NONE',  ( -0.000000000000000000, -0.000000000000000000, -1.000000000000000000 ) ) ;
#25507=VECTOR ( 'NONE', #9942, 1000.000000000000000 ) ;
#25508=EDGE_CURVE ( 'NONE', #13625, #33144, #14025, .T. ) ;
#25510=AXIS2_PLACEMENT_3D ( 'NONE', #47721, #8784, #20568 ) ;
#25511=EDGE_CURVE ( 'NONE', #36401, #45850, #2641, .T. ) ;
#25512=CARTESIAN_POINT ( 'NONE',  ( 195.0540265531851105, 2.143131898507880377E-16, 79.06828755692797017 ) ) ;
#25513=EDGE_LOOP ( 'NONE', ( #24698, #13136, #45275, #4318, #12647, #9473 ) ) ;
#25515=DIRECTION ( 'NONE',  ( -1.000000000000000000, -0.000000000000000000, -0.000000000000000000 ) ) ;
#25516=CARTESIAN_POINT ( 'NONE',  ( 153.3040265531850537, 1.750000000000009992, 0.8182875569279768335 ) ) ;
#25519=EDGE_CURVE ( 'NONE', #29900, #15646, #26352, .T. ) ;
#25526=DIRECTION ( 'NONE',  ( -1.000000000000000000, -0.000000000000000000, -0.000000000000000000 ) ) ;
#25535=EDGE_CURVE ( 'NONE', #25772, #11761, #13138, .T. ) ;
#25536=CARTESIAN_POINT ( 'NONE',  ( 33.30402655318503946, -1.750000000000010658, -119.1817124430720440 ) ) ;
#25537=CARTESIAN_POINT ( 'NONE',  ( 73.30402655318508209, 1.750000000000010658, -119.1817124430720440 ) ) ;
#25543=CARTESIAN_POINT ( 'NONE',  ( -208.4459734468149463, 0.000000000000000000, 119.0682875569279702 ) ) ;
#25545=EDGE_CURVE ( 'NONE', #14624, #40520, #47582, .T. ) ;
#25550=ADVANCED_FACE ( 'NONE', ( #12215 ), #3483, .T. ) ;
#25552=DIRECTION ( 'NONE',  ( -1.000000000000000000, -0.000000000000000000, -0.000000000000000000 ) ) ;
#25553=CARTESIAN_POINT ( 'NONE',  ( -126.6959734468149321, -1.749999999999997113, 40.81828755692798438 ) ) ;
#25554=CARTESIAN_POINT ( 'NONE',  ( -164.9459734468149463, 2.143131898507880377E-16, 165.0000000000000000 ) ) ;
#25557=VERTEX_POINT ( 'NONE', #46816 ) ;
#25558=CARTESIAN_POINT ( 'NONE',  ( -168.4459734468149463, 0.000000000000000000, -37.43171244307205825 ) ) ;
#25560=DIRECTION ( 'NONE',  ( -1.000000000000000000, -0.000000000000000000, -0.000000000000000000 ) ) ;
#25562=ORIENTED_EDGE ( 'NONE', *, *, #27738, .T. ) ;
#25563=CARTESIAN_POINT ( 'NONE',  ( -166.6959734468149463, 1.750000000000010658, 120.8182875569279702 ) ) ;
#25564=DIRECTION ( 'NONE',  ( -1.000000000000000000, -0.000000000000000000, -0.000000000000000000 ) ) ;
#25567=( BOUNDED_CURVE ( )  B_SPLINE_CURVE ( 3, ( #17878, #49399, #25849, #10950 ),
 .UNSPECIFIED., .F., .F. ) 
 B_SPLINE_CURVE_WITH_KNOTS ( ( 4, 4 ),
 ( 3.141592653589793116, 4.712388980384689674 ),
 .UNSPECIFIED. ) 
 CURVE ( )  GEOMETRIC_REPRESENTATION_ITEM ( )  RATIONAL_B_SPLINE_CURVE ( ( 1.000000000000000000, 0.8047378541243649375, 0.8047378541243649375, 1.000000000000000000 ) ) 
 REPRESENTATION_ITEM ( '' )  );
#25572=CARTESIAN_POINT ( 'NONE',  ( 33.30402655318503946, -1.750000000000010658, 120.8182875569279702 ) ) ;
#25580=EDGE_CURVE ( 'NONE', #16448, #20559, #9546, .T. ) ;
#25581=ORIENTED_EDGE ( 'NONE', *, *, #36530, .T. ) ;
#25582=CARTESIAN_POINT ( 'NONE',  ( 33.30402655318503946, 0.000000000000000000, 165.0000000000000000 ) ) ;
#25583=CARTESIAN_POINT ( 'NONE',  ( 112.2789002873379758, -1.749999999999996891, 121.8434138227750481 ) ) ;
#25584=( BOUNDED_CURVE ( )  B_SPLINE_CURVE ( 3, ( #9936, #9433, #44066, #25098 ),
 .UNSPECIFIED., .F., .F. ) 
 B_SPLINE_CURVE_WITH_KNOTS ( ( 4, 4 ),
 ( 4.712388980384689674, 6.283185307179586232 ),
 .UNSPECIFIED. ) 
 CURVE ( )  GEOMETRIC_REPRESENTATION_ITEM ( )  RATIONAL_B_SPLINE_CURVE ( ( 1.000000000000000000, 0.8047378541243649375, 0.8047378541243649375, 1.000000000000000000 ) ) 
 REPRESENTATION_ITEM ( '' )  );
#25585=CARTESIAN_POINT ( 'NONE',  ( 113.3040265531850537, 1.749999999999997113, -39.18171244307202983 ) ) ;
#25586=EDGE_LOOP ( 'NONE', ( #42825, #35048 ) ) ;
#25588=CARTESIAN_POINT ( 'NONE',  ( -85.67084718096784002, -1.750000000000009548, 161.8434138227750907 ) ) ;
#25594=ADVANCED_FACE ( 'NONE', ( #43258 ), #425, .T. ) ;
#25596=AXIS2_PLACEMENT_3D ( 'NONE', #20080, #35766, #36514 ) ;
#25598=CARTESIAN_POINT ( 'NONE',  ( -46.69597344681494633, 0.000000000000000000, 165.0000000000000000 ) ) ;
#25600=EDGE_CURVE ( 'NONE', #3985, #37708, #25040, .T. ) ;
#25603=AXIS2_PLACEMENT_3D ( 'NONE', #36916, #32794, #21228 ) ;
#25606=AXIS2_PLACEMENT_3D ( 'NONE', #32795, #12775, #40490 ) ;
#25608=CARTESIAN_POINT ( 'NONE',  ( 153.3040265531850537, 1.750000000000010214, 40.81828755692798438 ) ) ;
#25612=EDGE_CURVE ( 'NONE', #47251, #34400, #47011, .T. ) ;
#25614=CYLINDRICAL_SURFACE ( 'NONE', #830, 1.750000000000015543 ) ;
#25615=ORIENTED_EDGE ( 'NONE', *, *, #29922, .T. ) ;
#25618=CARTESIAN_POINT ( 'NONE',  ( -124.9459734468149463, 2.143131898507847836E-16, 2.568287556927950632 ) ) ;
#25624=ORIENTED_EDGE ( 'NONE', *, *, #45469, .T. ) ;
#25628=LINE ( 'NONE', #17169, #47788 ) ;
#25629=( BOUNDED_CURVE ( )  B_SPLINE_CURVE ( 3, ( #24283, #31737, #31471, #43506 ),
 .UNSPECIFIED., .F., .F. ) 
 B_SPLINE_CURVE_WITH_KNOTS ( ( 4, 4 ),
 ( 3.141592653589793116, 4.712388980384689674 ),
 .UNSPECIFIED. ) 
 CURVE ( )  GEOMETRIC_REPRESENTATION_ITEM ( )  RATIONAL_B_SPLINE_CURVE ( ( 1.000000000000000000, 0.8047378541243649375, 0.8047378541243649375, 1.000000000000000000 ) ) 
 REPRESENTATION_ITEM ( '' )  );
#25633=CARTESIAN_POINT ( 'NONE',  ( -4.945973446814916130, -1.025126265847097207, -77.43171244307197298 ) ) ;
#25636=VERTEX_POINT ( 'NONE', #935 ) ;
#25637=CARTESIAN_POINT ( 'NONE',  ( -210.0000000000000568, 2.143131898507890731E-16, -160.9317124430720298 ) ) ;
#25640=ORIENTED_EDGE ( 'NONE', *, *, #31719, .T. ) ;
#25648=DIRECTION ( 'NONE',  ( 0.000000000000000000, 0.000000000000000000, 1.000000000000000000 ) ) ;
#25651=CARTESIAN_POINT ( 'NONE',  ( 210.0000000000000568, 0.000000000000000000, 160.8182875569279702 ) ) ;
#25654=ADVANCED_FACE ( 'NONE', ( #32730 ), #16576, .T. ) ;
#25655=CARTESIAN_POINT ( 'NONE',  ( 113.3040265531850537, 1.749999999999997113, 40.81828755692798438 ) ) ;
#25656=ADVANCED_FACE ( 'NONE', ( #12717 ), #44254, .T. ) ;
#25663=ORIENTED_EDGE ( 'NONE', *, *, #39322, .F. ) ;
#25664=EDGE_CURVE ( 'NONE', #36853, #27926, #32187, .T. ) ;
#25665=EDGE_CURVE ( 'NONE', #11965, #34244, #28381, .T. ) ;
#25671=ORIENTED_EDGE ( 'NONE', *, *, #23201, .F. ) ;
#25672=DIRECTION ( 'NONE',  ( -1.000000000000000000, 0.000000000000000000, 0.000000000000000000 ) ) ;
#25674=ADVANCED_FACE ( 'NONE', ( #16829 ), #29135, .T. ) ;
#25679=ORIENTED_EDGE ( 'NONE', *, *, #1141, .T. ) ;
#25683=EDGE_LOOP ( 'NONE', ( #30108, #23260, #43676, #6060, #3747, #30934 ) ) ;
#25684=CARTESIAN_POINT ( 'NONE',  ( -164.9459734468149463, 2.143131898507880377E-16, 165.0000000000000000 ) ) ;
#25685=CARTESIAN_POINT ( 'NONE',  ( -204.9459734468149463, 2.143131898507880377E-16, -120.9317124430720156 ) ) ;
#25693=DIRECTION ( 'NONE',  ( 1.000000000000000000, 0.000000000000000000, -0.000000000000000000 ) ) ;
#25694=CARTESIAN_POINT ( 'NONE',  ( 210.0000000000000568, 0.000000000000000000, -39.18171244307202983 ) ) ;
#25695=CARTESIAN_POINT ( 'NONE',  ( 71.55402655318505367, 0.000000000000000000, -40.93171244307205825 ) ) ;
#25698=CARTESIAN_POINT ( 'NONE',  ( 35.05402655318504657, 2.143131898507880377E-16, -80.93171244307204404 ) ) ;
#25699=EDGE_CURVE ( 'NONE', #46387, #19943, #40424, .T. ) ;
#25704=CARTESIAN_POINT ( 'NONE',  ( 153.3040265531850537, -1.750000000000010658, -119.1817124430720440 ) ) ;
#25705=CYLINDRICAL_SURFACE ( 'NONE', #42291, 1.750000000000015543 ) ;
#25707=CARTESIAN_POINT ( 'NONE',  ( -4.945973446814917018, -1.025126265847096985, -160.9317124430720014 ) ) ;
#25708=DIRECTION ( 'NONE',  ( 0.000000000000000000, 0.000000000000000000, 1.000000000000000000 ) ) ;
#25709=CARTESIAN_POINT ( 'NONE',  ( -46.69597344681494633, -1.750000000000009992, -159.1817124430720298 ) ) ;
#25713=VERTEX_POINT ( 'NONE', #24527 ) ;
#25718=CARTESIAN_POINT ( 'NONE',  ( -128.4459734468149179, 0.000000000000000000, -0.9317124430719969652 ) ) ;
#25726=EDGE_CURVE ( 'NONE', #13539, #23942, #37440, .T. ) ;
#25727=CARTESIAN_POINT ( 'NONE',  ( 74.32915281903215998, 1.750000000000010214, -120.2068387089191219 ) ) ;
#25728=( BOUNDED_CURVE ( )  B_SPLINE_CURVE ( 3, ( #2543, #32862, #5631, #13331 ),
 .UNSPECIFIED., .F., .F. ) 
 B_SPLINE_CURVE_WITH_KNOTS ( ( 4, 4 ),
 ( 4.712388980384689674, 6.283185307179586232 ),
 .UNSPECIFIED. ) 
 CURVE ( )  GEOMETRIC_REPRESENTATION_ITEM ( )  RATIONAL_B_SPLINE_CURVE ( ( 1.000000000000000000, 0.8047378541243649375, 0.8047378541243649375, 1.000000000000000000 ) ) 
 REPRESENTATION_ITEM ( '' )  );
#25729=DIRECTION ( 'NONE',  ( 0.000000000000000000, 0.000000000000000000, -1.000000000000000000 ) ) ;
#25731=CARTESIAN_POINT ( 'NONE',  ( 151.5540265531850537, 0.000000000000000000, 165.0000000000000000 ) ) ;
#25732=CARTESIAN_POINT ( 'NONE',  ( -8.445973446814976526, 0.000000000000000000, 159.0682875569279418 ) ) ;
#25736=( BOUNDED_CURVE ( )  B_SPLINE_CURVE ( 3, ( #16920, #48159, #43844, #28213 ),
 .UNSPECIFIED., .F., .F. ) 
 B_SPLINE_CURVE_WITH_KNOTS ( ( 4, 4 ),
 ( 0.000000000000000000, 1.570796326794896780 ),
 .UNSPECIFIED. ) 
 CURVE ( )  GEOMETRIC_REPRESENTATION_ITEM ( )  RATIONAL_B_SPLINE_CURVE ( ( 1.000000000000000000, 0.8047378541243649375, 0.8047378541243649375, 1.000000000000000000 ) ) 
 REPRESENTATION_ITEM ( '' )  );
#25739=CARTESIAN_POINT ( 'NONE',  ( -167.7210997126620384, -1.750000000000010214, -78.15658617722490931 ) ) ;
#25740=CYLINDRICAL_SURFACE ( 'NONE', #7674, 1.750000000000008438 ) ;
#25745=DIRECTION ( 'NONE',  ( 1.000000000000000000, 0.000000000000000000, -0.000000000000000000 ) ) ;
#25753=CARTESIAN_POINT ( 'NONE',  ( -166.6959734468149463, -1.750000000000010658, 80.81828755692798438 ) ) ;
#25762=CARTESIAN_POINT ( 'NONE',  ( 73.30402655318508209, -1.750000000000009992, 160.8182875569279702 ) ) ;
#25763=CARTESIAN_POINT ( 'NONE',  ( -210.0000000000000568, 0.000000000000000000, -77.43171244307200141 ) ) ;
#25764=DIRECTION ( 'NONE',  ( -0.000000000000000000, -0.000000000000000000, -1.000000000000000000 ) ) ;
#25766=CARTESIAN_POINT ( 'NONE',  ( -206.6959734468149463, 0.000000000000000000, 165.0000000000000000 ) ) ;
#25771=VERTEX_POINT ( 'NONE', #29380 ) ;
#25772=VERTEX_POINT ( 'NONE', #8630 ) ;
#25773=AXIS2_PLACEMENT_3D ( 'NONE', #35534, #124, #8327 ) ;
#25774=CARTESIAN_POINT ( 'NONE',  ( -164.9459734468149463, 2.143131898507880377E-16, -0.9317124430720247208 ) ) ;
#25781=ORIENTED_EDGE ( 'NONE', *, *, #45534, .F. ) ;
#25782=CYLINDRICAL_SURFACE ( 'NONE', #8652, 1.750000000000036193 ) ;
#25787=CARTESIAN_POINT ( 'NONE',  ( 72.27890028733797578, 1.750000000000009548, -0.2068387089191121020 ) ) ;
#25790=CARTESIAN_POINT ( 'NONE',  ( -208.4459734468148611, 1.025126265847089213, 42.56828755692799149 ) ) ;
#25791=DIRECTION ( 'NONE',  ( -1.000000000000000000, 0.000000000000000000, 0.000000000000000000 ) ) ;
#25798=EDGE_CURVE ( 'NONE', #12438, #16264, #49332, .T. ) ;
#25800=CARTESIAN_POINT ( 'NONE',  ( -168.4459734468149747, 1.025126265847089435, 122.5682875569280128 ) ) ;
#25801=EDGE_CURVE ( 'NONE', #25772, #44745, #49505, .T. ) ;
#25802=EDGE_CURVE ( 'NONE', #34395, #43947, #45249, .T. ) ;
#25808=CYLINDRICAL_SURFACE ( 'NONE', #5694, 1.750000000000001554 ) ;
#25809=CARTESIAN_POINT ( 'NONE',  ( -204.9459734468148895, -1.025126265847089213, -160.9317124430720014 ) ) ;
#25810=CARTESIAN_POINT ( 'NONE',  ( -45.67084718096785423, -1.750000000000009548, -38.15658617722494483 ) ) ;
#25816=CARTESIAN_POINT ( 'NONE',  ( 210.0000000000000568, 0.000000000000000000, 82.56828755692799859 ) ) ;
#25818=EDGE_CURVE ( 'NONE', #31470, #27168, #11856, .T. ) ;
#25824=ORIENTED_EDGE ( 'NONE', *, *, #39649, .F. ) ;
#25832=CARTESIAN_POINT ( 'NONE',  ( 210.0000000000000568, 0.000000000000000000, 120.8182875569279702 ) ) ;
#25835=ORIENTED_EDGE ( 'NONE', *, *, #45038, .F. ) ;
#25841=EDGE_CURVE ( 'NONE', #42641, #23796, #49206, .T. ) ;
#25842=DIRECTION ( 'NONE',  ( 0.000000000000000000, 0.000000000000000000, -1.000000000000000000 ) ) ;
#25848=EDGE_CURVE ( 'NONE', #18366, #9801, #5342, .T. ) ;
#25849=CARTESIAN_POINT ( 'NONE',  ( 114.3291528190321173, -1.749999999999996225, 1.843413822775058497 ) ) ;
#25852=EDGE_CURVE ( 'NONE', #18024, #49373, #18076, .T. ) ;
#25854=CIRCLE ( 'NONE', #15197, 1.750000000000015543 ) ;
#25860=CARTESIAN_POINT ( 'NONE',  ( 154.3291528190321458, 1.750000000000010214, -120.2068387089191219 ) ) ;
#25861=( BOUNDED_CURVE ( )  B_SPLINE_CURVE ( 3, ( #22851, #2837, #42351, #18235 ),
 .UNSPECIFIED., .F., .F. ) 
 B_SPLINE_CURVE_WITH_KNOTS ( ( 4, 4 ),
 ( 3.141592653589793116, 4.712388980384689674 ),
 .UNSPECIFIED. ) 
 CURVE ( )  GEOMETRIC_REPRESENTATION_ITEM ( )  RATIONAL_B_SPLINE_CURVE ( ( 1.000000000000000000, 0.8047378541243649375, 0.8047378541243649375, 1.000000000000000000 ) ) 
 REPRESENTATION_ITEM ( '' )  );
#25862=ORIENTED_EDGE ( 'NONE', *, *, #5504, .F. ) ;
#25864=CARTESIAN_POINT ( 'NONE',  ( 153.3040265531850537, 1.750000000000010214, -39.18171244307202983 ) ) ;
#25871=( BOUNDED_CURVE ( )  B_SPLINE_CURVE ( 3, ( #22563, #38248, #3059, #49967 ),
 .UNSPECIFIED., .F., .F. ) 
 B_SPLINE_CURVE_WITH_KNOTS ( ( 4, 4 ),
 ( 0.000000000000000000, 1.570796326794896558 ),
 .UNSPECIFIED. ) 
 CURVE ( )  GEOMETRIC_REPRESENTATION_ITEM ( )  RATIONAL_B_SPLINE_CURVE ( ( 1.000000000000000000, 0.8047378541243649375, 0.8047378541243649375, 1.000000000000000000 ) ) 
 REPRESENTATION_ITEM ( '' )  );
#25875=EDGE_CURVE ( 'NONE', #35538, #6064, #36844, .T. ) ;
#25876=ORIENTED_EDGE ( 'NONE', *, *, #35600, .F. ) ;
#25880=AXIS2_PLACEMENT_3D ( 'NONE', #32331, #36708, #47924 ) ;
#25881=EDGE_CURVE ( 'NONE', #7107, #7456, #30396, .T. ) ;
#25884=CARTESIAN_POINT ( 'NONE',  ( 210.0000000000000568, 0.000000000000000000, -119.1817124430720440 ) ) ;
#25887=EDGE_CURVE ( 'NONE', #9233, #43863, #15496, .T. ) ;
#25888=CARTESIAN_POINT ( 'NONE',  ( -48.44597344681495343, 0.000000000000000000, 119.0682875569279702 ) ) ;
#25891=( BOUNDED_CURVE ( )  B_SPLINE_CURVE ( 3, ( #30171, #11435, #31204, #38150 ),
 .UNSPECIFIED., .F., .F. ) 
 B_SPLINE_CURVE_WITH_KNOTS ( ( 4, 4 ),
 ( 1.570796326794896558, 3.141592653589793116 ),
 .UNSPECIFIED. ) 
 CURVE ( )  GEOMETRIC_REPRESENTATION_ITEM ( )  RATIONAL_B_SPLINE_CURVE ( ( 1.000000000000000000, 0.8047378541243649375, 0.8047378541243649375, 1.000000000000000000 ) ) 
 REPRESENTATION_ITEM ( '' )  );
#25895=DIRECTION ( 'NONE',  ( -0.000000000000000000, -0.000000000000000000, -1.000000000000000000 ) ) ;
#25899=CARTESIAN_POINT ( 'NONE',  ( -168.4459734468149463, 0.000000000000000000, 42.56828755692798438 ) ) ;
#25904=VERTEX_POINT ( 'NONE', #50601 ) ;
#25906=CARTESIAN_POINT ( 'NONE',  ( -124.9459734468149463, 2.143131898507847836E-16, 165.0000000000000000 ) ) ;
#25907=ORIENTED_EDGE ( 'NONE', *, *, #14690, .T. ) ;
#25913=CARTESIAN_POINT ( 'NONE',  ( 195.0540265531851105, 2.143131898507880377E-16, 2.568287556927978166 ) ) ;
#25919=VERTEX_POINT ( 'NONE', #11152 ) ;
#25926=CARTESIAN_POINT ( 'NONE',  ( -124.9459734468149321, 1.025126265847082108, -117.4317124430720440 ) ) ;
#25928=DIRECTION ( 'NONE',  ( -0.000000000000000000, -0.000000000000000000, -1.000000000000000000 ) ) ;
#25929=ADVANCED_FACE ( 'NONE', ( #23192 ), #3950, .T. ) ;
#25932=CYLINDRICAL_SURFACE ( 'NONE', #29074, 1.750000000000015543 ) ;
#25935=ORIENTED_EDGE ( 'NONE', *, *, #41488, .T. ) ;
#25943=CARTESIAN_POINT ( 'NONE',  ( 115.0540265531850395, 2.143131898507842906E-16, -165.0000000000000000 ) ) ;
#25950=CARTESIAN_POINT ( 'NONE',  ( 193.3040265531851105, 1.750000000000009992, 160.8182875569279702 ) ) ;
#25951=CARTESIAN_POINT ( 'NONE',  ( 210.0000000000000568, 0.000000000000000000, 0.8182875569279768335 ) ) ;
#25953=CARTESIAN_POINT ( 'NONE',  ( 194.3291528190321742, 1.750000000000009548, -40.20683870891912193 ) ) ;
#25955=ORIENTED_EDGE ( 'NONE', *, *, #32367, .T. ) ;
#25957=VERTEX_POINT ( 'NONE', #46255 ) ;
#25958=CARTESIAN_POINT ( 'NONE',  ( 34.32915281903212446, -1.750000000000009548, 121.8434138227750623 ) ) ;
#25963=CARTESIAN_POINT ( 'NONE',  ( -124.9459734468149321, -1.025126265847081886, -80.93171244307201562 ) ) ;
#25967=EDGE_CURVE ( 'NONE', #48612, #7661, #43996, .T. ) ;
#25971=CARTESIAN_POINT ( 'NONE',  ( 153.3040265531850537, 1.750000000000010658, -119.1817124430720440 ) ) ;
#25976=CARTESIAN_POINT ( 'NONE',  ( 152.2789002873379900, 1.750000000000009548, -38.15658617722494483 ) ) ;
#25978=CARTESIAN_POINT ( 'NONE',  ( -88.44597344681497475, 0.000000000000000000, -165.0000000000000000 ) ) ;
#25979=EDGE_LOOP ( 'NONE', ( #49233, #19733, #47603, #36418, #15099, #43564 ) ) ;
#25982=ORIENTED_EDGE ( 'NONE', *, *, #18934, .F. ) ;
#25984=CYLINDRICAL_SURFACE ( 'NONE', #16246, 1.750000000000015543 ) ;
#25988=CYLINDRICAL_SURFACE ( 'NONE', #35485, 1.750000000000015543 ) ;
#25989=EDGE_LOOP ( 'NONE', ( #9720, #9659, #6868, #41581, #35164, #32031 ) ) ;
#25996=ORIENTED_EDGE ( 'NONE', *, *, #40386, .T. ) ;
#26001=CARTESIAN_POINT ( 'NONE',  ( 210.0000000000000568, 0.000000000000000000, -39.18171244307202983 ) ) ;
#26004=ADVANCED_FACE ( 'NONE', ( #17271 ), #13164, .T. ) ;
#26006=ORIENTED_EDGE ( 'NONE', *, *, #48586, .T. ) ;
#26010=EDGE_LOOP ( 'NONE', ( #35129, #35134, #44126, #32642, #13951, #48872 ) ) ;
#26018=CARTESIAN_POINT ( 'NONE',  ( 75.05402655318508209, 0.000000000000000000, 162.5682875569279702 ) ) ;
#26020=VERTEX_POINT ( 'NONE', #28315 ) ;
#26021=CARTESIAN_POINT ( 'NONE',  ( 113.3040265531850537, -1.749999999999996891, -159.1817124430720298 ) ) ;
#26025=( BOUNDED_CURVE ( )  B_SPLINE_CURVE ( 3, ( #35087, #15318, #50657, #173 ),
 .UNSPECIFIED., .F., .F. ) 
 B_SPLINE_CURVE_WITH_KNOTS ( ( 4, 4 ),
 ( 0.000000000000000000, 1.570796326794896558 ),
 .UNSPECIFIED. ) 
 CURVE ( )  GEOMETRIC_REPRESENTATION_ITEM ( )  RATIONAL_B_SPLINE_CURVE ( ( 1.000000000000000000, 0.8047378541243649375, 0.8047378541243649375, 1.000000000000000000 ) ) 
 REPRESENTATION_ITEM ( '' )  );
#26030=( BOUNDED_CURVE ( )  B_SPLINE_CURVE ( 3, ( #24140, #39536, #16669, #47180 ),
 .UNSPECIFIED., .F., .F. ) 
 B_SPLINE_CURVE_WITH_KNOTS ( ( 4, 4 ),
 ( 3.141592653589793116, 4.712388980384689674 ),
 .UNSPECIFIED. ) 
 CURVE ( )  GEOMETRIC_REPRESENTATION_ITEM ( )  RATIONAL_B_SPLINE_CURVE ( ( 1.000000000000000000, 0.8047378541243649375, 0.8047378541243649375, 1.000000000000000000 ) ) 
 REPRESENTATION_ITEM ( '' )  );
#26034=ORIENTED_EDGE ( 'NONE', *, *, #15636, .F. ) ;
#26035=DIRECTION ( 'NONE',  ( -1.000000000000000000, -0.000000000000000000, -0.000000000000000000 ) ) ;
#26036=CARTESIAN_POINT ( 'NONE',  ( 210.0000000000000568, 0.000000000000000000, 80.81828755692798438 ) ) ;
#26040=CARTESIAN_POINT ( 'NONE',  ( -88.44597344681494633, 1.025126265847089213, -160.9317124430720014 ) ) ;
#26043=CARTESIAN_POINT ( 'NONE',  ( 151.5540265531850537, -1.025126265847089435, -157.4317124430720582 ) ) ;
#26044=LINE ( 'NONE', #6537, #6001 ) ;
#26047=CARTESIAN_POINT ( 'NONE',  ( 71.55402655318505367, 0.000000000000000000, -37.43171244307200141 ) ) ;
#26052=CARTESIAN_POINT ( 'NONE',  ( 210.0000000000000568, 2.143131898507884075E-16, -40.93171244307203693 ) ) ;
#26064=LINE ( 'NONE', #6561, #25467 ) ;
#26065=ORIENTED_EDGE ( 'NONE', *, *, #43904, .F. ) ;
#26067=CARTESIAN_POINT ( 'NONE',  ( 195.0540265531851105, 2.143131898507880377E-16, -37.43171244307205825 ) ) ;
#26071=ORIENTED_EDGE ( 'NONE', *, *, #35068, .F. ) ;
#26076=CYLINDRICAL_SURFACE ( 'NONE', #19389, 1.750000000000015543 ) ;
#26077=CARTESIAN_POINT ( 'NONE',  ( -85.67084718096784002, 1.750000000000009548, -40.20683870891912193 ) ) ;
#26079=VERTEX_POINT ( 'NONE', #1129 ) ;
#26080=CARTESIAN_POINT ( 'NONE',  ( 113.3040265531850537, -1.749999999999996891, 160.8182875569279702 ) ) ;
#26086=CARTESIAN_POINT ( 'NONE',  ( -4.945973446814903696, 2.143131898507912917E-16, 122.5682875569279986 ) ) ;
#26087=CARTESIAN_POINT ( 'NONE',  ( -208.4459734468149463, 0.000000000000000000, 79.06828755692797017 ) ) ;
#26090=VERTEX_POINT ( 'NONE', #20612 ) ;
#26091=CARTESIAN_POINT ( 'NONE',  ( 31.55402655318503236, 0.000000000000000000, 165.0000000000000000 ) ) ;
#26095=DIRECTION ( 'NONE',  ( -1.000000000000000000, -0.000000000000000000, -0.000000000000000000 ) ) ;
#26096=VERTEX_POINT ( 'NONE', #37050 ) ;
#26098=DIRECTION ( 'NONE',  ( 0.000000000000000000, 0.000000000000000000, 1.000000000000000000 ) ) ;
#26104=CARTESIAN_POINT ( 'NONE',  ( -126.6959734468149321, -1.749999999999997335, -79.18171244307201562 ) ) ;
#26108=ORIENTED_EDGE ( 'NONE', *, *, #6367, .F. ) ;
#26109=CARTESIAN_POINT ( 'NONE',  ( 34.32915281903212446, -1.750000000000009326, 1.843413822775066269 ) ) ;
#26110=ORIENTED_EDGE ( 'NONE', *, *, #44214, .F. ) ;
#26111=EDGE_LOOP ( 'NONE', ( #24380, #49507, #5863, #1431, #24055, #16681 ) ) ;
#26115=ADVANCED_FACE ( 'NONE', ( #47526 ), #28564, .T. ) ;
#26122=EDGE_CURVE ( 'NONE', #41219, #28277, #32671, .T. ) ;
#26123=CARTESIAN_POINT ( 'NONE',  ( -48.44597344681496054, -1.025126265847089657, 119.0682875569279560 ) ) ;
#26127=EDGE_CURVE ( 'NONE', #4845, #43762, #44284, .T. ) ;
#26130=EDGE_CURVE ( 'NONE', #47298, #15646, #21362, .T. ) ;
#26131=CARTESIAN_POINT ( 'NONE',  ( -46.69597344681494633, 0.000000000000000000, -165.0000000000000000 ) ) ;
#26144=CARTESIAN_POINT ( 'NONE',  ( 75.05402655318509630, -1.025126265847089435, 122.5682875569280128 ) ) ;
#26146=CARTESIAN_POINT ( 'NONE',  ( -88.44597344681494633, -1.025126265847089657, 119.0682875569279560 ) ) ;
#26152=CARTESIAN_POINT ( 'NONE',  ( 210.0000000000000568, 0.000000000000000000, -77.43171244307200141 ) ) ;
#26159=( BOUNDED_CURVE ( )  B_SPLINE_CURVE ( 3, ( #25558, #41198, #37390, #17101 ),
 .UNSPECIFIED., .F., .F. ) 
 B_SPLINE_CURVE_WITH_KNOTS ( ( 4, 4 ),
 ( 3.141592653589793116, 4.712388980384689674 ),
 .UNSPECIFIED. ) 
 CURVE ( )  GEOMETRIC_REPRESENTATION_ITEM ( )  RATIONAL_B_SPLINE_CURVE ( ( 1.000000000000000000, 0.8047378541243649375, 0.8047378541243649375, 1.000000000000000000 ) ) 
 REPRESENTATION_ITEM ( '' )  );
#26160=CARTESIAN_POINT ( 'NONE',  ( -168.4459734468149463, 0.000000000000000000, 79.06828755692797017 ) ) ;
#26161=EDGE_CURVE ( 'NONE', #24507, #4778, #13669, .T. ) ;
#26163=AXIS2_PLACEMENT_3D ( 'NONE', #14166, #22139, #41127 ) ;
#26164=FACE_OUTER_BOUND ( 'NONE', #1455, .T. ) ;
#26165=LINE ( 'NONE', #41809, #41242 ) ;
#26167=ADVANCED_FACE ( 'NONE', ( #33192 ), #45690, .T. ) ;
#26168=CARTESIAN_POINT ( 'NONE',  ( -6.695973446814940111, 1.750000000000024203, 120.8182875569279702 ) ) ;
#26169=AXIS2_PLACEMENT_3D ( 'NONE', #49720, #21555, #2558 ) ;
#26171=( BOUNDED_CURVE ( )  B_SPLINE_CURVE ( 3, ( #46121, #26410, #18456, #2803 ),
 .UNSPECIFIED., .F., .F. ) 
 B_SPLINE_CURVE_WITH_KNOTS ( ( 4, 4 ),
 ( 4.712388980384689674, 6.283185307179586232 ),
 .UNSPECIFIED. ) 
 CURVE ( )  GEOMETRIC_REPRESENTATION_ITEM ( )  RATIONAL_B_SPLINE_CURVE ( ( 1.000000000000000000, 0.8047378541243649375, 0.8047378541243649375, 1.000000000000000000 ) ) 
 REPRESENTATION_ITEM ( '' )  );
#26173=CARTESIAN_POINT ( 'NONE',  ( 112.2789002873379758, -1.749999999999996669, -160.2068387089191219 ) ) ;
#26177=DIRECTION ( 'NONE',  ( -0.000000000000000000, -0.000000000000000000, -1.000000000000000000 ) ) ;
#26181=CARTESIAN_POINT ( 'NONE',  ( -84.94597344681494633, 2.143131898507880377E-16, -37.43171244307205825 ) ) ;
#26182=( BOUNDED_CURVE ( )  B_SPLINE_CURVE ( 3, ( #40362, #28047, #611, #43435 ),
 .UNSPECIFIED., .F., .F. ) 
 B_SPLINE_CURVE_WITH_KNOTS ( ( 4, 4 ),
 ( 3.141592653589793116, 4.712388980384689674 ),
 .UNSPECIFIED. ) 
 CURVE ( )  GEOMETRIC_REPRESENTATION_ITEM ( )  RATIONAL_B_SPLINE_CURVE ( ( 1.000000000000000000, 0.8047378541243649375, 0.8047378541243649375, 1.000000000000000000 ) ) 
 REPRESENTATION_ITEM ( '' )  );
#26183=VERTEX_POINT ( 'NONE', #14426 ) ;
#26184=CARTESIAN_POINT ( 'NONE',  ( 155.0540265531850537, 2.143131898507880377E-16, 159.0682875569279702 ) ) ;
#26189=EDGE_CURVE ( 'NONE', #38466, #48958, #33442, .T. ) ;
#26191=CARTESIAN_POINT ( 'NONE',  ( 31.55402655318503236, 0.000000000000000000, -77.43171244307198720 ) ) ;
#26195=CARTESIAN_POINT ( 'NONE',  ( -8.445973446814964092, -1.025126265847097429, -80.93171244307204404 ) ) ;
#26198=DIRECTION ( 'NONE',  ( -1.000000000000000000, -0.000000000000000000, -0.000000000000000000 ) ) ;
#26203=AXIS2_PLACEMENT_3D ( 'NONE', #48084, #9135, #5789 ) ;
#26204=ORIENTED_EDGE ( 'NONE', *, *, #9992, .F. ) ;
#26208=CARTESIAN_POINT ( 'NONE',  ( 151.5540265531850537, -1.025126265847089657, -120.9317124430720440 ) ) ;
#26210=CARTESIAN_POINT ( 'NONE',  ( 210.0000000000000568, 0.000000000000000000, -117.4317124430720298 ) ) ;
#26217=DIRECTION ( 'NONE',  ( 1.000000000000000000, 0.000000000000000000, 0.000000000000000000 ) ) ;
#26218=EDGE_LOOP ( 'NONE', ( #21494, #33744, #39340, #32848, #43938 ) ) ;
#26224=ORIENTED_EDGE ( 'NONE', *, *, #29996, .F. ) ;
#26226=CARTESIAN_POINT ( 'NONE',  ( 151.5540265531850537, 0.000000000000000000, 165.0000000000000000 ) ) ;
#26230=EDGE_CURVE ( 'NONE', #29044, #35915, #43143, .T. ) ;
#26236=EDGE_CURVE ( 'NONE', #24955, #214, #9242, .T. ) ;
#26247=VECTOR ( 'NONE', #25526, 1000.000000000000000 ) ;
#26250=AXIS2_PLACEMENT_3D ( 'NONE', #7415, #19955, #15610 ) ;
#26255=CIRCLE ( 'NONE', #19695, 1.750000000000009992 ) ;
#26257=EDGE_CURVE ( 'NONE', #12693, #11343, #38307, .T. ) ;
#26262=FACE_OUTER_BOUND ( 'NONE', #31727, .T. ) ;
#26265=DIRECTION ( 'NONE',  ( 0.000000000000000000, 0.000000000000000000, 1.000000000000000000 ) ) ;
#26271=DIRECTION ( 'NONE',  ( -1.000000000000000000, -0.000000000000000000, -0.000000000000000000 ) ) ;
#26272=ORIENTED_EDGE ( 'NONE', *, *, #33765, .T. ) ;
#26281=LINE ( 'NONE', #14472, #23229 ) ;
#26299=DIRECTION ( 'NONE',  ( -0.000000000000000000, -0.000000000000000000, -1.000000000000000000 ) ) ;
#26303=EDGE_CURVE ( 'NONE', #28349, #37476, #14931, .T. ) ;
#26304=CARTESIAN_POINT ( 'NONE',  ( -46.69597344681494633, 0.000000000000000000, 165.0000000000000000 ) ) ;
#26306=CARTESIAN_POINT ( 'NONE',  ( -84.94597344681493212, -1.025126265847088991, -157.4317124430720582 ) ) ;
#26316=CARTESIAN_POINT ( 'NONE',  ( -7.721099712662037540, 1.750000000000023315, -40.20683870891912903 ) ) ;
#26323=ORIENTED_EDGE ( 'NONE', *, *, #26447, .F. ) ;
#26324=CARTESIAN_POINT ( 'NONE',  ( 210.0000000000000568, 0.000000000000000000, 2.568287556927987048 ) ) ;
#26325=CARTESIAN_POINT ( 'NONE',  ( 191.5540265531851105, 0.000000000000000000, 2.568287556927978166 ) ) ;
#26326=DIRECTION ( 'NONE',  ( 1.000000000000000000, 0.000000000000000000, 0.000000000000000000 ) ) ;
#26327=ORIENTED_EDGE ( 'NONE', *, *, #37767, .F. ) ;
#26330=( BOUNDED_CURVE ( )  B_SPLINE_CURVE ( 3, ( #31833, #47418, #12306, #7972 ),
 .UNSPECIFIED., .F., .F. ) 
 B_SPLINE_CURVE_WITH_KNOTS ( ( 4, 4 ),
 ( 1.570796326794896558, 3.141592653589793116 ),
 .UNSPECIFIED. ) 
 CURVE ( )  GEOMETRIC_REPRESENTATION_ITEM ( )  RATIONAL_B_SPLINE_CURVE ( ( 1.000000000000000000, 0.8047378541243649375, 0.8047378541243649375, 1.000000000000000000 ) ) 
 REPRESENTATION_ITEM ( '' )  );
#26331=EDGE_CURVE ( 'NONE', #30887, #7661, #30850, .T. ) ;
#26337=CARTESIAN_POINT ( 'NONE',  ( -86.69597344681494633, 1.750000000000010214, -39.18171244307202983 ) ) ;
#26338=CARTESIAN_POINT ( 'NONE',  ( 35.05402655318504657, 2.143131898507880377E-16, -0.9317124430720247208 ) ) ;
#26340=ORIENTED_EDGE ( 'NONE', *, *, #3882, .T. ) ;
#26341=FACE_OUTER_BOUND ( 'NONE', #14971, .T. ) ;
#26348=CARTESIAN_POINT ( 'NONE',  ( -208.4459734468149463, 0.000000000000000000, -117.4317124430720725 ) ) ;
#26352=LINE ( 'NONE', #41996, #28195 ) ;
#26355=CARTESIAN_POINT ( 'NONE',  ( -165.6708471809677974, -1.750000000000009548, -38.15658617722494483 ) ) ;
#26371=CARTESIAN_POINT ( 'NONE',  ( -8.445973446814976526, 0.000000000000000000, 119.0682875569279418 ) ) ;
#26375=VERTEX_POINT ( 'NONE', #33832 ) ;
#26377=ORIENTED_EDGE ( 'NONE', *, *, #21949, .T. ) ;
#26381=DIRECTION ( 'NONE',  ( -1.000000000000000000, -0.000000000000000000, -0.000000000000000000 ) ) ;
#26393=ORIENTED_EDGE ( 'NONE', *, *, #29265, .T. ) ;
#26398=CARTESIAN_POINT ( 'NONE',  ( -46.69597344681494633, -1.750000000000009992, 160.8182875569279702 ) ) ;
#26399=CARTESIAN_POINT ( 'NONE',  ( 113.3040265531850537, 1.749999999999997335, 120.8182875569279702 ) ) ;
#26400=FACE_OUTER_BOUND ( 'NONE', #44220, .T. ) ;
#26402=CARTESIAN_POINT ( 'NONE',  ( -126.6959734468149321, -1.749999999999997335, 80.81828755692798438 ) ) ;
#26407=CARTESIAN_POINT ( 'NONE',  ( 71.55402655318505367, 1.025126265847089435, -77.43171244307200141 ) ) ;
#26409=AXIS2_PLACEMENT_3D ( 'NONE', #1657, #33226, #37079 ) ;
#26410=CARTESIAN_POINT ( 'NONE',  ( -45.67084718096785423, -1.750000000000009548, 39.79316129108089228 ) ) ;
#26416=CARTESIAN_POINT ( 'NONE',  ( 73.30402655318508209, 1.750000000000009992, 160.8182875569279702 ) ) ;
#26417=DIRECTION ( 'NONE',  ( -0.000000000000000000, -0.000000000000000000, -1.000000000000000000 ) ) ;
#26420=ORIENTED_EDGE ( 'NONE', *, *, #25089, .F. ) ;
#26424=CARTESIAN_POINT ( 'NONE',  ( 210.0000000000000568, 2.143131898507876926E-16, 79.06828755692797017 ) ) ;
#26425=CARTESIAN_POINT ( 'NONE',  ( 75.05402655318509630, 2.143131898507880377E-16, -120.9317124430720725 ) ) ;
#26426=ADVANCED_FACE ( 'NONE', ( #41517 ), #49166, .T. ) ;
#26427=ADVANCED_FACE ( 'NONE', ( #17896 ), #13793, .T. ) ;
#26430=ORIENTED_EDGE ( 'NONE', *, *, #28417, .F. ) ;
#26432=CARTESIAN_POINT ( 'NONE',  ( 191.5540265531851105, 0.000000000000000000, 82.56828755692798438 ) ) ;
#26433=ORIENTED_EDGE ( 'NONE', *, *, #25001, .T. ) ;
#26437=ORIENTED_EDGE ( 'NONE', *, *, #47534, .T. ) ;
#26438=CARTESIAN_POINT ( 'NONE',  ( 210.0000000000000568, 2.143131898507881856E-16, 79.06828755692797017 ) ) ;
#26441=EDGE_LOOP ( 'NONE', ( #40181, #40090 ) ) ;
#26442=ADVANCED_FACE ( 'NONE', ( #10218 ), #14048, .T. ) ;
#26443=ORIENTED_EDGE ( 'NONE', *, *, #12770, .F. ) ;
#26445=EDGE_CURVE ( 'NONE', #9702, #7456, #8944, .T. ) ;
#26447=EDGE_CURVE ( 'NONE', #8111, #40403, #7295, .T. ) ;
#26450=AXIS2_PLACEMENT_3D ( 'NONE', #49687, #14834, #3025 ) ;
#26454=CARTESIAN_POINT ( 'NONE',  ( -4.945973446814903696, 2.143131898507912917E-16, -120.9317124430720725 ) ) ;
#26455=EDGE_CURVE ( 'NONE', #7807, #37221, #36947, .T. ) ;
#26456=CARTESIAN_POINT ( 'NONE',  ( -208.4459734468149463, 0.000000000000000000, -77.43171244307204404 ) ) ;
#26458=LINE ( 'NONE', #50515, #32496 ) ;
#26459=CARTESIAN_POINT ( 'NONE',  ( 154.3291528190321458, 1.750000000000010214, -118.1565861772249519 ) ) ;
#26461=( BOUNDED_CURVE ( )  B_SPLINE_CURVE ( 3, ( #10708, #6869, #22511, #14045 ),
 .UNSPECIFIED., .F., .F. ) 
 B_SPLINE_CURVE_WITH_KNOTS ( ( 4, 4 ),
 ( 0.000000000000000000, 1.570796326794896558 ),
 .UNSPECIFIED. ) 
 CURVE ( )  GEOMETRIC_REPRESENTATION_ITEM ( )  RATIONAL_B_SPLINE_CURVE ( ( 1.000000000000000000, 0.8047378541243649375, 0.8047378541243649375, 1.000000000000000000 ) ) 
 REPRESENTATION_ITEM ( '' )  );
#26463=ORIENTED_EDGE ( 'NONE', *, *, #8185, .F. ) ;
#26466=( BOUNDED_CURVE ( )  B_SPLINE_CURVE ( 3, ( #8783, #4905, #20567, #40578 ),
 .UNSPECIFIED., .F., .F. ) 
 B_SPLINE_CURVE_WITH_KNOTS ( ( 4, 4 ),
 ( 0.000000000000000000, 1.570796326794896558 ),
 .UNSPECIFIED. ) 
 CURVE ( )  GEOMETRIC_REPRESENTATION_ITEM ( )  RATIONAL_B_SPLINE_CURVE ( ( 1.000000000000000000, 0.8047378541243649375, 0.8047378541243649375, 1.000000000000000000 ) ) 
 REPRESENTATION_ITEM ( '' )  );
#26468=EDGE_LOOP ( 'NONE', ( #45589, #4512, #26969, #14, #48253 ) ) ;
#26480=CARTESIAN_POINT ( 'NONE',  ( 153.3040265531850537, 1.750000000000010658, 80.81828755692798438 ) ) ;
#26484=( BOUNDED_CURVE ( )  B_SPLINE_CURVE ( 3, ( #46045, #11205, #11698, #11963 ),
 .UNSPECIFIED., .F., .F. ) 
 B_SPLINE_CURVE_WITH_KNOTS ( ( 4, 4 ),
 ( 3.141592653589793116, 4.712388980384689674 ),
 .UNSPECIFIED. ) 
 CURVE ( )  GEOMETRIC_REPRESENTATION_ITEM ( )  RATIONAL_B_SPLINE_CURVE ( ( 1.000000000000000000, 0.8047378541243649375, 0.8047378541243649375, 1.000000000000000000 ) ) 
 REPRESENTATION_ITEM ( '' )  );
#26486=DIRECTION ( 'NONE',  ( -0.000000000000000000, -0.000000000000000000, -1.000000000000000000 ) ) ;
#26488=EDGE_CURVE ( 'NONE', #23271, #26375, #24693, .T. ) ;
#26503=CARTESIAN_POINT ( 'NONE',  ( -88.44597344681497475, 0.000000000000000000, 122.5682875569279986 ) ) ;
#26504=VERTEX_POINT ( 'NONE', #38441 ) ;
#26506=PLANE ( 'NONE',  #41461 ) ;
#26511=ORIENTED_EDGE ( 'NONE', *, *, #48982, .F. ) ;
#26516=ORIENTED_EDGE ( 'NONE', *, *, #1178, .F. ) ;
#26521=EDGE_CURVE ( 'NONE', #4446, #45409, #3782, .T. ) ;
#26525=CARTESIAN_POINT ( 'NONE',  ( -168.4459734468149747, 1.025126265847089657, -80.93171244307201562 ) ) ;
#26529=ORIENTED_EDGE ( 'NONE', *, *, #6410, .T. ) ;
#26534=CARTESIAN_POINT ( 'NONE',  ( 73.30402655318508209, 0.000000000000000000, 165.0000000000000000 ) ) ;
#26539=CARTESIAN_POINT ( 'NONE',  ( 74.32915281903215998, -1.750000000000009548, -118.1565861772249519 ) ) ;
#26541=AXIS2_PLACEMENT_3D ( 'NONE', #7353, #39427, #22982 ) ;
#26545=CARTESIAN_POINT ( 'NONE',  ( 154.3291528190321458, -1.750000000000010436, 119.7931612910808781 ) ) ;
#26546=DIRECTION ( 'NONE',  ( -0.000000000000000000, -0.000000000000000000, -1.000000000000000000 ) ) ;
#26551=VECTOR ( 'NONE', #29230, 1000.000000000000000 ) ;
#26552=AXIS2_PLACEMENT_3D ( 'NONE', #49922, #46356, #26636 ) ;
#26553=CARTESIAN_POINT ( 'NONE',  ( 34.32915281903212446, -1.750000000000010436, -80.20683870891910772 ) ) ;
#26556=EDGE_CURVE ( 'NONE', #38220, #13983, #17790, .T. ) ;
#26558=CARTESIAN_POINT ( 'NONE',  ( -166.6959734468149463, 1.750000000000010658, 120.8182875569279702 ) ) ;
#26559=VECTOR ( 'NONE', #18911, 1000.000000000000000 ) ;
#26567=CARTESIAN_POINT ( 'NONE',  ( 72.27890028733797578, -1.750000000000010214, 119.7931612910808781 ) ) ;
#26568=ADVANCED_FACE ( 'NONE', ( #7640 ), #22514, .T. ) ;
#26570=EDGE_CURVE ( 'NONE', #29055, #13717, #24994, .T. ) ;
#26572=ORIENTED_EDGE ( 'NONE', *, *, #15287, .T. ) ;
#26575=CARTESIAN_POINT ( 'NONE',  ( -86.69597344681496054, 0.000000000000000000, 165.0000000000000000 ) ) ;
#26576=ORIENTED_EDGE ( 'NONE', *, *, #34367, .T. ) ;
#26577=ORIENTED_EDGE ( 'NONE', *, *, #42742, .T. ) ;
#26580=CARTESIAN_POINT ( 'NONE',  ( 75.05402655318509630, 2.143131898507880377E-16, 119.0682875569279560 ) ) ;
#26585=CARTESIAN_POINT ( 'NONE',  ( -48.44597344681495343, 0.000000000000000000, 165.0000000000000000 ) ) ;
#26586=CARTESIAN_POINT ( 'NONE',  ( 31.55402655318503236, 0.000000000000000000, 82.56828755692798438 ) ) ;
#26588=AXIS2_PLACEMENT_3D ( 'NONE', #13195, #20645, #4991 ) ;
#26593=CARTESIAN_POINT ( 'NONE',  ( -44.94597344681493922, 2.143131898507880377E-16, -40.93171244307205825 ) ) ;
#26597=ORIENTED_EDGE ( 'NONE', *, *, #41357, .T. ) ;
#26598=VECTOR ( 'NONE', #38154, 1000.000000000000000 ) ;
#26603=CARTESIAN_POINT ( 'NONE',  ( -204.9459734468148895, 1.025126265847089879, -77.43171244307200141 ) ) ;
#26604=ORIENTED_EDGE ( 'NONE', *, *, #19758, .T. ) ;
#26608=CYLINDRICAL_SURFACE ( 'NONE', #42700, 1.749999999999973799 ) ;
#26609=AXIS2_PLACEMENT_3D ( 'NONE', #5711, #47766, #36794 ) ;
#26610=CARTESIAN_POINT ( 'NONE',  ( -126.6959734468149321, 1.749999999999997335, -119.1817124430720440 ) ) ;
#26612=EDGE_LOOP ( 'NONE', ( #47800, #39899 ) ) ;
#26615=DIRECTION ( 'NONE',  ( -0.000000000000000000, -0.000000000000000000, -1.000000000000000000 ) ) ;
#26618=CARTESIAN_POINT ( 'NONE',  ( 113.3040265531850537, 1.749999999999997335, -79.18171244307201562 ) ) ;
#26623=CARTESIAN_POINT ( 'NONE',  ( -126.6959734468149321, 1.749999999999997335, 120.8182875569279702 ) ) ;
#26625=( BOUNDED_CURVE ( )  B_SPLINE_CURVE ( 3, ( #32964, #2394, #17545, #10094 ),
 .UNSPECIFIED., .F., .F. ) 
 B_SPLINE_CURVE_WITH_KNOTS ( ( 4, 4 ),
 ( 0.000000000000000000, 1.570796326794896558 ),
 .UNSPECIFIED. ) 
 CURVE ( )  GEOMETRIC_REPRESENTATION_ITEM ( )  RATIONAL_B_SPLINE_CURVE ( ( 1.000000000000000000, 0.8047378541243649375, 0.8047378541243649375, 1.000000000000000000 ) ) 
 REPRESENTATION_ITEM ( '' )  );
#26627=CARTESIAN_POINT ( 'NONE',  ( 33.30402655318503946, -1.750000000000009992, 0.8182875569279768335 ) ) ;
#26631=CARTESIAN_POINT ( 'NONE',  ( -84.94597344681494633, 2.143131898507880377E-16, 165.0000000000000000 ) ) ;
#26635=DIRECTION ( 'NONE',  ( -1.000000000000000000, -0.000000000000000000, -0.000000000000000000 ) ) ;
#26636=DIRECTION ( 'NONE',  ( 0.000000000000000000, 0.000000000000000000, 1.000000000000000000 ) ) ;
#26638=LINE ( 'NONE', #35379, #42334 ) ;
#26640=ORIENTED_EDGE ( 'NONE', *, *, #31652, .F. ) ;
#26643=EDGE_CURVE ( 'NONE', #27700, #40814, #33525, .T. ) ;
#26644=CYLINDRICAL_SURFACE ( 'NONE', #47965, 1.750000000000008438 ) ;
#26649=CARTESIAN_POINT ( 'NONE',  ( -204.9459734468149463, 2.143131898507880377E-16, -120.9317124430720156 ) ) ;
#26652=VECTOR ( 'NONE', #50422, 1000.000000000000000 ) ;
#26659=CARTESIAN_POINT ( 'NONE',  ( -208.4459734468149463, 0.000000000000000000, -0.9317124430720247208 ) ) ;
#26667=DIRECTION ( 'NONE',  ( -1.000000000000000000, 0.000000000000000000, 0.000000000000000000 ) ) ;
#26678=CYLINDRICAL_SURFACE ( 'NONE', #29462, 1.750000000000001554 ) ;
#26681=CARTESIAN_POINT ( 'NONE',  ( 72.27890028733797578, 1.750000000000009326, 1.843413822775066269 ) ) ;
#26682=EDGE_CURVE ( 'NONE', #24906, #35538, #42054, .T. ) ;
#26690=CARTESIAN_POINT ( 'NONE',  ( -84.94597344681493212, 1.025126265847089657, 119.0682875569279560 ) ) ;
#26694=LINE ( 'NONE', #8465, #38809 ) ;
#26697=ORIENTED_EDGE ( 'NONE', *, *, #35912, .T. ) ;
#26702=DIRECTION ( 'NONE',  ( -1.000000000000000000, -0.000000000000000000, -0.000000000000000000 ) ) ;
#26704=DIRECTION ( 'NONE',  ( -1.000000000000000000, 0.000000000000000000, 0.000000000000000000 ) ) ;
#26709=AXIS2_PLACEMENT_3D ( 'NONE', #37074, #16545, #25247 ) ;
#26711=EDGE_LOOP ( 'NONE', ( #34409, #20754, #49378, #30693, #39937, #7408 ) ) ;
#26714=( BOUNDED_CURVE ( )  B_SPLINE_CURVE ( 3, ( #14458, #5997, #33470, #45722 ),
 .UNSPECIFIED., .F., .F. ) 
 B_SPLINE_CURVE_WITH_KNOTS ( ( 4, 4 ),
 ( 1.570796326794896558, 3.141592653589793116 ),
 .UNSPECIFIED. ) 
 CURVE ( )  GEOMETRIC_REPRESENTATION_ITEM ( )  RATIONAL_B_SPLINE_CURVE ( ( 1.000000000000000000, 0.8047378541243649375, 0.8047378541243649375, 1.000000000000000000 ) ) 
 REPRESENTATION_ITEM ( '' )  );
#26716=CARTESIAN_POINT ( 'NONE',  ( -4.945973446814916130, 1.025126265847097429, -120.9317124430720440 ) ) ;
#26717=ADVANCED_FACE ( 'NONE', ( #12480 ), #691, .T. ) ;
#26718=CARTESIAN_POINT ( 'NONE',  ( -166.6959734468149463, 1.750000000000010658, 80.81828755692798438 ) ) ;
#26730=CARTESIAN_POINT ( 'NONE',  ( -86.69597344681494633, 1.750000000000009992, -159.1817124430720298 ) ) ;
#26738=CARTESIAN_POINT ( 'NONE',  ( 155.0540265531850537, 1.025126265847089435, 2.568287556927986159 ) ) ;
#26741=CARTESIAN_POINT ( 'NONE',  ( -168.4459734468149463, 0.000000000000000000, -120.9317124430720156 ) ) ;
#26752=CARTESIAN_POINT ( 'NONE',  ( 191.5540265531851105, 0.000000000000000000, -157.4317124430720582 ) ) ;
#26753=ORIENTED_EDGE ( 'NONE', *, *, #1857, .F. ) ;
#26757=EDGE_LOOP ( 'NONE', ( #17903, #12531, #19321, #4575, #85, #29184 ) ) ;
#26760=FACE_OUTER_BOUND ( 'NONE', #7071, .T. ) ;
#26761=DIRECTION ( 'NONE',  ( -1.000000000000000000, 0.000000000000000000, 0.000000000000000000 ) ) ;
#26762=ORIENTED_EDGE ( 'NONE', *, *, #19758, .F. ) ;
#26766=( BOUNDED_CURVE ( )  B_SPLINE_CURVE ( 3, ( #31379, #12123, #11104, #50299 ),
 .UNSPECIFIED., .F., .F. ) 
 B_SPLINE_CURVE_WITH_KNOTS ( ( 4, 4 ),
 ( 4.712388980384689674, 6.283185307179586232 ),
 .UNSPECIFIED. ) 
 CURVE ( )  GEOMETRIC_REPRESENTATION_ITEM ( )  RATIONAL_B_SPLINE_CURVE ( ( 1.000000000000000000, 0.8047378541243649375, 0.8047378541243649375, 1.000000000000000000 ) ) 
 REPRESENTATION_ITEM ( '' )  );
#26768=EDGE_CURVE ( 'NONE', #2436, #46647, #27901, .T. ) ;
#26773=EDGE_LOOP ( 'NONE', ( #47902, #22956, #23334, #16117, #10718, #13071 ) ) ;
#26777=( BOUNDED_CURVE ( )  B_SPLINE_CURVE ( 3, ( #4915, #20573, #41084, #36500 ),
 .UNSPECIFIED., .F., .F. ) 
 B_SPLINE_CURVE_WITH_KNOTS ( ( 4, 4 ),
 ( 0.000000000000000000, 1.570796326794896558 ),
 .UNSPECIFIED. ) 
 CURVE ( )  GEOMETRIC_REPRESENTATION_ITEM ( )  RATIONAL_B_SPLINE_CURVE ( ( 1.000000000000000000, 0.8047378541243649375, 0.8047378541243649375, 1.000000000000000000 ) ) 
 REPRESENTATION_ITEM ( '' )  );
#26778=CARTESIAN_POINT ( 'NONE',  ( 210.0000000000000568, 0.000000000000000000, 120.8182875569279702 ) ) ;
#26779=EDGE_CURVE ( 'NONE', #8816, #23986, #23329, .T. ) ;
#26782=EDGE_CURVE ( 'NONE', #27194, #38568, #16446, .T. ) ;
#26786=EDGE_LOOP ( 'NONE', ( #36980, #36462, #50574, #24165, #4747, #4324 ) ) ;
#26788=CARTESIAN_POINT ( 'NONE',  ( 73.30402655318508209, -1.750000000000010214, 40.81828755692798438 ) ) ;
#26791=ORIENTED_EDGE ( 'NONE', *, *, #7993, .F. ) ;
#26792=DIRECTION ( 'NONE',  ( 0.000000000000000000, 0.000000000000000000, 1.000000000000000000 ) ) ;
#26795=CYLINDRICAL_SURFACE ( 'NONE', #1475, 1.750000000000008438 ) ;
#26797=CYLINDRICAL_SURFACE ( 'NONE', #19556, 1.750000000000001554 ) ;
#26802=FACE_OUTER_BOUND ( 'NONE', #22586, .T. ) ;
#26811=EDGE_CURVE ( 'NONE', #12229, #10849, #22211, .T. ) ;
#26820=ORIENTED_EDGE ( 'NONE', *, *, #37276, .F. ) ;
#26825=AXIS2_PLACEMENT_3D ( 'NONE', #22802, #43309, #38724 ) ;
#26826=EDGE_LOOP ( 'NONE', ( #50074, #6150, #45134, #41425, #15403, #11851 ) ) ;
#26827=EDGE_CURVE ( 'NONE', #36974, #9702, #21376, .T. ) ;
#26828=ORIENTED_EDGE ( 'NONE', *, *, #40658, .F. ) ;
#26831=CARTESIAN_POINT ( 'NONE',  ( 193.3040265531851105, -1.750000000000010214, -39.18171244307202983 ) ) ;
#26832=ORIENTED_EDGE ( 'NONE', *, *, #11357, .T. ) ;
#26833=ORIENTED_EDGE ( 'NONE', *, *, #11138, .F. ) ;
#26834=ORIENTED_EDGE ( 'NONE', *, *, #13949, .T. ) ;
#26836=CARTESIAN_POINT ( 'NONE',  ( 210.0000000000000568, 2.143131898507881856E-16, 79.06828755692797017 ) ) ;
#26837=VERTEX_POINT ( 'NONE', #13493 ) ;
#26842=CARTESIAN_POINT ( 'NONE',  ( -4.945973446814903696, 2.143131898507912917E-16, 165.0000000000000000 ) ) ;
#26843=EDGE_CURVE ( 'NONE', #7812, #6992, #37387, .T. ) ;
#26849=CARTESIAN_POINT ( 'NONE',  ( 151.5540265531850537, 0.000000000000000000, -120.9317124430720156 ) ) ;
#26850=DIRECTION ( 'NONE',  ( -1.000000000000000000, 0.000000000000000000, 0.000000000000000000 ) ) ;
#26860=ADVANCED_FACE ( 'NONE', ( #21194 ), #9899, .T. ) ;
#26862=ORIENTED_EDGE ( 'NONE', *, *, #222, .T. ) ;
#26864=EDGE_CURVE ( 'NONE', #46895, #29584, #21679, .T. ) ;
#26865=CARTESIAN_POINT ( 'NONE',  ( 32.27890028733795447, -1.750000000000010214, 79.79316129108087807 ) ) ;
#26870=DIRECTION ( 'NONE',  ( 0.000000000000000000, 0.000000000000000000, 1.000000000000000000 ) ) ;
#26875=CARTESIAN_POINT ( 'NONE',  ( -204.9459734468149463, 2.143131898507880377E-16, 165.0000000000000000 ) ) ;
#26878=VERTEX_POINT ( 'NONE', #33770 ) ;
#26880=EDGE_LOOP ( 'NONE', ( #12931, #37095, #20208, #9154, #24541, #27736 ) ) ;
#26882=LINE ( 'NONE', #3514, #29561 ) ;
#26888=VERTEX_POINT ( 'NONE', #30940 ) ;
#26894=FACE_OUTER_BOUND ( 'NONE', #42783, .T. ) ;
#26900=DIRECTION ( 'NONE',  ( 0.000000000000000000, 0.000000000000000000, -1.000000000000000000 ) ) ;
#26902=VERTEX_POINT ( 'NONE', #7315 ) ;
#26904=CARTESIAN_POINT ( 'NONE',  ( -8.445973446814976526, 0.000000000000000000, -120.9317124430720725 ) ) ;
#26905=( BOUNDED_CURVE ( )  B_SPLINE_CURVE ( 3, ( #47633, #28441, #16131, #23831 ),
 .UNSPECIFIED., .F., .F. ) 
 B_SPLINE_CURVE_WITH_KNOTS ( ( 4, 4 ),
 ( 1.570796326794896558, 3.141592653589793116 ),
 .UNSPECIFIED. ) 
 CURVE ( )  GEOMETRIC_REPRESENTATION_ITEM ( )  RATIONAL_B_SPLINE_CURVE ( ( 1.000000000000000000, 0.8047378541243649375, 0.8047378541243649375, 1.000000000000000000 ) ) 
 REPRESENTATION_ITEM ( '' )  );
#26909=CARTESIAN_POINT ( 'NONE',  ( 210.0000000000000568, 2.143131898507881856E-16, -120.9317124430720582 ) ) ;
#26910=DIRECTION ( 'NONE',  ( -1.000000000000000000, 0.000000000000000000, 0.000000000000000000 ) ) ;
#26911=DIRECTION ( 'NONE',  ( -0.000000000000000000, -0.000000000000000000, -1.000000000000000000 ) ) ;
#26925=CARTESIAN_POINT ( 'NONE',  ( 111.5540265531850537, -1.025126265847081442, -160.9317124430720014 ) ) ;
#26931=FACE_OUTER_BOUND ( 'NONE', #4616, .T. ) ;
#26932=VECTOR ( 'NONE', #27885, 1000.000000000000000 ) ;
#26933=ORIENTED_EDGE ( 'NONE', *, *, #24034, .T. ) ;
#26938=CARTESIAN_POINT ( 'NONE',  ( 210.0000000000000568, 0.000000000000000000, 162.5682875569279702 ) ) ;
#26945=CARTESIAN_POINT ( 'NONE',  ( 191.5540265531851105, 0.000000000000000000, 82.56828755692798438 ) ) ;
#26948=CARTESIAN_POINT ( 'NONE',  ( -204.9459734468149463, 2.143131898507880377E-16, -160.9317124430720014 ) ) ;
#26949=CARTESIAN_POINT ( 'NONE',  ( -44.94597344681493922, 2.143131898507880377E-16, 2.568287556927978166 ) ) ;
#26954=ORIENTED_EDGE ( 'NONE', *, *, #9948, .T. ) ;
#26958=LINE ( 'NONE', #39035, #46636 ) ;
#26959=EDGE_CURVE ( 'NONE', #47057, #7107, #39092, .T. ) ;
#26967=PLANE ( 'NONE',  #10798 ) ;
#26969=ORIENTED_EDGE ( 'NONE', *, *, #16565, .T. ) ;
#26978=AXIS2_PLACEMENT_3D ( 'NONE', #15210, #14952, #42893 ) ;
#26982=CARTESIAN_POINT ( 'NONE',  ( 210.0000000000000568, 2.143131898507881856E-16, 119.0682875569279560 ) ) ;
#26984=ORIENTED_EDGE ( 'NONE', *, *, #40688, .T. ) ;
#26985=CARTESIAN_POINT ( 'NONE',  ( 154.3291528190321458, 1.750000000000009548, 39.79316129108089228 ) ) ;
#26989=CARTESIAN_POINT ( 'NONE',  ( -168.4459734468149747, 1.025126265847089435, 82.56828755692798438 ) ) ;
#26990=EDGE_LOOP ( 'NONE', ( #17223, #49728, #2660, #10625, #15846, #44221 ) ) ;
#26995=CARTESIAN_POINT ( 'NONE',  ( -46.69597344681494633, 0.000000000000000000, 165.0000000000000000 ) ) ;
#26996=DIRECTION ( 'NONE',  ( -1.000000000000000000, -0.000000000000000000, -0.000000000000000000 ) ) ;
#26997=DIRECTION ( 'NONE',  ( -1.000000000000000000, -0.000000000000000000, -0.000000000000000000 ) ) ;
#26999=ORIENTED_EDGE ( 'NONE', *, *, #49536, .T. ) ;
#27004=ORIENTED_EDGE ( 'NONE', *, *, #1726, .T. ) ;
#27006=( BOUNDED_CURVE ( )  B_SPLINE_CURVE ( 3, ( #12934, #37080, #43733, #910 ),
 .UNSPECIFIED., .F., .F. ) 
 B_SPLINE_CURVE_WITH_KNOTS ( ( 4, 4 ),
 ( 1.570796326794896558, 3.141592653589793116 ),
 .UNSPECIFIED. ) 
 CURVE ( )  GEOMETRIC_REPRESENTATION_ITEM ( )  RATIONAL_B_SPLINE_CURVE ( ( 1.000000000000000000, 0.8047378541243649375, 0.8047378541243649375, 1.000000000000000000 ) ) 
 REPRESENTATION_ITEM ( '' )  );
#27012=CARTESIAN_POINT ( 'NONE',  ( 113.3040265531850537, -1.749999999999997335, -119.1817124430720440 ) ) ;
#27017=CARTESIAN_POINT ( 'NONE',  ( -128.4459734468149463, -1.025126265847082108, -117.4317124430720440 ) ) ;
#27018=CARTESIAN_POINT ( 'NONE',  ( -86.69597344681494633, 1.750000000000010658, -119.1817124430720440 ) ) ;
#27019=FACE_OUTER_BOUND ( 'NONE', #3352, .T. ) ;
#27024=EDGE_CURVE ( 'NONE', #42417, #17157, #14757, .T. ) ;
#27032=ORIENTED_EDGE ( 'NONE', *, *, #37256, .F. ) ;
#27033=CARTESIAN_POINT ( 'NONE',  ( -88.44597344681494633, -1.025126265847089435, 39.06828755692797728 ) ) ;
#27035=EDGE_LOOP ( 'NONE', ( #45911, #35518, #1269, #30637, #44969, #28029 ) ) ;
#27036=FACE_OUTER_BOUND ( 'NONE', #14151, .T. ) ;
#27047=ORIENTED_EDGE ( 'NONE', *, *, #46824, .T. ) ;
#27049=VECTOR ( 'NONE', #45049, 1000.000000000000000 ) ;
#27063=( BOUNDED_CURVE ( )  B_SPLINE_CURVE ( 3, ( #11367, #3407, #3923, #38844 ),
 .UNSPECIFIED., .F., .F. ) 
 B_SPLINE_CURVE_WITH_KNOTS ( ( 4, 4 ),
 ( 0.000000000000000000, 1.570796326794896558 ),
 .UNSPECIFIED. ) 
 CURVE ( )  GEOMETRIC_REPRESENTATION_ITEM ( )  RATIONAL_B_SPLINE_CURVE ( ( 1.000000000000000000, 0.8047378541243649375, 0.8047378541243649375, 1.000000000000000000 ) ) 
 REPRESENTATION_ITEM ( '' )  );
#27064=CARTESIAN_POINT ( 'NONE',  ( 210.0000000000000568, 0.000000000000000000, -39.18171244307202983 ) ) ;
#27068=( BOUNDED_CURVE ( )  B_SPLINE_CURVE ( 3, ( #25543, #9641, #5023, #25049 ),
 .UNSPECIFIED., .F., .F. ) 
 B_SPLINE_CURVE_WITH_KNOTS ( ( 4, 4 ),
 ( 0.000000000000000000, 1.570796326794896558 ),
 .UNSPECIFIED. ) 
 CURVE ( )  GEOMETRIC_REPRESENTATION_ITEM ( )  RATIONAL_B_SPLINE_CURVE ( ( 1.000000000000000000, 0.8047378541243649375, 0.8047378541243649375, 1.000000000000000000 ) ) 
 REPRESENTATION_ITEM ( '' )  );
#27069=EDGE_CURVE ( 'NONE', #24870, #4802, #45470, .T. ) ;
#27070=ORIENTED_EDGE ( 'NONE', *, *, #43388, .T. ) ;
#27072=FACE_OUTER_BOUND ( 'NONE', #45159, .T. ) ;
#27074=AXIS2_PLACEMENT_3D ( 'NONE', #3132, #14693, #10591 ) ;
#27075=ADVANCED_FACE ( 'NONE', ( #9093 ), #35546, .T. ) ;
#27081=FACE_OUTER_BOUND ( 'NONE', #48768, .T. ) ;
#27083=ORIENTED_EDGE ( 'NONE', *, *, #49279, .F. ) ;
#27097=ORIENTED_EDGE ( 'NONE', *, *, #1369, .F. ) ;
#27108=CARTESIAN_POINT ( 'NONE',  ( 191.5540265531851105, 0.000000000000000000, 119.0682875569279702 ) ) ;
#27112=CARTESIAN_POINT ( 'NONE',  ( 72.27890028733797578, -1.750000000000009548, -158.1565861772249377 ) ) ;
#27118=DIRECTION ( 'NONE',  ( -1.000000000000000000, -0.000000000000000000, -0.000000000000000000 ) ) ;
#27119=ADVANCED_FACE ( 'NONE', ( #40401 ), #35299, .T. ) ;
#27121=VECTOR ( 'NONE', #45710, 1000.000000000000000 ) ;
#27124=ORIENTED_EDGE ( 'NONE', *, *, #7377, .F. ) ;
#27127=CARTESIAN_POINT ( 'NONE',  ( 210.0000000000000568, 0.000000000000000000, -37.43171244307202272 ) ) ;
#27136=CARTESIAN_POINT ( 'NONE',  ( -125.6708471809678542, 1.749999999999996891, 121.8434138227750481 ) ) ;
#27138=CARTESIAN_POINT ( 'NONE',  ( -88.44597344681497475, 0.000000000000000000, 42.56828755692799859 ) ) ;
#27145=CARTESIAN_POINT ( 'NONE',  ( 71.55402655318505367, 0.000000000000000000, -37.43171244307200141 ) ) ;
#27146=CARTESIAN_POINT ( 'NONE',  ( -6.695973446814940111, -1.750000000000023315, 160.8182875569279702 ) ) ;
#27152=CARTESIAN_POINT ( 'NONE',  ( 31.55402655318506788, 0.000000000000000000, 162.5682875569279702 ) ) ;
#27156=EDGE_CURVE ( 'NONE', #47093, #18308, #37145, .T. ) ;
#27160=ORIENTED_EDGE ( 'NONE', *, *, #47904, .F. ) ;
#27161=VERTEX_POINT ( 'NONE', #29348 ) ;
#27163=EDGE_CURVE ( 'NONE', #19943, #25904, #26625, .T. ) ;
#27166=CARTESIAN_POINT ( 'NONE',  ( 153.3040265531850537, -1.750000000000009992, 0.8182875569279768335 ) ) ;
#27168=VERTEX_POINT ( 'NONE', #25000 ) ;
#27170=CARTESIAN_POINT ( 'NONE',  ( 31.55402655318503236, 0.000000000000000000, 2.568287556927978166 ) ) ;
#27178=CYLINDRICAL_SURFACE ( 'NONE', #10076, 1.749999999999973799 ) ;
#27179=EDGE_LOOP ( 'NONE', ( #48292, #43532, #800, #8901, #14631, #41539 ) ) ;
#27187=DIRECTION ( 'NONE',  ( -0.000000000000000000, -0.000000000000000000, -1.000000000000000000 ) ) ;
#27191=CARTESIAN_POINT ( 'NONE',  ( 210.0000000000000568, 2.143131898507880377E-16, -0.9317124430720331585 ) ) ;
#27193=DIRECTION ( 'NONE',  ( -1.000000000000000000, -0.000000000000000000, -0.000000000000000000 ) ) ;
#27194=VERTEX_POINT ( 'NONE', #29098 ) ;
#27197=DIRECTION ( 'NONE',  ( -0.000000000000000000, -0.000000000000000000, -1.000000000000000000 ) ) ;
#27200=CARTESIAN_POINT ( 'NONE',  ( -125.6708471809678542, 1.749999999999996891, -78.15658617722492352 ) ) ;
#27201=ADVANCED_FACE ( 'NONE', ( #20886 ), #36573, .T. ) ;
#27204=ORIENTED_EDGE ( 'NONE', *, *, #23378, .T. ) ;
#27205=ORIENTED_EDGE ( 'NONE', *, *, #17136, .T. ) ;
#27215=( BOUNDED_CURVE ( )  B_SPLINE_CURVE ( 3, ( #32751, #12737, #36631, #4777 ),
 .UNSPECIFIED., .F., .F. ) 
 B_SPLINE_CURVE_WITH_KNOTS ( ( 4, 4 ),
 ( 1.570796326794896558, 3.141592653589793116 ),
 .UNSPECIFIED. ) 
 CURVE ( )  GEOMETRIC_REPRESENTATION_ITEM ( )  RATIONAL_B_SPLINE_CURVE ( ( 1.000000000000000000, 0.8047378541243649375, 0.8047378541243649375, 1.000000000000000000 ) ) 
 REPRESENTATION_ITEM ( '' )  );
#27216=EDGE_CURVE ( 'NONE', #42459, #25772, #2055, .T. ) ;
#27222=DIRECTION ( 'NONE',  ( 0.000000000000000000, 0.000000000000000000, 1.000000000000000000 ) ) ;
#27223=( BOUNDED_CURVE ( )  B_SPLINE_CURVE ( 3, ( #10633, #34252, #26043, #40934 ),
 .UNSPECIFIED., .F., .F. ) 
 B_SPLINE_CURVE_WITH_KNOTS ( ( 4, 4 ),
 ( 1.570796326794896558, 3.141592653589793116 ),
 .UNSPECIFIED. ) 
 CURVE ( )  GEOMETRIC_REPRESENTATION_ITEM ( )  RATIONAL_B_SPLINE_CURVE ( ( 1.000000000000000000, 0.8047378541243649375, 0.8047378541243649375, 1.000000000000000000 ) ) 
 REPRESENTATION_ITEM ( '' )  );
#27230=ADVANCED_FACE ( 'NONE', ( #48291 ), #1898, .T. ) ;
#27235=VECTOR ( 'NONE', #19377, 1000.000000000000000 ) ;
#27236=ORIENTED_EDGE ( 'NONE', *, *, #25801, .T. ) ;
#27238=ADVANCED_FACE ( 'NONE', ( #46722 ), #41649, .T. ) ;
#27239=( BOUNDED_CURVE ( )  B_SPLINE_CURVE ( 3, ( #25585, #49639, #3222, #41225 ),
 .UNSPECIFIED., .F., .F. ) 
 B_SPLINE_CURVE_WITH_KNOTS ( ( 4, 4 ),
 ( 1.570796326794896558, 3.141592653589793116 ),
 .UNSPECIFIED. ) 
 CURVE ( )  GEOMETRIC_REPRESENTATION_ITEM ( )  RATIONAL_B_SPLINE_CURVE ( ( 1.000000000000000000, 0.8047378541243649375, 0.8047378541243649375, 1.000000000000000000 ) ) 
 REPRESENTATION_ITEM ( '' )  );
#27241=ORIENTED_EDGE ( 'NONE', *, *, #12442, .F. ) ;
#27246=CARTESIAN_POINT ( 'NONE',  ( -204.9459734468149463, 2.143131898507880377E-16, -157.4317124430720582 ) ) ;
#27247=DIRECTION ( 'NONE',  ( -0.000000000000000000, -0.000000000000000000, -1.000000000000000000 ) ) ;
#27249=CARTESIAN_POINT ( 'NONE',  ( 194.3291528190321742, -1.750000000000010436, 119.7931612910808781 ) ) ;
#27252=DIRECTION ( 'NONE',  ( 0.000000000000000000, 0.000000000000000000, 1.000000000000000000 ) ) ;
#27253=EDGE_LOOP ( 'NONE', ( #9044, #34756, #38383, #8687, #36361 ) ) ;
#27256=CARTESIAN_POINT ( 'NONE',  ( 114.3291528190321173, 1.749999999999996669, -160.2068387089191219 ) ) ;
#27260=DIRECTION ( 'NONE',  ( 0.000000000000000000, 0.000000000000000000, 1.000000000000000000 ) ) ;
#27266=ADVANCED_FACE ( 'NONE', ( #3393 ), #38582, .T. ) ;
#27273=CARTESIAN_POINT ( 'NONE',  ( 210.0000000000000568, 2.143131898507881856E-16, -120.9317124430720582 ) ) ;
#27278=CARTESIAN_POINT ( 'NONE',  ( -206.6959734468149463, -1.750000000000010214, 40.81828755692798438 ) ) ;
#27280=LINE ( 'NONE', #86, #44565 ) ;
#27284=CARTESIAN_POINT ( 'NONE',  ( 153.3040265531850537, -1.750000000000010658, 80.81828755692798438 ) ) ;
#27299=EDGE_LOOP ( 'NONE', ( #18937, #20625, #33862, #28980, #32255, #41929 ) ) ;
#27305=CARTESIAN_POINT ( 'NONE',  ( -85.67084718096784002, -1.750000000000010436, 119.7931612910808781 ) ) ;
#27310=ORIENTED_EDGE ( 'NONE', *, *, #40658, .T. ) ;
#27313=CARTESIAN_POINT ( 'NONE',  ( -167.7210997126620384, -1.750000000000009548, 161.8434138227750907 ) ) ;
#27323=CARTESIAN_POINT ( 'NONE',  ( 115.0540265531850395, 2.143131898507847836E-16, -160.9317124430720014 ) ) ;
#27324=VECTOR ( 'NONE', #17895, 1000.000000000000000 ) ;
#27333=AXIS2_PLACEMENT_3D ( 'NONE', #48587, #13480, #18083 ) ;
#27338=CARTESIAN_POINT ( 'NONE',  ( -164.9459734468149463, 2.143131898507880377E-16, 82.56828755692798438 ) ) ;
#27340=ORIENTED_EDGE ( 'NONE', *, *, #25802, .T. ) ;
#27342=CARTESIAN_POINT ( 'NONE',  ( 195.0540265531851105, 2.143131898507890731E-16, 165.0000000000000000 ) ) ;
#27343=LINE ( 'NONE', #19120, #31665 ) ;
#27344=VERTEX_POINT ( 'NONE', #22396 ) ;
#27348=CARTESIAN_POINT ( 'NONE',  ( 71.55402655318505367, 1.025126265847089657, -120.9317124430720440 ) ) ;
#27352=ADVANCED_FACE ( 'NONE', ( #26262 ), #6495, .T. ) ;
#27353=CARTESIAN_POINT ( 'NONE',  ( -127.7210997126620242, -1.749999999999996669, 161.8434138227750907 ) ) ;
#27354=CARTESIAN_POINT ( 'NONE',  ( 192.2789002873380184, 1.750000000000009548, -118.1565861772249519 ) ) ;
#27359=LINE ( 'NONE', #42996, #30344 ) ;
#27369=AXIS2_PLACEMENT_3D ( 'NONE', #24056, #11995, #39709 ) ;
#27370=EDGE_CURVE ( 'NONE', #29584, #40814, #10847, .T. ) ;
#27371=VECTOR ( 'NONE', #44871, 1000.000000000000000 ) ;
#27376=( BOUNDED_CURVE ( )  B_SPLINE_CURVE ( 3, ( #6188, #21846, #37512, #25950 ),
 .UNSPECIFIED., .F., .F. ) 
 B_SPLINE_CURVE_WITH_KNOTS ( ( 4, 4 ),
 ( 3.141592653589793116, 4.712388980384689674 ),
 .UNSPECIFIED. ) 
 CURVE ( )  GEOMETRIC_REPRESENTATION_ITEM ( )  RATIONAL_B_SPLINE_CURVE ( ( 1.000000000000000000, 0.8047378541243649375, 0.8047378541243649375, 1.000000000000000000 ) ) 
 REPRESENTATION_ITEM ( '' )  );
#27378=EDGE_CURVE ( 'NONE', #25557, #39055, #10582, .T. ) ;
#27381=EDGE_CURVE ( 'NONE', #27344, #42411, #30217, .T. ) ;
#27384=VECTOR ( 'NONE', #24028, 1000.000000000000000 ) ;
#27388=LINE ( 'NONE', #26875, #273 ) ;
#27391=CARTESIAN_POINT ( 'NONE',  ( 115.0540265531850395, 2.143131898507847836E-16, -80.93171244307201562 ) ) ;
#27393=ORIENTED_EDGE ( 'NONE', *, *, #33478, .F. ) ;
#27395=DIRECTION ( 'NONE',  ( -1.000000000000000000, -0.000000000000000000, -0.000000000000000000 ) ) ;
#27396=VERTEX_POINT ( 'NONE', #18539 ) ;
#27398=DIRECTION ( 'NONE',  ( -0.000000000000000000, -0.000000000000000000, -1.000000000000000000 ) ) ;
#27399=AXIS2_PLACEMENT_3D ( 'NONE', #34339, #19171, #24321 ) ;
#27404=VECTOR ( 'NONE', #2542, 1000.000000000000000 ) ;
#27406=EDGE_CURVE ( 'NONE', #41782, #48234, #15838, .T. ) ;
#27407=ORIENTED_EDGE ( 'NONE', *, *, #37119, .T. ) ;
#27409=DIRECTION ( 'NONE',  ( 0.000000000000000000, 0.000000000000000000, 1.000000000000000000 ) ) ;
#27413=ORIENTED_EDGE ( 'NONE', *, *, #3635, .F. ) ;
#27417=ORIENTED_EDGE ( 'NONE', *, *, #26130, .F. ) ;
#27423=CARTESIAN_POINT ( 'NONE',  ( 151.5540265531850537, 0.000000000000000000, -37.43171244307205825 ) ) ;
#27424=CARTESIAN_POINT ( 'NONE',  ( 32.27890028733795447, -1.750000000000009548, -38.15658617722494483 ) ) ;
#27425=CARTESIAN_POINT ( 'NONE',  ( -205.6708471809678827, 1.750000000000010214, -80.20683870891910772 ) ) ;
#27429=CARTESIAN_POINT ( 'NONE',  ( -4.945973446814903696, 2.143131898507912917E-16, -37.43171244307200141 ) ) ;
#27431=LINE ( 'NONE', #27685, #30802 ) ;
#27434=FACE_OUTER_BOUND ( 'NONE', #12897, .T. ) ;
#27437=DIRECTION ( 'NONE',  ( -0.000000000000000000, -0.000000000000000000, -1.000000000000000000 ) ) ;
#27438=CARTESIAN_POINT ( 'NONE',  ( -88.44597344681497475, 0.000000000000000000, -77.43171244307198720 ) ) ;
#27439=EDGE_CURVE ( 'NONE', #38609, #31704, #14489, .T. ) ;
#27445=DIRECTION ( 'NONE',  ( 0.000000000000000000, 0.000000000000000000, 1.000000000000000000 ) ) ;
#27446=ADVANCED_FACE ( 'NONE', ( #8283 ), #4175, .T. ) ;
#27447=ORIENTED_EDGE ( 'NONE', *, *, #13284, .T. ) ;
#27451=CYLINDRICAL_SURFACE ( 'NONE', #19718, 1.750000000000015543 ) ;
#27453=EDGE_CURVE ( 'NONE', #35686, #15022, #20071, .T. ) ;
#27455=ORIENTED_EDGE ( 'NONE', *, *, #22940, .T. ) ;
#27460=CARTESIAN_POINT ( 'NONE',  ( 73.30402655318508209, -1.750000000000009992, 160.8182875569279702 ) ) ;
#27461=CARTESIAN_POINT ( 'NONE',  ( -204.9459734468149463, 2.143131898507880377E-16, 122.5682875569279702 ) ) ;
#27463=ORIENTED_EDGE ( 'NONE', *, *, #21594, .F. ) ;
#27464=DIRECTION ( 'NONE',  ( -0.000000000000000000, -0.000000000000000000, -1.000000000000000000 ) ) ;
#27470=CARTESIAN_POINT ( 'NONE',  ( -86.69597344681494633, -1.750000000000010658, -119.1817124430720440 ) ) ;
#27477=EDGE_LOOP ( 'NONE', ( #37351, #42333, #48175, #26006, #37765, #15565 ) ) ;
#27485=CYLINDRICAL_SURFACE ( 'NONE', #15715, 1.750000000000015543 ) ;
#27490=CYLINDRICAL_SURFACE ( 'NONE', #28900, 1.749999999999973799 ) ;
#27492=VERTEX_POINT ( 'NONE', #39849 ) ;
#27494=DIRECTION ( 'NONE',  ( -0.000000000000000000, -0.000000000000000000, -1.000000000000000000 ) ) ;
#27496=AXIS2_PLACEMENT_3D ( 'NONE', #12923, #48038, #1150 ) ;
#27497=CYLINDRICAL_SURFACE ( 'NONE', #14382, 1.749999999999973799 ) ;
#27499=ADVANCED_FACE ( 'NONE', ( #4683 ), #20576, .T. ) ;
#27500=VECTOR ( 'NONE', #16907, 1000.000000000000000 ) ;
#27501=CARTESIAN_POINT ( 'NONE',  ( -166.6959734468149463, 1.750000000000010214, 40.81828755692798438 ) ) ;
#27502=ORIENTED_EDGE ( 'NONE', *, *, #37460, .F. ) ;
#27505=FACE_OUTER_BOUND ( 'NONE', #21709, .T. ) ;
#27509=ORIENTED_EDGE ( 'NONE', *, *, #41644, .F. ) ;
#27510=CARTESIAN_POINT ( 'NONE',  ( 151.5540265531850537, 0.000000000000000000, -40.93171244307202983 ) ) ;
#27513=CARTESIAN_POINT ( 'NONE',  ( -210.0000000000000568, 2.143131898507880377E-16, -0.9317124430720331585 ) ) ;
#27518=EDGE_CURVE ( 'NONE', #14142, #45927, #31891, .T. ) ;
#27520=DIRECTION ( 'NONE',  ( -1.000000000000000000, -0.000000000000000000, -0.000000000000000000 ) ) ;
#27525=EDGE_CURVE ( 'NONE', #48817, #9702, #16144, .T. ) ;
#27526=( BOUNDED_CURVE ( )  B_SPLINE_CURVE ( 3, ( #12358, #40329, #24183, #36498 ),
 .UNSPECIFIED., .F., .F. ) 
 B_SPLINE_CURVE_WITH_KNOTS ( ( 4, 4 ),
 ( 0.000000000000000000, 1.570796326794896780 ),
 .UNSPECIFIED. ) 
 CURVE ( )  GEOMETRIC_REPRESENTATION_ITEM ( )  RATIONAL_B_SPLINE_CURVE ( ( 1.000000000000000000, 0.8047378541243649375, 0.8047378541243649375, 1.000000000000000000 ) ) 
 REPRESENTATION_ITEM ( '' )  );
#27531=FACE_OUTER_BOUND ( 'NONE', #17097, .T. ) ;
#27534=( BOUNDED_CURVE ( )  B_SPLINE_CURVE ( 3, ( #22489, #17629, #34054, #33548 ),
 .UNSPECIFIED., .F., .F. ) 
 B_SPLINE_CURVE_WITH_KNOTS ( ( 4, 4 ),
 ( 3.141592653589793116, 4.712388980384689674 ),
 .UNSPECIFIED. ) 
 CURVE ( )  GEOMETRIC_REPRESENTATION_ITEM ( )  RATIONAL_B_SPLINE_CURVE ( ( 1.000000000000000000, 0.8047378541243649375, 0.8047378541243649375, 1.000000000000000000 ) ) 
 REPRESENTATION_ITEM ( '' )  );
#27538=CYLINDRICAL_SURFACE ( 'NONE', #3810, 1.750000000000008438 ) ;
#27539=VECTOR ( 'NONE', #649, 1000.000000000000000 ) ;
#27542=CARTESIAN_POINT ( 'NONE',  ( -206.6959734468149463, -1.750000000000010658, -119.1817124430720440 ) ) ;
#27544=VECTOR ( 'NONE', #35831, 1000.000000000000000 ) ;
#27548=( BOUNDED_CURVE ( )  B_SPLINE_CURVE ( 3, ( #30330, #49772, #22876, #45941 ),
 .UNSPECIFIED., .F., .F. ) 
 B_SPLINE_CURVE_WITH_KNOTS ( ( 4, 4 ),
 ( 1.570796326794896558, 3.141592653589793116 ),
 .UNSPECIFIED. ) 
 CURVE ( )  GEOMETRIC_REPRESENTATION_ITEM ( )  RATIONAL_B_SPLINE_CURVE ( ( 1.000000000000000000, 0.8047378541243649375, 0.8047378541243649375, 1.000000000000000000 ) ) 
 REPRESENTATION_ITEM ( '' )  );
#27551=CARTESIAN_POINT ( 'NONE',  ( -206.6959734468149463, -1.750000000000010658, 120.8182875569279702 ) ) ;
#27553=ORIENTED_EDGE ( 'NONE', *, *, #28345, .F. ) ;
#27554=ORIENTED_EDGE ( 'NONE', *, *, #13566, .F. ) ;
#27555=EDGE_LOOP ( 'NONE', ( #29518, #43698, #45828, #44733, #2024, #18980 ) ) ;
#27557=CARTESIAN_POINT ( 'NONE',  ( -84.94597344681494633, 2.143131898507880377E-16, -40.93171244307202983 ) ) ;
#27560=LINE ( 'NONE', #40118, #1838 ) ;
#27561=ORIENTED_EDGE ( 'NONE', *, *, #12648, .T. ) ;
#27565=ORIENTED_EDGE ( 'NONE', *, *, #31292, .F. ) ;
#27568=CARTESIAN_POINT ( 'NONE',  ( -7.721099712662037540, 1.750000000000023315, -118.1565861772249519 ) ) ;
#27576=DIRECTION ( 'NONE',  ( -1.000000000000000000, -0.000000000000000000, -0.000000000000000000 ) ) ;
#27580=EDGE_CURVE ( 'NONE', #18060, #48199, #21077, .T. ) ;
#27590=CARTESIAN_POINT ( 'NONE',  ( -128.4459734468149179, 0.000000000000000000, -37.43171244307205825 ) ) ;
#27595=ORIENTED_EDGE ( 'NONE', *, *, #25244, .T. ) ;
#27597=DIRECTION ( 'NONE',  ( -1.000000000000000000, 0.000000000000000000, 0.000000000000000000 ) ) ;
#27602=CARTESIAN_POINT ( 'NONE',  ( -124.9459734468149463, 2.143131898507847836E-16, 39.06828755692798438 ) ) ;
#27606=ORIENTED_EDGE ( 'NONE', *, *, #40659, .T. ) ;
#27611=DIRECTION ( 'NONE',  ( 0.000000000000000000, 0.000000000000000000, -1.000000000000000000 ) ) ;
#27612=VECTOR ( 'NONE', #49693, 1000.000000000000000 ) ;
#27617=CARTESIAN_POINT ( 'NONE',  ( 111.5540265531850537, 1.025126265847081442, 159.0682875569279418 ) ) ;
#27618=ADVANCED_FACE ( 'NONE', ( #32901 ), #13375, .T. ) ;
#27625=LINE ( 'NONE', #47576, #11683 ) ;
#27627=DIRECTION ( 'NONE',  ( -1.000000000000000000, 0.000000000000000000, 0.000000000000000000 ) ) ;
#27630=( BOUNDED_CURVE ( )  B_SPLINE_CURVE ( 3, ( #50088, #14999, #30658, #31169 ),
 .UNSPECIFIED., .F., .F. ) 
 B_SPLINE_CURVE_WITH_KNOTS ( ( 4, 4 ),
 ( 4.712388980384689674, 6.283185307179586232 ),
 .UNSPECIFIED. ) 
 CURVE ( )  GEOMETRIC_REPRESENTATION_ITEM ( )  RATIONAL_B_SPLINE_CURVE ( ( 1.000000000000000000, 0.8047378541243649375, 0.8047378541243649375, 1.000000000000000000 ) ) 
 REPRESENTATION_ITEM ( '' )  );
#27634=DIRECTION ( 'NONE',  ( -1.000000000000000000, -0.000000000000000000, -0.000000000000000000 ) ) ;
#27635=CARTESIAN_POINT ( 'NONE',  ( 152.2789002873379900, -1.750000000000009548, -38.15658617722494483 ) ) ;
#27636=AXIS2_PLACEMENT_3D ( 'NONE', #49560, #30373, #10609 ) ;
#27640=EDGE_LOOP ( 'NONE', ( #29764, #21553, #46348, #43712, #17685, #35564 ) ) ;
#27642=VECTOR ( 'NONE', #9429, 1000.000000000000000 ) ;
#27644=ORIENTED_EDGE ( 'NONE', *, *, #15135, .F. ) ;
#27648=ORIENTED_EDGE ( 'NONE', *, *, #39037, .T. ) ;
#27649=CARTESIAN_POINT ( 'NONE',  ( -165.6708471809677974, -1.750000000000009548, -118.1565861772249519 ) ) ;
#27650=VERTEX_POINT ( 'NONE', #26948 ) ;
#27651=ORIENTED_EDGE ( 'NONE', *, *, #23634, .T. ) ;
#27653=CARTESIAN_POINT ( 'NONE',  ( -86.69597344681494633, -1.750000000000010214, -39.18171244307202983 ) ) ;
#27654=EDGE_LOOP ( 'NONE', ( #21760, #42234, #7700, #43908, #9518, #5427 ) ) ;
#27661=ORIENTED_EDGE ( 'NONE', *, *, #42894, .F. ) ;
#27663=FACE_OUTER_BOUND ( 'NONE', #26826, .T. ) ;
#27669=EDGE_LOOP ( 'NONE', ( #1767, #33524, #44536, #26576, #21863, #32153 ) ) ;
#27670=CARTESIAN_POINT ( 'NONE',  ( -206.6959734468149463, -1.750000000000010658, 80.81828755692798438 ) ) ;
#27673=( BOUNDED_CURVE ( )  B_SPLINE_CURVE ( 3, ( #11442, #43243, #50392, #11694 ),
 .UNSPECIFIED., .F., .F. ) 
 B_SPLINE_CURVE_WITH_KNOTS ( ( 4, 4 ),
 ( 3.141592653589793116, 4.712388980384689674 ),
 .UNSPECIFIED. ) 
 CURVE ( )  GEOMETRIC_REPRESENTATION_ITEM ( )  RATIONAL_B_SPLINE_CURVE ( ( 1.000000000000000000, 0.8047378541243649375, 0.8047378541243649375, 1.000000000000000000 ) ) 
 REPRESENTATION_ITEM ( '' )  );
#27675=CARTESIAN_POINT ( 'NONE',  ( -84.94597344681493212, 1.025126265847088991, 162.5682875569279133 ) ) ;
#27681=( BOUNDED_CURVE ( )  B_SPLINE_CURVE ( 3, ( #48071, #8378, #27878, #47823 ),
 .UNSPECIFIED., .F., .F. ) 
 B_SPLINE_CURVE_WITH_KNOTS ( ( 4, 4 ),
 ( 3.141592653589793116, 4.712388980384689674 ),
 .UNSPECIFIED. ) 
 CURVE ( )  GEOMETRIC_REPRESENTATION_ITEM ( )  RATIONAL_B_SPLINE_CURVE ( ( 1.000000000000000000, 0.8047378541243649375, 0.8047378541243649375, 1.000000000000000000 ) ) 
 REPRESENTATION_ITEM ( '' )  );
#27685=CARTESIAN_POINT ( 'NONE',  ( -164.9459734468149463, 2.143131898507880377E-16, 165.0000000000000000 ) ) ;
#27692=LINE ( 'NONE', #20242, #5646 ) ;
#27693=CARTESIAN_POINT ( 'NONE',  ( 193.3040265531851105, -1.750000000000010658, -119.1817124430720440 ) ) ;
#27697=ORIENTED_EDGE ( 'NONE', *, *, #34002, .F. ) ;
#27700=VERTEX_POINT ( 'NONE', #46416 ) ;
#27703=CARTESIAN_POINT ( 'NONE',  ( 193.3040265531851105, 1.750000000000010658, 120.8182875569279702 ) ) ;
#27706=ORIENTED_EDGE ( 'NONE', *, *, #39961, .F. ) ;
#27708=EDGE_CURVE ( 'NONE', #33144, #4629, #35191, .T. ) ;
#27711=DIRECTION ( 'NONE',  ( -1.000000000000000000, 0.000000000000000000, 0.000000000000000000 ) ) ;
#27720=EDGE_CURVE ( 'NONE', #6739, #22212, #30299, .T. ) ;
#27722=CARTESIAN_POINT ( 'NONE',  ( 210.0000000000000568, 0.000000000000000000, 82.56828755692799859 ) ) ;
#27723=CARTESIAN_POINT ( 'NONE',  ( 155.0540265531850537, -1.025126265847089435, 39.06828755692797728 ) ) ;
#27724=ORIENTED_EDGE ( 'NONE', *, *, #49624, .F. ) ;
#27725=DIRECTION ( 'NONE',  ( -1.000000000000000000, -0.000000000000000000, -0.000000000000000000 ) ) ;
#27731=DIRECTION ( 'NONE',  ( 0.000000000000000000, 0.000000000000000000, 1.000000000000000000 ) ) ;
#27733=LINE ( 'NONE', #27981, #11484 ) ;
#27736=ORIENTED_EDGE ( 'NONE', *, *, #14612, .T. ) ;
#27737=CARTESIAN_POINT ( 'NONE',  ( -46.69597344681494633, 0.000000000000000000, 165.0000000000000000 ) ) ;
#27738=EDGE_CURVE ( 'NONE', #40327, #960, #10788, .T. ) ;
#27747=VECTOR ( 'NONE', #10133, 1000.000000000000000 ) ;
#27749=ORIENTED_EDGE ( 'NONE', *, *, #37839, .F. ) ;
#27751=DIRECTION ( 'NONE',  ( -0.000000000000000000, -0.000000000000000000, -1.000000000000000000 ) ) ;
#27755=DIRECTION ( 'NONE',  ( -1.000000000000000000, -0.000000000000000000, -0.000000000000000000 ) ) ;
#27756=ORIENTED_EDGE ( 'NONE', *, *, #15031, .F. ) ;
#27757=EDGE_CURVE ( 'NONE', #45661, #33640, #28576, .T. ) ;
#27758=CARTESIAN_POINT ( 'NONE',  ( -84.94597344681494633, 2.143131898507880377E-16, 2.568287556927978166 ) ) ;
#27761=DIRECTION ( 'NONE',  ( -1.000000000000000000, 0.000000000000000000, 0.000000000000000000 ) ) ;
#27762=ORIENTED_EDGE ( 'NONE', *, *, #3410, .T. ) ;
#27765=DIRECTION ( 'NONE',  ( -1.000000000000000000, -0.000000000000000000, -0.000000000000000000 ) ) ;
#27766=CARTESIAN_POINT ( 'NONE',  ( 193.3040265531851105, 1.750000000000010214, 40.81828755692798438 ) ) ;
#27768=EDGE_CURVE ( 'NONE', #47057, #45409, #19431, .T. ) ;
#27770=CARTESIAN_POINT ( 'NONE',  ( 152.2789002873379900, 1.750000000000009548, -78.15658617722490931 ) ) ;
#27774=CARTESIAN_POINT ( 'NONE',  ( 210.0000000000000568, 2.143131898507880377E-16, 159.0682875569279702 ) ) ;
#27776=ORIENTED_EDGE ( 'NONE', *, *, #4611, .F. ) ;
#27781=ORIENTED_EDGE ( 'NONE', *, *, #47915, .T. ) ;
#27782=CARTESIAN_POINT ( 'NONE',  ( -45.67084718096785423, -1.750000000000009548, -78.15658617722490931 ) ) ;
#27783=LINE ( 'NONE', #39595, #1061 ) ;
#27784=ADVANCED_FACE ( 'NONE', ( #3082 ), #47666, .T. ) ;
#27788=VERTEX_POINT ( 'NONE', #31583 ) ;
#27799=CYLINDRICAL_SURFACE ( 'NONE', #491, 1.750000000000001554 ) ;
#27800=DIRECTION ( 'NONE',  ( -1.000000000000000000, 0.000000000000000000, 0.000000000000000000 ) ) ;
#27805=CARTESIAN_POINT ( 'NONE',  ( -7.721099712662037540, -1.750000000000023315, -0.2068387089191201234 ) ) ;
#27807=EDGE_CURVE ( 'NONE', #48103, #37518, #42648, .T. ) ;
#27813=CARTESIAN_POINT ( 'NONE',  ( 33.30402655318503946, -1.750000000000009992, 160.8182875569279702 ) ) ;
#27817=EDGE_LOOP ( 'NONE', ( #20846, #40412, #22879, #12688, #36637, #15153 ) ) ;
#27819=CARTESIAN_POINT ( 'NONE',  ( -48.44597344681496054, -1.025126265847089435, 2.568287556927986159 ) ) ;
#27823=( BOUNDED_CURVE ( )  B_SPLINE_CURVE ( 3, ( #36252, #24444, #48235, #40093 ),
 .UNSPECIFIED., .F., .F. ) 
 B_SPLINE_CURVE_WITH_KNOTS ( ( 4, 4 ),
 ( 1.570796326794896558, 3.141592653589793116 ),
 .UNSPECIFIED. ) 
 CURVE ( )  GEOMETRIC_REPRESENTATION_ITEM ( )  RATIONAL_B_SPLINE_CURVE ( ( 1.000000000000000000, 0.8047378541243649375, 0.8047378541243649375, 1.000000000000000000 ) ) 
 REPRESENTATION_ITEM ( '' )  );
#27827=CARTESIAN_POINT ( 'NONE',  ( 33.30402655318503946, -1.750000000000010214, 40.81828755692798438 ) ) ;
#27831=CARTESIAN_POINT ( 'NONE',  ( -208.4459734468149463, 0.000000000000000000, 165.0000000000000000 ) ) ;
#27832=( BOUNDED_CURVE ( )  B_SPLINE_CURVE ( 3, ( #4408, #20055, #36484, #1068 ),
 .UNSPECIFIED., .F., .F. ) 
 B_SPLINE_CURVE_WITH_KNOTS ( ( 4, 4 ),
 ( 0.000000000000000000, 1.570796326794896558 ),
 .UNSPECIFIED. ) 
 CURVE ( )  GEOMETRIC_REPRESENTATION_ITEM ( )  RATIONAL_B_SPLINE_CURVE ( ( 1.000000000000000000, 0.8047378541243649375, 0.8047378541243649375, 1.000000000000000000 ) ) 
 REPRESENTATION_ITEM ( '' )  );
#27839=( BOUNDED_CURVE ( )  B_SPLINE_CURVE ( 3, ( #23112, #14654, #41605, #41856 ),
 .UNSPECIFIED., .F., .F. ) 
 B_SPLINE_CURVE_WITH_KNOTS ( ( 4, 4 ),
 ( 3.141592653589793116, 4.712388980384689674 ),
 .UNSPECIFIED. ) 
 CURVE ( )  GEOMETRIC_REPRESENTATION_ITEM ( )  RATIONAL_B_SPLINE_CURVE ( ( 1.000000000000000000, 0.8047378541243649375, 0.8047378541243649375, 1.000000000000000000 ) ) 
 REPRESENTATION_ITEM ( '' )  );
#27842=ORIENTED_EDGE ( 'NONE', *, *, #46011, .F. ) ;
#27843=CARTESIAN_POINT ( 'NONE',  ( 195.0540265531851105, 2.143131898507880377E-16, -77.43171244307204404 ) ) ;
#27845=CARTESIAN_POINT ( 'NONE',  ( -46.69597344681494633, 1.750000000000009992, -159.1817124430720298 ) ) ;
#27850=CARTESIAN_POINT ( 'NONE',  ( 193.3040265531851105, 0.000000000000000000, 165.0000000000000000 ) ) ;
#27852=FACE_OUTER_BOUND ( 'NONE', #44595, .T. ) ;
#27853=ORIENTED_EDGE ( 'NONE', *, *, #25511, .F. ) ;
#27859=ORIENTED_EDGE ( 'NONE', *, *, #44865, .T. ) ;
#27865=CARTESIAN_POINT ( 'NONE',  ( -8.445973446814962315, -1.025126265847096985, -160.9317124430720014 ) ) ;
#27870=ORIENTED_EDGE ( 'NONE', *, *, #24635, .F. ) ;
#27876=EDGE_CURVE ( 'NONE', #24506, #7778, #26330, .T. ) ;
#27878=CARTESIAN_POINT ( 'NONE',  ( 152.2789002873379900, 1.750000000000009548, 121.8434138227750623 ) ) ;
#27880=DIRECTION ( 'NONE',  ( -1.000000000000000000, 0.000000000000000000, 0.000000000000000000 ) ) ;
#27883=CARTESIAN_POINT ( 'NONE',  ( 192.2789002873380184, 1.750000000000010436, -120.2068387089191219 ) ) ;
#27885=DIRECTION ( 'NONE',  ( -1.000000000000000000, -0.000000000000000000, -0.000000000000000000 ) ) ;
#27886=LINE ( 'NONE', #28388, #48389 ) ;
#27890=CIRCLE ( 'NONE', #49946, 1.750000000000001554 ) ;
#27897=ORIENTED_EDGE ( 'NONE', *, *, #8643, .F. ) ;
#27901=LINE ( 'NONE', #4293, #45438 ) ;
#27904=CARTESIAN_POINT ( 'NONE',  ( -164.9459734468149463, 2.143131898507880377E-16, -117.4317124430720725 ) ) ;
#27909=DIRECTION ( 'NONE',  ( 1.000000000000000000, 0.000000000000000000, 0.000000000000000000 ) ) ;
#27914=CARTESIAN_POINT ( 'NONE',  ( 75.05402655318509630, 2.143131898507880377E-16, 82.56828755692799859 ) ) ;
#27919=FACE_OUTER_BOUND ( 'NONE', #22155, .T. ) ;
#27924=CARTESIAN_POINT ( 'NONE',  ( -8.445973446814976526, 0.000000000000000000, 159.0682875569279418 ) ) ;
#27926=VERTEX_POINT ( 'NONE', #36958 ) ;
#27927=VECTOR ( 'NONE', #28906, 1000.000000000000000 ) ;
#27931=CARTESIAN_POINT ( 'NONE',  ( -88.44597344681494633, -1.025126265847089213, 159.0682875569279418 ) ) ;
#27933=LINE ( 'NONE', #20231, #21624 ) ;
#27942=DIRECTION ( 'NONE',  ( -0.000000000000000000, -0.000000000000000000, -1.000000000000000000 ) ) ;
#27948=ORIENTED_EDGE ( 'NONE', *, *, #2321, .T. ) ;
#27949=CARTESIAN_POINT ( 'NONE',  ( 153.3040265531850537, 0.000000000000000000, 165.0000000000000000 ) ) ;
#27951=ORIENTED_EDGE ( 'NONE', *, *, #48358, .T. ) ;
#27953=CARTESIAN_POINT ( 'NONE',  ( 210.0000000000000568, 0.000000000000000000, 122.5682875569279844 ) ) ;
#27954=CARTESIAN_POINT ( 'NONE',  ( -46.69597344681494633, 1.750000000000009992, 0.8182875569279768335 ) ) ;
#27955=ORIENTED_EDGE ( 'NONE', *, *, #39944, .F. ) ;
#27956=CARTESIAN_POINT ( 'NONE',  ( -207.7210997126620384, 1.750000000000009548, 159.7931612910809065 ) ) ;
#27958=EDGE_CURVE ( 'NONE', #46160, #42683, #28375, .T. ) ;
#27962=ORIENTED_EDGE ( 'NONE', *, *, #42189, .T. ) ;
#27968=CARTESIAN_POINT ( 'NONE',  ( -164.9459734468149463, 2.143131898507880377E-16, -117.4317124430720725 ) ) ;
#27977=CARTESIAN_POINT ( 'NONE',  ( -88.44597344681497475, 0.000000000000000000, 119.0682875569279418 ) ) ;
#27981=CARTESIAN_POINT ( 'NONE',  ( -8.445973446814976526, 0.000000000000000000, 165.0000000000000000 ) ) ;
#27982=ORIENTED_EDGE ( 'NONE', *, *, #9507, .T. ) ;
#27985=EDGE_CURVE ( 'NONE', #28555, #24870, #48671, .T. ) ;
#27990=DIRECTION ( 'NONE',  ( -1.000000000000000000, -0.000000000000000000, -0.000000000000000000 ) ) ;
#27993=CARTESIAN_POINT ( 'NONE',  ( -127.7210997126620242, -1.749999999999996891, 81.84341382277506227 ) ) ;
#27994=LINE ( 'NONE', #23644, #17477 ) ;
#28001=CARTESIAN_POINT ( 'NONE',  ( -164.9459734468149463, 2.143131898507880377E-16, 159.0682875569279702 ) ) ;
#28002=DIRECTION ( 'NONE',  ( -1.000000000000000000, -0.000000000000000000, -0.000000000000000000 ) ) ;
#28005=ORIENTED_EDGE ( 'NONE', *, *, #1126, .F. ) ;
#28008=DIRECTION ( 'NONE',  ( -0.000000000000000000, -0.000000000000000000, -1.000000000000000000 ) ) ;
#28013=LINE ( 'NONE', #4415, #42878 ) ;
#28017=EDGE_CURVE ( 'NONE', #2042, #41270, #29920, .T. ) ;
#28019=CARTESIAN_POINT ( 'NONE',  ( 151.5540265531850537, 0.000000000000000000, -117.4317124430720725 ) ) ;
#28021=ORIENTED_EDGE ( 'NONE', *, *, #19643, .T. ) ;
#28023=CARTESIAN_POINT ( 'NONE',  ( 31.55402655318503236, 0.000000000000000000, 42.56828755692798438 ) ) ;
#28029=ORIENTED_EDGE ( 'NONE', *, *, #46279, .F. ) ;
#28035=CARTESIAN_POINT ( 'NONE',  ( -210.0000000000000568, 0.000000000000000000, 160.8182875569279702 ) ) ;
#28038=ADVANCED_FACE ( 'NONE', ( #49616 ), #8971, .T. ) ;
#28047=CARTESIAN_POINT ( 'NONE',  ( -4.945973446814916130, -1.025126265847097207, 122.5682875569280128 ) ) ;
#28048=EDGE_CURVE ( 'NONE', #40908, #32767, #3459, .T. ) ;
#28050=AXIS2_PLACEMENT_3D ( 'NONE', #1416, #4993, #47304 ) ;
#28058=DIRECTION ( 'NONE',  ( 1.000000000000000000, 0.000000000000000000, 0.000000000000000000 ) ) ;
#28063=EDGE_LOOP ( 'NONE', ( #29252, #1430 ) ) ;
#28069=DIRECTION ( 'NONE',  ( -1.000000000000000000, -0.000000000000000000, -0.000000000000000000 ) ) ;
#28072=ADVANCED_FACE ( 'NONE', ( #27081 ), #22965, .T. ) ;
#28076=CARTESIAN_POINT ( 'NONE',  ( 195.0540265531851105, 2.143131898507880377E-16, -160.9317124430720014 ) ) ;
#28077=EDGE_CURVE ( 'NONE', #37476, #2131, #47866, .T. ) ;
#28083=CARTESIAN_POINT ( 'NONE',  ( -124.9459734468149321, 1.025126265847082108, 122.5682875569279702 ) ) ;
#28084=CARTESIAN_POINT ( 'NONE',  ( -166.6959734468149463, 1.750000000000009992, -159.1817124430720298 ) ) ;
#28085=ADVANCED_FACE ( 'NONE', ( #7081 ), #42462, .T. ) ;
#28090=ORIENTED_EDGE ( 'NONE', *, *, #9502, .F. ) ;
#28092=CARTESIAN_POINT ( 'NONE',  ( 155.0540265531850537, -1.025126265847089213, -0.9317124430720324924 ) ) ;
#28093=ORIENTED_EDGE ( 'NONE', *, *, #37265, .F. ) ;
#28096=CARTESIAN_POINT ( 'NONE',  ( -205.6708471809678827, -1.750000000000010436, 79.79316129108087807 ) ) ;
#28097=CARTESIAN_POINT ( 'NONE',  ( -8.445973446814976526, 0.000000000000000000, -80.93171244307204404 ) ) ;
#28101=ORIENTED_EDGE ( 'NONE', *, *, #50627, .T. ) ;
#28103=ORIENTED_EDGE ( 'NONE', *, *, #12222, .T. ) ;
#28107=EDGE_CURVE ( 'NONE', #5706, #41541, #6820, .T. ) ;
#28109=CARTESIAN_POINT ( 'NONE',  ( -6.695973446814940111, 0.000000000000000000, 165.0000000000000000 ) ) ;
#28111=ORIENTED_EDGE ( 'NONE', *, *, #29030, .F. ) ;
#28112=DIRECTION ( 'NONE',  ( -0.000000000000000000, -0.000000000000000000, -1.000000000000000000 ) ) ;
#28113=CARTESIAN_POINT ( 'NONE',  ( 113.3040265531850537, 1.749999999999997113, -39.18171244307202983 ) ) ;
#28120=( BOUNDED_CURVE ( )  B_SPLINE_CURVE ( 3, ( #3274, #18919, #35122, #50176 ),
 .UNSPECIFIED., .F., .F. ) 
 B_SPLINE_CURVE_WITH_KNOTS ( ( 4, 4 ),
 ( 4.712388980384689674, 6.283185307179586232 ),
 .UNSPECIFIED. ) 
 CURVE ( )  GEOMETRIC_REPRESENTATION_ITEM ( )  RATIONAL_B_SPLINE_CURVE ( ( 1.000000000000000000, 0.8047378541243649375, 0.8047378541243649375, 1.000000000000000000 ) ) 
 REPRESENTATION_ITEM ( '' )  );
#28121=DIRECTION ( 'NONE',  ( -1.000000000000000000, -0.000000000000000000, -0.000000000000000000 ) ) ;
#28122=CARTESIAN_POINT ( 'NONE',  ( -84.94597344681494633, 2.143131898507880377E-16, -160.9317124430720014 ) ) ;
#28124=CARTESIAN_POINT ( 'NONE',  ( -168.4459734468149463, 0.000000000000000000, 82.56828755692798438 ) ) ;
#28128=( BOUNDED_CURVE ( )  B_SPLINE_CURVE ( 3, ( #9394, #37380, #17342, #48090 ),
 .UNSPECIFIED., .F., .F. ) 
 B_SPLINE_CURVE_WITH_KNOTS ( ( 4, 4 ),
 ( 3.141592653589793116, 4.712388980384689674 ),
 .UNSPECIFIED. ) 
 CURVE ( )  GEOMETRIC_REPRESENTATION_ITEM ( )  RATIONAL_B_SPLINE_CURVE ( ( 1.000000000000000000, 0.8047378541243649375, 0.8047378541243649375, 1.000000000000000000 ) ) 
 REPRESENTATION_ITEM ( '' )  );
#28129=DIRECTION ( 'NONE',  ( 0.000000000000000000, 0.000000000000000000, 1.000000000000000000 ) ) ;
#28131=DIRECTION ( 'NONE',  ( -0.000000000000000000, -0.000000000000000000, -1.000000000000000000 ) ) ;
#28136=( BOUNDED_CURVE ( )  B_SPLINE_CURVE ( 3, ( #27693, #35414, #15390, #18961 ),
 .UNSPECIFIED., .F., .F. ) 
 B_SPLINE_CURVE_WITH_KNOTS ( ( 4, 4 ),
 ( 4.712388980384689674, 6.283185307179586232 ),
 .UNSPECIFIED. ) 
 CURVE ( )  GEOMETRIC_REPRESENTATION_ITEM ( )  RATIONAL_B_SPLINE_CURVE ( ( 1.000000000000000000, 0.8047378541243649375, 0.8047378541243649375, 1.000000000000000000 ) ) 
 REPRESENTATION_ITEM ( '' )  );
#28138=AXIS2_PLACEMENT_3D ( 'NONE', #23084, #3072, #18715 ) ;
#28141=EDGE_CURVE ( 'NONE', #23383, #3985, #42710, .T. ) ;
#28142=EDGE_CURVE ( 'NONE', #30870, #42453, #42353, .T. ) ;
#28145=ORIENTED_EDGE ( 'NONE', *, *, #14065, .T. ) ;
#28149=EDGE_CURVE ( 'NONE', #43794, #16197, #2343, .T. ) ;
#28154=ORIENTED_EDGE ( 'NONE', *, *, #11881, .T. ) ;
#28155=CARTESIAN_POINT ( 'NONE',  ( -7.721099712662037540, 1.750000000000022427, -158.1565861772249093 ) ) ;
#28156=EDGE_CURVE ( 'NONE', #34169, #31607, #32206, .T. ) ;
#28162=CARTESIAN_POINT ( 'NONE',  ( -7.721099712662037540, -1.750000000000022871, 161.8434138227750907 ) ) ;
#28163=VERTEX_POINT ( 'NONE', #20898 ) ;
#28164=EDGE_CURVE ( 'NONE', #31704, #40007, #35492, .T. ) ;
#28165=LINE ( 'NONE', #8670, #48043 ) ;
#28166=ORIENTED_EDGE ( 'NONE', *, *, #33972, .T. ) ;
#28169=CARTESIAN_POINT ( 'NONE',  ( -164.9459734468149747, 0.000000000000000000, 162.5682875569279702 ) ) ;
#28170=DIRECTION ( 'NONE',  ( -1.000000000000000000, -0.000000000000000000, -0.000000000000000000 ) ) ;
#28177=VERTEX_POINT ( 'NONE', #28097 ) ;
#28182=AXIS2_PLACEMENT_3D ( 'NONE', #48162, #37442, #1768 ) ;
#28183=PLANE ( 'NONE',  #36469 ) ;
#28184=CARTESIAN_POINT ( 'NONE',  ( 194.3291528190321742, 1.750000000000010214, -80.20683870891910772 ) ) ;
#28185=CIRCLE ( 'NONE', #41275, 1.750000000000008438 ) ;
#28188=CARTESIAN_POINT ( 'NONE',  ( -88.44597344681497475, 0.000000000000000000, 159.0682875569279418 ) ) ;
#28190=CARTESIAN_POINT ( 'NONE',  ( 73.30402655318508209, 0.000000000000000000, 165.0000000000000000 ) ) ;
#28193=EDGE_CURVE ( 'NONE', #37343, #6842, #18080, .T. ) ;
#28194=DIRECTION ( 'NONE',  ( -1.000000000000000000, 0.000000000000000000, 0.000000000000000000 ) ) ;
#28195=VECTOR ( 'NONE', #6850, 1000.000000000000000 ) ;
#28201=CARTESIAN_POINT ( 'NONE',  ( 210.0000000000000568, 2.143131898507881116E-16, -40.93171244307203693 ) ) ;
#28203=CARTESIAN_POINT ( 'NONE',  ( 210.0000000000000568, 0.000000000000000000, -79.18171244307201562 ) ) ;
#28205=EDGE_CURVE ( 'NONE', #49797, #47427, #38780, .T. ) ;
#28213=CARTESIAN_POINT ( 'NONE',  ( -46.69597344681494633, 1.750000000000009992, 0.8182875569279768335 ) ) ;
#28223=CARTESIAN_POINT ( 'NONE',  ( -4.945973446814938335, 0.000000000000000000, 162.5682875569279702 ) ) ;
#28224=ORIENTED_EDGE ( 'NONE', *, *, #27738, .F. ) ;
#28236=ORIENTED_EDGE ( 'NONE', *, *, #30104, .T. ) ;
#28244=DIRECTION ( 'NONE',  ( 0.000000000000000000, 0.000000000000000000, 1.000000000000000000 ) ) ;
#28247=DIRECTION ( 'NONE',  ( -0.000000000000000000, -0.000000000000000000, -1.000000000000000000 ) ) ;
#28250=ORIENTED_EDGE ( 'NONE', *, *, #28393, .T. ) ;
#28255=CARTESIAN_POINT ( 'NONE',  ( 210.0000000000000568, 2.143131898507881856E-16, -80.93171244307202983 ) ) ;
#28264=CARTESIAN_POINT ( 'NONE',  ( -44.94597344681493922, 2.143131898507880377E-16, 79.06828755692797017 ) ) ;
#28265=ORIENTED_EDGE ( 'NONE', *, *, #3045, .T. ) ;
#28271=CARTESIAN_POINT ( 'NONE',  ( -205.6708471809678827, 1.750000000000009548, 159.7931612910809065 ) ) ;
#28275=ORIENTED_EDGE ( 'NONE', *, *, #1607, .F. ) ;
#28276=DIRECTION ( 'NONE',  ( -0.000000000000000000, -0.000000000000000000, -1.000000000000000000 ) ) ;
#28277=VERTEX_POINT ( 'NONE', #25763 ) ;
#28279=DIRECTION ( 'NONE',  ( -0.000000000000000000, -0.000000000000000000, -1.000000000000000000 ) ) ;
#28281=CARTESIAN_POINT ( 'NONE',  ( 210.0000000000000568, 0.000000000000000000, 80.81828755692798438 ) ) ;
#28283=( BOUNDED_CURVE ( )  B_SPLINE_CURVE ( 3, ( #29, #28484, #12827, #31840 ),
 .UNSPECIFIED., .F., .F. ) 
 B_SPLINE_CURVE_WITH_KNOTS ( ( 4, 4 ),
 ( 3.141592653589793116, 4.712388980384689674 ),
 .UNSPECIFIED. ) 
 CURVE ( )  GEOMETRIC_REPRESENTATION_ITEM ( )  RATIONAL_B_SPLINE_CURVE ( ( 1.000000000000000000, 0.8047378541243649375, 0.8047378541243649375, 1.000000000000000000 ) ) 
 REPRESENTATION_ITEM ( '' )  );
#28298=ORIENTED_EDGE ( 'NONE', *, *, #7839, .F. ) ;
#28306=CARTESIAN_POINT ( 'NONE',  ( 210.0000000000000568, 0.000000000000000000, 120.8182875569279702 ) ) ;
#28309=VERTEX_POINT ( 'NONE', #29108 ) ;
#28315=CARTESIAN_POINT ( 'NONE',  ( 35.05402655318504657, 2.143131898507880377E-16, -160.9317124430720582 ) ) ;
#28318=ORIENTED_EDGE ( 'NONE', *, *, #34611, .F. ) ;
#28327=EDGE_LOOP ( 'NONE', ( #40102, #8022, #43622, #1466, #46479 ) ) ;
#28333=CARTESIAN_POINT ( 'NONE',  ( -128.4459734468149463, 1.025126265847081664, -37.43171244307203693 ) ) ;
#28334=CARTESIAN_POINT ( 'NONE',  ( -8.445973446814976526, 0.000000000000000000, 159.0682875569279418 ) ) ;
#28335=AXIS2_PLACEMENT_3D ( 'NONE', #2410, #6279, #1423 ) ;
#28338=EDGE_CURVE ( 'NONE', #33571, #49500, #17805, .T. ) ;
#28340=EDGE_LOOP ( 'NONE', ( #10495, #26340 ) ) ;
#28345=EDGE_CURVE ( 'NONE', #40611, #24906, #47568, .T. ) ;
#28349=VERTEX_POINT ( 'NONE', #37340 ) ;
#28351=CARTESIAN_POINT ( 'NONE',  ( 73.30402655318508209, 1.750000000000010658, 80.81828755692798438 ) ) ;
#28356=VERTEX_POINT ( 'NONE', #18048 ) ;
#28362=EDGE_LOOP ( 'NONE', ( #15296, #1977, #28021, #14063, #39887, #10919 ) ) ;
#28363=( BOUNDED_CURVE ( )  B_SPLINE_CURVE ( 3, ( #40707, #36883, #8889, #24546 ),
 .UNSPECIFIED., .F., .F. ) 
 B_SPLINE_CURVE_WITH_KNOTS ( ( 4, 4 ),
 ( 4.712388980384689674, 6.283185307179586232 ),
 .UNSPECIFIED. ) 
 CURVE ( )  GEOMETRIC_REPRESENTATION_ITEM ( )  RATIONAL_B_SPLINE_CURVE ( ( 1.000000000000000000, 0.8047378541243649375, 0.8047378541243649375, 1.000000000000000000 ) ) 
 REPRESENTATION_ITEM ( '' )  );
#28366=DIRECTION ( 'NONE',  ( -1.000000000000000000, -0.000000000000000000, -0.000000000000000000 ) ) ;
#28367=ORIENTED_EDGE ( 'NONE', *, *, #5895, .T. ) ;
#28370=ORIENTED_EDGE ( 'NONE', *, *, #11567, .F. ) ;
#28374=EDGE_CURVE ( 'NONE', #7223, #22379, #31597, .T. ) ;
#28375=CIRCLE ( 'NONE', #44711, 1.749999999999987566 ) ;
#28376=DIRECTION ( 'NONE',  ( 1.000000000000000000, 0.000000000000000000, -0.000000000000000000 ) ) ;
#28377=CARTESIAN_POINT ( 'NONE',  ( -86.69597344681496054, 0.000000000000000000, 165.0000000000000000 ) ) ;
#28379=EDGE_CURVE ( 'NONE', #31866, #29044, #3699, .T. ) ;
#28380=VECTOR ( 'NONE', #6136, 1000.000000000000000 ) ;
#28381=LINE ( 'NONE', #9126, #46238 ) ;
#28386=DIRECTION ( 'NONE',  ( -1.000000000000000000, -0.000000000000000000, -0.000000000000000000 ) ) ;
#28388=CARTESIAN_POINT ( 'NONE',  ( 31.55402655318503236, 0.000000000000000000, 165.0000000000000000 ) ) ;
#28389=AXIS2_PLACEMENT_3D ( 'NONE', #47871, #13250, #24330 ) ;
#28392=CARTESIAN_POINT ( 'NONE',  ( -86.69597344681494633, 1.750000000000010658, 120.8182875569279702 ) ) ;
#28393=EDGE_CURVE ( 'NONE', #5041, #40908, #7603, .T. ) ;
#28396=ORIENTED_EDGE ( 'NONE', *, *, #39469, .T. ) ;
#28398=EDGE_CURVE ( 'NONE', #49373, #5769, #12840, .T. ) ;
#28400=CYLINDRICAL_SURFACE ( 'NONE', #18846, 1.750000000000015543 ) ;
#28406=FACE_OUTER_BOUND ( 'NONE', #9678, .T. ) ;
#28413=DIRECTION ( 'NONE',  ( -1.000000000000000000, -0.000000000000000000, -0.000000000000000000 ) ) ;
#28415=ORIENTED_EDGE ( 'NONE', *, *, #48672, .T. ) ;
#28417=EDGE_CURVE ( 'NONE', #49373, #43794, #3147, .T. ) ;
#28423=( BOUNDED_CURVE ( )  B_SPLINE_CURVE ( 3, ( #48956, #13845, #12854, #47964 ),
 .UNSPECIFIED., .F., .F. ) 
 B_SPLINE_CURVE_WITH_KNOTS ( ( 4, 4 ),
 ( 4.712388980384689674, 6.283185307179586232 ),
 .UNSPECIFIED. ) 
 CURVE ( )  GEOMETRIC_REPRESENTATION_ITEM ( )  RATIONAL_B_SPLINE_CURVE ( ( 1.000000000000000000, 0.8047378541243649375, 0.8047378541243649375, 1.000000000000000000 ) ) 
 REPRESENTATION_ITEM ( '' )  );
#28424=ORIENTED_EDGE ( 'NONE', *, *, #3400, .T. ) ;
#28427=EDGE_LOOP ( 'NONE', ( #145, #10179, #24176, #36255, #40396, #37362 ) ) ;
#28429=ORIENTED_EDGE ( 'NONE', *, *, #8906, .T. ) ;
#28432=( BOUNDED_CURVE ( )  B_SPLINE_CURVE ( 3, ( #46156, #11051, #22846, #38524 ),
 .UNSPECIFIED., .F., .F. ) 
 B_SPLINE_CURVE_WITH_KNOTS ( ( 4, 4 ),
 ( 3.141592653589793116, 4.712388980384689674 ),
 .UNSPECIFIED. ) 
 CURVE ( )  GEOMETRIC_REPRESENTATION_ITEM ( )  RATIONAL_B_SPLINE_CURVE ( ( 1.000000000000000000, 0.8047378541243649375, 0.8047378541243649375, 1.000000000000000000 ) ) 
 REPRESENTATION_ITEM ( '' )  );
#28436=CARTESIAN_POINT ( 'NONE',  ( 153.3040265531850537, 1.750000000000010214, 40.81828755692798438 ) ) ;
#28438=CYLINDRICAL_SURFACE ( 'NONE', #25606, 1.750000000000001554 ) ;
#28441=CARTESIAN_POINT ( 'NONE',  ( -167.7210997126620384, -1.750000000000009548, -158.1565861772249377 ) ) ;
#28445=CARTESIAN_POINT ( 'NONE',  ( -87.72109971266203843, 1.750000000000009548, -118.1565861772249519 ) ) ;
#28446=ADVANCED_FACE ( 'NONE', ( #22405 ), #7531, .T. ) ;
#28448=LINE ( 'NONE', #16633, #13773 ) ;
#28455=CARTESIAN_POINT ( 'NONE',  ( -128.4459734468149179, 0.000000000000000000, 165.0000000000000000 ) ) ;
#28457=CARTESIAN_POINT ( 'NONE',  ( 115.0540265531850395, 2.143131898507847836E-16, 159.0682875569279702 ) ) ;
#28460=ORIENTED_EDGE ( 'NONE', *, *, #9578, .T. ) ;
#28461=CYLINDRICAL_SURFACE ( 'NONE', #37932, 1.750000000000015543 ) ;
#28467=ORIENTED_EDGE ( 'NONE', *, *, #9208, .T. ) ;
#28470=VERTEX_POINT ( 'NONE', #30890 ) ;
#28473=CARTESIAN_POINT ( 'NONE',  ( 210.0000000000000568, 0.000000000000000000, 40.81828755692798438 ) ) ;
#28474=CARTESIAN_POINT ( 'NONE',  ( -168.4459734468149747, 0.000000000000000000, 162.5682875569279702 ) ) ;
#28478=DIRECTION ( 'NONE',  ( -1.000000000000000000, -0.000000000000000000, -0.000000000000000000 ) ) ;
#28481=DIRECTION ( 'NONE',  ( 0.000000000000000000, 0.000000000000000000, 1.000000000000000000 ) ) ;
#28482=EDGE_LOOP ( 'NONE', ( #5818, #18709 ) ) ;
#28484=CARTESIAN_POINT ( 'NONE',  ( 155.0540265531850537, -1.025126265847089213, -37.43171244307202272 ) ) ;
#28486=VERTEX_POINT ( 'NONE', #38590 ) ;
#28488=CARTESIAN_POINT ( 'NONE',  ( -48.44597344681496054, 1.025126265847089435, 39.06828755692797728 ) ) ;
#28490=CARTESIAN_POINT ( 'NONE',  ( -4.945973446814917018, -1.025126265847097207, -40.93171244307204404 ) ) ;
#28494=EDGE_CURVE ( 'NONE', #7807, #25713, #45628, .T. ) ;
#28495=EDGE_CURVE ( 'NONE', #16448, #26090, #35004, .T. ) ;
#28502=ORIENTED_EDGE ( 'NONE', *, *, #31661, .T. ) ;
#28505=EDGE_CURVE ( 'NONE', #47505, #41166, #18796, .T. ) ;
#28507=CARTESIAN_POINT ( 'NONE',  ( 192.2789002873380184, -1.750000000000010214, -120.2068387089191219 ) ) ;
#28508=DIRECTION ( 'NONE',  ( -0.000000000000000000, -0.000000000000000000, -1.000000000000000000 ) ) ;
#28511=EDGE_CURVE ( 'NONE', #25029, #47386, #122, .T. ) ;
#28516=CARTESIAN_POINT ( 'NONE',  ( 210.0000000000000568, 2.143131898507881856E-16, 119.0682875569279560 ) ) ;
#28523=CARTESIAN_POINT ( 'NONE',  ( 194.3291528190321742, -1.750000000000010436, -80.20683870891910772 ) ) ;
#28526=CARTESIAN_POINT ( 'NONE',  ( -124.9459734468149463, 2.143131898507847836E-16, -117.4317124430720725 ) ) ;
#28528=CARTESIAN_POINT ( 'NONE',  ( -8.445973446814964092, 1.025126265847097207, -77.43171244307197298 ) ) ;
#28530=CARTESIAN_POINT ( 'NONE',  ( -85.67084718096784002, 1.750000000000009548, -0.2068387089191121020 ) ) ;
#28540=CARTESIAN_POINT ( 'NONE',  ( -208.4459734468149463, 0.000000000000000000, -120.9317124430720156 ) ) ;
#28541=CARTESIAN_POINT ( 'NONE',  ( 193.3040265531851105, 1.750000000000009992, 160.8182875569279702 ) ) ;
#28543=CARTESIAN_POINT ( 'NONE',  ( 73.30402655318508209, 1.750000000000009992, -159.1817124430720298 ) ) ;
#28546=CARTESIAN_POINT ( 'NONE',  ( 210.0000000000000568, 0.000000000000000000, -159.1817124430720298 ) ) ;
#28549=VECTOR ( 'NONE', #32947, 1000.000000000000000 ) ;
#28550=VERTEX_POINT ( 'NONE', #8799 ) ;
#28555=VERTEX_POINT ( 'NONE', #23680 ) ;
#28559=( BOUNDED_CURVE ( )  B_SPLINE_CURVE ( 3, ( #25864, #41512, #37679, #15336 ),
 .UNSPECIFIED., .F., .F. ) 
 B_SPLINE_CURVE_WITH_KNOTS ( ( 4, 4 ),
 ( 1.570796326794896558, 3.141592653589793116 ),
 .UNSPECIFIED. ) 
 CURVE ( )  GEOMETRIC_REPRESENTATION_ITEM ( )  RATIONAL_B_SPLINE_CURVE ( ( 1.000000000000000000, 0.8047378541243649375, 0.8047378541243649375, 1.000000000000000000 ) ) 
 REPRESENTATION_ITEM ( '' )  );
#28560=DIRECTION ( 'NONE',  ( 0.000000000000000000, 0.000000000000000000, 1.000000000000000000 ) ) ;
#28561=CARTESIAN_POINT ( 'NONE',  ( -88.44597344681491791, 2.143131898507880377E-16, -160.9317124430720298 ) ) ;
#28563=CARTESIAN_POINT ( 'NONE',  ( -47.72109971266203132, 1.750000000000009548, 81.84341382277507648 ) ) ;
#28564=CYLINDRICAL_SURFACE ( 'NONE', #38088, 1.749999999999973799 ) ;
#28565=CARTESIAN_POINT ( 'NONE',  ( -127.7210997126620242, -1.749999999999996891, 79.79316129108087807 ) ) ;
#28566=ORIENTED_EDGE ( 'NONE', *, *, #46563, .F. ) ;
#28571=DIRECTION ( 'NONE',  ( 1.000000000000000000, 0.000000000000000000, 0.000000000000000000 ) ) ;
#28572=VERTEX_POINT ( 'NONE', #15985 ) ;
#28576=( BOUNDED_CURVE ( )  B_SPLINE_CURVE ( 3, ( #15149, #22333, #38010, #2826 ),
 .UNSPECIFIED., .F., .F. ) 
 B_SPLINE_CURVE_WITH_KNOTS ( ( 4, 4 ),
 ( 1.570796326794896558, 3.141592653589793116 ),
 .UNSPECIFIED. ) 
 CURVE ( )  GEOMETRIC_REPRESENTATION_ITEM ( )  RATIONAL_B_SPLINE_CURVE ( ( 1.000000000000000000, 0.8047378541243649375, 0.8047378541243649375, 1.000000000000000000 ) ) 
 REPRESENTATION_ITEM ( '' )  );
#28577=DIRECTION ( 'NONE',  ( 1.000000000000000000, 0.000000000000000000, 0.000000000000000000 ) ) ;
#28578=ORIENTED_EDGE ( 'NONE', *, *, #35773, .F. ) ;
#28581=AXIS2_PLACEMENT_3D ( 'NONE', #41063, #21821, #21057 ) ;
#28583=CARTESIAN_POINT ( 'NONE',  ( -206.6959734468149463, -1.750000000000010214, 40.81828755692798438 ) ) ;
#28585=EDGE_LOOP ( 'NONE', ( #3163, #50687, #39722, #38387, #5696 ) ) ;
#28596=CARTESIAN_POINT ( 'NONE',  ( 113.3040265531850537, -1.749999999999997335, -119.1817124430720440 ) ) ;
#28598=EDGE_LOOP ( 'NONE', ( #36612, #39570, #31015, #3575, #601, #4982 ) ) ;
#28602=EDGE_LOOP ( 'NONE', ( #31129, #40571, #49415, #40117, #46075, #5882 ) ) ;
#28606=ORIENTED_EDGE ( 'NONE', *, *, #37535, .T. ) ;
#28622=CARTESIAN_POINT ( 'NONE',  ( 113.3040265531850537, 0.000000000000000000, -165.0000000000000000 ) ) ;
#28625=EDGE_CURVE ( 'NONE', #34290, #48865, #33833, .T. ) ;
#28626=AXIS2_PLACEMENT_3D ( 'NONE', #1208, #29157, #13490 ) ;
#28629=DIRECTION ( 'NONE',  ( 1.000000000000000000, 0.000000000000000000, 0.000000000000000000 ) ) ;
#28630=EDGE_CURVE ( 'NONE', #50033, #38220, #4000, .T. ) ;
#28631=CARTESIAN_POINT ( 'NONE',  ( 73.30402655318508209, 0.000000000000000000, -165.0000000000000000 ) ) ;
#28638=CARTESIAN_POINT ( 'NONE',  ( 210.0000000000000568, 0.000000000000000000, 80.81828755692798438 ) ) ;
#28641=ORIENTED_EDGE ( 'NONE', *, *, #40242, .F. ) ;
#28643=EDGE_CURVE ( 'NONE', #9127, #2518, #40722, .T. ) ;
#28646=VECTOR ( 'NONE', #26635, 1000.000000000000000 ) ;
#28649=VECTOR ( 'NONE', #39764, 1000.000000000000000 ) ;
#28650=EDGE_CURVE ( 'NONE', #16704, #11488, #45920, .T. ) ;
#28655=CARTESIAN_POINT ( 'NONE',  ( 210.0000000000000568, 0.000000000000000000, -159.1817124430720298 ) ) ;
#28656=( BOUNDED_CURVE ( )  B_SPLINE_CURVE ( 3, ( #11118, #7265, #42399, #22912 ),
 .UNSPECIFIED., .F., .F. ) 
 B_SPLINE_CURVE_WITH_KNOTS ( ( 4, 4 ),
 ( 0.000000000000000000, 1.570796326794896780 ),
 .UNSPECIFIED. ) 
 CURVE ( )  GEOMETRIC_REPRESENTATION_ITEM ( )  RATIONAL_B_SPLINE_CURVE ( ( 1.000000000000000000, 0.8047378541243649375, 0.8047378541243649375, 1.000000000000000000 ) ) 
 REPRESENTATION_ITEM ( '' )  );
#28657=ORIENTED_EDGE ( 'NONE', *, *, #25545, .T. ) ;
#28662=ORIENTED_EDGE ( 'NONE', *, *, #14868, .F. ) ;
#28664=DIRECTION ( 'NONE',  ( -0.000000000000000000, -0.000000000000000000, -1.000000000000000000 ) ) ;
#28666=ORIENTED_EDGE ( 'NONE', *, *, #43268, .T. ) ;
#28670=ORIENTED_EDGE ( 'NONE', *, *, #49121, .T. ) ;
#28676=CARTESIAN_POINT ( 'NONE',  ( 75.05402655318508209, 0.000000000000000000, 162.5682875569279702 ) ) ;
#28681=EDGE_CURVE ( 'NONE', #29172, #16166, #415, .T. ) ;
#28682=DIRECTION ( 'NONE',  ( -0.000000000000000000, -0.000000000000000000, -1.000000000000000000 ) ) ;
#28686=LINE ( 'NONE', #13530, #22373 ) ;
#28690=DIRECTION ( 'NONE',  ( 1.000000000000000000, 0.000000000000000000, 0.000000000000000000 ) ) ;
#28694=CARTESIAN_POINT ( 'NONE',  ( 191.5540265531851105, 0.000000000000000000, 159.0682875569279702 ) ) ;
#28695=ORIENTED_EDGE ( 'NONE', *, *, #33122, .T. ) ;
#28701=CARTESIAN_POINT ( 'NONE',  ( -164.9459734468149463, 2.143131898507880377E-16, 159.0682875569279702 ) ) ;
#28702=EDGE_CURVE ( 'NONE', #2436, #11997, #5637, .T. ) ;
#28705=FACE_OUTER_BOUND ( 'NONE', #40679, .T. ) ;
#28706=CARTESIAN_POINT ( 'NONE',  ( -47.72109971266203132, 1.750000000000009548, -160.2068387089191219 ) ) ;
#28711=CARTESIAN_POINT ( 'NONE',  ( -47.72109971266203132, 1.750000000000009326, 1.843413822775066269 ) ) ;
#28714=ORIENTED_EDGE ( 'NONE', *, *, #9041, .F. ) ;
#28715=EDGE_LOOP ( 'NONE', ( #48715, #45222, #48757, #9548, #12508 ) ) ;
#28717=ADVANCED_FACE ( 'NONE', ( #21857 ), #21082, .T. ) ;
#28719=ORIENTED_EDGE ( 'NONE', *, *, #24034, .F. ) ;
#28721=CARTESIAN_POINT ( 'NONE',  ( -4.945973446814916130, -1.025126265847097429, -80.93171244307204404 ) ) ;
#28723=DIRECTION ( 'NONE',  ( -1.000000000000000000, -0.000000000000000000, -0.000000000000000000 ) ) ;
#28727=( BOUNDED_CURVE ( )  B_SPLINE_CURVE ( 3, ( #22330, #22587, #41586, #38270 ),
 .UNSPECIFIED., .F., .F. ) 
 B_SPLINE_CURVE_WITH_KNOTS ( ( 4, 4 ),
 ( 1.570796326794896558, 3.141592653589793116 ),
 .UNSPECIFIED. ) 
 CURVE ( )  GEOMETRIC_REPRESENTATION_ITEM ( )  RATIONAL_B_SPLINE_CURVE ( ( 1.000000000000000000, 0.8047378541243649375, 0.8047378541243649375, 1.000000000000000000 ) ) 
 REPRESENTATION_ITEM ( '' )  );
#28728=EDGE_CURVE ( 'NONE', #14882, #42480, #10892, .T. ) ;
#28731=EDGE_CURVE ( 'NONE', #3643, #19789, #29041, .T. ) ;
#28732=CARTESIAN_POINT ( 'NONE',  ( 191.5540265531851105, 0.000000000000000000, 42.56828755692798438 ) ) ;
#28733=AXIS2_PLACEMENT_3D ( 'NONE', #26995, #23411, #3647 ) ;
#28743=VECTOR ( 'NONE', #48714, 1000.000000000000000 ) ;
#28747=CARTESIAN_POINT ( 'NONE',  ( -208.4459734468149463, 0.000000000000000000, -157.4317124430720582 ) ) ;
#28748=EDGE_CURVE ( 'NONE', #28277, #24712, #12001, .T. ) ;
#28750=CARTESIAN_POINT ( 'NONE',  ( -44.94597344681493922, 1.025126265847089657, 119.0682875569279560 ) ) ;
#28751=CARTESIAN_POINT ( 'NONE',  ( -88.44597344681497475, 0.000000000000000000, -80.93171244307204404 ) ) ;
#28758=DIRECTION ( 'NONE',  ( 0.000000000000000000, 0.000000000000000000, 1.000000000000000000 ) ) ;
#28759=ORIENTED_EDGE ( 'NONE', *, *, #12214, .T. ) ;
#28763=CARTESIAN_POINT ( 'NONE',  ( -85.67084718096784002, 1.750000000000010214, 79.79316129108087807 ) ) ;
#28764=DIRECTION ( 'NONE',  ( -0.000000000000000000, -0.000000000000000000, -1.000000000000000000 ) ) ;
#28767=CARTESIAN_POINT ( 'NONE',  ( 210.0000000000000568, 0.000000000000000000, 42.56828755692799149 ) ) ;
#28778=EDGE_CURVE ( 'NONE', #21304, #1914, #35804, .T. ) ;
#28781=DIRECTION ( 'NONE',  ( -1.000000000000000000, 0.000000000000000000, 0.000000000000000000 ) ) ;
#28784=EDGE_CURVE ( 'NONE', #29991, #3878, #23014, .T. ) ;
#28797=FACE_OUTER_BOUND ( 'NONE', #39563, .T. ) ;
#28805=DIRECTION ( 'NONE',  ( -1.000000000000000000, -0.000000000000000000, -0.000000000000000000 ) ) ;
#28807=ORIENTED_EDGE ( 'NONE', *, *, #27525, .F. ) ;
#28808=VERTEX_POINT ( 'NONE', #50250 ) ;
#28815=ORIENTED_EDGE ( 'NONE', *, *, #16786, .T. ) ;
#28823=CARTESIAN_POINT ( 'NONE',  ( 210.0000000000000568, 0.000000000000000000, -119.1817124430720440 ) ) ;
#28828=ORIENTED_EDGE ( 'NONE', *, *, #45075, .F. ) ;
#28834=CARTESIAN_POINT ( 'NONE',  ( -44.94597344681493922, 2.143131898507880377E-16, -117.4317124430720156 ) ) ;
#28835=ORIENTED_EDGE ( 'NONE', *, *, #35539, .T. ) ;
#28843=ORIENTED_EDGE ( 'NONE', *, *, #44165, .F. ) ;
#28848=ORIENTED_EDGE ( 'NONE', *, *, #5933, .T. ) ;
#28854=ORIENTED_EDGE ( 'NONE', *, *, #42364, .F. ) ;
#28859=( BOUNDED_CURVE ( )  B_SPLINE_CURVE ( 3, ( #3546, #34884, #37295, #38234 ),
 .UNSPECIFIED., .F., .F. ) 
 B_SPLINE_CURVE_WITH_KNOTS ( ( 4, 4 ),
 ( 3.141592653589793116, 4.712388980384689674 ),
 .UNSPECIFIED. ) 
 CURVE ( )  GEOMETRIC_REPRESENTATION_ITEM ( )  RATIONAL_B_SPLINE_CURVE ( ( 1.000000000000000000, 0.8047378541243649375, 0.8047378541243649375, 1.000000000000000000 ) ) 
 REPRESENTATION_ITEM ( '' )  );
#28862=ORIENTED_EDGE ( 'NONE', *, *, #464, .T. ) ;
#28865=( BOUNDED_CURVE ( )  B_SPLINE_CURVE ( 3, ( #17829, #10132, #22194, #34509 ),
 .UNSPECIFIED., .F., .F. ) 
 B_SPLINE_CURVE_WITH_KNOTS ( ( 4, 4 ),
 ( 0.000000000000000000, 1.570796326794896558 ),
 .UNSPECIFIED. ) 
 CURVE ( )  GEOMETRIC_REPRESENTATION_ITEM ( )  RATIONAL_B_SPLINE_CURVE ( ( 1.000000000000000000, 0.8047378541243649375, 0.8047378541243649375, 1.000000000000000000 ) ) 
 REPRESENTATION_ITEM ( '' )  );
#28866=CARTESIAN_POINT ( 'NONE',  ( -8.445973446814976526, 0.000000000000000000, -77.43171244307198720 ) ) ;
#28869=EDGE_LOOP ( 'NONE', ( #9981, #22652, #19330, #9986, #47109, #31673 ) ) ;
#28880=ORIENTED_EDGE ( 'NONE', *, *, #39850, .T. ) ;
#28882=CARTESIAN_POINT ( 'NONE',  ( 35.05402655318504657, 2.143131898507880377E-16, -117.4317124430720156 ) ) ;
#28883=( BOUNDED_CURVE ( )  B_SPLINE_CURVE ( 3, ( #4933, #46543, #42229, #34811 ),
 .UNSPECIFIED., .F., .F. ) 
 B_SPLINE_CURVE_WITH_KNOTS ( ( 4, 4 ),
 ( 0.000000000000000000, 1.570796326794896558 ),
 .UNSPECIFIED. ) 
 CURVE ( )  GEOMETRIC_REPRESENTATION_ITEM ( )  RATIONAL_B_SPLINE_CURVE ( ( 1.000000000000000000, 0.8047378541243649375, 0.8047378541243649375, 1.000000000000000000 ) ) 
 REPRESENTATION_ITEM ( '' )  );
#28892=CARTESIAN_POINT ( 'NONE',  ( 191.5540265531851105, 0.000000000000000000, -80.93171244307201562 ) ) ;
#28893=ORIENTED_EDGE ( 'NONE', *, *, #29341, .F. ) ;
#28896=STYLED_ITEM('',(#50754),#5787);
#28899=CARTESIAN_POINT ( 'NONE',  ( 210.0000000000000568, 0.000000000000000000, 40.81828755692798438 ) ) ;
#28900=AXIS2_PLACEMENT_3D ( 'NONE', #43133, #8000, #31610 ) ;
#28906=DIRECTION ( 'NONE',  ( -0.000000000000000000, -0.000000000000000000, -1.000000000000000000 ) ) ;
#28910=CARTESIAN_POINT ( 'NONE',  ( 210.0000000000000568, 0.000000000000000000, -157.4317124430720298 ) ) ;
#28918=CARTESIAN_POINT ( 'NONE',  ( 115.0540265531850395, -1.025126265847081886, 79.06828755692797017 ) ) ;
#28922=ORIENTED_EDGE ( 'NONE', *, *, #30649, .T. ) ;
#28924=CARTESIAN_POINT ( 'NONE',  ( -204.9459734468148895, -1.025126265847089435, 122.5682875569280128 ) ) ;
#28928=CARTESIAN_POINT ( 'NONE',  ( 151.5540265531850537, 1.025126265847089213, 42.56828755692799149 ) ) ;
#28935=AXIS2_PLACEMENT_3D ( 'NONE', #19464, #39496, #16135 ) ;
#28937=CARTESIAN_POINT ( 'NONE',  ( -88.44597344681497475, 0.000000000000000000, -157.4317124430720014 ) ) ;
#28942=ADVANCED_FACE ( 'NONE', ( #38530 ), #32339, .T. ) ;
#28945=ORIENTED_EDGE ( 'NONE', *, *, #47434, .F. ) ;
#28952=( BOUNDED_CURVE ( )  B_SPLINE_CURVE ( 3, ( #4079, #32300, #31548, #12782 ),
 .UNSPECIFIED., .F., .F. ) 
 B_SPLINE_CURVE_WITH_KNOTS ( ( 4, 4 ),
 ( 0.000000000000000000, 1.570796326794896558 ),
 .UNSPECIFIED. ) 
 CURVE ( )  GEOMETRIC_REPRESENTATION_ITEM ( )  RATIONAL_B_SPLINE_CURVE ( ( 1.000000000000000000, 0.8047378541243649375, 0.8047378541243649375, 1.000000000000000000 ) ) 
 REPRESENTATION_ITEM ( '' )  );
#28954=CARTESIAN_POINT ( 'NONE',  ( -45.67084718096785423, -1.750000000000009548, -118.1565861772249519 ) ) ;
#28955=CARTESIAN_POINT ( 'NONE',  ( 151.5540265531850537, 0.000000000000000000, -120.9317124430720156 ) ) ;
#28961=EDGE_CURVE ( 'NONE', #38646, #20559, #28283, .T. ) ;
#28970=AXIS2_PLACEMENT_3D ( 'NONE', #25281, #28386, #44008 ) ;
#28971=CARTESIAN_POINT ( 'NONE',  ( 113.3040265531850537, 0.000000000000000000, 165.0000000000000000 ) ) ;
#28975=ADVANCED_FACE ( 'NONE', ( #4862 ), #8485, .T. ) ;
#28977=ORIENTED_EDGE ( 'NONE', *, *, #42773, .T. ) ;
#28979=FACE_OUTER_BOUND ( 'NONE', #26990, .T. ) ;
#28980=ORIENTED_EDGE ( 'NONE', *, *, #31140, .T. ) ;
#28986=ORIENTED_EDGE ( 'NONE', *, *, #25967, .F. ) ;
#28987=DIRECTION ( 'NONE',  ( -0.000000000000000000, -0.000000000000000000, -1.000000000000000000 ) ) ;
#28990=AXIS2_PLACEMENT_3D ( 'NONE', #43997, #48061, #32986 ) ;
#28992=LINE ( 'NONE', #44611, #8458 ) ;
#28995=EDGE_CURVE ( 'NONE', #47564, #27344, #3862, .T. ) ;
#28996=ORIENTED_EDGE ( 'NONE', *, *, #7999, .T. ) ;
#29000=DIRECTION ( 'NONE',  ( 0.000000000000000000, 0.000000000000000000, -1.000000000000000000 ) ) ;
#29003=EDGE_CURVE ( 'NONE', #13632, #37343, #26030, .T. ) ;
#29004=AXIS2_PLACEMENT_3D ( 'NONE', #3594, #30813, #34929 ) ;
#29007=CARTESIAN_POINT ( 'NONE',  ( -166.6959734468149463, 1.750000000000010658, -119.1817124430720440 ) ) ;
#29011=EDGE_CURVE ( 'NONE', #15143, #27194, #12077, .T. ) ;
#29016=( BOUNDED_CURVE ( )  B_SPLINE_CURVE ( 3, ( #35725, #24414, #20789, #36472 ),
 .UNSPECIFIED., .F., .F. ) 
 B_SPLINE_CURVE_WITH_KNOTS ( ( 4, 4 ),
 ( 4.712388980384689674, 6.283185307179586232 ),
 .UNSPECIFIED. ) 
 CURVE ( )  GEOMETRIC_REPRESENTATION_ITEM ( )  RATIONAL_B_SPLINE_CURVE ( ( 1.000000000000000000, 0.8047378541243649375, 0.8047378541243649375, 1.000000000000000000 ) ) 
 REPRESENTATION_ITEM ( '' )  );
#29019=EDGE_LOOP ( 'NONE', ( #29232, #5864, #28670, #26597, #26933, #32597 ) ) ;
#29022=CARTESIAN_POINT ( 'NONE',  ( 195.0540265531851105, -1.025126265847089657, -80.93171244307201562 ) ) ;
#29024=( BOUNDED_CURVE ( )  B_SPLINE_CURVE ( 3, ( #46412, #31320, #11299, #7460 ),
 .UNSPECIFIED., .F., .F. ) 
 B_SPLINE_CURVE_WITH_KNOTS ( ( 4, 4 ),
 ( 1.570796326794896558, 3.141592653589793116 ),
 .UNSPECIFIED. ) 
 CURVE ( )  GEOMETRIC_REPRESENTATION_ITEM ( )  RATIONAL_B_SPLINE_CURVE ( ( 1.000000000000000000, 0.8047378541243649375, 0.8047378541243649375, 1.000000000000000000 ) ) 
 REPRESENTATION_ITEM ( '' )  );
#29025=EDGE_CURVE ( 'NONE', #14767, #6739, #12235, .T. ) ;
#29027=AXIS2_PLACEMENT_3D ( 'NONE', #3549, #25462, #26910 ) ;
#29029=CARTESIAN_POINT ( 'NONE',  ( 210.0000000000000568, 0.000000000000000000, -119.1817124430720440 ) ) ;
#29030=EDGE_CURVE ( 'NONE', #4778, #16264, #44356, .T. ) ;
#29038=ORIENTED_EDGE ( 'NONE', *, *, #24678, .F. ) ;
#29041=LINE ( 'NONE', #17492, #32493 ) ;
#29044=VERTEX_POINT ( 'NONE', #41280 ) ;
#29049=ORIENTED_EDGE ( 'NONE', *, *, #21139, .F. ) ;
#29052=CYLINDRICAL_SURFACE ( 'NONE', #17710, 1.750000000000015543 ) ;
#29054=CARTESIAN_POINT ( 'NONE',  ( -86.69597344681496054, 0.000000000000000000, 165.0000000000000000 ) ) ;
#29055=VERTEX_POINT ( 'NONE', #21276 ) ;
#29062=CARTESIAN_POINT ( 'NONE',  ( 71.55402655318505367, -1.025126265847089435, 2.568287556927986159 ) ) ;
#29065=EDGE_LOOP ( 'NONE', ( #14643, #40273, #6063, #29812, #14115, #20255 ) ) ;
#29067=LINE ( 'NONE', #44691, #22788 ) ;
#29072=CYLINDRICAL_SURFACE ( 'NONE', #47931, 1.750000000000015543 ) ;
#29073=CARTESIAN_POINT ( 'NONE',  ( -44.94597344681493922, -1.025126265847089657, 119.0682875569279560 ) ) ;
#29074=AXIS2_PLACEMENT_3D ( 'NONE', #14104, #41567, #37739 ) ;
#29077=CARTESIAN_POINT ( 'NONE',  ( 195.0540265531851105, 2.143131898507880377E-16, -40.93171244307202983 ) ) ;
#29078=EDGE_CURVE ( 'NONE', #48234, #38333, #16941, .T. ) ;
#29082=EDGE_CURVE ( 'NONE', #9162, #16655, #2280, .T. ) ;
#29084=ORIENTED_EDGE ( 'NONE', *, *, #49281, .F. ) ;
#29085=AXIS2_PLACEMENT_3D ( 'NONE', #7404, #38461, #42288 ) ;
#29087=ORIENTED_EDGE ( 'NONE', *, *, #35637, .T. ) ;
#29088=CARTESIAN_POINT ( 'NONE',  ( -46.69597344681494633, 1.750000000000010658, 80.81828755692798438 ) ) ;
#29089=DIRECTION ( 'NONE',  ( -1.000000000000000000, -0.000000000000000000, -0.000000000000000000 ) ) ;
#29097=DIRECTION ( 'NONE',  ( 0.000000000000000000, 0.000000000000000000, 1.000000000000000000 ) ) ;
#29098=CARTESIAN_POINT ( 'NONE',  ( -84.94597344681494633, 2.143131898507880377E-16, 82.56828755692798438 ) ) ;
#29102=CARTESIAN_POINT ( 'NONE',  ( -126.6959734468149321, 1.749999999999997113, -39.18171244307202983 ) ) ;
#29104=ORIENTED_EDGE ( 'NONE', *, *, #16314, .F. ) ;
#29108=CARTESIAN_POINT ( 'NONE',  ( 111.5540265531850679, 0.000000000000000000, 82.56828755692797017 ) ) ;
#29110=ORIENTED_EDGE ( 'NONE', *, *, #1159, .T. ) ;
#29113=ORIENTED_EDGE ( 'NONE', *, *, #22242, .F. ) ;
#29115=CARTESIAN_POINT ( 'NONE',  ( -8.445973446814976526, 0.000000000000000000, -40.93171244307205825 ) ) ;
#29116=CARTESIAN_POINT ( 'NONE',  ( 194.3291528190321742, 1.750000000000010214, 119.7931612910808781 ) ) ;
#29122=DIRECTION ( 'NONE',  ( 0.000000000000000000, 0.000000000000000000, 1.000000000000000000 ) ) ;
#29127=CARTESIAN_POINT ( 'NONE',  ( -46.69597344681494633, 0.000000000000000000, 165.0000000000000000 ) ) ;
#29128=ORIENTED_EDGE ( 'NONE', *, *, #15632, .T. ) ;
#29129=CARTESIAN_POINT ( 'NONE',  ( 151.5540265531850537, -1.025126265847089879, 122.5682875569280128 ) ) ;
#29135=CYLINDRICAL_SURFACE ( 'NONE', #6938, 1.750000000000001554 ) ;
#29138=CYLINDRICAL_SURFACE ( 'NONE', #2737, 1.750000000000015543 ) ;
#29140=CARTESIAN_POINT ( 'NONE',  ( -46.69597344681494633, 0.000000000000000000, 165.0000000000000000 ) ) ;
#29141=CARTESIAN_POINT ( 'NONE',  ( 31.55402655318503236, 0.000000000000000000, -40.93171244307205825 ) ) ;
#29143=EDGE_CURVE ( 'NONE', #18308, #11343, #46965, .T. ) ;
#29145=AXIS2_PLACEMENT_3D ( 'NONE', #34041, #17861, #18359 ) ;
#29151=EDGE_LOOP ( 'NONE', ( #43455, #43999, #39918, #44834, #49559 ) ) ;
#29152=CARTESIAN_POINT ( 'NONE',  ( -48.44597344681496054, 1.025126265847089435, 122.5682875569280128 ) ) ;
#29153=VECTOR ( 'NONE', #2777, 1000.000000000000000 ) ;
#29157=DIRECTION ( 'NONE',  ( -0.000000000000000000, -0.000000000000000000, -1.000000000000000000 ) ) ;
#29162=VERTEX_POINT ( 'NONE', #26649 ) ;
#29165=AXIS2_PLACEMENT_3D ( 'NONE', #11675, #7578, #23213 ) ;
#29166=CARTESIAN_POINT ( 'NONE',  ( 75.05402655318509630, 2.143131898507880377E-16, -157.4317124430720014 ) ) ;
#29167=( BOUNDED_CURVE ( )  B_SPLINE_CURVE ( 3, ( #24965, #5447, #21350, #13149 ),
 .UNSPECIFIED., .F., .F. ) 
 B_SPLINE_CURVE_WITH_KNOTS ( ( 4, 4 ),
 ( 1.570796326794896558, 3.141592653589793116 ),
 .UNSPECIFIED. ) 
 CURVE ( )  GEOMETRIC_REPRESENTATION_ITEM ( )  RATIONAL_B_SPLINE_CURVE ( ( 1.000000000000000000, 0.8047378541243649375, 0.8047378541243649375, 1.000000000000000000 ) ) 
 REPRESENTATION_ITEM ( '' )  );
#29170=DIRECTION ( 'NONE',  ( -0.000000000000000000, -0.000000000000000000, -1.000000000000000000 ) ) ;
#29171=EDGE_LOOP ( 'NONE', ( #2427, #23702, #19209, #27595, #17697 ) ) ;
#29172=VERTEX_POINT ( 'NONE', #23037 ) ;
#29174=( BOUNDED_CURVE ( )  B_SPLINE_CURVE ( 3, ( #35531, #14998, #15752, #22689 ),
 .UNSPECIFIED., .F., .F. ) 
 B_SPLINE_CURVE_WITH_KNOTS ( ( 4, 4 ),
 ( 4.712388980384689674, 6.283185307179586232 ),
 .UNSPECIFIED. ) 
 CURVE ( )  GEOMETRIC_REPRESENTATION_ITEM ( )  RATIONAL_B_SPLINE_CURVE ( ( 1.000000000000000000, 0.8047378541243649375, 0.8047378541243649375, 1.000000000000000000 ) ) 
 REPRESENTATION_ITEM ( '' )  );
#29176=CARTESIAN_POINT ( 'NONE',  ( 35.05402655318504657, 2.143131898507880377E-16, 119.0682875569279702 ) ) ;
#29177=CARTESIAN_POINT ( 'NONE',  ( -206.6959734468149463, 1.750000000000010658, -119.1817124430720440 ) ) ;
#29182=FACE_OUTER_BOUND ( 'NONE', #31452, .T. ) ;
#29184=ORIENTED_EDGE ( 'NONE', *, *, #719, .F. ) ;
#29188=( BOUNDED_CURVE ( )  B_SPLINE_CURVE ( 3, ( #29438, #47887, #32551, #12780 ),
 .UNSPECIFIED., .F., .F. ) 
 B_SPLINE_CURVE_WITH_KNOTS ( ( 4, 4 ),
 ( 0.000000000000000000, 1.570796326794896558 ),
 .UNSPECIFIED. ) 
 CURVE ( )  GEOMETRIC_REPRESENTATION_ITEM ( )  RATIONAL_B_SPLINE_CURVE ( ( 1.000000000000000000, 0.8047378541243649375, 0.8047378541243649375, 1.000000000000000000 ) ) 
 REPRESENTATION_ITEM ( '' )  );
#29191=DIRECTION ( 'NONE',  ( -1.000000000000000000, -0.000000000000000000, -0.000000000000000000 ) ) ;
#29195=CARTESIAN_POINT ( 'NONE',  ( 71.55402655318505367, 0.000000000000000000, 42.56828755692799859 ) ) ;
#29198=CARTESIAN_POINT ( 'NONE',  ( -46.69597344681494633, -1.750000000000009992, 160.8182875569279702 ) ) ;
#29200=DIRECTION ( 'NONE',  ( -1.000000000000000000, 0.000000000000000000, 0.000000000000000000 ) ) ;
#29205=ORIENTED_EDGE ( 'NONE', *, *, #12961, .T. ) ;
#29206=EDGE_CURVE ( 'NONE', #34290, #20654, #33240, .T. ) ;
#29208=CARTESIAN_POINT ( 'NONE',  ( -168.4459734468149747, -1.025126265847089435, 2.568287556927986159 ) ) ;
#29214=ORIENTED_EDGE ( 'NONE', *, *, #12073, .T. ) ;
#29215=CARTESIAN_POINT ( 'NONE',  ( -165.6708471809677974, 1.750000000000010214, 79.79316129108087807 ) ) ;
#29217=DIRECTION ( 'NONE',  ( -0.000000000000000000, -0.000000000000000000, -1.000000000000000000 ) ) ;
#29223=VECTOR ( 'NONE', #31599, 1000.000000000000000 ) ;
#29226=CARTESIAN_POINT ( 'NONE',  ( 210.0000000000000568, 0.000000000000000000, -37.43171244307202272 ) ) ;
#29230=DIRECTION ( 'NONE',  ( -1.000000000000000000, -0.000000000000000000, -0.000000000000000000 ) ) ;
#29232=ORIENTED_EDGE ( 'NONE', *, *, #37169, .F. ) ;
#29234=CARTESIAN_POINT ( 'NONE',  ( -46.69597344681494633, -1.750000000000010658, -119.1817124430720440 ) ) ;
#29238=ORIENTED_EDGE ( 'NONE', *, *, #11766, .F. ) ;
#29245=CARTESIAN_POINT ( 'NONE',  ( 210.0000000000000568, 0.000000000000000000, 120.8182875569279702 ) ) ;
#29248=ORIENTED_EDGE ( 'NONE', *, *, #24569, .T. ) ;
#29250=DIRECTION ( 'NONE',  ( -0.000000000000000000, -0.000000000000000000, -1.000000000000000000 ) ) ;
#29252=ORIENTED_EDGE ( 'NONE', *, *, #14563, .F. ) ;
#29254=CARTESIAN_POINT ( 'NONE',  ( 115.0540265531850395, 1.025126265847082108, -117.4317124430720440 ) ) ;
#29256=( BOUNDED_CURVE ( )  B_SPLINE_CURVE ( 3, ( #13083, #5632, #5384, #28747 ),
 .UNSPECIFIED., .F., .F. ) 
 B_SPLINE_CURVE_WITH_KNOTS ( ( 4, 4 ),
 ( 1.570796326794896558, 3.141592653589793116 ),
 .UNSPECIFIED. ) 
 CURVE ( )  GEOMETRIC_REPRESENTATION_ITEM ( )  RATIONAL_B_SPLINE_CURVE ( ( 1.000000000000000000, 0.8047378541243649375, 0.8047378541243649375, 1.000000000000000000 ) ) 
 REPRESENTATION_ITEM ( '' )  );
#29261=ADVANCED_FACE ( 'NONE', ( #26894 ), #29999, .T. ) ;
#29262=CYLINDRICAL_SURFACE ( 'NONE', #26169, 1.750000000000008438 ) ;
#29265=EDGE_CURVE ( 'NONE', #13085, #12365, #34890, .T. ) ;
#29268=VERTEX_POINT ( 'NONE', #15097 ) ;
#29269=ORIENTED_EDGE ( 'NONE', *, *, #18350, .T. ) ;
#29272=ORIENTED_EDGE ( 'NONE', *, *, #29082, .T. ) ;
#29273=CARTESIAN_POINT ( 'NONE',  ( -166.6959734468149463, 0.000000000000000000, 165.0000000000000000 ) ) ;
#29275=EDGE_CURVE ( 'NONE', #16751, #21151, #50243, .T. ) ;
#29277=CARTESIAN_POINT ( 'NONE',  ( -5.670847180967843570, 1.750000000000023537, -80.20683870891910772 ) ) ;
#29280=CARTESIAN_POINT ( 'NONE',  ( -84.94597344681494633, 2.143131898507880377E-16, -0.9317124430720247208 ) ) ;
#29285=FACE_OUTER_BOUND ( 'NONE', #28063, .T. ) ;
#29292=EDGE_CURVE ( 'NONE', #38442, #48485, #22287, .T. ) ;
#29296=CARTESIAN_POINT ( 'NONE',  ( 191.5540265531850537, 1.025126265847088991, -157.4317124430720582 ) ) ;
#29298=ORIENTED_EDGE ( 'NONE', *, *, #15626, .F. ) ;
#29301=ADVANCED_FACE ( 'NONE', ( #8423 ), #472, .T. ) ;
#29312=DIRECTION ( 'NONE',  ( -0.000000000000000000, -0.000000000000000000, -1.000000000000000000 ) ) ;
#29313=CARTESIAN_POINT ( 'NONE',  ( 210.0000000000000568, 0.000000000000000000, 80.81828755692798438 ) ) ;
#29314=VERTEX_POINT ( 'NONE', #42781 ) ;
#29315=ADVANCED_FACE ( 'NONE', ( #32028 ), #43297, .T. ) ;
#29316=CARTESIAN_POINT ( 'NONE',  ( 111.5540265531850537, 1.025126265847081664, 42.56828755692797017 ) ) ;
#29317=VERTEX_POINT ( 'NONE', #47363 ) ;
#29320=CARTESIAN_POINT ( 'NONE',  ( 210.0000000000000568, 0.000000000000000000, 120.8182875569279702 ) ) ;
#29321=CARTESIAN_POINT ( 'NONE',  ( -6.695973446814940111, -1.750000000000024203, 120.8182875569279702 ) ) ;
#29324=ADVANCED_FACE ( 'NONE', ( #16115 ), #31016, .T. ) ;
#29330=( BOUNDED_CURVE ( )  B_SPLINE_CURVE ( 3, ( #29633, #45255, #2441, #25537 ),
 .UNSPECIFIED., .F., .F. ) 
 B_SPLINE_CURVE_WITH_KNOTS ( ( 4, 4 ),
 ( 3.141592653589793116, 4.712388980384689674 ),
 .UNSPECIFIED. ) 
 CURVE ( )  GEOMETRIC_REPRESENTATION_ITEM ( )  RATIONAL_B_SPLINE_CURVE ( ( 1.000000000000000000, 0.8047378541243649375, 0.8047378541243649375, 1.000000000000000000 ) ) 
 REPRESENTATION_ITEM ( '' )  );
#29337=VERTEX_POINT ( 'NONE', #35883 ) ;
#29341=EDGE_CURVE ( 'NONE', #29584, #45429, #8677, .T. ) ;
#29346=ADVANCED_FACE ( 'NONE', ( #27919 ), #11504, .T. ) ;
#29348=CARTESIAN_POINT ( 'NONE',  ( 155.0540265531850537, 0.000000000000000000, 162.5682875569279702 ) ) ;
#29351=DIRECTION ( 'NONE',  ( -0.000000000000000000, -0.000000000000000000, -1.000000000000000000 ) ) ;
#29357=ORIENTED_EDGE ( 'NONE', *, *, #11890, .T. ) ;
#29359=CYLINDRICAL_SURFACE ( 'NONE', #33998, 1.750000000000015543 ) ;
#29363=ADVANCED_FACE ( 'NONE', ( #31526 ), #47111, .T. ) ;
#29364=ADVANCED_FACE ( 'NONE', ( #8915 ), #33293, .F. ) ;
#29366=VERTEX_POINT ( 'NONE', #13510 ) ;
#29368=DIRECTION ( 'NONE',  ( -1.000000000000000000, -0.000000000000000000, -0.000000000000000000 ) ) ;
#29371=EDGE_LOOP ( 'NONE', ( #38845, #22238, #2402, #17807, #10024, #36719 ) ) ;
#29377=CARTESIAN_POINT ( 'NONE',  ( 210.0000000000000568, 0.000000000000000000, -39.18171244307202983 ) ) ;
#29380=CARTESIAN_POINT ( 'NONE',  ( 71.55402655318505367, 0.000000000000000000, -77.43171244307198720 ) ) ;
#29382=CARTESIAN_POINT ( 'NONE',  ( 113.3040265531850537, -1.749999999999997335, 80.81828755692798438 ) ) ;
#29384=CARTESIAN_POINT ( 'NONE',  ( -166.6959734468149463, -1.750000000000010658, 120.8182875569279702 ) ) ;
#29390=CARTESIAN_POINT ( 'NONE',  ( -86.69597344681496054, 0.000000000000000000, 165.0000000000000000 ) ) ;
#29395=( BOUNDED_CURVE ( )  B_SPLINE_CURVE ( 3, ( #20230, #35900, #730, #5770 ),
 .UNSPECIFIED., .F., .F. ) 
 B_SPLINE_CURVE_WITH_KNOTS ( ( 4, 4 ),
 ( 0.000000000000000000, 1.570796326794896558 ),
 .UNSPECIFIED. ) 
 CURVE ( )  GEOMETRIC_REPRESENTATION_ITEM ( )  RATIONAL_B_SPLINE_CURVE ( ( 1.000000000000000000, 0.8047378541243649375, 0.8047378541243649375, 1.000000000000000000 ) ) 
 REPRESENTATION_ITEM ( '' )  );
#29396=CYLINDRICAL_SURFACE ( 'NONE', #28626, 1.750000000000001554 ) ;
#29407=ORIENTED_EDGE ( 'NONE', *, *, #33487, .T. ) ;
#29410=ORIENTED_EDGE ( 'NONE', *, *, #48474, .F. ) ;
#29423=DIRECTION ( 'NONE',  ( -0.000000000000000000, -0.000000000000000000, -1.000000000000000000 ) ) ;
#29425=ORIENTED_EDGE ( 'NONE', *, *, #13113, .T. ) ;
#29426=CARTESIAN_POINT ( 'NONE',  ( 112.2789002873379758, -1.749999999999996669, -40.20683870891911482 ) ) ;
#29432=ORIENTED_EDGE ( 'NONE', *, *, #16419, .F. ) ;
#29434=FACE_OUTER_BOUND ( 'NONE', #41144, .T. ) ;
#29438=CARTESIAN_POINT ( 'NONE',  ( -88.44597344681497475, 0.000000000000000000, 79.06828755692795596 ) ) ;
#29443=CARTESIAN_POINT ( 'NONE',  ( 210.0000000000000568, 2.143131898507884075E-16, 39.06828755692797728 ) ) ;
#29453=( BOUNDED_CURVE ( )  B_SPLINE_CURVE ( 3, ( #394, #20379, #47545, #42962 ),
 .UNSPECIFIED., .F., .F. ) 
 B_SPLINE_CURVE_WITH_KNOTS ( ( 4, 4 ),
 ( 1.570796326794896558, 3.141592653589793116 ),
 .UNSPECIFIED. ) 
 CURVE ( )  GEOMETRIC_REPRESENTATION_ITEM ( )  RATIONAL_B_SPLINE_CURVE ( ( 1.000000000000000000, 0.8047378541243649375, 0.8047378541243649375, 1.000000000000000000 ) ) 
 REPRESENTATION_ITEM ( '' )  );
#29457=CARTESIAN_POINT ( 'NONE',  ( -48.44597344681496054, 1.025126265847089213, 162.5682875569279133 ) ) ;
#29460=CARTESIAN_POINT ( 'NONE',  ( -6.695973446814940111, -1.750000000000024203, 120.8182875569279702 ) ) ;
#29462=AXIS2_PLACEMENT_3D ( 'NONE', #14874, #18957, #30523 ) ;
#29464=( BOUNDED_CURVE ( )  B_SPLINE_CURVE ( 3, ( #46056, #41235, #26355, #6345 ),
 .UNSPECIFIED., .F., .F. ) 
 B_SPLINE_CURVE_WITH_KNOTS ( ( 4, 4 ),
 ( 3.141592653589793116, 4.712388980384689674 ),
 .UNSPECIFIED. ) 
 CURVE ( )  GEOMETRIC_REPRESENTATION_ITEM ( )  RATIONAL_B_SPLINE_CURVE ( ( 1.000000000000000000, 0.8047378541243649375, 0.8047378541243649375, 1.000000000000000000 ) ) 
 REPRESENTATION_ITEM ( '' )  );
#29465=ORIENTED_EDGE ( 'NONE', *, *, #40839, .F. ) ;
#29466=CARTESIAN_POINT ( 'NONE',  ( 71.55402655318505367, 0.000000000000000000, -80.93171244307204404 ) ) ;
#29468=ORIENTED_EDGE ( 'NONE', *, *, #29695, .F. ) ;
#29471=ORIENTED_EDGE ( 'NONE', *, *, #48337, .F. ) ;
#29472=CARTESIAN_POINT ( 'NONE',  ( -166.6959734468149463, 1.750000000000010214, 40.81828755692798438 ) ) ;
#29473=CARTESIAN_POINT ( 'NONE',  ( -167.7210997126620384, 1.750000000000009548, 161.8434138227750907 ) ) ;
#29477=( BOUNDED_CURVE ( )  B_SPLINE_CURVE ( 3, ( #36843, #21160, #1672, #17312 ),
 .UNSPECIFIED., .F., .F. ) 
 B_SPLINE_CURVE_WITH_KNOTS ( ( 4, 4 ),
 ( 4.712388980384689674, 6.283185307179586232 ),
 .UNSPECIFIED. ) 
 CURVE ( )  GEOMETRIC_REPRESENTATION_ITEM ( )  RATIONAL_B_SPLINE_CURVE ( ( 1.000000000000000000, 0.8047378541243649375, 0.8047378541243649375, 1.000000000000000000 ) ) 
 REPRESENTATION_ITEM ( '' )  );
#29479=ORIENTED_EDGE ( 'NONE', *, *, #22385, .F. ) ;
#29485=CARTESIAN_POINT ( 'NONE',  ( 210.0000000000000568, 0.000000000000000000, 80.81828755692798438 ) ) ;
#29489=CARTESIAN_POINT ( 'NONE',  ( -4.945973446814917018, 1.025126265847097207, -157.4317124430720014 ) ) ;
#29496=CARTESIAN_POINT ( 'NONE',  ( -6.695973446814940111, 0.000000000000000000, 165.0000000000000000 ) ) ;
#29497=DIRECTION ( 'NONE',  ( 0.000000000000000000, 0.000000000000000000, 1.000000000000000000 ) ) ;
#29498=VECTOR ( 'NONE', #41130, 1000.000000000000000 ) ;
#29500=VERTEX_POINT ( 'NONE', #5313 ) ;
#29508=CARTESIAN_POINT ( 'NONE',  ( -124.9459734468149321, 1.025126265847081886, 119.0682875569279702 ) ) ;
#29510=DIRECTION ( 'NONE',  ( 0.000000000000000000, 0.000000000000000000, 1.000000000000000000 ) ) ;
#29517=EDGE_CURVE ( 'NONE', #42480, #50107, #18809, .T. ) ;
#29518=ORIENTED_EDGE ( 'NONE', *, *, #7184, .F. ) ;
#29520=ORIENTED_EDGE ( 'NONE', *, *, #26189, .T. ) ;
#29523=CARTESIAN_POINT ( 'NONE',  ( 111.5540265531850537, 0.000000000000000000, 162.5682875569279702 ) ) ;
#29526=ORIENTED_EDGE ( 'NONE', *, *, #25437, .F. ) ;
#29528=CARTESIAN_POINT ( 'NONE',  ( -204.9459734468149463, 2.143131898507880377E-16, 165.0000000000000000 ) ) ;
#29529=ORIENTED_EDGE ( 'NONE', *, *, #43963, .T. ) ;
#29531=CARTESIAN_POINT ( 'NONE',  ( 210.0000000000000568, 0.000000000000000000, 162.5682875569279702 ) ) ;
#29532=CARTESIAN_POINT ( 'NONE',  ( 73.30402655318508209, -1.750000000000009992, 160.8182875569279702 ) ) ;
#29539=ORIENTED_EDGE ( 'NONE', *, *, #18897, .F. ) ;
#29540=CARTESIAN_POINT ( 'NONE',  ( 210.0000000000000568, 0.000000000000000000, -79.18171244307201562 ) ) ;
#29541=CARTESIAN_POINT ( 'NONE',  ( -126.6959734468149321, -1.749999999999997335, 120.8182875569279702 ) ) ;
#29549=LINE ( 'NONE', #29807, #34140 ) ;
#29550=CARTESIAN_POINT ( 'NONE',  ( 31.55402655318503236, 0.000000000000000000, -117.4317124430720156 ) ) ;
#29551=FACE_OUTER_BOUND ( 'NONE', #38194, .T. ) ;
#29554=CARTESIAN_POINT ( 'NONE',  ( 151.5540265531850537, 1.025126265847089213, -37.43171244307202272 ) ) ;
#29561=VECTOR ( 'NONE', #42277, 1000.000000000000000 ) ;
#29565=CARTESIAN_POINT ( 'NONE',  ( -125.6708471809678542, -1.749999999999996225, 159.7931612910809065 ) ) ;
#29569=CARTESIAN_POINT ( 'NONE',  ( -46.69597344681494633, 0.000000000000000000, 165.0000000000000000 ) ) ;
#29571=CARTESIAN_POINT ( 'NONE',  ( -44.94597344681493922, 1.025126265847089657, -120.9317124430720440 ) ) ;
#29572=VERTEX_POINT ( 'NONE', #33533 ) ;
#29574=LINE ( 'NONE', #1631, #28549 ) ;
#29579=ADVANCED_FACE ( 'NONE', ( #14781 ), #26076, .T. ) ;
#29580=EDGE_CURVE ( 'NONE', #15732, #30427, #41977, .T. ) ;
#29583=DIRECTION ( 'NONE',  ( 0.000000000000000000, 0.000000000000000000, 1.000000000000000000 ) ) ;
#29584=VERTEX_POINT ( 'NONE', #42231 ) ;
#29589=ORIENTED_EDGE ( 'NONE', *, *, #3434, .T. ) ;
#29591=CYLINDRICAL_SURFACE ( 'NONE', #18831, 1.750000000000008438 ) ;
#29600=VERTEX_POINT ( 'NONE', #14010 ) ;
#29601=EDGE_CURVE ( 'NONE', #40803, #10095, #15538, .T. ) ;
#29605=DIRECTION ( 'NONE',  ( -0.000000000000000000, -0.000000000000000000, -1.000000000000000000 ) ) ;
#29607=ORIENTED_EDGE ( 'NONE', *, *, #6752, .T. ) ;
#29608=CARTESIAN_POINT ( 'NONE',  ( 73.30402655318508209, 1.750000000000010658, 80.81828755692798438 ) ) ;
#29610=VERTEX_POINT ( 'NONE', #6331 ) ;
#29611=AXIS2_PLACEMENT_3D ( 'NONE', #15568, #11222, #3764 ) ;
#29612=CIRCLE ( 'NONE', #18136, 1.750000000000015543 ) ;
#29613=ADVANCED_FACE ( 'NONE', ( #37647 ), #14522, .T. ) ;
#29614=CYLINDRICAL_SURFACE ( 'NONE', #28335, 1.750000000000008438 ) ;
#29617=ORIENTED_EDGE ( 'NONE', *, *, #41058, .T. ) ;
#29618=CARTESIAN_POINT ( 'NONE',  ( -4.945973446814903696, 2.143131898507912917E-16, 159.0682875569279418 ) ) ;
#29619=( BOUNDED_CURVE ( )  B_SPLINE_CURVE ( 3, ( #29833, #18261, #22130, #21117 ),
 .UNSPECIFIED., .F., .F. ) 
 B_SPLINE_CURVE_WITH_KNOTS ( ( 4, 4 ),
 ( 4.712388980384689674, 6.283185307179586232 ),
 .UNSPECIFIED. ) 
 CURVE ( )  GEOMETRIC_REPRESENTATION_ITEM ( )  RATIONAL_B_SPLINE_CURVE ( ( 1.000000000000000000, 0.8047378541243649375, 0.8047378541243649375, 1.000000000000000000 ) ) 
 REPRESENTATION_ITEM ( '' )  );
#29622=VERTEX_POINT ( 'NONE', #18118 ) ;
#29632=DIRECTION ( 'NONE',  ( -1.000000000000000000, -0.000000000000000000, -0.000000000000000000 ) ) ;
#29633=CARTESIAN_POINT ( 'NONE',  ( 71.55402655318505367, 0.000000000000000000, -117.4317124430720156 ) ) ;
#29640=VECTOR ( 'NONE', #12411, 1000.000000000000000 ) ;
#29643=DIRECTION ( 'NONE',  ( -1.000000000000000000, 0.000000000000000000, 0.000000000000000000 ) ) ;
#29655=CARTESIAN_POINT ( 'NONE',  ( 75.05402655318509630, 1.025126265847089657, 42.56828755692799149 ) ) ;
#29657=ORIENTED_EDGE ( 'NONE', *, *, #49872, .T. ) ;
#29660=CARTESIAN_POINT ( 'NONE',  ( 153.3040265531850537, 0.000000000000000000, 165.0000000000000000 ) ) ;
#29667=CARTESIAN_POINT ( 'NONE',  ( 75.05402655318509630, -1.025126265847089657, 119.0682875569279560 ) ) ;
#29669=CARTESIAN_POINT ( 'NONE',  ( 35.05402655318504657, 2.143131898507880377E-16, 165.0000000000000000 ) ) ;
#29672=VECTOR ( 'NONE', #7977, 1000.000000000000000 ) ;
#29680=DIRECTION ( 'NONE',  ( -0.000000000000000000, -0.000000000000000000, -1.000000000000000000 ) ) ;
#29682=CARTESIAN_POINT ( 'NONE',  ( -206.6959734468149463, -1.750000000000010658, -119.1817124430720440 ) ) ;
#29685=CARTESIAN_POINT ( 'NONE',  ( -44.94597344681493922, 2.143131898507880377E-16, -160.9317124430720582 ) ) ;
#29691=DIRECTION ( 'NONE',  ( -1.000000000000000000, -0.000000000000000000, -0.000000000000000000 ) ) ;
#29693=CARTESIAN_POINT ( 'NONE',  ( 193.3040265531851105, 1.750000000000010658, 80.81828755692798438 ) ) ;
#29695=EDGE_CURVE ( 'NONE', #25164, #41719, #33401, .T. ) ;
#29696=( BOUNDED_CURVE ( )  B_SPLINE_CURVE ( 3, ( #18312, #33992, #2184, #49579 ),
 .UNSPECIFIED., .F., .F. ) 
 B_SPLINE_CURVE_WITH_KNOTS ( ( 4, 4 ),
 ( 1.570796326794896558, 3.141592653589793116 ),
 .UNSPECIFIED. ) 
 CURVE ( )  GEOMETRIC_REPRESENTATION_ITEM ( )  RATIONAL_B_SPLINE_CURVE ( ( 1.000000000000000000, 0.8047378541243649375, 0.8047378541243649375, 1.000000000000000000 ) ) 
 REPRESENTATION_ITEM ( '' )  );
#29697=LINE ( 'NONE', #49151, #19143 ) ;
#29699=ORIENTED_EDGE ( 'NONE', *, *, #35359, .F. ) ;
#29710=FACE_OUTER_BOUND ( 'NONE', #10678, .T. ) ;
#29711=ORIENTED_EDGE ( 'NONE', *, *, #37796, .T. ) ;
#29713=DIRECTION ( 'NONE',  ( -0.000000000000000000, -0.000000000000000000, -1.000000000000000000 ) ) ;
#29714=CARTESIAN_POINT ( 'NONE',  ( 210.0000000000000568, 2.143131898507881856E-16, -80.93171244307202983 ) ) ;
#29715=CARTESIAN_POINT ( 'NONE',  ( -84.94597344681494633, 2.143131898507880377E-16, 165.0000000000000000 ) ) ;
#29716=EDGE_CURVE ( 'NONE', #17436, #3012, #24095, .T. ) ;
#29717=ORIENTED_EDGE ( 'NONE', *, *, #43706, .T. ) ;
#29720=EDGE_LOOP ( 'NONE', ( #45918, #39278, #43777, #11359, #33763, #42881 ) ) ;
#29726=ORIENTED_EDGE ( 'NONE', *, *, #17680, .F. ) ;
#29727=CARTESIAN_POINT ( 'NONE',  ( -128.4459734468149179, 2.143131898507880377E-16, -160.9317124430720298 ) ) ;
#29739=ORIENTED_EDGE ( 'NONE', *, *, #33972, .F. ) ;
#29742=AXIS2_PLACEMENT_3D ( 'NONE', #9491, #14091, #40801 ) ;
#29745=AXIS2_PLACEMENT_3D ( 'NONE', #7123, #33823, #26870 ) ;
#29746=ADVANCED_FACE ( 'NONE', ( #48994 ), #48500, .T. ) ;
#29747=LINE ( 'NONE', #22041, #29856 ) ;
#29750=CARTESIAN_POINT ( 'NONE',  ( 195.0540265531851105, -1.025126265847088991, 2.568287556927986159 ) ) ;
#29754=LINE ( 'NONE', #5387, #33308 ) ;
#29758=( BOUNDED_CURVE ( )  B_SPLINE_CURVE ( 3, ( #24453, #44419, #44173, #16737 ),
 .UNSPECIFIED., .F., .F. ) 
 B_SPLINE_CURVE_WITH_KNOTS ( ( 4, 4 ),
 ( 4.712388980384689674, 6.283185307179586232 ),
 .UNSPECIFIED. ) 
 CURVE ( )  GEOMETRIC_REPRESENTATION_ITEM ( )  RATIONAL_B_SPLINE_CURVE ( ( 1.000000000000000000, 0.8047378541243649375, 0.8047378541243649375, 1.000000000000000000 ) ) 
 REPRESENTATION_ITEM ( '' )  );
#29761=EDGE_CURVE ( 'NONE', #8521, #5511, #4749, .T. ) ;
#29764=ORIENTED_EDGE ( 'NONE', *, *, #33765, .F. ) ;
#29767=( BOUNDED_CURVE ( )  B_SPLINE_CURVE ( 3, ( #43784, #32011, #4036, #12744 ),
 .UNSPECIFIED., .F., .F. ) 
 B_SPLINE_CURVE_WITH_KNOTS ( ( 4, 4 ),
 ( 1.570796326794896558, 3.141592653589793116 ),
 .UNSPECIFIED. ) 
 CURVE ( )  GEOMETRIC_REPRESENTATION_ITEM ( )  RATIONAL_B_SPLINE_CURVE ( ( 1.000000000000000000, 0.8047378541243649375, 0.8047378541243649375, 1.000000000000000000 ) ) 
 REPRESENTATION_ITEM ( '' )  );
#29774=ORIENTED_EDGE ( 'NONE', *, *, #45840, .F. ) ;
#29781=CARTESIAN_POINT ( 'NONE',  ( -125.6708471809678542, -1.749999999999996669, 161.8434138227750907 ) ) ;
#29782=( BOUNDED_CURVE ( )  B_SPLINE_CURVE ( 3, ( #19022, #25739, #21888, #42122 ),
 .UNSPECIFIED., .F., .F. ) 
 B_SPLINE_CURVE_WITH_KNOTS ( ( 4, 4 ),
 ( 1.570796326794896558, 3.141592653589793116 ),
 .UNSPECIFIED. ) 
 CURVE ( )  GEOMETRIC_REPRESENTATION_ITEM ( )  RATIONAL_B_SPLINE_CURVE ( ( 1.000000000000000000, 0.8047378541243649375, 0.8047378541243649375, 1.000000000000000000 ) ) 
 REPRESENTATION_ITEM ( '' )  );
#29789=CARTESIAN_POINT ( 'NONE',  ( -166.6959734468149463, 1.750000000000010658, 80.81828755692798438 ) ) ;
#29797=ORIENTED_EDGE ( 'NONE', *, *, #35190, .T. ) ;
#29799=CARTESIAN_POINT ( 'NONE',  ( -127.7210997126620242, -1.749999999999996891, 121.8434138227750481 ) ) ;
#29803=CARTESIAN_POINT ( 'NONE',  ( -44.94597344681493922, 2.143131898507882349E-16, -165.0000000000000000 ) ) ;
#29804=ORIENTED_EDGE ( 'NONE', *, *, #38948, .F. ) ;
#29806=EDGE_CURVE ( 'NONE', #35123, #31511, #6390, .T. ) ;
#29807=CARTESIAN_POINT ( 'NONE',  ( 210.0000000000000568, 0.000000000000000000, -37.43171244307202272 ) ) ;
#29808=CARTESIAN_POINT ( 'NONE',  ( -168.4459734468149463, 0.000000000000000000, 165.0000000000000000 ) ) ;
#29811=EDGE_LOOP ( 'NONE', ( #28367, #11310, #4505, #18892, #43688, #6816 ) ) ;
#29812=ORIENTED_EDGE ( 'NONE', *, *, #81, .F. ) ;
#29816=VECTOR ( 'NONE', #41808, 1000.000000000000000 ) ;
#29818=CARTESIAN_POINT ( 'NONE',  ( 73.30402655318508209, -1.750000000000009992, 0.8182875569279768335 ) ) ;
#29820=AXIS2_PLACEMENT_3D ( 'NONE', #44028, #39203, #43280 ) ;
#29825=CYLINDRICAL_SURFACE ( 'NONE', #45688, 1.750000000000001554 ) ;
#29829=CARTESIAN_POINT ( 'NONE',  ( -46.69597344681494633, 1.750000000000010658, -119.1817124430720440 ) ) ;
#29830=ORIENTED_EDGE ( 'NONE', *, *, #32504, .F. ) ;
#29833=CARTESIAN_POINT ( 'NONE',  ( 33.30402655318503946, -1.750000000000010214, -39.18171244307202983 ) ) ;
#29845=ORIENTED_EDGE ( 'NONE', *, *, #39944, .T. ) ;
#29846=DIRECTION ( 'NONE',  ( -0.000000000000000000, -0.000000000000000000, -1.000000000000000000 ) ) ;
#29847=ORIENTED_EDGE ( 'NONE', *, *, #48489, .T. ) ;
#29848=CARTESIAN_POINT ( 'NONE',  ( 195.0540265531851105, -1.025126265847088991, 159.0682875569279418 ) ) ;
#29850=DIRECTION ( 'NONE',  ( 0.000000000000000000, 0.000000000000000000, 1.000000000000000000 ) ) ;
#29856=VECTOR ( 'NONE', #49452, 1000.000000000000000 ) ;
#29860=CARTESIAN_POINT ( 'NONE',  ( 35.05402655318504657, 1.025126265847089657, -120.9317124430720440 ) ) ;
#29863=ORIENTED_EDGE ( 'NONE', *, *, #45662, .T. ) ;
#29872=CARTESIAN_POINT ( 'NONE',  ( 210.0000000000000568, 0.000000000000000000, 42.56828755692799149 ) ) ;
#29875=DIRECTION ( 'NONE',  ( -1.000000000000000000, -0.000000000000000000, -0.000000000000000000 ) ) ;
#29882=CARTESIAN_POINT ( 'NONE',  ( -86.69597344681494633, 1.750000000000009992, -159.1817124430720298 ) ) ;
#29886=CARTESIAN_POINT ( 'NONE',  ( -126.6959734468149321, 1.749999999999996891, -159.1817124430720298 ) ) ;
#29887=DIRECTION ( 'NONE',  ( -0.000000000000000000, -0.000000000000000000, -1.000000000000000000 ) ) ;
#29888=CARTESIAN_POINT ( 'NONE',  ( -168.4459734468149747, 1.025126265847088991, -157.4317124430720582 ) ) ;
#29890=AXIS2_PLACEMENT_3D ( 'NONE', #36340, #12950, #9120 ) ;
#29894=CARTESIAN_POINT ( 'NONE',  ( 151.5540265531850537, 0.000000000000000000, -0.9317124430720247208 ) ) ;
#29900=VERTEX_POINT ( 'NONE', #12806 ) ;
#29905=VECTOR ( 'NONE', #3638, 1000.000000000000000 ) ;
#29909=ORIENTED_EDGE ( 'NONE', *, *, #12028, .F. ) ;
#29910=ORIENTED_EDGE ( 'NONE', *, *, #43970, .F. ) ;
#29914=DIRECTION ( 'NONE',  ( -1.000000000000000000, -0.000000000000000000, -0.000000000000000000 ) ) ;
#29915=CARTESIAN_POINT ( 'NONE',  ( 195.0540265531851105, 1.025126265847089657, -37.43171244307202272 ) ) ;
#29920=( BOUNDED_CURVE ( )  B_SPLINE_CURVE ( 3, ( #14514, #34033, #13562, #25377 ),
 .UNSPECIFIED., .F., .F. ) 
 B_SPLINE_CURVE_WITH_KNOTS ( ( 4, 4 ),
 ( 4.712388980384689674, 6.283185307179586232 ),
 .UNSPECIFIED. ) 
 CURVE ( )  GEOMETRIC_REPRESENTATION_ITEM ( )  RATIONAL_B_SPLINE_CURVE ( ( 1.000000000000000000, 0.8047378541243649375, 0.8047378541243649375, 1.000000000000000000 ) ) 
 REPRESENTATION_ITEM ( '' )  );
#29922=EDGE_CURVE ( 'NONE', #44427, #34969, #40128, .T. ) ;
#29929=ORIENTED_EDGE ( 'NONE', *, *, #22103, .F. ) ;
#29937=EDGE_CURVE ( 'NONE', #13146, #7036, #25736, .T. ) ;
#29939=EDGE_CURVE ( 'NONE', #23932, #7036, #22129, .T. ) ;
#29942=LINE ( 'NONE', #48882, #50308 ) ;
#29945=CARTESIAN_POINT ( 'NONE',  ( -4.945973446814916130, 1.025126265847097651, 122.5682875569280128 ) ) ;
#29948=AXIS2_PLACEMENT_3D ( 'NONE', #13784, #2745, #34316 ) ;
#29949=ORIENTED_EDGE ( 'NONE', *, *, #28393, .F. ) ;
#29954=CARTESIAN_POINT ( 'NONE',  ( -204.9459734468149463, 2.143131898507890731E-16, 165.0000000000000000 ) ) ;
#29960=FACE_OUTER_BOUND ( 'NONE', #35076, .T. ) ;
#29967=EDGE_CURVE ( 'NONE', #21965, #34539, #1169, .T. ) ;
#29975=DIRECTION ( 'NONE',  ( -0.000000000000000000, -0.000000000000000000, -1.000000000000000000 ) ) ;
#29980=CARTESIAN_POINT ( 'NONE',  ( -4.945973446814903696, 2.143131898507912917E-16, -120.9317124430720725 ) ) ;
#29981=AXIS2_PLACEMENT_3D ( 'NONE', #26575, #22719, #11946 ) ;
#29982=ORIENTED_EDGE ( 'NONE', *, *, #19095, .F. ) ;
#29985=EDGE_CURVE ( 'NONE', #19548, #30870, #13864, .T. ) ;
#29991=VERTEX_POINT ( 'NONE', #41049 ) ;
#29993=CARTESIAN_POINT ( 'NONE',  ( -88.44597344681497475, 0.000000000000000000, 82.56828755692801280 ) ) ;
#29996=EDGE_CURVE ( 'NONE', #41657, #38451, #30258, .T. ) ;
#29998=ADVANCED_FACE ( 'NONE', ( #37229 ), #14086, .F. ) ;
#29999=CYLINDRICAL_SURFACE ( 'NONE', #48861, 1.750000000000008438 ) ;
#30000=CARTESIAN_POINT ( 'NONE',  ( -204.9459734468149463, 2.143131898507880377E-16, 39.06828755692798438 ) ) ;
#30006=EDGE_CURVE ( 'NONE', #13383, #43783, #36238, .T. ) ;
#30007=PLANE ( 'NONE',  #25056 ) ;
#30008=EDGE_LOOP ( 'NONE', ( #12506, #16086, #18210, #16101, #34272, #24720 ) ) ;
#30016=( BOUNDED_CURVE ( )  B_SPLINE_CURVE ( 3, ( #30772, #14858, #6910, #39236 ),
 .UNSPECIFIED., .F., .F. ) 
 B_SPLINE_CURVE_WITH_KNOTS ( ( 4, 4 ),
 ( 1.570796326794896558, 3.141592653589793116 ),
 .UNSPECIFIED. ) 
 CURVE ( )  GEOMETRIC_REPRESENTATION_ITEM ( )  RATIONAL_B_SPLINE_CURVE ( ( 1.000000000000000000, 0.8047378541243649375, 0.8047378541243649375, 1.000000000000000000 ) ) 
 REPRESENTATION_ITEM ( '' )  );
#30023=CARTESIAN_POINT ( 'NONE',  ( 113.3040265531850537, 1.749999999999997335, -119.1817124430720440 ) ) ;
#30027=ADVANCED_FACE ( 'NONE', ( #2050 ), #17696, .T. ) ;
#30032=CARTESIAN_POINT ( 'NONE',  ( 195.0540265531851105, 2.143131898507880377E-16, 165.0000000000000000 ) ) ;
#30034=DIRECTION ( 'NONE',  ( 0.000000000000000000, 0.000000000000000000, -1.000000000000000000 ) ) ;
#30035=LINE ( 'NONE', #45640, #20058 ) ;
#30036=CARTESIAN_POINT ( 'NONE',  ( 113.3040265531850537, 1.749999999999997335, 80.81828755692798438 ) ) ;
#30037=VECTOR ( 'NONE', #38781, 1000.000000000000000 ) ;
#30039=DIRECTION ( 'NONE',  ( -1.000000000000000000, 0.000000000000000000, 0.000000000000000000 ) ) ;
#30041=CARTESIAN_POINT ( 'NONE',  ( 74.32915281903215998, -1.750000000000009548, -40.20683870891912193 ) ) ;
#30049=CARTESIAN_POINT ( 'NONE',  ( 34.32915281903212446, -1.750000000000009548, 39.79316129108089228 ) ) ;
#30054=CARTESIAN_POINT ( 'NONE',  ( 193.3040265531851105, 1.750000000000010214, -39.18171244307202983 ) ) ;
#30056=VERTEX_POINT ( 'NONE', #37474 ) ;
#30059=EDGE_CURVE ( 'NONE', #24640, #26096, #48898, .T. ) ;
#30061=EDGE_CURVE ( 'NONE', #45355, #39370, #47275, .T. ) ;
#30062=AXIS2_PLACEMENT_3D ( 'NONE', #2474, #49628, #45791 ) ;
#30065=ORIENTED_EDGE ( 'NONE', *, *, #7420, .T. ) ;
#30069=ORIENTED_EDGE ( 'NONE', *, *, #42974, .F. ) ;
#30072=CARTESIAN_POINT ( 'NONE',  ( -48.44597344681495343, 0.000000000000000000, -117.4317124430720156 ) ) ;
#30073=EDGE_CURVE ( 'NONE', #13712, #24906, #48602, .T. ) ;
#30074=( BOUNDED_CURVE ( )  B_SPLINE_CURVE ( 3, ( #1678, #13212, #5266, #44494 ),
 .UNSPECIFIED., .F., .F. ) 
 B_SPLINE_CURVE_WITH_KNOTS ( ( 4, 4 ),
 ( 3.141592653589793116, 4.712388980384689674 ),
 .UNSPECIFIED. ) 
 CURVE ( )  GEOMETRIC_REPRESENTATION_ITEM ( )  RATIONAL_B_SPLINE_CURVE ( ( 1.000000000000000000, 0.8047378541243649375, 0.8047378541243649375, 1.000000000000000000 ) ) 
 REPRESENTATION_ITEM ( '' )  );
#30076=ORIENTED_EDGE ( 'NONE', *, *, #41215, .F. ) ;
#30078=( BOUNDED_CURVE ( )  B_SPLINE_CURVE ( 3, ( #24542, #20687, #17090, #45012 ),
 .UNSPECIFIED., .F., .F. ) 
 B_SPLINE_CURVE_WITH_KNOTS ( ( 4, 4 ),
 ( 0.000000000000000000, 1.570796326794896558 ),
 .UNSPECIFIED. ) 
 CURVE ( )  GEOMETRIC_REPRESENTATION_ITEM ( )  RATIONAL_B_SPLINE_CURVE ( ( 1.000000000000000000, 0.8047378541243649375, 0.8047378541243649375, 1.000000000000000000 ) ) 
 REPRESENTATION_ITEM ( '' )  );
#30079=ADVANCED_FACE ( 'NONE', ( #16130 ), #7162, .T. ) ;
#30088=LINE ( 'NONE', #33441, #37349 ) ;
#30091=ORIENTED_EDGE ( 'NONE', *, *, #32564, .F. ) ;
#30099=ORIENTED_EDGE ( 'NONE', *, *, #43706, .F. ) ;
#30104=EDGE_CURVE ( 'NONE', #16089, #42464, #31291, .T. ) ;
#30107=CARTESIAN_POINT ( 'NONE',  ( -5.670847180967843570, 1.750000000000022427, 161.8434138227750907 ) ) ;
#30108=ORIENTED_EDGE ( 'NONE', *, *, #39974, .F. ) ;
#30109=EDGE_LOOP ( 'NONE', ( #46274, #31359, #2170, #40119, #11961, #45879 ) ) ;
#30114=DIRECTION ( 'NONE',  ( -1.000000000000000000, 0.000000000000000000, 0.000000000000000000 ) ) ;
#30116=CARTESIAN_POINT ( 'NONE',  ( 31.55402655318503236, 0.000000000000000000, 159.0682875569279702 ) ) ;
#30123=AXIS2_PLACEMENT_3D ( 'NONE', #46560, #35088, #15561 ) ;
#30125=ORIENTED_EDGE ( 'NONE', *, *, #38669, .T. ) ;
#30130=DIRECTION ( 'NONE',  ( -1.000000000000000000, -0.000000000000000000, -0.000000000000000000 ) ) ;
#30139=CARTESIAN_POINT ( 'NONE',  ( -86.69597344681494633, 1.750000000000010214, -39.18171244307202983 ) ) ;
#30140=CARTESIAN_POINT ( 'NONE',  ( -165.6708471809677974, -1.750000000000010436, -120.2068387089191219 ) ) ;
#30141=ORIENTED_EDGE ( 'NONE', *, *, #3999, .T. ) ;
#30144=DIRECTION ( 'NONE',  ( 0.000000000000000000, 0.000000000000000000, 1.000000000000000000 ) ) ;
#30145=DIRECTION ( 'NONE',  ( 1.000000000000000000, 0.000000000000000000, 0.000000000000000000 ) ) ;
#30146=DIRECTION ( 'NONE',  ( -1.000000000000000000, 0.000000000000000000, 0.000000000000000000 ) ) ;
#30147=FACE_OUTER_BOUND ( 'NONE', #13402, .T. ) ;
#30159=ORIENTED_EDGE ( 'NONE', *, *, #21901, .T. ) ;
#30160=ORIENTED_EDGE ( 'NONE', *, *, #1547, .F. ) ;
#30171=CARTESIAN_POINT ( 'NONE',  ( 113.3040265531850537, -1.749999999999997113, -39.18171244307202983 ) ) ;
#30173=ORIENTED_EDGE ( 'NONE', *, *, #48394, .T. ) ;
#30174=DIRECTION ( 'NONE',  ( 0.000000000000000000, 0.000000000000000000, 1.000000000000000000 ) ) ;
#30179=CARTESIAN_POINT ( 'NONE',  ( 75.05402655318509630, 2.143131898507880377E-16, 165.0000000000000000 ) ) ;
#30182=CARTESIAN_POINT ( 'NONE',  ( 71.55402655318505367, 0.000000000000000000, 79.06828755692797017 ) ) ;
#30186=DIRECTION ( 'NONE',  ( 0.000000000000000000, 0.000000000000000000, 1.000000000000000000 ) ) ;
#30187=DIRECTION ( 'NONE',  ( -0.000000000000000000, -0.000000000000000000, -1.000000000000000000 ) ) ;
#30190=VERTEX_POINT ( 'NONE', #42545 ) ;
#30195=ADVANCED_FACE ( 'NONE', ( #38981 ), #3814, .T. ) ;
#30204=EDGE_CURVE ( 'NONE', #14675, #36229, #6995, .T. ) ;
#30206=CARTESIAN_POINT ( 'NONE',  ( 115.0540265531850395, 2.143131898507847836E-16, -157.4317124430720582 ) ) ;
#30207=EDGE_CURVE ( 'NONE', #15732, #40036, #31791, .T. ) ;
#30212=DIRECTION ( 'NONE',  ( 1.000000000000000000, 0.000000000000000000, 0.000000000000000000 ) ) ;
#30213=CARTESIAN_POINT ( 'NONE',  ( 151.5540265531850537, 0.000000000000000000, 159.0682875569279702 ) ) ;
#30215=CARTESIAN_POINT ( 'NONE',  ( -46.69597344681494633, 1.750000000000010658, 120.8182875569279702 ) ) ;
#30216=EDGE_CURVE ( 'NONE', #21335, #16313, #6686, .T. ) ;
#30217=( BOUNDED_CURVE ( )  B_SPLINE_CURVE ( 3, ( #14960, #49548, #30107, #41898 ),
 .UNSPECIFIED., .F., .F. ) 
 B_SPLINE_CURVE_WITH_KNOTS ( ( 4, 4 ),
 ( 3.141592653589793116, 4.712388980384689674 ),
 .UNSPECIFIED. ) 
 CURVE ( )  GEOMETRIC_REPRESENTATION_ITEM ( )  RATIONAL_B_SPLINE_CURVE ( ( 1.000000000000000000, 0.8047378541243649375, 0.8047378541243649375, 1.000000000000000000 ) ) 
 REPRESENTATION_ITEM ( '' )  );
#30219=DIRECTION ( 'NONE',  ( -1.000000000000000000, -0.000000000000000000, -0.000000000000000000 ) ) ;
#30220=ORIENTED_EDGE ( 'NONE', *, *, #45075, .T. ) ;
#30221=ORIENTED_EDGE ( 'NONE', *, *, #15192, .F. ) ;
#30227=CYLINDRICAL_SURFACE ( 'NONE', #27399, 1.750000000000010214 ) ;
#30236=FACE_OUTER_BOUND ( 'NONE', #28585, .T. ) ;
#30237=CARTESIAN_POINT ( 'NONE',  ( 75.05402655318509630, 2.143131898507880377E-16, 159.0682875569279702 ) ) ;
#30247=ORIENTED_EDGE ( 'NONE', *, *, #30906, .F. ) ;
#30249=CARTESIAN_POINT ( 'NONE',  ( -164.9459734468149463, 2.143131898507880377E-16, -80.93171244307201562 ) ) ;
#30250=EDGE_CURVE ( 'NONE', #10906, #21159, #36549, .T. ) ;
#30252=PRODUCT_DEFINITION_SHAPE ( 'NONE', 'NONE',  #38783 ) ;
#30254=EDGE_CURVE ( 'NONE', #17123, #29900, #11953, .T. ) ;
#30255=CARTESIAN_POINT ( 'NONE',  ( 113.3040265531850537, 0.000000000000000000, 165.0000000000000000 ) ) ;
#30258=LINE ( 'NONE', #17929, #46423 ) ;
#30262=DIRECTION ( 'NONE',  ( 0.000000000000000000, 0.000000000000000000, 1.000000000000000000 ) ) ;
#30264=ORIENTED_EDGE ( 'NONE', *, *, #459, .T. ) ;
#30273=ORIENTED_EDGE ( 'NONE', *, *, #36311, .T. ) ;
#30274=CARTESIAN_POINT ( 'NONE',  ( -4.945973446814903696, 2.143131898507912917E-16, -40.93171244307205825 ) ) ;
#30276=CARTESIAN_POINT ( 'NONE',  ( -45.67084718096785423, 1.750000000000010214, -78.15658617722490931 ) ) ;
#30277=VECTOR ( 'NONE', #10152, 1000.000000000000000 ) ;
#30283=CARTESIAN_POINT ( 'NONE',  ( -4.945973446814903696, 2.143131898507912917E-16, 159.0682875569279418 ) ) ;
#30284=ORIENTED_EDGE ( 'NONE', *, *, #44048, .T. ) ;
#30286=CARTESIAN_POINT ( 'NONE',  ( 210.0000000000000568, 0.000000000000000000, 122.5682875569279844 ) ) ;
#30287=CARTESIAN_POINT ( 'NONE',  ( -126.6959734468149321, -1.749999999999996891, 160.8182875569279702 ) ) ;
#30288=EDGE_CURVE ( 'NONE', #11124, #38096, #44307, .T. ) ;
#30292=EDGE_CURVE ( 'NONE', #1914, #21304, #50508, .T. ) ;
#30293=CYLINDRICAL_SURFACE ( 'NONE', #19339, 1.749999999999973799 ) ;
#30299=LINE ( 'NONE', #49993, #47955 ) ;
#30303=VECTOR ( 'NONE', #20818, 1000.000000000000000 ) ;
#30309=( BOUNDED_CURVE ( )  B_SPLINE_CURVE ( 3, ( #9971, #29473, #33336, #28474 ),
 .UNSPECIFIED., .F., .F. ) 
 B_SPLINE_CURVE_WITH_KNOTS ( ( 4, 4 ),
 ( 4.712388980384689674, 6.283185307179586232 ),
 .UNSPECIFIED. ) 
 CURVE ( )  GEOMETRIC_REPRESENTATION_ITEM ( )  RATIONAL_B_SPLINE_CURVE ( ( 1.000000000000000000, 0.8047378541243649375, 0.8047378541243649375, 1.000000000000000000 ) ) 
 REPRESENTATION_ITEM ( '' )  );
#30311=CARTESIAN_POINT ( 'NONE',  ( 115.0540265531850395, 2.143131898507847836E-16, 165.0000000000000000 ) ) ;
#30313=DIRECTION ( 'NONE',  ( 0.000000000000000000, 0.000000000000000000, 1.000000000000000000 ) ) ;
#30314=ORIENTED_EDGE ( 'NONE', *, *, #44747, .F. ) ;
#30317=DIRECTION ( 'NONE',  ( -1.000000000000000000, -0.000000000000000000, -0.000000000000000000 ) ) ;
#30318=VECTOR ( 'NONE', #17969, 1000.000000000000000 ) ;
#30320=ORIENTED_EDGE ( 'NONE', *, *, #1178, .T. ) ;
#30325=EDGE_LOOP ( 'NONE', ( #43600, #50456, #26577, #30429, #39704, #36649 ) ) ;
#30328=CARTESIAN_POINT ( 'NONE',  ( 210.0000000000000568, 0.000000000000000000, 40.81828755692798438 ) ) ;
#30330=CARTESIAN_POINT ( 'NONE',  ( -126.6959734468149321, 1.749999999999996891, -159.1817124430720298 ) ) ;
#30331=DIRECTION ( 'NONE',  ( -0.000000000000000000, -0.000000000000000000, -1.000000000000000000 ) ) ;
#30337=AXIS2_PLACEMENT_3D ( 'NONE', #9151, #40466, #40718 ) ;
#30342=EDGE_CURVE ( 'NONE', #30870, #10383, #40987, .T. ) ;
#30343=ORIENTED_EDGE ( 'NONE', *, *, #44643, .T. ) ;
#30344=VECTOR ( 'NONE', #7875, 1000.000000000000000 ) ;
#30347=CIRCLE ( 'NONE', #49957, 1.750000000000001554 ) ;
#30348=DIRECTION ( 'NONE',  ( -1.000000000000000000, 0.000000000000000000, 0.000000000000000000 ) ) ;
#30351=EDGE_CURVE ( 'NONE', #50360, #7318, #20473, .T. ) ;
#30363=ORIENTED_EDGE ( 'NONE', *, *, #18018, .F. ) ;
#30366=( BOUNDED_CURVE ( )  B_SPLINE_CURVE ( 3, ( #46911, #46148, #275, #42835 ),
 .UNSPECIFIED., .F., .F. ) 
 B_SPLINE_CURVE_WITH_KNOTS ( ( 4, 4 ),
 ( 1.570796326794896558, 3.141592653589793116 ),
 .UNSPECIFIED. ) 
 CURVE ( )  GEOMETRIC_REPRESENTATION_ITEM ( )  RATIONAL_B_SPLINE_CURVE ( ( 1.000000000000000000, 0.8047378541243649375, 0.8047378541243649375, 1.000000000000000000 ) ) 
 REPRESENTATION_ITEM ( '' )  );
#30372=ORIENTED_EDGE ( 'NONE', *, *, #28077, .T. ) ;
#30373=DIRECTION ( 'NONE',  ( -0.000000000000000000, -0.000000000000000000, -1.000000000000000000 ) ) ;
#30374=ORIENTED_EDGE ( 'NONE', *, *, #15506, .F. ) ;
#30375=( BOUNDED_CURVE ( )  B_SPLINE_CURVE ( 3, ( #37061, #2143, #17787, #17533 ),
 .UNSPECIFIED., .F., .F. ) 
 B_SPLINE_CURVE_WITH_KNOTS ( ( 4, 4 ),
 ( 1.570796326794896558, 3.141592653589793116 ),
 .UNSPECIFIED. ) 
 CURVE ( )  GEOMETRIC_REPRESENTATION_ITEM ( )  RATIONAL_B_SPLINE_CURVE ( ( 1.000000000000000000, 0.8047378541243649375, 0.8047378541243649375, 1.000000000000000000 ) ) 
 REPRESENTATION_ITEM ( '' )  );
#30378=VECTOR ( 'NONE', #10977, 1000.000000000000000 ) ;
#30382=VERTEX_POINT ( 'NONE', #18378 ) ;
#30389=AXIS2_PLACEMENT_3D ( 'NONE', #5851, #9697, #48401 ) ;
#30396=LINE ( 'NONE', #7291, #21659 ) ;
#30401=DIRECTION ( 'NONE',  ( -1.000000000000000000, -0.000000000000000000, -0.000000000000000000 ) ) ;
#30403=ADVANCED_FACE ( 'NONE', ( #37162 ), #34058, .T. ) ;
#30404=CARTESIAN_POINT ( 'NONE',  ( 114.3291528190321173, -1.749999999999996669, -0.2068387089191042749 ) ) ;
#30413=DIRECTION ( 'NONE',  ( -1.000000000000000000, 0.000000000000000000, 0.000000000000000000 ) ) ;
#30419=AXIS2_PLACEMENT_3D ( 'NONE', #38627, #39393, #11167 ) ;
#30421=DIRECTION ( 'NONE',  ( -0.000000000000000000, -0.000000000000000000, -1.000000000000000000 ) ) ;
#30426=CARTESIAN_POINT ( 'NONE',  ( 35.05402655318504657, 2.143131898507880377E-16, 165.0000000000000000 ) ) ;
#30427=VERTEX_POINT ( 'NONE', #9931 ) ;
#30428=ORIENTED_EDGE ( 'NONE', *, *, #26189, .F. ) ;
#30429=ORIENTED_EDGE ( 'NONE', *, *, #4280, .T. ) ;
#30431=CYLINDRICAL_SURFACE ( 'NONE', #5397, 1.750000000000015543 ) ;
#30435=CARTESIAN_POINT ( 'NONE',  ( -204.9459734468149463, 2.143131898507880377E-16, 2.568287556927978166 ) ) ;
#30438=ORIENTED_EDGE ( 'NONE', *, *, #39696, .F. ) ;
#30441=AXIS2_PLACEMENT_3D ( 'NONE', #17458, #25928, #25414 ) ;
#30442=CARTESIAN_POINT ( 'NONE',  ( 73.30402655318508209, -1.750000000000010658, 80.81828755692798438 ) ) ;
#30444=ORIENTED_EDGE ( 'NONE', *, *, #44072, .T. ) ;
#30445=ADVANCED_FACE ( 'NONE', ( #17873 ), #33552, .T. ) ;
#30447=FACE_OUTER_BOUND ( 'NONE', #19010, .T. ) ;
#30451=CARTESIAN_POINT ( 'NONE',  ( -205.6708471809678827, 1.750000000000010214, -78.15658617722490931 ) ) ;
#30453=DIRECTION ( 'NONE',  ( -1.000000000000000000, -0.000000000000000000, -0.000000000000000000 ) ) ;
#30455=DIRECTION ( 'NONE',  ( 0.000000000000000000, 0.000000000000000000, 1.000000000000000000 ) ) ;
#30458=FACE_OUTER_BOUND ( 'NONE', #16616, .T. ) ;
#30464=ORIENTED_EDGE ( 'NONE', *, *, #11357, .F. ) ;
#30470=EDGE_CURVE ( 'NONE', #27492, #17731, #45320, .T. ) ;
#30479=ORIENTED_EDGE ( 'NONE', *, *, #19898, .F. ) ;
#30482=CYLINDRICAL_SURFACE ( 'NONE', #35590, 1.750000000000001554 ) ;
#30483=CARTESIAN_POINT ( 'NONE',  ( -208.4459734468149463, 0.000000000000000000, -120.9317124430720156 ) ) ;
#30484=CARTESIAN_POINT ( 'NONE',  ( -47.72109971266203132, -1.750000000000010214, 119.7931612910808781 ) ) ;
#30487=EDGE_CURVE ( 'NONE', #15638, #43597, #3084, .T. ) ;
#30493=CARTESIAN_POINT ( 'NONE',  ( -167.7210997126620384, -1.750000000000009548, 41.84341382277508359 ) ) ;
#30495=VERTEX_POINT ( 'NONE', #31224 ) ;
#30496=EDGE_LOOP ( 'NONE', ( #42822, #38532, #13931, #18449, #5930, #17356 ) ) ;
#30503=CARTESIAN_POINT ( 'NONE',  ( 195.0540265531851105, 2.143131898507880377E-16, 165.0000000000000000 ) ) ;
#30506=CARTESIAN_POINT ( 'NONE',  ( 112.2789002873379758, 1.749999999999996891, 39.79316129108089228 ) ) ;
#30508=DIRECTION ( 'NONE',  ( -0.000000000000000000, -0.000000000000000000, -1.000000000000000000 ) ) ;
#30511=( BOUNDED_CURVE ( )  B_SPLINE_CURVE ( 3, ( #11325, #18509, #34955, #42863 ),
 .UNSPECIFIED., .F., .F. ) 
 B_SPLINE_CURVE_WITH_KNOTS ( ( 4, 4 ),
 ( 0.000000000000000000, 1.570796326794896558 ),
 .UNSPECIFIED. ) 
 CURVE ( )  GEOMETRIC_REPRESENTATION_ITEM ( )  RATIONAL_B_SPLINE_CURVE ( ( 1.000000000000000000, 0.8047378541243649375, 0.8047378541243649375, 1.000000000000000000 ) ) 
 REPRESENTATION_ITEM ( '' )  );
#30519=CARTESIAN_POINT ( 'NONE',  ( -124.9459734468149463, 2.143131898507847836E-16, 122.5682875569279560 ) ) ;
#30521=ORIENTED_EDGE ( 'NONE', *, *, #17701, .F. ) ;
#30523=DIRECTION ( 'NONE',  ( 0.000000000000000000, 0.000000000000000000, 1.000000000000000000 ) ) ;
#30525=( BOUNDED_CURVE ( )  B_SPLINE_CURVE ( 3, ( #7097, #10682, #6841, #22736 ),
 .UNSPECIFIED., .F., .F. ) 
 B_SPLINE_CURVE_WITH_KNOTS ( ( 4, 4 ),
 ( 4.712388980384689674, 6.283185307179586232 ),
 .UNSPECIFIED. ) 
 CURVE ( )  GEOMETRIC_REPRESENTATION_ITEM ( )  RATIONAL_B_SPLINE_CURVE ( ( 1.000000000000000000, 0.8047378541243649375, 0.8047378541243649375, 1.000000000000000000 ) ) 
 REPRESENTATION_ITEM ( '' )  );
#30531=CARTESIAN_POINT ( 'NONE',  ( 35.05402655318504657, -1.025126265847089435, 82.56828755692798438 ) ) ;
#30536=CARTESIAN_POINT ( 'NONE',  ( -84.94597344681494633, 2.143131898507880377E-16, 119.0682875569279702 ) ) ;
#30538=CARTESIAN_POINT ( 'NONE',  ( 74.32915281903215998, -1.750000000000009548, -38.15658617722494483 ) ) ;
#30544=ADVANCED_FACE ( 'NONE', ( #50140 ), #3228, .T. ) ;
#30550=LINE ( 'NONE', #7201, #4925 ) ;
#30555=ORIENTED_EDGE ( 'NONE', *, *, #30470, .F. ) ;
#30562=DIRECTION ( 'NONE',  ( -1.000000000000000000, 0.000000000000000000, 0.000000000000000000 ) ) ;
#30564=DIRECTION ( 'NONE',  ( 1.000000000000000000, 0.000000000000000000, 0.000000000000000000 ) ) ;
#30565=CARTESIAN_POINT ( 'NONE',  ( 154.3291528190321458, 1.750000000000010214, -80.20683870891910772 ) ) ;
#30573=LINE ( 'NONE', #45679, #13247 ) ;
#30576=VECTOR ( 'NONE', #28121, 1000.000000000000000 ) ;
#30578=CYLINDRICAL_SURFACE ( 'NONE', #25333, 1.750000000000015543 ) ;
#30579=ADVANCED_FACE ( 'NONE', ( #22743 ), #23243, .T. ) ;
#30581=ADVANCED_FACE ( 'NONE', ( #7357 ), #38663, .T. ) ;
#30583=ORIENTED_EDGE ( 'NONE', *, *, #30634, .T. ) ;
#30585=CARTESIAN_POINT ( 'NONE',  ( 155.0540265531850537, 2.143131898507880377E-16, 2.568287556927978166 ) ) ;
#30591=AXIS2_PLACEMENT_3D ( 'NONE', #45507, #26546, #25791 ) ;
#30598=EDGE_CURVE ( 'NONE', #23271, #47489, #50550, .T. ) ;
#30602=DIRECTION ( 'NONE',  ( -0.000000000000000000, -0.000000000000000000, -1.000000000000000000 ) ) ;
#30604=CARTESIAN_POINT ( 'NONE',  ( -45.67084718096785423, 1.750000000000009548, 159.7931612910809065 ) ) ;
#30607=FACE_OUTER_BOUND ( 'NONE', #16824, .T. ) ;
#30611=( BOUNDED_CURVE ( )  B_SPLINE_CURVE ( 3, ( #16350, #50442, #31259, #31513 ),
 .UNSPECIFIED., .F., .F. ) 
 B_SPLINE_CURVE_WITH_KNOTS ( ( 4, 4 ),
 ( 4.712388980384689674, 6.283185307179586232 ),
 .UNSPECIFIED. ) 
 CURVE ( )  GEOMETRIC_REPRESENTATION_ITEM ( )  RATIONAL_B_SPLINE_CURVE ( ( 1.000000000000000000, 0.8047378541243649375, 0.8047378541243649375, 1.000000000000000000 ) ) 
 REPRESENTATION_ITEM ( '' )  );
#30612=CARTESIAN_POINT ( 'NONE',  ( 154.3291528190321458, -1.750000000000009548, -78.15658617722490931 ) ) ;
#30620=EDGE_LOOP ( 'NONE', ( #4068, #46727, #915, #23818, #31006, #27951 ) ) ;
#30621=CARTESIAN_POINT ( 'NONE',  ( 191.5540265531850537, 1.025126265847089435, -77.43171244307200141 ) ) ;
#30622=DIRECTION ( 'NONE',  ( -1.000000000000000000, -0.000000000000000000, -0.000000000000000000 ) ) ;
#30631=CARTESIAN_POINT ( 'NONE',  ( 195.0540265531851105, 2.143131898507880377E-16, 82.56828755692798438 ) ) ;
#30633=CARTESIAN_POINT ( 'NONE',  ( -48.44597344681495343, 0.000000000000000000, -120.9317124430720725 ) ) ;
#30634=EDGE_CURVE ( 'NONE', #30766, #40036, #11644, .T. ) ;
#30637=ORIENTED_EDGE ( 'NONE', *, *, #44681, .T. ) ;
#30638=EDGE_LOOP ( 'NONE', ( #31051, #50077, #29949, #20830, #34679, #29982 ) ) ;
#30640=CARTESIAN_POINT ( 'NONE',  ( -206.6959734468149463, 0.000000000000000000, 165.0000000000000000 ) ) ;
#30642=ORIENTED_EDGE ( 'NONE', *, *, #36594, .T. ) ;
#30648=EDGE_LOOP ( 'NONE', ( #48363, #20003, #26420, #33371, #5231, #27706 ) ) ;
#30649=EDGE_CURVE ( 'NONE', #39727, #29268, #27681, .T. ) ;
#30650=CARTESIAN_POINT ( 'NONE',  ( 33.30402655318503946, -1.750000000000009992, 160.8182875569279702 ) ) ;
#30654=VECTOR ( 'NONE', #38418, 1000.000000000000000 ) ;
#30658=CARTESIAN_POINT ( 'NONE',  ( 31.55402655318503236, 1.025126265847089213, -160.9317124430720014 ) ) ;
#30661=CARTESIAN_POINT ( 'NONE',  ( -210.0000000000000568, 0.000000000000000000, -159.1817124430720298 ) ) ;
#30670=ORIENTED_EDGE ( 'NONE', *, *, #6252, .T. ) ;
#30671=( BOUNDED_CURVE ( )  B_SPLINE_CURVE ( 3, ( #34228, #10857, #42912, #19057 ),
 .UNSPECIFIED., .F., .F. ) 
 B_SPLINE_CURVE_WITH_KNOTS ( ( 4, 4 ),
 ( 3.141592653589793116, 4.712388980384689674 ),
 .UNSPECIFIED. ) 
 CURVE ( )  GEOMETRIC_REPRESENTATION_ITEM ( )  RATIONAL_B_SPLINE_CURVE ( ( 1.000000000000000000, 0.8047378541243649375, 0.8047378541243649375, 1.000000000000000000 ) ) 
 REPRESENTATION_ITEM ( '' )  );
#30675=( BOUNDED_CURVE ( )  B_SPLINE_CURVE ( 3, ( #6565, #17607, #45779, #21704 ),
 .UNSPECIFIED., .F., .F. ) 
 B_SPLINE_CURVE_WITH_KNOTS ( ( 4, 4 ),
 ( 3.141592653589793116, 4.712388980384689674 ),
 .UNSPECIFIED. ) 
 CURVE ( )  GEOMETRIC_REPRESENTATION_ITEM ( )  RATIONAL_B_SPLINE_CURVE ( ( 1.000000000000000000, 0.8047378541243649375, 0.8047378541243649375, 1.000000000000000000 ) ) 
 REPRESENTATION_ITEM ( '' )  );
#30680=EDGE_CURVE ( 'NONE', #1904, #28356, #5034, .T. ) ;
#30683=VERTEX_POINT ( 'NONE', #20406 ) ;
#30685=CARTESIAN_POINT ( 'NONE',  ( -88.44597344681497475, 0.000000000000000000, -120.9317124430720725 ) ) ;
#30686=CARTESIAN_POINT ( 'NONE',  ( -208.4459734468148611, 1.025126265847089435, -117.4317124430720156 ) ) ;
#30688=ORIENTED_EDGE ( 'NONE', *, *, #19219, .F. ) ;
#30690=CARTESIAN_POINT ( 'NONE',  ( 191.5540265531851105, 0.000000000000000000, 159.0682875569279702 ) ) ;
#30691=DIRECTION ( 'NONE',  ( 0.000000000000000000, 0.000000000000000000, 1.000000000000000000 ) ) ;
#30693=ORIENTED_EDGE ( 'NONE', *, *, #19283, .T. ) ;
#30694=EDGE_CURVE ( 'NONE', #33167, #25636, #8018, .T. ) ;
#30697=FACE_OUTER_BOUND ( 'NONE', #40711, .T. ) ;
#30698=CARTESIAN_POINT ( 'NONE',  ( -128.4459734468149179, 0.000000000000000000, -77.43171244307204404 ) ) ;
#30701=EDGE_LOOP ( 'NONE', ( #24308, #43392, #42965, #14094, #33267, #40532 ) ) ;
#30704=CARTESIAN_POINT ( 'NONE',  ( 113.3040265531850537, 1.749999999999997335, -79.18171244307201562 ) ) ;
#30706=ORIENTED_EDGE ( 'NONE', *, *, #19863, .F. ) ;
#30711=EDGE_CURVE ( 'NONE', #2022, #46718, #6293, .T. ) ;
#30713=CARTESIAN_POINT ( 'NONE',  ( 35.05402655318504657, 2.143131898507880377E-16, -37.43171244307200141 ) ) ;
#30715=ORIENTED_EDGE ( 'NONE', *, *, #38539, .F. ) ;
#30717=ADVANCED_FACE ( 'NONE', ( #40685 ), #14217, .T. ) ;
#30720=CARTESIAN_POINT ( 'NONE',  ( 114.3291528190321173, 1.749999999999996669, 41.84341382277508359 ) ) ;
#30721=FACE_OUTER_BOUND ( 'NONE', #13888, .T. ) ;
#30722=VECTOR ( 'NONE', #50083, 1000.000000000000000 ) ;
#30724=AXIS2_PLACEMENT_3D ( 'NONE', #5402, #32365, #16459 ) ;
#30727=LINE ( 'NONE', #27127, #26652 ) ;
#30728=CARTESIAN_POINT ( 'NONE',  ( -206.6959734468149463, 1.750000000000009992, 160.8182875569279702 ) ) ;
#30734=CARTESIAN_POINT ( 'NONE',  ( 153.3040265531850537, 1.750000000000010214, -39.18171244307202983 ) ) ;
#30745=DIRECTION ( 'NONE',  ( 0.000000000000000000, 0.000000000000000000, 1.000000000000000000 ) ) ;
#30753=CARTESIAN_POINT ( 'NONE',  ( 115.0540265531850395, 2.143131898507847836E-16, -120.9317124430720156 ) ) ;
#30762=ORIENTED_EDGE ( 'NONE', *, *, #36282, .T. ) ;
#30765=DIRECTION ( 'NONE',  ( 1.000000000000000000, 0.000000000000000000, 0.000000000000000000 ) ) ;
#30766=VERTEX_POINT ( 'NONE', #5521 ) ;
#30768=CARTESIAN_POINT ( 'NONE',  ( -6.695973446814940111, 1.750000000000024203, -119.1817124430720440 ) ) ;
#30771=CYLINDRICAL_SURFACE ( 'NONE', #15680, 1.750000000000001554 ) ;
#30772=CARTESIAN_POINT ( 'NONE',  ( 73.30402655318508209, -1.750000000000010658, 80.81828755692798438 ) ) ;
#30776=CYLINDRICAL_SURFACE ( 'NONE', #16809, 1.750000000000015543 ) ;
#30777=EDGE_CURVE ( 'NONE', #9118, #50130, #16896, .T. ) ;
#30781=VECTOR ( 'NONE', #43946, 1000.000000000000000 ) ;
#30782=VERTEX_POINT ( 'NONE', #1682 ) ;
#30784=CARTESIAN_POINT ( 'NONE',  ( -8.445973446814964092, -1.025126265847097429, -37.43171244307200851 ) ) ;
#30794=AXIS2_PLACEMENT_3D ( 'NONE', #44219, #36056, #638 ) ;
#30796=ORIENTED_EDGE ( 'NONE', *, *, #14065, .F. ) ;
#30802=VECTOR ( 'NONE', #34631, 1000.000000000000000 ) ;
#30803=ORIENTED_EDGE ( 'NONE', *, *, #28107, .T. ) ;
#30804=CARTESIAN_POINT ( 'NONE',  ( 155.0540265531850537, 1.025126265847089435, 159.0682875569279418 ) ) ;
#30808=ORIENTED_EDGE ( 'NONE', *, *, #16083, .T. ) ;
#30813=DIRECTION ( 'NONE',  ( -1.000000000000000000, -0.000000000000000000, -0.000000000000000000 ) ) ;
#30816=DIRECTION ( 'NONE',  ( -1.000000000000000000, -0.000000000000000000, -0.000000000000000000 ) ) ;
#30819=( BOUNDED_CURVE ( )  B_SPLINE_CURVE ( 3, ( #44278, #5551, #47607, #1468 ),
 .UNSPECIFIED., .F., .F. ) 
 B_SPLINE_CURVE_WITH_KNOTS ( ( 4, 4 ),
 ( 0.000000000000000000, 1.570796326794896558 ),
 .UNSPECIFIED. ) 
 CURVE ( )  GEOMETRIC_REPRESENTATION_ITEM ( )  RATIONAL_B_SPLINE_CURVE ( ( 1.000000000000000000, 0.8047378541243649375, 0.8047378541243649375, 1.000000000000000000 ) ) 
 REPRESENTATION_ITEM ( '' )  );
#30825=( BOUNDED_CURVE ( )  B_SPLINE_CURVE ( 3, ( #3993, #14782, #10928, #26586 ),
 .UNSPECIFIED., .F., .F. ) 
 B_SPLINE_CURVE_WITH_KNOTS ( ( 4, 4 ),
 ( 1.570796326794896558, 3.141592653589793116 ),
 .UNSPECIFIED. ) 
 CURVE ( )  GEOMETRIC_REPRESENTATION_ITEM ( )  RATIONAL_B_SPLINE_CURVE ( ( 1.000000000000000000, 0.8047378541243649375, 0.8047378541243649375, 1.000000000000000000 ) ) 
 REPRESENTATION_ITEM ( '' )  );
#30829=CARTESIAN_POINT ( 'NONE',  ( 192.2789002873380184, 1.750000000000009548, -160.2068387089191219 ) ) ;
#30831=LINE ( 'NONE', #34183, #44372 ) ;
#30832=VECTOR ( 'NONE', #34665, 1000.000000000000000 ) ;
#30834=EDGE_LOOP ( 'NONE', ( #3013, #18921 ) ) ;
#30836=AXIS2_PLACEMENT_3D ( 'NONE', #3930, #19572, #40108 ) ;
#30839=( BOUNDED_CURVE ( )  B_SPLINE_CURVE ( 3, ( #1793, #5884, #28488, #5627 ),
 .UNSPECIFIED., .F., .F. ) 
 B_SPLINE_CURVE_WITH_KNOTS ( ( 4, 4 ),
 ( 4.712388980384689674, 6.283185307179586232 ),
 .UNSPECIFIED. ) 
 CURVE ( )  GEOMETRIC_REPRESENTATION_ITEM ( )  RATIONAL_B_SPLINE_CURVE ( ( 1.000000000000000000, 0.8047378541243649375, 0.8047378541243649375, 1.000000000000000000 ) ) 
 REPRESENTATION_ITEM ( '' )  );
#30841=ORIENTED_EDGE ( 'NONE', *, *, #36336, .T. ) ;
#30846=CARTESIAN_POINT ( 'NONE',  ( -125.6708471809678542, -1.749999999999996669, 81.84341382277506227 ) ) ;
#30847=VECTOR ( 'NONE', #15791, 1000.000000000000000 ) ;
#30848=CARTESIAN_POINT ( 'NONE',  ( -125.6708471809678542, -1.749999999999996891, -40.20683870891911482 ) ) ;
#30850=LINE ( 'NONE', #26982, #6134 ) ;
#30852=ORIENTED_EDGE ( 'NONE', *, *, #44739, .T. ) ;
#30857=CARTESIAN_POINT ( 'NONE',  ( 115.0540265531850395, 2.143131898507847836E-16, -40.93171244307202983 ) ) ;
#30863=CARTESIAN_POINT ( 'NONE',  ( 210.0000000000000568, 2.143131898507880377E-16, -0.9317124430720331585 ) ) ;
#30864=VERTEX_POINT ( 'NONE', #15494 ) ;
#30865=DIRECTION ( 'NONE',  ( -0.000000000000000000, -0.000000000000000000, -1.000000000000000000 ) ) ;
#30870=VERTEX_POINT ( 'NONE', #42178 ) ;
#30875=CARTESIAN_POINT ( 'NONE',  ( 35.05402655318504657, 1.025126265847089435, -40.93171244307204404 ) ) ;
#30880=EDGE_CURVE ( 'NONE', #39755, #24104, #41456, .T. ) ;
#30885=CARTESIAN_POINT ( 'NONE',  ( -166.6959734468149463, 0.000000000000000000, -165.0000000000000000 ) ) ;
#30887=VERTEX_POINT ( 'NONE', #11392 ) ;
#30890=CARTESIAN_POINT ( 'NONE',  ( -88.44597344681497475, 0.000000000000000000, 119.0682875569279418 ) ) ;
#30893=ORIENTED_EDGE ( 'NONE', *, *, #48338, .F. ) ;
#30895=EDGE_CURVE ( 'NONE', #25557, #24452, #17484, .T. ) ;
#30899=EDGE_CURVE ( 'NONE', #10372, #5041, #1754, .T. ) ;
#30901=EDGE_CURVE ( 'NONE', #7812, #32944, #22724, .T. ) ;
#30902=ORIENTED_EDGE ( 'NONE', *, *, #23146, .T. ) ;
#30904=CARTESIAN_POINT ( 'NONE',  ( -7.721099712662037540, 1.750000000000023315, 161.8434138227750907 ) ) ;
#30905=CARTESIAN_POINT ( 'NONE',  ( -6.695973446814940111, 1.750000000000024203, -79.18171244307201562 ) ) ;
#30906=EDGE_CURVE ( 'NONE', #34157, #30766, #43700, .T. ) ;
#30912=FACE_OUTER_BOUND ( 'NONE', #34380, .T. ) ;
#30915=LINE ( 'NONE', #39123, #8034 ) ;
#30923=CARTESIAN_POINT ( 'NONE',  ( -126.6959734468149321, -1.749999999999997335, 80.81828755692798438 ) ) ;
#30924=CARTESIAN_POINT ( 'NONE',  ( -168.4459734468149747, 0.000000000000000000, 162.5682875569279702 ) ) ;
#30925=CARTESIAN_POINT ( 'NONE',  ( -84.94597344681494633, 2.143131898507880377E-16, 165.0000000000000000 ) ) ;
#30928=( BOUNDED_CURVE ( )  B_SPLINE_CURVE ( 3, ( #19258, #34949, #31605, #20284 ),
 .UNSPECIFIED., .F., .F. ) 
 B_SPLINE_CURVE_WITH_KNOTS ( ( 4, 4 ),
 ( 3.141592653589793116, 4.712388980384689674 ),
 .UNSPECIFIED. ) 
 CURVE ( )  GEOMETRIC_REPRESENTATION_ITEM ( )  RATIONAL_B_SPLINE_CURVE ( ( 1.000000000000000000, 0.8047378541243649375, 0.8047378541243649375, 1.000000000000000000 ) ) 
 REPRESENTATION_ITEM ( '' )  );
#30929=ADVANCED_FACE ( 'NONE', ( #43447 ), #4951, .F. ) ;
#30931=ORIENTED_EDGE ( 'NONE', *, *, #2896, .T. ) ;
#30934=ORIENTED_EDGE ( 'NONE', *, *, #43209, .F. ) ;
#30935=EDGE_CURVE ( 'NONE', #14506, #3878, #12901, .T. ) ;
#30937=CARTESIAN_POINT ( 'NONE',  ( -166.6959734468149463, 0.000000000000000000, 165.0000000000000000 ) ) ;
#30938=CARTESIAN_POINT ( 'NONE',  ( 153.3040265531850537, -1.750000000000010658, 120.8182875569279702 ) ) ;
#30940=CARTESIAN_POINT ( 'NONE',  ( -88.44597344681497475, 0.000000000000000000, 39.06828755692795596 ) ) ;
#30952=ORIENTED_EDGE ( 'NONE', *, *, #49111, .T. ) ;
#30965=DIRECTION ( 'NONE',  ( 0.000000000000000000, 0.000000000000000000, 1.000000000000000000 ) ) ;
#30974=CARTESIAN_POINT ( 'NONE',  ( 153.3040265531850537, -1.750000000000010214, -39.18171244307202983 ) ) ;
#30977=CARTESIAN_POINT ( 'NONE',  ( 71.55402655318505367, 0.000000000000000000, 165.0000000000000000 ) ) ;
#30981=( BOUNDED_CURVE ( )  B_SPLINE_CURVE ( 3, ( #41660, #22161, #17303, #25254 ),
 .UNSPECIFIED., .F., .F. ) 
 B_SPLINE_CURVE_WITH_KNOTS ( ( 4, 4 ),
 ( 0.000000000000000000, 1.570796326794896558 ),
 .UNSPECIFIED. ) 
 CURVE ( )  GEOMETRIC_REPRESENTATION_ITEM ( )  RATIONAL_B_SPLINE_CURVE ( ( 1.000000000000000000, 0.8047378541243649375, 0.8047378541243649375, 1.000000000000000000 ) ) 
 REPRESENTATION_ITEM ( '' )  );
#30985=( BOUNDED_CURVE ( )  B_SPLINE_CURVE ( 3, ( #8636, #40184, #24534, #44503 ),
 .UNSPECIFIED., .F., .F. ) 
 B_SPLINE_CURVE_WITH_KNOTS ( ( 4, 4 ),
 ( 1.570796326794896558, 3.141592653589793116 ),
 .UNSPECIFIED. ) 
 CURVE ( )  GEOMETRIC_REPRESENTATION_ITEM ( )  RATIONAL_B_SPLINE_CURVE ( ( 1.000000000000000000, 0.8047378541243649375, 0.8047378541243649375, 1.000000000000000000 ) ) 
 REPRESENTATION_ITEM ( '' )  );
#30991=CARTESIAN_POINT ( 'NONE',  ( 72.27890028733797578, -1.750000000000009548, -0.2068387089191121020 ) ) ;
#30992=ORIENTED_EDGE ( 'NONE', *, *, #38681, .F. ) ;
#30997=ADVANCED_FACE ( 'NONE', ( #9568 ), #45436, .T. ) ;
#30998=EDGE_LOOP ( 'NONE', ( #10376, #22029, #28835, #12394, #50494 ) ) ;
#31006=ORIENTED_EDGE ( 'NONE', *, *, #24668, .F. ) ;
#31007=CARTESIAN_POINT ( 'NONE',  ( 210.0000000000000568, 0.000000000000000000, -77.43171244307200141 ) ) ;
#31008=DIRECTION ( 'NONE',  ( -1.000000000000000000, -0.000000000000000000, -0.000000000000000000 ) ) ;
#31015=ORIENTED_EDGE ( 'NONE', *, *, #20884, .T. ) ;
#31016=CYLINDRICAL_SURFACE ( 'NONE', #3824, 1.750000000000015543 ) ;
#31029=CARTESIAN_POINT ( 'NONE',  ( 31.55402655318503236, 0.000000000000000000, -37.43171244307200141 ) ) ;
#31030=CARTESIAN_POINT ( 'NONE',  ( -206.6959734468149463, 1.750000000000010658, -79.18171244307201562 ) ) ;
#31038=CARTESIAN_POINT ( 'NONE',  ( -210.0000000000000568, 0.000000000000000000, 0.8182875569279768335 ) ) ;
#31046=AXIS2_PLACEMENT_3D ( 'NONE', #3755, #8126, #31473 ) ;
#31049=VERTEX_POINT ( 'NONE', #9314 ) ;
#31051=ORIENTED_EDGE ( 'NONE', *, *, #40472, .F. ) ;
#31058=EDGE_CURVE ( 'NONE', #24452, #27194, #40864, .T. ) ;
#31060=DIRECTION ( 'NONE',  ( -0.000000000000000000, -0.000000000000000000, -1.000000000000000000 ) ) ;
#31061=DIRECTION ( 'NONE',  ( 1.000000000000000000, 0.000000000000000000, 0.000000000000000000 ) ) ;
#31065=ADVANCED_FACE ( 'NONE', ( #48774 ), #29825, .T. ) ;
#31066=ORIENTED_EDGE ( 'NONE', *, *, #47279, .T. ) ;
#31067=CARTESIAN_POINT ( 'NONE',  ( 210.0000000000000568, 0.000000000000000000, 162.5682875569279702 ) ) ;
#31072=ORIENTED_EDGE ( 'NONE', *, *, #27876, .F. ) ;
#31076=LINE ( 'NONE', #43361, #33296 ) ;
#31077=AXIS2_PLACEMENT_3D ( 'NONE', #34718, #31368, #38815 ) ;
#31078=CARTESIAN_POINT ( 'NONE',  ( 71.55402655318505367, 0.000000000000000000, 159.0682875569279702 ) ) ;
#31079=CARTESIAN_POINT ( 'NONE',  ( -86.69597344681494633, 1.750000000000009992, 160.8182875569279702 ) ) ;
#31084=VECTOR ( 'NONE', #3530, 1000.000000000000000 ) ;
#31085=AXIS2_PLACEMENT_3D ( 'NONE', #22819, #38500, #3313 ) ;
#31087=ORIENTED_EDGE ( 'NONE', *, *, #6372, .F. ) ;
#31093=DIRECTION ( 'NONE',  ( -1.000000000000000000, -0.000000000000000000, -0.000000000000000000 ) ) ;
#31094=CARTESIAN_POINT ( 'NONE',  ( 31.55402655318503236, 1.025126265847089435, -40.93171244307204404 ) ) ;
#31100=CARTESIAN_POINT ( 'NONE',  ( -206.6959734468149463, 1.750000000000010658, 80.81828755692798438 ) ) ;
#31103=ORIENTED_EDGE ( 'NONE', *, *, #40374, .T. ) ;
#31106=CYLINDRICAL_SURFACE ( 'NONE', #28733, 1.750000000000008438 ) ;
#31110=ORIENTED_EDGE ( 'NONE', *, *, #19676, .F. ) ;
#31112=( BOUNDED_CURVE ( )  B_SPLINE_CURVE ( 3, ( #4804, #32787, #21219, #44297 ),
 .UNSPECIFIED., .F., .F. ) 
 B_SPLINE_CURVE_WITH_KNOTS ( ( 4, 4 ),
 ( 4.712388980384689674, 6.283185307179586232 ),
 .UNSPECIFIED. ) 
 CURVE ( )  GEOMETRIC_REPRESENTATION_ITEM ( )  RATIONAL_B_SPLINE_CURVE ( ( 1.000000000000000000, 0.8047378541243649375, 0.8047378541243649375, 1.000000000000000000 ) ) 
 REPRESENTATION_ITEM ( '' )  );
#31114=CARTESIAN_POINT ( 'NONE',  ( 210.0000000000000568, 0.000000000000000000, 160.8182875569279702 ) ) ;
#31115=CARTESIAN_POINT ( 'NONE',  ( 34.32915281903212446, 1.750000000000009548, -40.20683870891912193 ) ) ;
#31118=DIRECTION ( 'NONE',  ( -0.000000000000000000, -0.000000000000000000, -1.000000000000000000 ) ) ;
#31120=DIRECTION ( 'NONE',  ( -0.000000000000000000, -0.000000000000000000, -1.000000000000000000 ) ) ;
#31122=CIRCLE ( 'NONE', #840, 1.750000000000001554 ) ;
#31123=( BOUNDED_CURVE ( )  B_SPLINE_CURVE ( 3, ( #23057, #23314, #38988, #15377 ),
 .UNSPECIFIED., .F., .F. ) 
 B_SPLINE_CURVE_WITH_KNOTS ( ( 4, 4 ),
 ( 0.000000000000000000, 1.570796326794896558 ),
 .UNSPECIFIED. ) 
 CURVE ( )  GEOMETRIC_REPRESENTATION_ITEM ( )  RATIONAL_B_SPLINE_CURVE ( ( 1.000000000000000000, 0.8047378541243649375, 0.8047378541243649375, 1.000000000000000000 ) ) 
 REPRESENTATION_ITEM ( '' )  );
#31129=ORIENTED_EDGE ( 'NONE', *, *, #2659, .F. ) ;
#31130=ORIENTED_EDGE ( 'NONE', *, *, #25699, .F. ) ;
#31136=ORIENTED_EDGE ( 'NONE', *, *, #28494, .F. ) ;
#31137=ADVANCED_FACE ( 'NONE', ( #10332 ), #25984, .T. ) ;
#31138=( BOUNDED_CURVE ( )  B_SPLINE_CURVE ( 3, ( #4403, #50539, #3890, #28001 ),
 .UNSPECIFIED., .F., .F. ) 
 B_SPLINE_CURVE_WITH_KNOTS ( ( 4, 4 ),
 ( 1.570796326794896558, 3.141592653589793116 ),
 .UNSPECIFIED. ) 
 CURVE ( )  GEOMETRIC_REPRESENTATION_ITEM ( )  RATIONAL_B_SPLINE_CURVE ( ( 1.000000000000000000, 0.8047378541243649375, 0.8047378541243649375, 1.000000000000000000 ) ) 
 REPRESENTATION_ITEM ( '' )  );
#31140=EDGE_CURVE ( 'NONE', #18060, #10849, #6229, .T. ) ;
#31145=ORIENTED_EDGE ( 'NONE', *, *, #42484, .T. ) ;
#31147=DIRECTION ( 'NONE',  ( -1.000000000000000000, -0.000000000000000000, -0.000000000000000000 ) ) ;
#31148=CARTESIAN_POINT ( 'NONE',  ( 191.5540265531850537, -1.025126265847089213, 162.5682875569279133 ) ) ;
#31150=ORIENTED_EDGE ( 'NONE', *, *, #19095, .T. ) ;
#31152=EDGE_CURVE ( 'NONE', #44363, #29337, #29067, .T. ) ;
#31153=ADVANCED_FACE ( 'NONE', ( #2126 ), #49012, .T. ) ;
#31158=ORIENTED_EDGE ( 'NONE', *, *, #46143, .F. ) ;
#31160=CARTESIAN_POINT ( 'NONE',  ( -48.44597344681495343, 0.000000000000000000, 82.56828755692798438 ) ) ;
#31162=LINE ( 'NONE', #43202, #17675 ) ;
#31165=ORIENTED_EDGE ( 'NONE', *, *, #4981, .F. ) ;
#31168=AXIS2_PLACEMENT_3D ( 'NONE', #35894, #8433, #24086 ) ;
#31169=CARTESIAN_POINT ( 'NONE',  ( 31.55402655318506788, 2.143131898507880377E-16, -160.9317124430720298 ) ) ;
#31170=CARTESIAN_POINT ( 'NONE',  ( -206.6959734468149463, 0.000000000000000000, 165.0000000000000000 ) ) ;
#31172=VECTOR ( 'NONE', #46213, 1000.000000000000000 ) ;
#31178=CARTESIAN_POINT ( 'NONE',  ( 210.0000000000000568, 0.000000000000000000, -119.1817124430720440 ) ) ;
#31186=EDGE_CURVE ( 'NONE', #45850, #46718, #3383, .T. ) ;
#31188=ORIENTED_EDGE ( 'NONE', *, *, #42484, .F. ) ;
#31190=EDGE_CURVE ( 'NONE', #33167, #28808, #16136, .T. ) ;
#31197=CARTESIAN_POINT ( 'NONE',  ( 113.3040265531850537, -1.749999999999997113, 40.81828755692798438 ) ) ;
#31204=CARTESIAN_POINT ( 'NONE',  ( 111.5540265531850537, -1.025126265847082108, -37.43171244307203693 ) ) ;
#31211=ORIENTED_EDGE ( 'NONE', *, *, #22080, .F. ) ;
#31212=CARTESIAN_POINT ( 'NONE',  ( 35.05402655318504657, 1.025126265847089657, -37.43171244307202272 ) ) ;
#31215=ORIENTED_EDGE ( 'NONE', *, *, #37764, .T. ) ;
#31218=ORIENTED_EDGE ( 'NONE', *, *, #44670, .T. ) ;
#31220=CARTESIAN_POINT ( 'NONE',  ( -124.9459734468149463, 2.143131898507847836E-16, 79.06828755692798438 ) ) ;
#31223=DIRECTION ( 'NONE',  ( 0.000000000000000000, 0.000000000000000000, 1.000000000000000000 ) ) ;
#31224=CARTESIAN_POINT ( 'NONE',  ( -48.44597344681495343, 0.000000000000000000, -0.9317124430720247208 ) ) ;
#31231=ADVANCED_FACE ( 'NONE', ( #19974 ), #31799, .T. ) ;
#31235=CARTESIAN_POINT ( 'NONE',  ( -88.44597344681497475, 0.000000000000000000, -77.43171244307198720 ) ) ;
#31237=ORIENTED_EDGE ( 'NONE', *, *, #29341, .T. ) ;
#31242=CARTESIAN_POINT ( 'NONE',  ( -164.9459734468149463, 2.143131898507880377E-16, 165.0000000000000000 ) ) ;
#31245=CARTESIAN_POINT ( 'NONE',  ( -166.6959734468149463, 1.750000000000010658, 120.8182875569279702 ) ) ;
#31253=ORIENTED_EDGE ( 'NONE', *, *, #10622, .F. ) ;
#31258=CARTESIAN_POINT ( 'NONE',  ( -124.9459734468149463, 2.143131898507847836E-16, 122.5682875569279560 ) ) ;
#31259=CARTESIAN_POINT ( 'NONE',  ( -128.4459734468149463, 1.025126265847081442, 162.5682875569279133 ) ) ;
#31263=ORIENTED_EDGE ( 'NONE', *, *, #6529, .F. ) ;
#31264=AXIS2_PLACEMENT_3D ( 'NONE', #44063, #32043, #15875 ) ;
#31271=ORIENTED_EDGE ( 'NONE', *, *, #34700, .F. ) ;
#31272=EDGE_CURVE ( 'NONE', #16751, #45714, #20994, .T. ) ;
#31276=AXIS2_PLACEMENT_3D ( 'NONE', #38178, #34311, #38936 ) ;
#31281=CARTESIAN_POINT ( 'NONE',  ( -165.6708471809677974, -1.750000000000009548, -78.15658617722490931 ) ) ;
#31284=( BOUNDED_CURVE ( )  B_SPLINE_CURVE ( 3, ( #49270, #6716, #25727, #49768 ),
 .UNSPECIFIED., .F., .F. ) 
 B_SPLINE_CURVE_WITH_KNOTS ( ( 4, 4 ),
 ( 0.000000000000000000, 1.570796326794896558 ),
 .UNSPECIFIED. ) 
 CURVE ( )  GEOMETRIC_REPRESENTATION_ITEM ( )  RATIONAL_B_SPLINE_CURVE ( ( 1.000000000000000000, 0.8047378541243649375, 0.8047378541243649375, 1.000000000000000000 ) ) 
 REPRESENTATION_ITEM ( '' )  );
#31286=CARTESIAN_POINT ( 'NONE',  ( 31.55402655318503236, 0.000000000000000000, -80.93171244307204404 ) ) ;
#31288=EDGE_CURVE ( 'NONE', #10041, #44104, #12147, .T. ) ;
#31289=DIRECTION ( 'NONE',  ( -0.000000000000000000, -0.000000000000000000, -1.000000000000000000 ) ) ;
#31291=( BOUNDED_CURVE ( )  B_SPLINE_CURVE ( 3, ( #23308, #11771, #42797, #50464 ),
 .UNSPECIFIED., .F., .F. ) 
 B_SPLINE_CURVE_WITH_KNOTS ( ( 4, 4 ),
 ( 3.141592653589793116, 4.712388980384689674 ),
 .UNSPECIFIED. ) 
 CURVE ( )  GEOMETRIC_REPRESENTATION_ITEM ( )  RATIONAL_B_SPLINE_CURVE ( ( 1.000000000000000000, 0.8047378541243649375, 0.8047378541243649375, 1.000000000000000000 ) ) 
 REPRESENTATION_ITEM ( '' )  );
#31292=EDGE_CURVE ( 'NONE', #27788, #12513, #8657, .T. ) ;
#31306=LINE ( 'NONE', #31559, #47114 ) ;
#31314=CARTESIAN_POINT ( 'NONE',  ( 153.3040265531850537, -1.750000000000010214, 40.81828755692798438 ) ) ;
#31320=CARTESIAN_POINT ( 'NONE',  ( -85.67084718096784002, 1.750000000000009548, -38.15658617722494483 ) ) ;
#31321=CARTESIAN_POINT ( 'NONE',  ( -204.9459734468148895, 1.025126265847089435, 39.06828755692797728 ) ) ;
#31326=ORIENTED_EDGE ( 'NONE', *, *, #50337, .F. ) ;
#31335=CARTESIAN_POINT ( 'NONE',  ( 210.0000000000000568, 0.000000000000000000, -39.18171244307202983 ) ) ;
#31338=ORIENTED_EDGE ( 'NONE', *, *, #28164, .F. ) ;
#31341=CARTESIAN_POINT ( 'NONE',  ( 155.0540265531850537, -1.025126265847089435, -117.4317124430720156 ) ) ;
#31342=CARTESIAN_POINT ( 'NONE',  ( -4.945973446814903696, 2.143131898507912917E-16, 39.06828755692792754 ) ) ;
#31346=ORIENTED_EDGE ( 'NONE', *, *, #12723, .T. ) ;
#31350=ORIENTED_EDGE ( 'NONE', *, *, #15466, .F. ) ;
#31352=EDGE_CURVE ( 'NONE', #19994, #21654, #28448, .T. ) ;
#31357=DIRECTION ( 'NONE',  ( -0.000000000000000000, -0.000000000000000000, -1.000000000000000000 ) ) ;
#31359=ORIENTED_EDGE ( 'NONE', *, *, #28142, .T. ) ;
#31360=ADVANCED_FACE ( 'NONE', ( #14542 ), #41746, .T. ) ;
#31363=CARTESIAN_POINT ( 'NONE',  ( -166.6959734468149463, 0.000000000000000000, -165.0000000000000000 ) ) ;
#31364=( NAMED_UNIT ( * ) PLANE_ANGLE_UNIT ( ) SI_UNIT ( $, .RADIAN. ) );
#31366=DIRECTION ( 'NONE',  ( -0.000000000000000000, -0.000000000000000000, -1.000000000000000000 ) ) ;
#31368=DIRECTION ( 'NONE',  ( 0.000000000000000000, 0.000000000000000000, 1.000000000000000000 ) ) ;
#31376=CYLINDRICAL_SURFACE ( 'NONE', #14031, 1.750000000000015543 ) ;
#31379=CARTESIAN_POINT ( 'NONE',  ( -166.6959734468149463, -1.750000000000010658, -79.18171244307201562 ) ) ;
#31380=VECTOR ( 'NONE', #35969, 1000.000000000000000 ) ;
#31382=ORIENTED_EDGE ( 'NONE', *, *, #41987, .F. ) ;
#31383=CARTESIAN_POINT ( 'NONE',  ( -207.7210997126620384, 1.750000000000009548, -38.15658617722494483 ) ) ;
#31385=CARTESIAN_POINT ( 'NONE',  ( 153.3040265531850537, -1.750000000000010658, -79.18171244307201562 ) ) ;
#31388=ORIENTED_EDGE ( 'NONE', *, *, #18036, .F. ) ;
#31389=DIRECTION ( 'NONE',  ( 1.000000000000000000, 0.000000000000000000, 0.000000000000000000 ) ) ;
#31393=CARTESIAN_POINT ( 'NONE',  ( -207.7210997126620384, -1.750000000000010214, -120.2068387089191219 ) ) ;
#31394=VECTOR ( 'NONE', #47579, 1000.000000000000000 ) ;
#31405=ORIENTED_EDGE ( 'NONE', *, *, #4837, .F. ) ;
#31407=CARTESIAN_POINT ( 'NONE',  ( 192.2789002873380184, -1.750000000000009548, 161.8434138227750907 ) ) ;
#31409=CARTESIAN_POINT ( 'NONE',  ( 33.30402655318503946, 0.000000000000000000, 165.0000000000000000 ) ) ;
#31411=CARTESIAN_POINT ( 'NONE',  ( 193.3040265531851105, 0.000000000000000000, -165.0000000000000000 ) ) ;
#31421=ORIENTED_EDGE ( 'NONE', *, *, #39084, .F. ) ;
#31428=( BOUNDED_CURVE ( )  B_SPLINE_CURVE ( 3, ( #29608, #5306, #705, #27914 ),
 .UNSPECIFIED., .F., .F. ) 
 B_SPLINE_CURVE_WITH_KNOTS ( ( 4, 4 ),
 ( 1.570796326794896558, 3.141592653589793116 ),
 .UNSPECIFIED. ) 
 CURVE ( )  GEOMETRIC_REPRESENTATION_ITEM ( )  RATIONAL_B_SPLINE_CURVE ( ( 1.000000000000000000, 0.8047378541243649375, 0.8047378541243649375, 1.000000000000000000 ) ) 
 REPRESENTATION_ITEM ( '' )  );
#31431=ORIENTED_EDGE ( 'NONE', *, *, #48136, .F. ) ;
#31433=( BOUNDED_CURVE ( )  B_SPLINE_CURVE ( 3, ( #24671, #8263, #1327, #12859 ),
 .UNSPECIFIED., .F., .F. ) 
 B_SPLINE_CURVE_WITH_KNOTS ( ( 4, 4 ),
 ( 4.712388980384689674, 6.283185307179586232 ),
 .UNSPECIFIED. ) 
 CURVE ( )  GEOMETRIC_REPRESENTATION_ITEM ( )  RATIONAL_B_SPLINE_CURVE ( ( 1.000000000000000000, 0.8047378541243649375, 0.8047378541243649375, 1.000000000000000000 ) ) 
 REPRESENTATION_ITEM ( '' )  );
#31440=( BOUNDED_CURVE ( )  B_SPLINE_CURVE ( 3, ( #35782, #361, #36021, #31671 ),
 .UNSPECIFIED., .F., .F. ) 
 B_SPLINE_CURVE_WITH_KNOTS ( ( 4, 4 ),
 ( 3.141592653589793116, 4.712388980384689674 ),
 .UNSPECIFIED. ) 
 CURVE ( )  GEOMETRIC_REPRESENTATION_ITEM ( )  RATIONAL_B_SPLINE_CURVE ( ( 1.000000000000000000, 0.8047378541243649375, 0.8047378541243649375, 1.000000000000000000 ) ) 
 REPRESENTATION_ITEM ( '' )  );
#31441=ORIENTED_EDGE ( 'NONE', *, *, #39696, .T. ) ;
#31444=CYLINDRICAL_SURFACE ( 'NONE', #17297, 1.750000000000015543 ) ;
#31447=CARTESIAN_POINT ( 'NONE',  ( 210.0000000000000568, 0.000000000000000000, 42.56828755692799149 ) ) ;
#31450=CARTESIAN_POINT ( 'NONE',  ( 71.55402655318505367, 0.000000000000000000, 165.0000000000000000 ) ) ;
#31451=ORIENTED_EDGE ( 'NONE', *, *, #48672, .F. ) ;
#31452=EDGE_LOOP ( 'NONE', ( #36195, #36000, #5518, #42908, #14969, #49632 ) ) ;
#31460=ORIENTED_EDGE ( 'NONE', *, *, #45266, .F. ) ;
#31461=ORIENTED_EDGE ( 'NONE', *, *, #37839, .T. ) ;
#31464=FACE_OUTER_BOUND ( 'NONE', #5736, .T. ) ;
#31465=ORIENTED_EDGE ( 'NONE', *, *, #19941, .F. ) ;
#31468=DIRECTION ( 'NONE',  ( 0.000000000000000000, 0.000000000000000000, -1.000000000000000000 ) ) ;
#31470=VERTEX_POINT ( 'NONE', #29954 ) ;
#31471=CARTESIAN_POINT ( 'NONE',  ( -85.67084718096784002, -1.750000000000009548, 121.8434138227750623 ) ) ;
#31473=DIRECTION ( 'NONE',  ( 0.000000000000000000, 0.000000000000000000, -1.000000000000000000 ) ) ;
#31474=EDGE_CURVE ( 'NONE', #14709, #16946, #17186, .T. ) ;
#31482=CARTESIAN_POINT ( 'NONE',  ( 210.0000000000000568, 0.000000000000000000, -117.4317124430720298 ) ) ;
#31488=EDGE_LOOP ( 'NONE', ( #5223, #35722, #31072, #21029, #31158, #27870 ) ) ;
#31490=EDGE_CURVE ( 'NONE', #23447, #38145, #19118, .T. ) ;
#31493=ORIENTED_EDGE ( 'NONE', *, *, #2002, .T. ) ;
#31496=CARTESIAN_POINT ( 'NONE',  ( 71.55402655318505367, -1.025126265847089213, -0.9317124430720324924 ) ) ;
#31500=CARTESIAN_POINT ( 'NONE',  ( -88.44597344681494633, 1.025126265847089213, 42.56828755692799149 ) ) ;
#31511=VERTEX_POINT ( 'NONE', #21995 ) ;
#31513=CARTESIAN_POINT ( 'NONE',  ( -128.4459734468149179, 0.000000000000000000, 162.5682875569279702 ) ) ;
#31516=VECTOR ( 'NONE', #35679, 1000.000000000000000 ) ;
#31517=EDGE_CURVE ( 'NONE', #19548, #8682, #39837, .T. ) ;
#31526=FACE_OUTER_BOUND ( 'NONE', #13941, .T. ) ;
#31527=CARTESIAN_POINT ( 'NONE',  ( 74.32915281903215998, 1.750000000000010214, 121.8434138227750623 ) ) ;
#31528=ORIENTED_EDGE ( 'NONE', *, *, #23641, .T. ) ;
#31538=VECTOR ( 'NONE', #37550, 1000.000000000000000 ) ;
#31539=EDGE_CURVE ( 'NONE', #20559, #16655, #10295, .T. ) ;
#31548=CARTESIAN_POINT ( 'NONE',  ( 34.32915281903212446, 1.750000000000010214, 119.7931612910808781 ) ) ;
#31559=CARTESIAN_POINT ( 'NONE',  ( 210.0000000000000568, 0.000000000000000000, 42.56828755692799149 ) ) ;
#31560=VECTOR ( 'NONE', #45112, 1000.000000000000000 ) ;
#31569=CARTESIAN_POINT ( 'NONE',  ( 154.3291528190321458, -1.750000000000009548, -160.2068387089191219 ) ) ;
#31570=CARTESIAN_POINT ( 'NONE',  ( -44.94597344681493922, 2.143131898507880377E-16, 165.0000000000000000 ) ) ;
#31572=CARTESIAN_POINT ( 'NONE',  ( 210.0000000000000568, 2.143131898507880377E-16, 159.0682875569279702 ) ) ;
#31576=ADVANCED_FACE ( 'NONE', ( #8135 ), #19666, .T. ) ;
#31577=ORIENTED_EDGE ( 'NONE', *, *, #20245, .T. ) ;
#31579=CYLINDRICAL_SURFACE ( 'NONE', #15049, 1.750000000000015543 ) ;
#31583=CARTESIAN_POINT ( 'NONE',  ( -126.6959734468149321, -1.749999999999997335, 120.8182875569279702 ) ) ;
#31592=AXIS2_PLACEMENT_3D ( 'NONE', #16108, #20209, #31773 ) ;
#31593=FACE_OUTER_BOUND ( 'NONE', #46812, .T. ) ;
#31596=FACE_OUTER_BOUND ( 'NONE', #11711, .T. ) ;
#31597=( BOUNDED_CURVE ( )  B_SPLINE_CURVE ( 3, ( #44728, #5498, #21148, #10103 ),
 .UNSPECIFIED., .F., .F. ) 
 B_SPLINE_CURVE_WITH_KNOTS ( ( 4, 4 ),
 ( 0.000000000000000000, 1.570796326794896558 ),
 .UNSPECIFIED. ) 
 CURVE ( )  GEOMETRIC_REPRESENTATION_ITEM ( )  RATIONAL_B_SPLINE_CURVE ( ( 1.000000000000000000, 0.8047378541243649375, 0.8047378541243649375, 1.000000000000000000 ) ) 
 REPRESENTATION_ITEM ( '' )  );
#31599=DIRECTION ( 'NONE',  ( -1.000000000000000000, -0.000000000000000000, -0.000000000000000000 ) ) ;
#31600=VERTEX_POINT ( 'NONE', #46821 ) ;
#31604=CARTESIAN_POINT ( 'NONE',  ( -8.445973446814976526, 0.000000000000000000, -120.9317124430720725 ) ) ;
#31605=CARTESIAN_POINT ( 'NONE',  ( -85.67084718096784002, -1.750000000000009326, 1.843413822775066269 ) ) ;
#31607=VERTEX_POINT ( 'NONE', #7110 ) ;
#31610=DIRECTION ( 'NONE',  ( -1.000000000000000000, 0.000000000000000000, 0.000000000000000000 ) ) ;
#31614=DIRECTION ( 'NONE',  ( 0.000000000000000000, 0.000000000000000000, 1.000000000000000000 ) ) ;
#31616=AXIS2_PLACEMENT_3D ( 'NONE', #40144, #43223, #19619 ) ;
#31622=CARTESIAN_POINT ( 'NONE',  ( -166.6959734468149463, 1.750000000000010658, -79.18171244307201562 ) ) ;
#31624=DIRECTION ( 'NONE',  ( 0.000000000000000000, 0.000000000000000000, 1.000000000000000000 ) ) ;
#31625=ORIENTED_EDGE ( 'NONE', *, *, #36900, .T. ) ;
#31630=ORIENTED_EDGE ( 'NONE', *, *, #32434, .F. ) ;
#31631=FACE_OUTER_BOUND ( 'NONE', #5176, .T. ) ;
#31633=CARTESIAN_POINT ( 'NONE',  ( -84.94597344681493212, 1.025126265847089435, 39.06828755692797728 ) ) ;
#31635=VECTOR ( 'NONE', #24030, 1000.000000000000000 ) ;
#31641=CARTESIAN_POINT ( 'NONE',  ( 151.5540265531850537, 0.000000000000000000, -77.43171244307204404 ) ) ;
#31643=CARTESIAN_POINT ( 'NONE',  ( -208.4459734468149463, 0.000000000000000000, -37.43171244307205825 ) ) ;
#31645=CARTESIAN_POINT ( 'NONE',  ( -204.9459734468148895, -1.025126265847089213, -0.9317124430720324924 ) ) ;
#31646=VERTEX_POINT ( 'NONE', #19913 ) ;
#31651=ADVANCED_FACE ( 'NONE', ( #1444 ), #8873, .T. ) ;
#31652=EDGE_CURVE ( 'NONE', #8676, #10849, #30985, .T. ) ;
#31656=FACE_OUTER_BOUND ( 'NONE', #32329, .T. ) ;
#31658=ORIENTED_EDGE ( 'NONE', *, *, #44072, .F. ) ;
#31661=EDGE_CURVE ( 'NONE', #29268, #48485, #24395, .T. ) ;
#31665=VECTOR ( 'NONE', #43930, 1000.000000000000000 ) ;
#31667=ORIENTED_EDGE ( 'NONE', *, *, #45385, .T. ) ;
#31671=CARTESIAN_POINT ( 'NONE',  ( -86.69597344681494633, -1.750000000000009992, 160.8182875569279702 ) ) ;
#31672=CARTESIAN_POINT ( 'NONE',  ( -166.6959734468149463, 1.750000000000010658, -119.1817124430720440 ) ) ;
#31673=ORIENTED_EDGE ( 'NONE', *, *, #29761, .T. ) ;
#31680=CARTESIAN_POINT ( 'NONE',  ( 35.05402655318504657, 1.025126265847088991, 162.5682875569279133 ) ) ;
#31695=CARTESIAN_POINT ( 'NONE',  ( -165.6708471809677974, 1.750000000000009548, -0.2068387089191121020 ) ) ;
#31700=VECTOR ( 'NONE', #26911, 1000.000000000000000 ) ;
#31702=CARTESIAN_POINT ( 'NONE',  ( -128.4459734468149179, 0.000000000000000000, 119.0682875569279986 ) ) ;
#31704=VERTEX_POINT ( 'NONE', #33003 ) ;
#31709=CARTESIAN_POINT ( 'NONE',  ( 155.0540265531850537, 1.025126265847089657, 79.06828755692797017 ) ) ;
#31716=CARTESIAN_POINT ( 'NONE',  ( 210.0000000000000568, 0.000000000000000000, 0.8182875569279768335 ) ) ;
#31719=EDGE_CURVE ( 'NONE', #42713, #9801, #32736, .T. ) ;
#31720=ORIENTED_EDGE ( 'NONE', *, *, #32170, .T. ) ;
#31722=ORIENTED_EDGE ( 'NONE', *, *, #41446, .F. ) ;
#31727=EDGE_LOOP ( 'NONE', ( #32774, #3340, #3469, #34754, #42117, #4251 ) ) ;
#31728=CARTESIAN_POINT ( 'NONE',  ( -8.445973446814976526, 0.000000000000000000, 165.0000000000000000 ) ) ;
#31730=CARTESIAN_POINT ( 'NONE',  ( 210.0000000000000568, 0.000000000000000000, 82.56828755692799859 ) ) ;
#31736=( BOUNDED_CURVE ( )  B_SPLINE_CURVE ( 3, ( #24043, #43011, #19422, #42748 ),
 .UNSPECIFIED., .F., .F. ) 
 B_SPLINE_CURVE_WITH_KNOTS ( ( 4, 4 ),
 ( 0.000000000000000000, 1.570796326794896558 ),
 .UNSPECIFIED. ) 
 CURVE ( )  GEOMETRIC_REPRESENTATION_ITEM ( )  RATIONAL_B_SPLINE_CURVE ( ( 1.000000000000000000, 0.8047378541243649375, 0.8047378541243649375, 1.000000000000000000 ) ) 
 REPRESENTATION_ITEM ( '' )  );
#31737=CARTESIAN_POINT ( 'NONE',  ( -84.94597344681493212, -1.025126265847089435, 122.5682875569280128 ) ) ;
#31739=CARTESIAN_POINT ( 'NONE',  ( 153.3040265531850537, 0.000000000000000000, 165.0000000000000000 ) ) ;
#31742=( BOUNDED_CURVE ( )  B_SPLINE_CURVE ( 3, ( #4990, #40662, #43732, #48048 ),
 .UNSPECIFIED., .F., .F. ) 
 B_SPLINE_CURVE_WITH_KNOTS ( ( 4, 4 ),
 ( 3.141592653589793116, 4.712388980384689674 ),
 .UNSPECIFIED. ) 
 CURVE ( )  GEOMETRIC_REPRESENTATION_ITEM ( )  RATIONAL_B_SPLINE_CURVE ( ( 1.000000000000000000, 0.8047378541243649375, 0.8047378541243649375, 1.000000000000000000 ) ) 
 REPRESENTATION_ITEM ( '' )  );
#31749=( BOUNDED_CURVE ( )  B_SPLINE_CURVE ( 3, ( #19130, #34820, #27353, #14787 ),
 .UNSPECIFIED., .F., .F. ) 
 B_SPLINE_CURVE_WITH_KNOTS ( ( 4, 4 ),
 ( 0.000000000000000000, 1.570796326794896558 ),
 .UNSPECIFIED. ) 
 CURVE ( )  GEOMETRIC_REPRESENTATION_ITEM ( )  RATIONAL_B_SPLINE_CURVE ( ( 1.000000000000000000, 0.8047378541243649375, 0.8047378541243649375, 1.000000000000000000 ) ) 
 REPRESENTATION_ITEM ( '' )  );
#31753=CARTESIAN_POINT ( 'NONE',  ( 75.05402655318509630, 2.143131898507880377E-16, 165.0000000000000000 ) ) ;
#31762=ORIENTED_EDGE ( 'NONE', *, *, #25498, .F. ) ;
#31764=CARTESIAN_POINT ( 'NONE',  ( -6.695973446814940111, 1.750000000000023315, -159.1817124430720298 ) ) ;
#31765=CARTESIAN_POINT ( 'NONE',  ( 210.0000000000000568, 2.143131898507880377E-16, -0.9317124430720331585 ) ) ;
#31766=ORIENTED_EDGE ( 'NONE', *, *, #21891, .F. ) ;
#31769=ORIENTED_EDGE ( 'NONE', *, *, #27024, .F. ) ;
#31773=DIRECTION ( 'NONE',  ( 0.000000000000000000, 0.000000000000000000, 1.000000000000000000 ) ) ;
#31774=DIRECTION ( 'NONE',  ( -1.000000000000000000, -0.000000000000000000, -0.000000000000000000 ) ) ;
#31775=CARTESIAN_POINT ( 'NONE',  ( 210.0000000000000568, 2.143131898507881856E-16, 119.0682875569279560 ) ) ;
#31777=CARTESIAN_POINT ( 'NONE',  ( 193.3040265531851105, 0.000000000000000000, 165.0000000000000000 ) ) ;
#31780=ORIENTED_EDGE ( 'NONE', *, *, #27518, .T. ) ;
#31786=ORIENTED_EDGE ( 'NONE', *, *, #12073, .F. ) ;
#31791=LINE ( 'NONE', #16626, #27642 ) ;
#31792=CARTESIAN_POINT ( 'NONE',  ( -85.67084718096784002, 1.750000000000009326, 161.8434138227750907 ) ) ;
#31793=VECTOR ( 'NONE', #36287, 1000.000000000000000 ) ;
#31796=CARTESIAN_POINT ( 'NONE',  ( 191.5540265531851105, 0.000000000000000000, -37.43171244307205825 ) ) ;
#31799=CYLINDRICAL_SURFACE ( 'NONE', #9684, 1.750000000000008438 ) ;
#31803=EDGE_CURVE ( 'NONE', #50130, #48877, #13730, .T. ) ;
#31804=CARTESIAN_POINT ( 'NONE',  ( -206.6959734468149463, 1.750000000000010214, -39.18171244307202983 ) ) ;
#31811=CARTESIAN_POINT ( 'NONE',  ( 151.5540265531850537, -1.025126265847089213, 162.5682875569279133 ) ) ;
#31814=ORIENTED_EDGE ( 'NONE', *, *, #40244, .T. ) ;
#31815=FACE_OUTER_BOUND ( 'NONE', #48402, .T. ) ;
#31817=LINE ( 'NONE', #46901, #33642 ) ;
#31821=CARTESIAN_POINT ( 'NONE',  ( -208.4459734468148611, 1.025126265847089213, 159.0682875569279418 ) ) ;
#31827=EDGE_CURVE ( 'NONE', #8241, #23844, #41751, .T. ) ;
#31829=CYLINDRICAL_SURFACE ( 'NONE', #22091, 1.749999999999987566 ) ;
#31830=DIRECTION ( 'NONE',  ( 0.000000000000000000, 0.000000000000000000, 1.000000000000000000 ) ) ;
#31833=CARTESIAN_POINT ( 'NONE',  ( 113.3040265531850537, 1.749999999999997335, -79.18171244307201562 ) ) ;
#31834=EDGE_CURVE ( 'NONE', #19505, #26902, #29330, .T. ) ;
#31835=CARTESIAN_POINT ( 'NONE',  ( 210.0000000000000568, 0.000000000000000000, 0.8182875569279768335 ) ) ;
#31837=ADVANCED_FACE ( 'NONE', ( #2193 ), #34004, .T. ) ;
#31840=CARTESIAN_POINT ( 'NONE',  ( 153.3040265531850537, -1.750000000000010214, -39.18171244307202983 ) ) ;
#31841=CARTESIAN_POINT ( 'NONE',  ( 155.0540265531850537, 2.143131898507880377E-16, 39.06828755692798438 ) ) ;
#31843=CARTESIAN_POINT ( 'NONE',  ( -87.72109971266203843, 1.750000000000009548, -0.2068387089191121020 ) ) ;
#31846=ORIENTED_EDGE ( 'NONE', *, *, #2071, .T. ) ;
#31847=FACE_OUTER_BOUND ( 'NONE', #41519, .T. ) ;
#31848=DIRECTION ( 'NONE',  ( -1.000000000000000000, 0.000000000000000000, 0.000000000000000000 ) ) ;
#31849=CARTESIAN_POINT ( 'NONE',  ( -44.94597344681493922, -1.025126265847089657, -80.93171244307201562 ) ) ;
#31852=EDGE_CURVE ( 'NONE', #7869, #5114, #4797, .T. ) ;
#31859=LINE ( 'NONE', #47453, #11405 ) ;
#31860=CARTESIAN_POINT ( 'NONE',  ( -126.6959734468149321, -1.749999999999997113, -39.18171244307202983 ) ) ;
#31862=ADVANCED_FACE ( 'NONE', ( #33754 ), #10396, .T. ) ;
#31865=LINE ( 'NONE', #8767, #31380 ) ;
#31866=VERTEX_POINT ( 'NONE', #37609 ) ;
#31867=EDGE_CURVE ( 'NONE', #17646, #47659, #22420, .T. ) ;
#31873=FACE_OUTER_BOUND ( 'NONE', #49001, .T. ) ;
#31875=CARTESIAN_POINT ( 'NONE',  ( 193.3040265531851105, 0.000000000000000000, 165.0000000000000000 ) ) ;
#31889=CARTESIAN_POINT ( 'NONE',  ( -125.6708471809678542, 1.749999999999996669, 159.7931612910809065 ) ) ;
#31891=( BOUNDED_CURVE ( )  B_SPLINE_CURVE ( 3, ( #33647, #40335, #37018, #29532 ),
 .UNSPECIFIED., .F., .F. ) 
 B_SPLINE_CURVE_WITH_KNOTS ( ( 4, 4 ),
 ( 3.141592653589793116, 4.712388980384689674 ),
 .UNSPECIFIED. ) 
 CURVE ( )  GEOMETRIC_REPRESENTATION_ITEM ( )  RATIONAL_B_SPLINE_CURVE ( ( 1.000000000000000000, 0.8047378541243649375, 0.8047378541243649375, 1.000000000000000000 ) ) 
 REPRESENTATION_ITEM ( '' )  );
#31892=EDGE_LOOP ( 'NONE', ( #40211, #48758, #6235, #9056, #43806, #49863 ) ) ;
#31903=VECTOR ( 'NONE', #27494, 1000.000000000000000 ) ;
#31908=CARTESIAN_POINT ( 'NONE',  ( 210.0000000000000568, 0.000000000000000000, 2.568287556927987048 ) ) ;
#31913=ORIENTED_EDGE ( 'NONE', *, *, #47710, .T. ) ;
#31919=CARTESIAN_POINT ( 'NONE',  ( -8.445973446814962315, -1.025126265847096985, -0.9317124430720461481 ) ) ;
#31923=CARTESIAN_POINT ( 'NONE',  ( 0.000000000000000000, 0.000000000000000000, 0.000000000000000000 ) ) ;
#31936=FACE_OUTER_BOUND ( 'NONE', #48913, .T. ) ;
#31939=VECTOR ( 'NONE', #48280, 1000.000000000000000 ) ;
#31940=CARTESIAN_POINT ( 'NONE',  ( -4.945973446814903696, 2.143131898507912917E-16, 165.0000000000000000 ) ) ;
#31944=EDGE_CURVE ( 'NONE', #24104, #19505, #9989, .T. ) ;
#31949=CARTESIAN_POINT ( 'NONE',  ( 155.0540265531850537, -1.025126265847089435, 122.5682875569280128 ) ) ;
#31957=DIRECTION ( 'NONE',  ( -1.000000000000000000, 0.000000000000000000, 0.000000000000000000 ) ) ;
#31963=ORIENTED_EDGE ( 'NONE', *, *, #45914, .T. ) ;
#31969=CARTESIAN_POINT ( 'NONE',  ( 71.55402655318505367, 0.000000000000000000, -120.9317124430720725 ) ) ;
#31971=( BOUNDED_CURVE ( )  B_SPLINE_CURVE ( 3, ( #21128, #25231, #9830, #17029 ),
 .UNSPECIFIED., .F., .F. ) 
 B_SPLINE_CURVE_WITH_KNOTS ( ( 4, 4 ),
 ( 3.141592653589793116, 4.712388980384689674 ),
 .UNSPECIFIED. ) 
 CURVE ( )  GEOMETRIC_REPRESENTATION_ITEM ( )  RATIONAL_B_SPLINE_CURVE ( ( 1.000000000000000000, 0.8047378541243649375, 0.8047378541243649375, 1.000000000000000000 ) ) 
 REPRESENTATION_ITEM ( '' )  );
#31973=CARTESIAN_POINT ( 'NONE',  ( -6.695973446814940111, -1.750000000000023315, -159.1817124430720298 ) ) ;
#31979=CARTESIAN_POINT ( 'NONE',  ( 35.05402655318504657, 2.143131898507880377E-16, -157.4317124430720014 ) ) ;
#31980=ORIENTED_EDGE ( 'NONE', *, *, #2614, .F. ) ;
#31981=AXIS2_PLACEMENT_3D ( 'NONE', #19303, #31118, #19551 ) ;
#31982=LINE ( 'NONE', #43755, #30576 ) ;
#31983=CARTESIAN_POINT ( 'NONE',  ( -208.4459734468149463, 0.000000000000000000, 122.5682875569279702 ) ) ;
#31984=CARTESIAN_POINT ( 'NONE',  ( 210.0000000000000568, 0.000000000000000000, 162.5682875569279702 ) ) ;
#31990=CARTESIAN_POINT ( 'NONE',  ( -126.6959734468149321, -1.749999999999996891, 160.8182875569279702 ) ) ;
#31992=ADVANCED_FACE ( 'NONE', ( #46008 ), #19086, .T. ) ;
#31993=CARTESIAN_POINT ( 'NONE',  ( 33.30402655318503946, 1.750000000000009992, 0.8182875569279768335 ) ) ;
#31994=EDGE_CURVE ( 'NONE', #1434, #20980, #15246, .T. ) ;
#31996=CARTESIAN_POINT ( 'NONE',  ( 31.55402655318503236, 1.025126265847089657, 119.0682875569279560 ) ) ;
#32002=VECTOR ( 'NONE', #37503, 1000.000000000000000 ) ;
#32005=CARTESIAN_POINT ( 'NONE',  ( -7.721099712662037540, -1.750000000000023537, -120.2068387089191219 ) ) ;
#32008=DIRECTION ( 'NONE',  ( -1.000000000000000000, -0.000000000000000000, -0.000000000000000000 ) ) ;
#32009=AXIS2_PLACEMENT_3D ( 'NONE', #29496, #37227, #17927 ) ;
#32011=CARTESIAN_POINT ( 'NONE',  ( 194.3291528190321742, 1.750000000000010214, -118.1565861772249519 ) ) ;
#32014=CARTESIAN_POINT ( 'NONE',  ( -8.445973446814962315, 1.025126265847096763, -157.4317124430720014 ) ) ;
#32015=DIRECTION ( 'NONE',  ( -0.000000000000000000, -0.000000000000000000, -1.000000000000000000 ) ) ;
#32017=DIRECTION ( 'NONE',  ( 0.000000000000000000, 0.000000000000000000, 1.000000000000000000 ) ) ;
#32018=DIRECTION ( 'NONE',  ( -1.000000000000000000, 0.000000000000000000, 0.000000000000000000 ) ) ;
#32026=( BOUNDED_CURVE ( )  B_SPLINE_CURVE ( 3, ( #32511, #25051, #40189, #33009 ),
 .UNSPECIFIED., .F., .F. ) 
 B_SPLINE_CURVE_WITH_KNOTS ( ( 4, 4 ),
 ( 0.000000000000000000, 1.570796326794896558 ),
 .UNSPECIFIED. ) 
 CURVE ( )  GEOMETRIC_REPRESENTATION_ITEM ( )  RATIONAL_B_SPLINE_CURVE ( ( 1.000000000000000000, 0.8047378541243649375, 0.8047378541243649375, 1.000000000000000000 ) ) 
 REPRESENTATION_ITEM ( '' )  );
#32028=FACE_OUTER_BOUND ( 'NONE', #42561, .T. ) ;
#32030=ORIENTED_EDGE ( 'NONE', *, *, #37769, .F. ) ;
#32031=ORIENTED_EDGE ( 'NONE', *, *, #41987, .T. ) ;
#32034=( BOUNDED_CURVE ( )  B_SPLINE_CURVE ( 3, ( #30536, #26690, #45139, #21565 ),
 .UNSPECIFIED., .F., .F. ) 
 B_SPLINE_CURVE_WITH_KNOTS ( ( 4, 4 ),
 ( 0.000000000000000000, 1.570796326794896558 ),
 .UNSPECIFIED. ) 
 CURVE ( )  GEOMETRIC_REPRESENTATION_ITEM ( )  RATIONAL_B_SPLINE_CURVE ( ( 1.000000000000000000, 0.8047378541243649375, 0.8047378541243649375, 1.000000000000000000 ) ) 
 REPRESENTATION_ITEM ( '' )  );
#32038=CYLINDRICAL_SURFACE ( 'NONE', #47868, 1.750000000000008438 ) ;
#32039=DIRECTION ( 'NONE',  ( -0.000000000000000000, -0.000000000000000000, -1.000000000000000000 ) ) ;
#32042=CARTESIAN_POINT ( 'NONE',  ( -125.6708471809678542, 1.749999999999996891, 81.84341382277506227 ) ) ;
#32043=DIRECTION ( 'NONE',  ( -1.000000000000000000, -0.000000000000000000, -0.000000000000000000 ) ) ;
#32048=VECTOR ( 'NONE', #26615, 1000.000000000000000 ) ;
#32050=FACE_OUTER_BOUND ( 'NONE', #22046, .T. ) ;
#32053=ORIENTED_EDGE ( 'NONE', *, *, #38424, .F. ) ;
#32054=EDGE_CURVE ( 'NONE', #37949, #34748, #32946, .T. ) ;
#32066=CARTESIAN_POINT ( 'NONE',  ( 73.30402655318508209, 0.000000000000000000, 165.0000000000000000 ) ) ;
#32068=ORIENTED_EDGE ( 'NONE', *, *, #23288, .T. ) ;
#32070=EDGE_LOOP ( 'NONE', ( #45576, #32853, #18274, #12357, #1330, #33905 ) ) ;
#32072=CARTESIAN_POINT ( 'NONE',  ( -204.9459734468148895, 1.025126265847089879, 122.5682875569280128 ) ) ;
#32079=CARTESIAN_POINT ( 'NONE',  ( -168.4459734468149747, -1.025126265847089213, 159.0682875569279418 ) ) ;
#32082=ORIENTED_EDGE ( 'NONE', *, *, #25309, .F. ) ;
#32088=ORIENTED_EDGE ( 'NONE', *, *, #11171, .T. ) ;
#32089=DIRECTION ( 'NONE',  ( -1.000000000000000000, -0.000000000000000000, -0.000000000000000000 ) ) ;
#32090=FACE_OUTER_BOUND ( 'NONE', #26786, .T. ) ;
#32093=ORIENTED_EDGE ( 'NONE', *, *, #43417, .F. ) ;
#32094=DIRECTION ( 'NONE',  ( -1.000000000000000000, -0.000000000000000000, -0.000000000000000000 ) ) ;
#32098=VERTEX_POINT ( 'NONE', #12657 ) ;
#32114=CARTESIAN_POINT ( 'NONE',  ( 155.0540265531850537, -1.025126265847089657, -80.93171244307201562 ) ) ;
#32120=EDGE_LOOP ( 'NONE', ( #24516, #39514, #37961, #37220, #33160, #43374 ) ) ;
#32122=DIRECTION ( 'NONE',  ( 0.000000000000000000, 0.000000000000000000, -1.000000000000000000 ) ) ;
#32127=ORIENTED_EDGE ( 'NONE', *, *, #34840, .T. ) ;
#32135=ORIENTED_EDGE ( 'NONE', *, *, #19643, .F. ) ;
#32140=ADVANCED_FACE ( 'NONE', ( #36551 ), #17020, .T. ) ;
#32141=ORIENTED_EDGE ( 'NONE', *, *, #42134, .F. ) ;
#32146=ORIENTED_EDGE ( 'NONE', *, *, #41556, .T. ) ;
#32148=EDGE_CURVE ( 'NONE', #13512, #38070, #46665, .T. ) ;
#32152=EDGE_LOOP ( 'NONE', ( #33334, #20696, #3403, #16312, #49646, #28236 ) ) ;
#32153=ORIENTED_EDGE ( 'NONE', *, *, #1092, .F. ) ;
#32159=ORIENTED_EDGE ( 'NONE', *, *, #5675, .T. ) ;
#32160=CARTESIAN_POINT ( 'NONE',  ( 115.0540265531850395, 1.025126265847081219, 162.5682875569279133 ) ) ;
#32164=ORIENTED_EDGE ( 'NONE', *, *, #47432, .T. ) ;
#32165=( LENGTH_UNIT ( ) NAMED_UNIT ( * ) SI_UNIT ( .MILLI., .METRE. ) );
#32166=( BOUNDED_CURVE ( )  B_SPLINE_CURVE ( 3, ( #12031, #488, #27931, #28188 ),
 .UNSPECIFIED., .F., .F. ) 
 B_SPLINE_CURVE_WITH_KNOTS ( ( 4, 4 ),
 ( 4.712388980384689674, 6.283185307179586232 ),
 .UNSPECIFIED. ) 
 CURVE ( )  GEOMETRIC_REPRESENTATION_ITEM ( )  RATIONAL_B_SPLINE_CURVE ( ( 1.000000000000000000, 0.8047378541243649375, 0.8047378541243649375, 1.000000000000000000 ) ) 
 REPRESENTATION_ITEM ( '' )  );
#32169=CARTESIAN_POINT ( 'NONE',  ( 152.2789002873379900, -1.750000000000009548, 39.79316129108089228 ) ) ;
#32170=EDGE_CURVE ( 'NONE', #25384, #40502, #29619, .T. ) ;
#32177=CYLINDRICAL_SURFACE ( 'NONE', #9969, 1.750000000000001554 ) ;
#32186=DIRECTION ( 'NONE',  ( -0.000000000000000000, -0.000000000000000000, -1.000000000000000000 ) ) ;
#32187=( BOUNDED_CURVE ( )  B_SPLINE_CURVE ( 3, ( #32495, #32998, #17578, #1439 ),
 .UNSPECIFIED., .F., .F. ) 
 B_SPLINE_CURVE_WITH_KNOTS ( ( 4, 4 ),
 ( 4.712388980384689674, 6.283185307179586232 ),
 .UNSPECIFIED. ) 
 CURVE ( )  GEOMETRIC_REPRESENTATION_ITEM ( )  RATIONAL_B_SPLINE_CURVE ( ( 1.000000000000000000, 0.8047378541243649375, 0.8047378541243649375, 1.000000000000000000 ) ) 
 REPRESENTATION_ITEM ( '' )  );
#32205=CYLINDRICAL_SURFACE ( 'NONE', #11872, 1.750000000000015543 ) ;
#32206=LINE ( 'NONE', #43981, #27539 ) ;
#32207=DIRECTION ( 'NONE',  ( -1.000000000000000000, -0.000000000000000000, -0.000000000000000000 ) ) ;
#32209=VERTEX_POINT ( 'NONE', #6475 ) ;
#32215=EDGE_CURVE ( 'NONE', #43597, #35332, #1463, .T. ) ;
#32218=CARTESIAN_POINT ( 'NONE',  ( -204.9459734468148895, 1.025126265847089435, 162.5682875569279133 ) ) ;
#32221=CARTESIAN_POINT ( 'NONE',  ( -7.721099712662037540, -1.750000000000022871, -160.2068387089191219 ) ) ;
#32224=DIRECTION ( 'NONE',  ( -1.000000000000000000, -0.000000000000000000, -0.000000000000000000 ) ) ;
#32228=DIRECTION ( 'NONE',  ( 0.000000000000000000, 0.000000000000000000, 1.000000000000000000 ) ) ;
#32229=ORIENTED_EDGE ( 'NONE', *, *, #46847, .F. ) ;
#32242=CARTESIAN_POINT ( 'NONE',  ( -46.69597344681494633, -1.750000000000010658, -79.18171244307201562 ) ) ;
#32243=VECTOR ( 'NONE', #27634, 1000.000000000000000 ) ;
#32245=CARTESIAN_POINT ( 'NONE',  ( 151.5540265531850537, 0.000000000000000000, 39.06828755692798438 ) ) ;
#32250=FACE_OUTER_BOUND ( 'NONE', #34030, .T. ) ;
#32252=CARTESIAN_POINT ( 'NONE',  ( -128.4459734468149179, 0.000000000000000000, 2.568287556927950632 ) ) ;
#32253=FACE_OUTER_BOUND ( 'NONE', #23590, .T. ) ;
#32254=CARTESIAN_POINT ( 'NONE',  ( 210.0000000000000568, 0.000000000000000000, 120.8182875569279702 ) ) ;
#32255=ORIENTED_EDGE ( 'NONE', *, *, #39947, .T. ) ;
#32256=CARTESIAN_POINT ( 'NONE',  ( -165.6708471809677974, -1.750000000000009548, -40.20683870891912193 ) ) ;
#32261=CARTESIAN_POINT ( 'NONE',  ( -46.69597344681494633, 0.000000000000000000, 165.0000000000000000 ) ) ;
#32263=VECTOR ( 'NONE', #19895, 1000.000000000000000 ) ;
#32264=EDGE_CURVE ( 'NONE', #19656, #6992, #29574, .T. ) ;
#32265=EDGE_LOOP ( 'NONE', ( #15764, #49187, #179, #19709, #14924, #39851 ) ) ;
#32268=( BOUNDED_CURVE ( )  B_SPLINE_CURVE ( 3, ( #37438, #41255, #10216, #25618 ),
 .UNSPECIFIED., .F., .F. ) 
 B_SPLINE_CURVE_WITH_KNOTS ( ( 4, 4 ),
 ( 1.570796326794896558, 3.141592653589793116 ),
 .UNSPECIFIED. ) 
 CURVE ( )  GEOMETRIC_REPRESENTATION_ITEM ( )  RATIONAL_B_SPLINE_CURVE ( ( 1.000000000000000000, 0.8047378541243649375, 0.8047378541243649375, 1.000000000000000000 ) ) 
 REPRESENTATION_ITEM ( '' )  );
#32272=CARTESIAN_POINT ( 'NONE',  ( 210.0000000000000568, 0.000000000000000000, 80.81828755692798438 ) ) ;
#32273=ORIENTED_EDGE ( 'NONE', *, *, #50525, .F. ) ;
#32274=CARTESIAN_POINT ( 'NONE',  ( 71.55402655318505367, 1.025126265847089435, 122.5682875569280128 ) ) ;
#32275=ADVANCED_FACE ( 'NONE', ( #13673 ), #13412, .T. ) ;
#32283=VERTEX_POINT ( 'NONE', #37555 ) ;
#32285=ORIENTED_EDGE ( 'NONE', *, *, #4630, .F. ) ;
#32290=CARTESIAN_POINT ( 'NONE',  ( 210.0000000000000568, 2.143131898507881116E-16, -40.93171244307203693 ) ) ;
#32293=DIRECTION ( 'NONE',  ( -0.000000000000000000, -0.000000000000000000, -1.000000000000000000 ) ) ;
#32300=CARTESIAN_POINT ( 'NONE',  ( 35.05402655318504657, 1.025126265847089657, 119.0682875569279560 ) ) ;
#32304=AXIS2_PLACEMENT_3D ( 'NONE', #5523, #39936, #13473 ) ;
#32307=CARTESIAN_POINT ( 'NONE',  ( 73.30402655318508209, 1.750000000000010214, -39.18171244307202983 ) ) ;
#32312=ADVANCED_FACE ( 'NONE', ( #46698 ), #34711, .T. ) ;
#32316=DIRECTION ( 'NONE',  ( 0.000000000000000000, 0.000000000000000000, -1.000000000000000000 ) ) ;
#32319=CARTESIAN_POINT ( 'NONE',  ( 73.30402655318508209, -1.750000000000010658, -119.1817124430720440 ) ) ;
#32329=EDGE_LOOP ( 'NONE', ( #32146, #22715, #5828, #43626, #9345, #14370 ) ) ;
#32331=CARTESIAN_POINT ( 'NONE',  ( 73.30402655318508209, 0.000000000000000000, 165.0000000000000000 ) ) ;
#32333=( BOUNDED_CURVE ( )  B_SPLINE_CURVE ( 3, ( #7326, #7849, #38642, #147 ),
 .UNSPECIFIED., .F., .F. ) 
 B_SPLINE_CURVE_WITH_KNOTS ( ( 4, 4 ),
 ( 1.570796326794896558, 3.141592653589793116 ),
 .UNSPECIFIED. ) 
 CURVE ( )  GEOMETRIC_REPRESENTATION_ITEM ( )  RATIONAL_B_SPLINE_CURVE ( ( 1.000000000000000000, 0.8047378541243649375, 0.8047378541243649375, 1.000000000000000000 ) ) 
 REPRESENTATION_ITEM ( '' )  );
#32335=ORIENTED_EDGE ( 'NONE', *, *, #49627, .F. ) ;
#32337=VECTOR ( 'NONE', #7048, 1000.000000000000000 ) ;
#32339=CYLINDRICAL_SURFACE ( 'NONE', #22643, 1.750000000000010214 ) ;
#32350=ORIENTED_EDGE ( 'NONE', *, *, #15540, .T. ) ;
#32360=CARTESIAN_POINT ( 'NONE',  ( -205.6708471809678827, 1.750000000000009548, -40.20683870891912193 ) ) ;
#32364=CYLINDRICAL_SURFACE ( 'NONE', #7299, 1.750000000000036193 ) ;
#32365=DIRECTION ( 'NONE',  ( -1.000000000000000000, -0.000000000000000000, -0.000000000000000000 ) ) ;
#32366=CARTESIAN_POINT ( 'NONE',  ( 193.3040265531851105, 1.750000000000010214, -39.18171244307202983 ) ) ;
#32367=EDGE_CURVE ( 'NONE', #46904, #33640, #6727, .T. ) ;
#32370=CYLINDRICAL_SURFACE ( 'NONE', #3466, 1.750000000000001554 ) ;
#32373=AXIS2_PLACEMENT_3D ( 'NONE', #47708, #24422, #12593 ) ;
#32374=ORIENTED_EDGE ( 'NONE', *, *, #5891, .F. ) ;
#32376=CARTESIAN_POINT ( 'NONE',  ( -204.9459734468149463, 2.143131898507880377E-16, -37.43171244307205825 ) ) ;
#32379=CARTESIAN_POINT ( 'NONE',  ( -6.695973446814940111, 1.750000000000023759, 40.81828755692798438 ) ) ;
#32381=LINE ( 'NONE', #13859, #11556 ) ;
#32383=CARTESIAN_POINT ( 'NONE',  ( -8.445973446814976526, 0.000000000000000000, 165.0000000000000000 ) ) ;
#32384=DIRECTION ( 'NONE',  ( -1.000000000000000000, 0.000000000000000000, 0.000000000000000000 ) ) ;
#32388=DIRECTION ( 'NONE',  ( -1.000000000000000000, -0.000000000000000000, -0.000000000000000000 ) ) ;
#32390=ORIENTED_EDGE ( 'NONE', *, *, #23522, .F. ) ;
#32393=CYLINDRICAL_SURFACE ( 'NONE', #25596, 1.749999999999973799 ) ;
#32408=VECTOR ( 'NONE', #47899, 1000.000000000000000 ) ;
#32410=CARTESIAN_POINT ( 'NONE',  ( 113.3040265531850537, -1.749999999999997335, -119.1817124430720440 ) ) ;
#32414=ADVANCED_FACE ( 'NONE', ( #18522 ), #46448, .T. ) ;
#32415=CYLINDRICAL_SURFACE ( 'NONE', #42804, 1.750000000000015543 ) ;
#32417=CARTESIAN_POINT ( 'NONE',  ( -166.6959734468149463, 1.750000000000010214, -39.18171244307202983 ) ) ;
#32423=CARTESIAN_POINT ( 'NONE',  ( -45.67084718096785423, 1.750000000000010214, -118.1565861772249519 ) ) ;
#32427=VECTOR ( 'NONE', #29680, 1000.000000000000000 ) ;
#32428=LINE ( 'NONE', #8572, #46073 ) ;
#32429=VERTEX_POINT ( 'NONE', #8256 ) ;
#32432=DIRECTION ( 'NONE',  ( -1.000000000000000000, 0.000000000000000000, 0.000000000000000000 ) ) ;
#32433=EDGE_CURVE ( 'NONE', #24770, #37466, #38186, .T. ) ;
#32434=EDGE_CURVE ( 'NONE', #6557, #17311, #20798, .T. ) ;
#32440=LINE ( 'NONE', #31940, #31939 ) ;
#32447=VECTOR ( 'NONE', #17172, 1000.000000000000000 ) ;
#32453=AXIS2_PLACEMENT_3D ( 'NONE', #30661, #15265, #22693 ) ;
#32456=EDGE_CURVE ( 'NONE', #48958, #25250, #43397, .T. ) ;
#32465=LINE ( 'NONE', #36320, #24989 ) ;
#32467=CARTESIAN_POINT ( 'NONE',  ( -125.6708471809678542, 1.749999999999996669, -160.2068387089191219 ) ) ;
#32469=ORIENTED_EDGE ( 'NONE', *, *, #35342, .F. ) ;
#32473=ADVANCED_FACE ( 'NONE', ( #24167 ), #32364, .T. ) ;
#32474=AXIS2_PLACEMENT_3D ( 'NONE', #37134, #13240, #49108 ) ;
#32475=LINE ( 'NONE', #40161, #43087 ) ;
#32476=( BOUNDED_CURVE ( )  B_SPLINE_CURVE ( 3, ( #50044, #46208, #11105, #42895 ),
 .UNSPECIFIED., .F., .F. ) 
 B_SPLINE_CURVE_WITH_KNOTS ( ( 4, 4 ),
 ( 3.141592653589793116, 4.712388980384689674 ),
 .UNSPECIFIED. ) 
 CURVE ( )  GEOMETRIC_REPRESENTATION_ITEM ( )  RATIONAL_B_SPLINE_CURVE ( ( 1.000000000000000000, 0.8047378541243649375, 0.8047378541243649375, 1.000000000000000000 ) ) 
 REPRESENTATION_ITEM ( '' )  );
#32480=( BOUNDED_CURVE ( )  B_SPLINE_CURVE ( 3, ( #13972, #41174, #6297, #17828 ),
 .UNSPECIFIED., .F., .F. ) 
 B_SPLINE_CURVE_WITH_KNOTS ( ( 4, 4 ),
 ( 0.000000000000000000, 1.570796326794896558 ),
 .UNSPECIFIED. ) 
 CURVE ( )  GEOMETRIC_REPRESENTATION_ITEM ( )  RATIONAL_B_SPLINE_CURVE ( ( 1.000000000000000000, 0.8047378541243649375, 0.8047378541243649375, 1.000000000000000000 ) ) 
 REPRESENTATION_ITEM ( '' )  );
#32482=FACE_OUTER_BOUND ( 'NONE', #26218, .T. ) ;
#32483=EDGE_LOOP ( 'NONE', ( #41419, #44857, #2262, #29087, #14985 ) ) ;
#32486=CARTESIAN_POINT ( 'NONE',  ( 195.0540265531851105, 2.143131898507880377E-16, 42.56828755692798438 ) ) ;
#32488=ORIENTED_EDGE ( 'NONE', *, *, #43469, .F. ) ;
#32490=DIRECTION ( 'NONE',  ( -0.000000000000000000, -0.000000000000000000, -1.000000000000000000 ) ) ;
#32493=VECTOR ( 'NONE', #2102, 1000.000000000000000 ) ;
#32495=CARTESIAN_POINT ( 'NONE',  ( -46.69597344681494633, -1.750000000000010658, -119.1817124430720440 ) ) ;
#32496=VECTOR ( 'NONE', #19254, 1000.000000000000000 ) ;
#32499=FACE_OUTER_BOUND ( 'NONE', #29171, .T. ) ;
#32500=( BOUNDED_CURVE ( )  B_SPLINE_CURVE ( 3, ( #23289, #7406, #19181, #34601 ),
 .UNSPECIFIED., .F., .F. ) 
 B_SPLINE_CURVE_WITH_KNOTS ( ( 4, 4 ),
 ( 0.000000000000000000, 1.570796326794896558 ),
 .UNSPECIFIED. ) 
 CURVE ( )  GEOMETRIC_REPRESENTATION_ITEM ( )  RATIONAL_B_SPLINE_CURVE ( ( 1.000000000000000000, 0.8047378541243649375, 0.8047378541243649375, 1.000000000000000000 ) ) 
 REPRESENTATION_ITEM ( '' )  );
#32504=EDGE_CURVE ( 'NONE', #49119, #10420, #8360, .T. ) ;
#32511=CARTESIAN_POINT ( 'NONE',  ( 155.0540265531850537, 2.143131898507880377E-16, -160.9317124430720014 ) ) ;
#32513=ADVANCED_FACE ( 'NONE', ( #33134 ), #37248, .T. ) ;
#32515=CARTESIAN_POINT ( 'NONE',  ( 31.55402655318503236, 0.000000000000000000, 122.5682875569279702 ) ) ;
#32518=CYLINDRICAL_SURFACE ( 'NONE', #20450, 1.750000000000001554 ) ;
#32521=CARTESIAN_POINT ( 'NONE',  ( 210.0000000000000568, 0.000000000000000000, -159.1817124430720298 ) ) ;
#32525=CARTESIAN_POINT ( 'NONE',  ( 210.0000000000000568, 0.000000000000000000, 40.81828755692798438 ) ) ;
#32526=AXIS2_PLACEMENT_3D ( 'NONE', #48619, #40729, #12763 ) ;
#32527=EDGE_LOOP ( 'NONE', ( #14660, #760, #11036, #467, #8264, #19585 ) ) ;
#32530=ORIENTED_EDGE ( 'NONE', *, *, #41853, .T. ) ;
#32531=EDGE_LOOP ( 'NONE', ( #23754, #44472, #9109, #13700, #24645, #32579 ) ) ;
#32543=CARTESIAN_POINT ( 'NONE',  ( -124.9459734468149463, 2.143131898507847836E-16, 119.0682875569279844 ) ) ;
#32544=ADVANCED_FACE ( 'NONE', ( #17461 ), #10014, .T. ) ;
#32550=CARTESIAN_POINT ( 'NONE',  ( 155.0540265531850537, 2.143131898507880377E-16, 82.56828755692798438 ) ) ;
#32551=CARTESIAN_POINT ( 'NONE',  ( -87.72109971266203843, -1.750000000000010214, 79.79316129108087807 ) ) ;
#32552=CARTESIAN_POINT ( 'NONE',  ( 195.0540265531851105, 2.143131898507880377E-16, 2.568287556927978166 ) ) ;
#32554=CARTESIAN_POINT ( 'NONE',  ( 210.0000000000000568, 0.000000000000000000, -159.1817124430720298 ) ) ;
#32555=CARTESIAN_POINT ( 'NONE',  ( -126.6959734468149321, -1.749999999999997335, 120.8182875569279702 ) ) ;
#32559=AXIS2_PLACEMENT_3D ( 'NONE', #6148, #49706, #33363 ) ;
#32562=DIRECTION ( 'NONE',  ( -0.000000000000000000, -0.000000000000000000, -1.000000000000000000 ) ) ;
#32564=EDGE_CURVE ( 'NONE', #8390, #41541, #19869, .T. ) ;
#32568=CARTESIAN_POINT ( 'NONE',  ( 73.30402655318508209, -1.750000000000010658, 80.81828755692798438 ) ) ;
#32570=ADVANCED_FACE ( 'NONE', ( #41566 ), #36743, .T. ) ;
#32571=ORIENTED_EDGE ( 'NONE', *, *, #40874, .T. ) ;
#32576=CARTESIAN_POINT ( 'NONE',  ( 75.05402655318509630, 2.143131898507880377E-16, -120.9317124430720725 ) ) ;
#32577=CARTESIAN_POINT ( 'NONE',  ( -128.4459734468149179, 0.000000000000000000, 159.0682875569279986 ) ) ;
#32579=ORIENTED_EDGE ( 'NONE', *, *, #4909, .T. ) ;
#32580=ORIENTED_EDGE ( 'NONE', *, *, #30006, .F. ) ;
#32583=CARTESIAN_POINT ( 'NONE',  ( -168.4459734468149463, 0.000000000000000000, 39.06828755692798438 ) ) ;
#32597=ORIENTED_EDGE ( 'NONE', *, *, #15933, .T. ) ;
#32609=VERTEX_POINT ( 'NONE', #23070 ) ;
#32614=CARTESIAN_POINT ( 'NONE',  ( -165.6708471809677974, 1.750000000000010214, -120.2068387089191219 ) ) ;
#32617=CARTESIAN_POINT ( 'NONE',  ( -48.44597344681496054, -1.025126265847089657, 42.56828755692799149 ) ) ;
#32619=EDGE_CURVE ( 'NONE', #6739, #17123, #46374, .T. ) ;
#32620=EDGE_CURVE ( 'NONE', #50433, #14892, #9746, .T. ) ;
#32621=( BOUNDED_CURVE ( )  B_SPLINE_CURVE ( 3, ( #37531, #10056, #32218, #41356 ),
 .UNSPECIFIED., .F., .F. ) 
 B_SPLINE_CURVE_WITH_KNOTS ( ( 4, 4 ),
 ( 1.570796326794896558, 3.141592653589793116 ),
 .UNSPECIFIED. ) 
 CURVE ( )  GEOMETRIC_REPRESENTATION_ITEM ( )  RATIONAL_B_SPLINE_CURVE ( ( 1.000000000000000000, 0.8047378541243649375, 0.8047378541243649375, 1.000000000000000000 ) ) 
 REPRESENTATION_ITEM ( '' )  );
#32629=FACE_OUTER_BOUND ( 'NONE', #36215, .T. ) ;
#32630=CYLINDRICAL_SURFACE ( 'NONE', #39686, 1.750000000000015543 ) ;
#32631=( BOUNDED_CURVE ( )  B_SPLINE_CURVE ( 3, ( #47414, #20262, #15, #39020 ),
 .UNSPECIFIED., .F., .F. ) 
 B_SPLINE_CURVE_WITH_KNOTS ( ( 4, 4 ),
 ( 4.712388980384689674, 6.283185307179586232 ),
 .UNSPECIFIED. ) 
 CURVE ( )  GEOMETRIC_REPRESENTATION_ITEM ( )  RATIONAL_B_SPLINE_CURVE ( ( 1.000000000000000000, 0.8047378541243649375, 0.8047378541243649375, 1.000000000000000000 ) ) 
 REPRESENTATION_ITEM ( '' )  );
#32634=CARTESIAN_POINT ( 'NONE',  ( -8.445973446814976526, 0.000000000000000000, 39.06828755692792754 ) ) ;
#32637=CYLINDRICAL_SURFACE ( 'NONE', #24076, 1.750000000000010214 ) ;
#32642=ORIENTED_EDGE ( 'NONE', *, *, #31867, .F. ) ;
#32643=DIRECTION ( 'NONE',  ( -1.000000000000000000, -0.000000000000000000, -0.000000000000000000 ) ) ;
#32644=ORIENTED_EDGE ( 'NONE', *, *, #16270, .T. ) ;
#32650=CARTESIAN_POINT ( 'NONE',  ( 210.0000000000000568, 0.000000000000000000, -119.1817124430720440 ) ) ;
#32653=FACE_OUTER_BOUND ( 'NONE', #23337, .T. ) ;
#32655=CARTESIAN_POINT ( 'NONE',  ( -6.695973446814940111, -1.750000000000024203, -119.1817124430720440 ) ) ;
#32656=EDGE_LOOP ( 'NONE', ( #42667, #13258, #8723, #9465, #48364 ) ) ;
#32658=ORIENTED_EDGE ( 'NONE', *, *, #29517, .F. ) ;
#32659=ORIENTED_EDGE ( 'NONE', *, *, #20668, .F. ) ;
#32660=CARTESIAN_POINT ( 'NONE',  ( 193.3040265531851105, -1.750000000000010658, -119.1817124430720440 ) ) ;
#32668=CARTESIAN_POINT ( 'NONE',  ( -84.94597344681494633, 2.143131898507880377E-16, 165.0000000000000000 ) ) ;
#32671=LINE ( 'NONE', #1627, #37263 ) ;
#32673=ORIENTED_EDGE ( 'NONE', *, *, #13046, .F. ) ;
#32674=FACE_OUTER_BOUND ( 'NONE', #27299, .T. ) ;
#32677=DIRECTION ( 'NONE',  ( -0.000000000000000000, -0.000000000000000000, -1.000000000000000000 ) ) ;
#32686=ORIENTED_EDGE ( 'NONE', *, *, #39135, .T. ) ;
#32700=DIRECTION ( 'NONE',  ( -1.000000000000000000, 0.000000000000000000, 0.000000000000000000 ) ) ;
#32704=CARTESIAN_POINT ( 'NONE',  ( -126.6959734468149321, 0.000000000000000000, 165.0000000000000000 ) ) ;
#32705=CARTESIAN_POINT ( 'NONE',  ( 72.27890028733797578, 1.750000000000009548, 81.84341382277507648 ) ) ;
#32707=CARTESIAN_POINT ( 'NONE',  ( -124.9459734468149463, 2.143131898507847836E-16, -160.9317124430720014 ) ) ;
#32719=CARTESIAN_POINT ( 'NONE',  ( -204.9459734468148895, -1.025126265847088991, 2.568287556927986159 ) ) ;
#32725=ORIENTED_EDGE ( 'NONE', *, *, #7691, .T. ) ;
#32730=FACE_OUTER_BOUND ( 'NONE', #36515, .T. ) ;
#32732=AXIS2_PLACEMENT_3D ( 'NONE', #44799, #29423, #9670 ) ;
#32736=LINE ( 'NONE', #20677, #26932 ) ;
#32738=EDGE_CURVE ( 'NONE', #50107, #8682, #27692, .T. ) ;
#32742=CARTESIAN_POINT ( 'NONE',  ( 113.3040265531850537, 1.749999999999997335, 120.8182875569279702 ) ) ;
#32746=CARTESIAN_POINT ( 'NONE',  ( -164.9459734468149747, 0.000000000000000000, 162.5682875569279702 ) ) ;
#32747=FACE_OUTER_BOUND ( 'NONE', #26010, .T. ) ;
#32751=CARTESIAN_POINT ( 'NONE',  ( 153.3040265531850537, 1.750000000000010214, 40.81828755692798438 ) ) ;
#32752=CARTESIAN_POINT ( 'NONE',  ( 210.0000000000000568, 0.000000000000000000, 40.81828755692798438 ) ) ;
#32754=CARTESIAN_POINT ( 'NONE',  ( -206.6959734468149463, -1.750000000000010658, -79.18171244307201562 ) ) ;
#32755=ORIENTED_EDGE ( 'NONE', *, *, #27768, .F. ) ;
#32758=AXIS2_PLACEMENT_3D ( 'NONE', #39774, #35431, #42579 ) ;
#32762=( BOUNDED_CURVE ( )  B_SPLINE_CURVE ( 3, ( #42076, #30049, #48729, #5920 ),
 .UNSPECIFIED., .F., .F. ) 
 B_SPLINE_CURVE_WITH_KNOTS ( ( 4, 4 ),
 ( 4.712388980384689674, 6.283185307179586232 ),
 .UNSPECIFIED. ) 
 CURVE ( )  GEOMETRIC_REPRESENTATION_ITEM ( )  RATIONAL_B_SPLINE_CURVE ( ( 1.000000000000000000, 0.8047378541243649375, 0.8047378541243649375, 1.000000000000000000 ) ) 
 REPRESENTATION_ITEM ( '' )  );
#32767=VERTEX_POINT ( 'NONE', #47898 ) ;
#32768=ORIENTED_EDGE ( 'NONE', *, *, #42364, .T. ) ;
#32769=AXIS2_PLACEMENT_3D ( 'NONE', #7213, #30564, #41851 ) ;
#32770=( BOUNDED_CURVE ( )  B_SPLINE_CURVE ( 3, ( #41113, #29316, #45430, #37541 ),
 .UNSPECIFIED., .F., .F. ) 
 B_SPLINE_CURVE_WITH_KNOTS ( ( 4, 4 ),
 ( 3.141592653589793116, 4.712388980384689674 ),
 .UNSPECIFIED. ) 
 CURVE ( )  GEOMETRIC_REPRESENTATION_ITEM ( )  RATIONAL_B_SPLINE_CURVE ( ( 1.000000000000000000, 0.8047378541243649375, 0.8047378541243649375, 1.000000000000000000 ) ) 
 REPRESENTATION_ITEM ( '' )  );
#32771=DIRECTION ( 'NONE',  ( -1.000000000000000000, -0.000000000000000000, -0.000000000000000000 ) ) ;
#32773=EDGE_CURVE ( 'NONE', #3643, #34063, #44432, .T. ) ;
#32774=ORIENTED_EDGE ( 'NONE', *, *, #38467, .F. ) ;
#32775=CARTESIAN_POINT ( 'NONE',  ( 115.0540265531850395, 2.143131898507847836E-16, -80.93171244307201562 ) ) ;
#32776=CARTESIAN_POINT ( 'NONE',  ( 210.0000000000000568, 0.000000000000000000, 80.81828755692798438 ) ) ;
#32777=DIRECTION ( 'NONE',  ( 0.000000000000000000, 0.000000000000000000, 1.000000000000000000 ) ) ;
#32780=EDGE_LOOP ( 'NONE', ( #7607, #27962, #42465, #4253, #40071, #36386 ) ) ;
#32787=CARTESIAN_POINT ( 'NONE',  ( -87.72109971266203843, 1.750000000000010436, 79.79316129108087807 ) ) ;
#32790=( BOUNDED_CURVE ( )  B_SPLINE_CURVE ( 3, ( #26456, #38288, #10800, #42093 ),
 .UNSPECIFIED., .F., .F. ) 
 B_SPLINE_CURVE_WITH_KNOTS ( ( 4, 4 ),
 ( 3.141592653589793116, 4.712388980384689674 ),
 .UNSPECIFIED. ) 
 CURVE ( )  GEOMETRIC_REPRESENTATION_ITEM ( )  RATIONAL_B_SPLINE_CURVE ( ( 1.000000000000000000, 0.8047378541243649375, 0.8047378541243649375, 1.000000000000000000 ) ) 
 REPRESENTATION_ITEM ( '' )  );
#32794=DIRECTION ( 'NONE',  ( 0.000000000000000000, 0.000000000000000000, 1.000000000000000000 ) ) ;
#32795=CARTESIAN_POINT ( 'NONE',  ( 193.3040265531851105, 0.000000000000000000, 165.0000000000000000 ) ) ;
#32796=CARTESIAN_POINT ( 'NONE',  ( -45.67084718096785423, -1.750000000000009548, -160.2068387089191219 ) ) ;
#32800=DIRECTION ( 'NONE',  ( -0.000000000000000000, -0.000000000000000000, -1.000000000000000000 ) ) ;
#32801=CARTESIAN_POINT ( 'NONE',  ( 153.3040265531850537, 0.000000000000000000, -165.0000000000000000 ) ) ;
#32802=VECTOR ( 'NONE', #7398, 1000.000000000000000 ) ;
#32804=AXIS2_PLACEMENT_3D ( 'NONE', #27064, #42697, #7066 ) ;
#32808=EDGE_CURVE ( 'NONE', #3579, #48120, #35157, .T. ) ;
#32823=DIRECTION ( 'NONE',  ( 0.000000000000000000, 0.000000000000000000, -1.000000000000000000 ) ) ;
#32828=CARTESIAN_POINT ( 'NONE',  ( 112.2789002873379758, 1.749999999999997113, -120.2068387089191219 ) ) ;
#32831=EDGE_LOOP ( 'NONE', ( #5668, #6501, #15199, #31150, #5016 ) ) ;
#32833=ORIENTED_EDGE ( 'NONE', *, *, #26782, .F. ) ;
#32835=LINE ( 'NONE', #29226, #49431 ) ;
#32836=( BOUNDED_CURVE ( )  B_SPLINE_CURVE ( 3, ( #22935, #16258, #11908, #31160 ),
 .UNSPECIFIED., .F., .F. ) 
 B_SPLINE_CURVE_WITH_KNOTS ( ( 4, 4 ),
 ( 1.570796326794896558, 3.141592653589793116 ),
 .UNSPECIFIED. ) 
 CURVE ( )  GEOMETRIC_REPRESENTATION_ITEM ( )  RATIONAL_B_SPLINE_CURVE ( ( 1.000000000000000000, 0.8047378541243649375, 0.8047378541243649375, 1.000000000000000000 ) ) 
 REPRESENTATION_ITEM ( '' )  );
#32844=DIRECTION ( 'NONE',  ( 1.000000000000000000, 0.000000000000000000, 0.000000000000000000 ) ) ;
#32848=ORIENTED_EDGE ( 'NONE', *, *, #2036, .F. ) ;
#32849=EDGE_CURVE ( 'NONE', #37221, #30766, #37587, .T. ) ;
#32850=DIRECTION ( 'NONE',  ( -0.000000000000000000, -0.000000000000000000, -1.000000000000000000 ) ) ;
#32852=ORIENTED_EDGE ( 'NONE', *, *, #33068, .T. ) ;
#32853=ORIENTED_EDGE ( 'NONE', *, *, #7184, .T. ) ;
#32855=FACE_OUTER_BOUND ( 'NONE', #46645, .T. ) ;
#32858=CIRCLE ( 'NONE', #2505, 1.750000000000015543 ) ;
#32859=ORIENTED_EDGE ( 'NONE', *, *, #2294, .T. ) ;
#32860=EDGE_CURVE ( 'NONE', #5763, #47457, #42787, .T. ) ;
#32862=CARTESIAN_POINT ( 'NONE',  ( -85.67084718096784002, -1.750000000000010436, 79.79316129108087807 ) ) ;
#32865=ORIENTED_EDGE ( 'NONE', *, *, #15627, .T. ) ;
#32867=LINE ( 'NONE', #21543, #11173 ) ;
#32875=( BOUNDED_CURVE ( )  B_SPLINE_CURVE ( 3, ( #8062, #32160, #23701, #43943 ),
 .UNSPECIFIED., .F., .F. ) 
 B_SPLINE_CURVE_WITH_KNOTS ( ( 4, 4 ),
 ( 3.141592653589793116, 4.712388980384689674 ),
 .UNSPECIFIED. ) 
 CURVE ( )  GEOMETRIC_REPRESENTATION_ITEM ( )  RATIONAL_B_SPLINE_CURVE ( ( 1.000000000000000000, 0.8047378541243649375, 0.8047378541243649375, 1.000000000000000000 ) ) 
 REPRESENTATION_ITEM ( '' )  );
#32883=ORIENTED_EDGE ( 'NONE', *, *, #20381, .F. ) ;
#32884=CARTESIAN_POINT ( 'NONE',  ( -168.4459734468149463, 0.000000000000000000, 2.568287556927978166 ) ) ;
#32890=CARTESIAN_POINT ( 'NONE',  ( -204.9459734468148895, 1.025126265847089657, -120.9317124430720440 ) ) ;
#32891=VECTOR ( 'NONE', #45263, 1000.000000000000000 ) ;
#32894=EDGE_CURVE ( 'NONE', #9162, #13539, #34269, .T. ) ;
#32898=DIRECTION ( 'NONE',  ( 0.000000000000000000, 0.000000000000000000, 1.000000000000000000 ) ) ;
#32899=CARTESIAN_POINT ( 'NONE',  ( 111.5540265531850679, 0.000000000000000000, 165.0000000000000000 ) ) ;
#32900=CARTESIAN_POINT ( 'NONE',  ( 195.0540265531851105, 2.143131898507880377E-16, 159.0682875569279702 ) ) ;
#32901=FACE_OUTER_BOUND ( 'NONE', #7856, .T. ) ;
#32906=EDGE_CURVE ( 'NONE', #24906, #10600, #48008, .T. ) ;
#32907=EDGE_LOOP ( 'NONE', ( #45090, #30099, #19319, #46775, #19579, #46848 ) ) ;
#32910=FACE_OUTER_BOUND ( 'NONE', #8411, .T. ) ;
#32911=ORIENTED_EDGE ( 'NONE', *, *, #10431, .F. ) ;
#32913=AXIS2_PLACEMENT_3D ( 'NONE', #9918, #33294, #22230 ) ;
#32922=EDGE_CURVE ( 'NONE', #36821, #23935, #3212, .T. ) ;
#32927=CARTESIAN_POINT ( 'NONE',  ( 151.5540265531850537, 0.000000000000000000, -40.93171244307202983 ) ) ;
#32934=LINE ( 'NONE', #17263, #8663 ) ;
#32938=( BOUNDED_CURVE ( )  B_SPLINE_CURVE ( 3, ( #7160, #10498, #42304, #18690 ),
 .UNSPECIFIED., .F., .F. ) 
 B_SPLINE_CURVE_WITH_KNOTS ( ( 4, 4 ),
 ( 4.712388980384689674, 6.283185307179586232 ),
 .UNSPECIFIED. ) 
 CURVE ( )  GEOMETRIC_REPRESENTATION_ITEM ( )  RATIONAL_B_SPLINE_CURVE ( ( 1.000000000000000000, 0.8047378541243649375, 0.8047378541243649375, 1.000000000000000000 ) ) 
 REPRESENTATION_ITEM ( '' )  );
#32943=LINE ( 'NONE', #13408, #36300 ) ;
#32944=VERTEX_POINT ( 'NONE', #20999 ) ;
#32946=( BOUNDED_CURVE ( )  B_SPLINE_CURVE ( 3, ( #40129, #47276, #47772, #48023 ),
 .UNSPECIFIED., .F., .F. ) 
 B_SPLINE_CURVE_WITH_KNOTS ( ( 4, 4 ),
 ( 4.712388980384689674, 6.283185307179586232 ),
 .UNSPECIFIED. ) 
 CURVE ( )  GEOMETRIC_REPRESENTATION_ITEM ( )  RATIONAL_B_SPLINE_CURVE ( ( 1.000000000000000000, 0.8047378541243649375, 0.8047378541243649375, 1.000000000000000000 ) ) 
 REPRESENTATION_ITEM ( '' )  );
#32947=DIRECTION ( 'NONE',  ( -0.000000000000000000, -0.000000000000000000, -1.000000000000000000 ) ) ;
#32956=CARTESIAN_POINT ( 'NONE',  ( -6.695973446814940111, 1.750000000000024203, 120.8182875569279702 ) ) ;
#32957=CARTESIAN_POINT ( 'NONE',  ( 71.55402655318505367, 0.000000000000000000, 82.56828755692799859 ) ) ;
#32959=ORIENTED_EDGE ( 'NONE', *, *, #19286, .F. ) ;
#32964=CARTESIAN_POINT ( 'NONE',  ( -208.4459734468149463, 0.000000000000000000, -40.93171244307202983 ) ) ;
#32965=ORIENTED_EDGE ( 'NONE', *, *, #27381, .F. ) ;
#32967=CARTESIAN_POINT ( 'NONE',  ( 151.5540265531850537, -1.025126265847089879, -117.4317124430720156 ) ) ;
#32972=LINE ( 'NONE', #13449, #47021 ) ;
#32984=CARTESIAN_POINT ( 'NONE',  ( 111.5540265531850537, 0.000000000000000000, 162.5682875569279702 ) ) ;
#32986=DIRECTION ( 'NONE',  ( -1.000000000000000000, 0.000000000000000000, 0.000000000000000000 ) ) ;
#32992=ORIENTED_EDGE ( 'NONE', *, *, #25841, .F. ) ;
#32997=VECTOR ( 'NONE', #34674, 1000.000000000000000 ) ;
#32998=CARTESIAN_POINT ( 'NONE',  ( -45.67084718096785423, -1.750000000000010436, -120.2068387089191219 ) ) ;
#33001=CARTESIAN_POINT ( 'NONE',  ( 210.0000000000000568, 0.000000000000000000, -117.4317124430720298 ) ) ;
#33003=CARTESIAN_POINT ( 'NONE',  ( -204.9459734468149463, 2.143131898507880377E-16, -0.9317124430720247208 ) ) ;
#33009=CARTESIAN_POINT ( 'NONE',  ( 153.3040265531850537, 1.750000000000009992, -159.1817124430720298 ) ) ;
#33010=VERTEX_POINT ( 'NONE', #27827 ) ;
#33014=CARTESIAN_POINT ( 'NONE',  ( -128.4459734468149463, 1.025126265847081219, 2.568287556927973281 ) ) ;
#33015=CARTESIAN_POINT ( 'NONE',  ( 73.30402655318508209, 1.750000000000009992, 0.8182875569279768335 ) ) ;
#33016=CARTESIAN_POINT ( 'NONE',  ( 32.27890028733795447, 1.750000000000009548, 39.79316129108089228 ) ) ;
#33017=ORIENTED_EDGE ( 'NONE', *, *, #12431, .T. ) ;
#33019=EDGE_LOOP ( 'NONE', ( #20744, #23824, #26110, #49724, #16815, #32833 ) ) ;
#33021=VECTOR ( 'NONE', #573, 1000.000000000000000 ) ;
#33022=CARTESIAN_POINT ( 'NONE',  ( -48.44597344681495343, 0.000000000000000000, -0.9317124430720247208 ) ) ;
#33024=CIRCLE ( 'NONE', #13370, 1.750000000000015543 ) ;
#33025=CARTESIAN_POINT ( 'NONE',  ( 113.3040265531850537, 0.000000000000000000, 165.0000000000000000 ) ) ;
#33031=CARTESIAN_POINT ( 'NONE',  ( -208.4459734468149463, 0.000000000000000000, 165.0000000000000000 ) ) ;
#33032=ORIENTED_EDGE ( 'NONE', *, *, #3386, .T. ) ;
#33033=DIRECTION ( 'NONE',  ( 0.000000000000000000, 0.000000000000000000, 1.000000000000000000 ) ) ;
#33035=ORIENTED_EDGE ( 'NONE', *, *, #14239, .T. ) ;
#33036=ORIENTED_EDGE ( 'NONE', *, *, #16338, .F. ) ;
#33038=FACE_OUTER_BOUND ( 'NONE', #349, .T. ) ;
#33044=CARTESIAN_POINT ( 'NONE',  ( -4.945973446814916130, 1.025126265847097651, -117.4317124430720014 ) ) ;
#33046=CARTESIAN_POINT ( 'NONE',  ( -8.445973446814976526, 0.000000000000000000, 165.0000000000000000 ) ) ;
#33048=AXIS2_PLACEMENT_3D ( 'NONE', #14047, #6614, #14306 ) ;
#33052=CYLINDRICAL_SURFACE ( 'NONE', #48524, 1.750000000000001554 ) ;
#33055=AXIS2_PLACEMENT_3D ( 'NONE', #44327, #21495, #36687 ) ;
#33062=CARTESIAN_POINT ( 'NONE',  ( -85.67084718096784002, -1.750000000000009326, -158.1565861772249377 ) ) ;
#33067=( BOUNDED_CURVE ( )  B_SPLINE_CURVE ( 3, ( #42475, #19129, #31212, #46549 ),
 .UNSPECIFIED., .F., .F. ) 
 B_SPLINE_CURVE_WITH_KNOTS ( ( 4, 4 ),
 ( 1.570796326794896558, 3.141592653589793116 ),
 .UNSPECIFIED. ) 
 CURVE ( )  GEOMETRIC_REPRESENTATION_ITEM ( )  RATIONAL_B_SPLINE_CURVE ( ( 1.000000000000000000, 0.8047378541243649375, 0.8047378541243649375, 1.000000000000000000 ) ) 
 REPRESENTATION_ITEM ( '' )  );
#33068=EDGE_CURVE ( 'NONE', #30056, #46777, #14627, .T. ) ;
#33070=CARTESIAN_POINT ( 'NONE',  ( -124.9459734468149321, 1.025126265847081886, -80.93171244307201562 ) ) ;
#33073=ORIENTED_EDGE ( 'NONE', *, *, #50257, .T. ) ;
#33086=CARTESIAN_POINT ( 'NONE',  ( 191.5540265531850537, -1.025126265847089657, 79.06828755692797017 ) ) ;
#33094=( BOUNDED_CURVE ( )  B_SPLINE_CURVE ( 3, ( #48115, #36129, #1479, #40216 ),
 .UNSPECIFIED., .F., .F. ) 
 B_SPLINE_CURVE_WITH_KNOTS ( ( 4, 4 ),
 ( 3.141592653589793116, 4.712388980384689674 ),
 .UNSPECIFIED. ) 
 CURVE ( )  GEOMETRIC_REPRESENTATION_ITEM ( )  RATIONAL_B_SPLINE_CURVE ( ( 1.000000000000000000, 0.8047378541243649375, 0.8047378541243649375, 1.000000000000000000 ) ) 
 REPRESENTATION_ITEM ( '' )  );
#33097=ORIENTED_EDGE ( 'NONE', *, *, #17552, .F. ) ;
#33100=AXIS2_PLACEMENT_3D ( 'NONE', #1501, #36414, #28194 ) ;
#33104=DIRECTION ( 'NONE',  ( -1.000000000000000000, -0.000000000000000000, -0.000000000000000000 ) ) ;
#33109=CARTESIAN_POINT ( 'NONE',  ( 195.0540265531851105, 2.143131898507880377E-16, 165.0000000000000000 ) ) ;
#33118=ORIENTED_EDGE ( 'NONE', *, *, #24834, .F. ) ;
#33120=CARTESIAN_POINT ( 'NONE',  ( 153.3040265531850537, -1.750000000000010658, -79.18171244307201562 ) ) ;
#33122=EDGE_CURVE ( 'NONE', #2781, #43783, #32440, .T. ) ;
#33123=ORIENTED_EDGE ( 'NONE', *, *, #31652, .T. ) ;
#33124=DIRECTION ( 'NONE',  ( -0.000000000000000000, -0.000000000000000000, -1.000000000000000000 ) ) ;
#33129=CARTESIAN_POINT ( 'NONE',  ( -166.6959734468149463, 0.000000000000000000, 165.0000000000000000 ) ) ;
#33130=EDGE_LOOP ( 'NONE', ( #39002, #37225, #19004, #36994, #49061, #421 ) ) ;
#33133=CARTESIAN_POINT ( 'NONE',  ( -204.9459734468149463, 2.143131898507880377E-16, 82.56828755692798438 ) ) ;
#33134=FACE_OUTER_BOUND ( 'NONE', #20817, .T. ) ;
#33135=CARTESIAN_POINT ( 'NONE',  ( -84.94597344681494633, 2.143131898507880377E-16, 79.06828755692797017 ) ) ;
#33136=VECTOR ( 'NONE', #30219, 1000.000000000000000 ) ;
#33137=CARTESIAN_POINT ( 'NONE',  ( 191.5540265531850537, 1.025126265847089435, -40.93171244307204404 ) ) ;
#33144=VERTEX_POINT ( 'NONE', #1139 ) ;
#33145=EDGE_CURVE ( 'NONE', #44889, #43082, #43109, .T. ) ;
#33147=CARTESIAN_POINT ( 'NONE',  ( 210.0000000000000568, 0.000000000000000000, 160.8182875569279702 ) ) ;
#33151=EDGE_CURVE ( 'NONE', #41405, #5869, #21252, .T. ) ;
#33153=FACE_OUTER_BOUND ( 'NONE', #41728, .T. ) ;
#33159=CYLINDRICAL_SURFACE ( 'NONE', #4432, 1.750000000000008438 ) ;
#33160=ORIENTED_EDGE ( 'NONE', *, *, #35010, .T. ) ;
#33165=DIRECTION ( 'NONE',  ( 0.000000000000000000, 0.000000000000000000, -1.000000000000000000 ) ) ;
#33166=CARTESIAN_POINT ( 'NONE',  ( 153.3040265531850537, 0.000000000000000000, 165.0000000000000000 ) ) ;
#33167=VERTEX_POINT ( 'NONE', #40391 ) ;
#33171=ORIENTED_EDGE ( 'NONE', *, *, #33873, .F. ) ;
#33173=CARTESIAN_POINT ( 'NONE',  ( -5.670847180967843570, -1.750000000000023315, -160.2068387089191219 ) ) ;
#33179=EDGE_LOOP ( 'NONE', ( #47539, #27204, #25170, #33965, #7568, #14823 ) ) ;
#33180=CARTESIAN_POINT ( 'NONE',  ( -126.6959734468149321, 1.749999999999997335, 120.8182875569279702 ) ) ;
#33181=CARTESIAN_POINT ( 'NONE',  ( -44.94597344681493922, 2.143131898507880377E-16, 42.56828755692798438 ) ) ;
#33182=FACE_OUTER_BOUND ( 'NONE', #13338, .T. ) ;
#33192=FACE_OUTER_BOUND ( 'NONE', #11906, .T. ) ;
#33194=CARTESIAN_POINT ( 'NONE',  ( -127.7210997126620242, 1.749999999999996669, -0.2068387089191042749 ) ) ;
#33201=EDGE_CURVE ( 'NONE', #39980, #14882, #35937, .T. ) ;
#33204=CARTESIAN_POINT ( 'NONE',  ( -166.6959734468149463, 0.000000000000000000, 165.0000000000000000 ) ) ;
#33211=EDGE_CURVE ( 'NONE', #31704, #20835, #45451, .T. ) ;
#33218=ADVANCED_FACE ( 'NONE', ( #10346 ), #37059, .T. ) ;
#33220=ORIENTED_EDGE ( 'NONE', *, *, #12725, .F. ) ;
#33222=CARTESIAN_POINT ( 'NONE',  ( 73.30402655318508209, -1.750000000000010658, -79.18171244307201562 ) ) ;
#33225=ORIENTED_EDGE ( 'NONE', *, *, #35125, .F. ) ;
#33226=DIRECTION ( 'NONE',  ( -0.000000000000000000, -0.000000000000000000, -1.000000000000000000 ) ) ;
#33229=LINE ( 'NONE', #17558, #42788 ) ;
#33232=ORIENTED_EDGE ( 'NONE', *, *, #5097, .F. ) ;
#33235=AXIS2_PLACEMENT_3D ( 'NONE', #6231, #15436, #22367 ) ;
#33236=ORIENTED_EDGE ( 'NONE', *, *, #45211, .T. ) ;
#33237=AXIS2_PLACEMENT_3D ( 'NONE', #21282, #9990, #25648 ) ;
#33240=( BOUNDED_CURVE ( )  B_SPLINE_CURVE ( 3, ( #49936, #30493, #50452, #25899 ),
 .UNSPECIFIED., .F., .F. ) 
 B_SPLINE_CURVE_WITH_KNOTS ( ( 4, 4 ),
 ( 1.570796326794896558, 3.141592653589793116 ),
 .UNSPECIFIED. ) 
 CURVE ( )  GEOMETRIC_REPRESENTATION_ITEM ( )  RATIONAL_B_SPLINE_CURVE ( ( 1.000000000000000000, 0.8047378541243649375, 0.8047378541243649375, 1.000000000000000000 ) ) 
 REPRESENTATION_ITEM ( '' )  );
#33261=CARTESIAN_POINT ( 'NONE',  ( -205.6708471809678827, 1.750000000000010214, -118.1565861772249519 ) ) ;
#33267=ORIENTED_EDGE ( 'NONE', *, *, #26643, .F. ) ;
#33268=DIRECTION ( 'NONE',  ( -0.000000000000000000, -0.000000000000000000, -1.000000000000000000 ) ) ;
#33270=CARTESIAN_POINT ( 'NONE',  ( -88.44597344681497475, 0.000000000000000000, 165.0000000000000000 ) ) ;
#33272=DIRECTION ( 'NONE',  ( -0.000000000000000000, -0.000000000000000000, -1.000000000000000000 ) ) ;
#33277=FACE_OUTER_BOUND ( 'NONE', #22670, .T. ) ;
#33282=CARTESIAN_POINT ( 'NONE',  ( 113.3040265531850537, -1.749999999999997335, 120.8182875569279702 ) ) ;
#33284=LINE ( 'NONE', #22218, #34451 ) ;
#33286=ORIENTED_EDGE ( 'NONE', *, *, #6542, .T. ) ;
#33290=DIRECTION ( 'NONE',  ( 0.000000000000000000, 0.000000000000000000, 1.000000000000000000 ) ) ;
#33293=PLANE ( 'NONE',  #32526 ) ;
#33294=DIRECTION ( 'NONE',  ( -1.000000000000000000, -0.000000000000000000, -0.000000000000000000 ) ) ;
#33296=VECTOR ( 'NONE', #32089, 1000.000000000000000 ) ;
#33299=CARTESIAN_POINT ( 'NONE',  ( 111.5540265531850679, 0.000000000000000000, 159.0682875569279702 ) ) ;
#33300=DIRECTION ( 'NONE',  ( 0.000000000000000000, 0.000000000000000000, 1.000000000000000000 ) ) ;
#33304=CARTESIAN_POINT ( 'NONE',  ( 115.0540265531850395, 2.143131898507847836E-16, -120.9317124430720156 ) ) ;
#33308=VECTOR ( 'NONE', #36981, 1000.000000000000000 ) ;
#33312=LINE ( 'NONE', #25342, #49359 ) ;
#33319=EDGE_LOOP ( 'NONE', ( #5620, #45566, #24289, #38506, #28566, #2273 ) ) ;
#33320=CARTESIAN_POINT ( 'NONE',  ( -88.44597344681497475, 0.000000000000000000, -120.9317124430720725 ) ) ;
#33329=ORIENTED_EDGE ( 'NONE', *, *, #2002, .F. ) ;
#33331=VERTEX_POINT ( 'NONE', #40878 ) ;
#33334=ORIENTED_EDGE ( 'NONE', *, *, #8923, .T. ) ;
#33336=CARTESIAN_POINT ( 'NONE',  ( -168.4459734468149747, 1.025126265847089213, 162.5682875569279133 ) ) ;
#33338=CARTESIAN_POINT ( 'NONE',  ( -128.4459734468149463, 1.025126265847081442, -160.9317124430720014 ) ) ;
#33340=CARTESIAN_POINT ( 'NONE',  ( 210.0000000000000568, 2.143131898507881856E-16, -80.93171244307202983 ) ) ;
#33341=ADVANCED_FACE ( 'NONE', ( #6480 ), #1886, .T. ) ;
#33343=ORIENTED_EDGE ( 'NONE', *, *, #30250, .F. ) ;
#33344=VECTOR ( 'NONE', #16355, 1000.000000000000000 ) ;
#33349=CARTESIAN_POINT ( 'NONE',  ( 111.5540265531850537, 2.143131898507880377E-16, -160.9317124430720298 ) ) ;
#33354=LINE ( 'NONE', #37223, #49567 ) ;
#33356=EDGE_LOOP ( 'NONE', ( #10065, #45105 ) ) ;
#33358=DIRECTION ( 'NONE',  ( -1.000000000000000000, 0.000000000000000000, 0.000000000000000000 ) ) ;
#33360=CYLINDRICAL_SURFACE ( 'NONE', #46005, 1.750000000000001554 ) ;
#33363=DIRECTION ( 'NONE',  ( 0.000000000000000000, 0.000000000000000000, 1.000000000000000000 ) ) ;
#33371=ORIENTED_EDGE ( 'NONE', *, *, #38426, .T. ) ;
#33373=( BOUNDED_CURVE ( )  B_SPLINE_CURVE ( 3, ( #42564, #35410, #47142, #19211 ),
 .UNSPECIFIED., .F., .F. ) 
 B_SPLINE_CURVE_WITH_KNOTS ( ( 4, 4 ),
 ( 4.712388980384689674, 6.283185307179586232 ),
 .UNSPECIFIED. ) 
 CURVE ( )  GEOMETRIC_REPRESENTATION_ITEM ( )  RATIONAL_B_SPLINE_CURVE ( ( 1.000000000000000000, 0.8047378541243649375, 0.8047378541243649375, 1.000000000000000000 ) ) 
 REPRESENTATION_ITEM ( '' )  );
#33376=DIRECTION ( 'NONE',  ( -1.000000000000000000, -0.000000000000000000, -0.000000000000000000 ) ) ;
#33378=DIRECTION ( 'NONE',  ( -0.000000000000000000, -0.000000000000000000, -1.000000000000000000 ) ) ;
#33380=( BOUNDED_CURVE ( )  B_SPLINE_CURVE ( 3, ( #21817, #40310, #32614, #29007 ),
 .UNSPECIFIED., .F., .F. ) 
 B_SPLINE_CURVE_WITH_KNOTS ( ( 4, 4 ),
 ( 0.000000000000000000, 1.570796326794896558 ),
 .UNSPECIFIED. ) 
 CURVE ( )  GEOMETRIC_REPRESENTATION_ITEM ( )  RATIONAL_B_SPLINE_CURVE ( ( 1.000000000000000000, 0.8047378541243649375, 0.8047378541243649375, 1.000000000000000000 ) ) 
 REPRESENTATION_ITEM ( '' )  );
#33384=CARTESIAN_POINT ( 'NONE',  ( 195.0540265531851105, 2.143131898507890731E-16, -165.0000000000000000 ) ) ;
#33387=FACE_OUTER_BOUND ( 'NONE', #6099, .T. ) ;
#33389=EDGE_CURVE ( 'NONE', #23796, #4361, #42125, .T. ) ;
#33393=DIRECTION ( 'NONE',  ( -1.000000000000000000, -0.000000000000000000, -0.000000000000000000 ) ) ;
#33400=CARTESIAN_POINT ( 'NONE',  ( -126.6959734468149321, 0.000000000000000000, 165.0000000000000000 ) ) ;
#33401=CIRCLE ( 'NONE', #4716, 1.750000000000015543 ) ;
#33404=CARTESIAN_POINT ( 'NONE',  ( -46.69597344681494633, 0.000000000000000000, 165.0000000000000000 ) ) ;
#33407=CARTESIAN_POINT ( 'NONE',  ( 73.30402655318508209, 1.750000000000010214, -39.18171244307202983 ) ) ;
#33414=EDGE_CURVE ( 'NONE', #28555, #20580, #27068, .T. ) ;
#33415=ORIENTED_EDGE ( 'NONE', *, *, #22650, .T. ) ;
#33417=CARTESIAN_POINT ( 'NONE',  ( 210.0000000000000568, 0.000000000000000000, -119.1817124430720440 ) ) ;
#33420=ADVANCED_FACE ( 'NONE', ( #1946 ), #5535, .T. ) ;
#33423=CARTESIAN_POINT ( 'NONE',  ( 32.27890028733795447, -1.750000000000009548, -0.2068387089191121020 ) ) ;
#33431=CARTESIAN_POINT ( 'NONE',  ( -127.7210997126620242, -1.749999999999996669, -0.2068387089191042749 ) ) ;
#33437=CARTESIAN_POINT ( 'NONE',  ( 73.30402655318508209, -1.750000000000009992, -159.1817124430720298 ) ) ;
#33441=CARTESIAN_POINT ( 'NONE',  ( 210.0000000000000568, 0.000000000000000000, 122.5682875569279844 ) ) ;
#33442=LINE ( 'NONE', #48779, #31538 ) ;
#33443=CARTESIAN_POINT ( 'NONE',  ( 31.55402655318503236, 1.025126265847089435, 82.56828755692798438 ) ) ;
#33452=ORIENTED_EDGE ( 'NONE', *, *, #4252, .T. ) ;
#33457=ORIENTED_EDGE ( 'NONE', *, *, #32367, .F. ) ;
#33465=LINE ( 'NONE', #13934, #9098 ) ;
#33469=CARTESIAN_POINT ( 'NONE',  ( 73.30402655318508209, -1.750000000000009992, 0.8182875569279768335 ) ) ;
#33470=CARTESIAN_POINT ( 'NONE',  ( -84.94597344681493212, 1.025126265847089879, -77.43171244307200141 ) ) ;
#33474=VERTEX_POINT ( 'NONE', #13980 ) ;
#33478=EDGE_CURVE ( 'NONE', #44104, #10041, #44236, .T. ) ;
#33479=EDGE_CURVE ( 'NONE', #14675, #45829, #9391, .T. ) ;
#33481=ORIENTED_EDGE ( 'NONE', *, *, #30207, .T. ) ;
#33484=ADVANCED_FACE ( 'NONE', ( #9390 ), #1695, .T. ) ;
#33486=ORIENTED_EDGE ( 'NONE', *, *, #2358, .T. ) ;
#33487=EDGE_CURVE ( 'NONE', #24426, #9029, #43403, .T. ) ;
#33493=DIRECTION ( 'NONE',  ( 0.000000000000000000, 0.000000000000000000, 1.000000000000000000 ) ) ;
#33498=ORIENTED_EDGE ( 'NONE', *, *, #2626, .F. ) ;
#33502=DIRECTION ( 'NONE',  ( -1.000000000000000000, 0.000000000000000000, 0.000000000000000000 ) ) ;
#33514=ORIENTED_EDGE ( 'NONE', *, *, #17194, .F. ) ;
#33516=EDGE_LOOP ( 'NONE', ( #25982, #42365, #32141, #3397, #10244, #27241 ) ) ;
#33518=EDGE_CURVE ( 'NONE', #36323, #12663, #44768, .T. ) ;
#33524=ORIENTED_EDGE ( 'NONE', *, *, #16558, .F. ) ;
#33525=( BOUNDED_CURVE ( )  B_SPLINE_CURVE ( 3, ( #24804, #19930, #44026, #43278 ),
 .UNSPECIFIED., .F., .F. ) 
 B_SPLINE_CURVE_WITH_KNOTS ( ( 4, 4 ),
 ( 1.570796326794896558, 3.141592653589793116 ),
 .UNSPECIFIED. ) 
 CURVE ( )  GEOMETRIC_REPRESENTATION_ITEM ( )  RATIONAL_B_SPLINE_CURVE ( ( 1.000000000000000000, 0.8047378541243649375, 0.8047378541243649375, 1.000000000000000000 ) ) 
 REPRESENTATION_ITEM ( '' )  );
#33529=DIRECTION ( 'NONE',  ( 0.000000000000000000, 0.000000000000000000, 1.000000000000000000 ) ) ;
#33533=CARTESIAN_POINT ( 'NONE',  ( -210.0000000000000568, 0.000000000000000000, 2.568287556927987048 ) ) ;
#33537=ORIENTED_EDGE ( 'NONE', *, *, #42841, .F. ) ;
#33539=CARTESIAN_POINT ( 'NONE',  ( -88.44597344681497475, 0.000000000000000000, -157.4317124430720014 ) ) ;
#33543=CYLINDRICAL_SURFACE ( 'NONE', #10357, 1.750000000000008438 ) ;
#33544=DIRECTION ( 'NONE',  ( -1.000000000000000000, -0.000000000000000000, -0.000000000000000000 ) ) ;
#33546=ORIENTED_EDGE ( 'NONE', *, *, #37488, .T. ) ;
#33548=CARTESIAN_POINT ( 'NONE',  ( -6.695973446814940111, -1.750000000000023759, -39.18171244307202983 ) ) ;
#33549=CARTESIAN_POINT ( 'NONE',  ( -208.4459734468149463, 0.000000000000000000, 39.06828755692798438 ) ) ;
#33552=CYLINDRICAL_SURFACE ( 'NONE', #39148, 1.750000000000008438 ) ;
#33553=CARTESIAN_POINT ( 'NONE',  ( -44.94597344681493922, -1.025126265847089213, -160.9317124430720014 ) ) ;
#33554=CARTESIAN_POINT ( 'NONE',  ( -45.67084718096785423, -1.750000000000009326, 159.7931612910809065 ) ) ;
#33562=ORIENTED_EDGE ( 'NONE', *, *, #47793, .F. ) ;
#33566=AXIS2_PLACEMENT_3D ( 'NONE', #40256, #4834, #32316 ) ;
#33571=VERTEX_POINT ( 'NONE', #19093 ) ;
#33583=AXIS2_PLACEMENT_3D ( 'NONE', #13184, #29097, #1402 ) ;
#33585=CARTESIAN_POINT ( 'NONE',  ( -167.7210997126620384, 1.750000000000009548, 41.84341382277508359 ) ) ;
#33586=DIRECTION ( 'NONE',  ( -1.000000000000000000, -0.000000000000000000, -0.000000000000000000 ) ) ;
#33590=FACE_OUTER_BOUND ( 'NONE', #45394, .T. ) ;
#33596=ORIENTED_EDGE ( 'NONE', *, *, #17538, .T. ) ;
#33601=ORIENTED_EDGE ( 'NONE', *, *, #29265, .F. ) ;
#33607=CARTESIAN_POINT ( 'NONE',  ( -208.4459734468149463, 0.000000000000000000, 82.56828755692798438 ) ) ;
#33611=CARTESIAN_POINT ( 'NONE',  ( 194.3291528190321742, -1.750000000000009326, 1.843413822775066269 ) ) ;
#33613=( BOUNDED_CURVE ( )  B_SPLINE_CURVE ( 3, ( #47233, #588, #9031, #28023 ),
 .UNSPECIFIED., .F., .F. ) 
 B_SPLINE_CURVE_WITH_KNOTS ( ( 4, 4 ),
 ( 1.570796326794896558, 3.141592653589793116 ),
 .UNSPECIFIED. ) 
 CURVE ( )  GEOMETRIC_REPRESENTATION_ITEM ( )  RATIONAL_B_SPLINE_CURVE ( ( 1.000000000000000000, 0.8047378541243649375, 0.8047378541243649375, 1.000000000000000000 ) ) 
 REPRESENTATION_ITEM ( '' )  );
#33615=LINE ( 'NONE', #2297, #24298 ) ;
#33619=CYLINDRICAL_SURFACE ( 'NONE', #29742, 1.750000000000008438 ) ;
#33624=CARTESIAN_POINT ( 'NONE',  ( -126.6959734468149321, 1.749999999999997335, 120.8182875569279702 ) ) ;
#33628=DIRECTION ( 'NONE',  ( -1.000000000000000000, 0.000000000000000000, 0.000000000000000000 ) ) ;
#33640=VERTEX_POINT ( 'NONE', #11166 ) ;
#33642=VECTOR ( 'NONE', #12294, 1000.000000000000000 ) ;
#33645=DIRECTION ( 'NONE',  ( 0.000000000000000000, 0.000000000000000000, 1.000000000000000000 ) ) ;
#33646=DIRECTION ( 'NONE',  ( 0.000000000000000000, 0.000000000000000000, 1.000000000000000000 ) ) ;
#33647=CARTESIAN_POINT ( 'NONE',  ( 75.05402655318509630, 2.143131898507880377E-16, 159.0682875569279702 ) ) ;
#33662=CARTESIAN_POINT ( 'NONE',  ( -168.4459734468149463, 0.000000000000000000, -120.9317124430720156 ) ) ;
#33663=CARTESIAN_POINT ( 'NONE',  ( 210.0000000000000568, 0.000000000000000000, -79.18171244307201562 ) ) ;
#33664=CARTESIAN_POINT ( 'NONE',  ( -128.4459734468149179, 0.000000000000000000, 159.0682875569279986 ) ) ;
#33665=( BOUNDED_CURVE ( )  B_SPLINE_CURVE ( 3, ( #31220, #4761, #7609, #667 ),
 .UNSPECIFIED., .F., .F. ) 
 B_SPLINE_CURVE_WITH_KNOTS ( ( 4, 4 ),
 ( 0.000000000000000000, 1.570796326794896558 ),
 .UNSPECIFIED. ) 
 CURVE ( )  GEOMETRIC_REPRESENTATION_ITEM ( )  RATIONAL_B_SPLINE_CURVE ( ( 1.000000000000000000, 0.8047378541243649375, 0.8047378541243649375, 1.000000000000000000 ) ) 
 REPRESENTATION_ITEM ( '' )  );
#33667=ORIENTED_EDGE ( 'NONE', *, *, #11444, .T. ) ;
#33673=( BOUNDED_CURVE ( )  B_SPLINE_CURVE ( 3, ( #13039, #33070, #13289, #1267 ),
 .UNSPECIFIED., .F., .F. ) 
 B_SPLINE_CURVE_WITH_KNOTS ( ( 4, 4 ),
 ( 0.000000000000000000, 1.570796326794896558 ),
 .UNSPECIFIED. ) 
 CURVE ( )  GEOMETRIC_REPRESENTATION_ITEM ( )  RATIONAL_B_SPLINE_CURVE ( ( 1.000000000000000000, 0.8047378541243649375, 0.8047378541243649375, 1.000000000000000000 ) ) 
 REPRESENTATION_ITEM ( '' )  );
#33676=ORIENTED_EDGE ( 'NONE', *, *, #24401, .T. ) ;
#33686=FACE_OUTER_BOUND ( 'NONE', #50182, .T. ) ;
#33688=CARTESIAN_POINT ( 'NONE',  ( 210.0000000000000568, 0.000000000000000000, -77.43171244307200141 ) ) ;
#33694=DIRECTION ( 'NONE',  ( -1.000000000000000000, 0.000000000000000000, 0.000000000000000000 ) ) ;
#33695=ORIENTED_EDGE ( 'NONE', *, *, #858, .T. ) ;
#33698=FACE_OUTER_BOUND ( 'NONE', #42257, .T. ) ;
#33699=DIRECTION ( 'NONE',  ( 0.000000000000000000, 0.000000000000000000, 1.000000000000000000 ) ) ;
#33701=CARTESIAN_POINT ( 'NONE',  ( -8.445973446814976526, 0.000000000000000000, -40.93171244307205825 ) ) ;
#33709=CARTESIAN_POINT ( 'NONE',  ( 153.3040265531850537, 1.750000000000010658, -79.18171244307201562 ) ) ;
#33714=EDGE_LOOP ( 'NONE', ( #5478, #42163, #29589, #14578, #44402, #30173 ) ) ;
#33716=DIRECTION ( 'NONE',  ( -0.000000000000000000, -0.000000000000000000, -1.000000000000000000 ) ) ;
#33721=CARTESIAN_POINT ( 'NONE',  ( 75.05402655318509630, -1.025126265847089435, 162.5682875569279133 ) ) ;
#33724=ORIENTED_EDGE ( 'NONE', *, *, #25001, .F. ) ;
#33737=CARTESIAN_POINT ( 'NONE',  ( -48.44597344681496054, -1.025126265847089657, -37.43171244307202272 ) ) ;
#33741=EDGE_CURVE ( 'NONE', #49918, #7079, #16532, .T. ) ;
#33743=CARTESIAN_POINT ( 'NONE',  ( 71.55402655318505367, 0.000000000000000000, -40.93171244307205825 ) ) ;
#33744=ORIENTED_EDGE ( 'NONE', *, *, #18348, .T. ) ;
#33749=DIRECTION ( 'NONE',  ( 1.000000000000000000, 0.000000000000000000, 0.000000000000000000 ) ) ;
#33754=FACE_OUTER_BOUND ( 'NONE', #32070, .T. ) ;
#33755=CARTESIAN_POINT ( 'NONE',  ( -166.6959734468149463, -1.750000000000010658, -119.1817124430720440 ) ) ;
#33756=CARTESIAN_POINT ( 'NONE',  ( 153.3040265531850537, -1.750000000000009992, 160.8182875569279702 ) ) ;
#33758=VECTOR ( 'NONE', #8075, 1000.000000000000000 ) ;
#33763=ORIENTED_EDGE ( 'NONE', *, *, #27378, .F. ) ;
#33765=EDGE_CURVE ( 'NONE', #14506, #23447, #862, .T. ) ;
#33767=CARTESIAN_POINT ( 'NONE',  ( 155.0540265531850537, 2.143131898507880377E-16, 165.0000000000000000 ) ) ;
#33770=CARTESIAN_POINT ( 'NONE',  ( -48.44597344681495343, 0.000000000000000000, 39.06828755692798438 ) ) ;
#33779=CARTESIAN_POINT ( 'NONE',  ( 113.3040265531850537, 0.000000000000000000, 165.0000000000000000 ) ) ;
#33784=ORIENTED_EDGE ( 'NONE', *, *, #28505, .F. ) ;
#33787=CARTESIAN_POINT ( 'NONE',  ( -208.4459734468148611, 1.025126265847089657, -120.9317124430720440 ) ) ;
#33795=ORIENTED_EDGE ( 'NONE', *, *, #34275, .T. ) ;
#33796=VERTEX_POINT ( 'NONE', #39897 ) ;
#33798=CARTESIAN_POINT ( 'NONE',  ( -206.6959734468149463, 0.000000000000000000, 165.0000000000000000 ) ) ;
#33806=CARTESIAN_POINT ( 'NONE',  ( -44.94597344681493922, 2.143131898507880377E-16, 159.0682875569279702 ) ) ;
#33811=DIRECTION ( 'NONE',  ( 0.000000000000000000, 0.000000000000000000, 1.000000000000000000 ) ) ;
#33813=( BOUNDED_CURVE ( )  B_SPLINE_CURVE ( 3, ( #3114, #45687, #2854, #17771 ),
 .UNSPECIFIED., .F., .F. ) 
 B_SPLINE_CURVE_WITH_KNOTS ( ( 4, 4 ),
 ( 0.000000000000000000, 1.570796326794896558 ),
 .UNSPECIFIED. ) 
 CURVE ( )  GEOMETRIC_REPRESENTATION_ITEM ( )  RATIONAL_B_SPLINE_CURVE ( ( 1.000000000000000000, 0.8047378541243649375, 0.8047378541243649375, 1.000000000000000000 ) ) 
 REPRESENTATION_ITEM ( '' )  );
#33814=CYLINDRICAL_SURFACE ( 'NONE', #15053, 1.750000000000015543 ) ;
#33817=DIRECTION ( 'NONE',  ( -1.000000000000000000, 0.000000000000000000, 0.000000000000000000 ) ) ;
#33823=DIRECTION ( 'NONE',  ( -1.000000000000000000, -0.000000000000000000, -0.000000000000000000 ) ) ;
#33831=CARTESIAN_POINT ( 'NONE',  ( -166.6959734468149463, 1.750000000000009992, -159.1817124430720298 ) ) ;
#33832=CARTESIAN_POINT ( 'NONE',  ( -44.94597344681493922, 2.143131898507880377E-16, 122.5682875569279702 ) ) ;
#33833=( BOUNDED_CURVE ( )  B_SPLINE_CURVE ( 3, ( #15723, #35498, #20582, #11884 ),
 .UNSPECIFIED., .F., .F. ) 
 B_SPLINE_CURVE_WITH_KNOTS ( ( 4, 4 ),
 ( 4.712388980384689674, 6.283185307179586232 ),
 .UNSPECIFIED. ) 
 CURVE ( )  GEOMETRIC_REPRESENTATION_ITEM ( )  RATIONAL_B_SPLINE_CURVE ( ( 1.000000000000000000, 0.8047378541243649375, 0.8047378541243649375, 1.000000000000000000 ) ) 
 REPRESENTATION_ITEM ( '' )  );
#33839=EDGE_CURVE ( 'NONE', #16057, #25771, #30375, .T. ) ;
#33842=VERTEX_POINT ( 'NONE', #24992 ) ;
#33854=CARTESIAN_POINT ( 'NONE',  ( 210.0000000000000568, 0.000000000000000000, 40.81828755692798438 ) ) ;
#33861=DIRECTION ( 'NONE',  ( -0.000000000000000000, -0.000000000000000000, -1.000000000000000000 ) ) ;
#33862=ORIENTED_EDGE ( 'NONE', *, *, #49636, .T. ) ;
#33864=DIRECTION ( 'NONE',  ( -0.000000000000000000, -0.000000000000000000, -1.000000000000000000 ) ) ;
#33867=CARTESIAN_POINT ( 'NONE',  ( -126.6959734468149321, -1.749999999999997113, 40.81828755692798438 ) ) ;
#33873=EDGE_CURVE ( 'NONE', #45829, #44745, #12668, .T. ) ;
#33874=ORIENTED_EDGE ( 'NONE', *, *, #36594, .F. ) ;
#33878=DIRECTION ( 'NONE',  ( -0.000000000000000000, -0.000000000000000000, -1.000000000000000000 ) ) ;
#33882=CARTESIAN_POINT ( 'NONE',  ( -44.94597344681493922, 2.143131898507880377E-16, -157.4317124430720014 ) ) ;
#33884=CARTESIAN_POINT ( 'NONE',  ( 71.55402655318506788, 2.143131898507880377E-16, -160.9317124430720298 ) ) ;
#33886=CYLINDRICAL_SURFACE ( 'NONE', #24810, 1.750000000000001554 ) ;
#33890=CARTESIAN_POINT ( 'NONE',  ( -8.445973446814964092, -1.025126265847097429, 42.56828755692800570 ) ) ;
#33893=CARTESIAN_POINT ( 'NONE',  ( 33.30402655318503946, 1.750000000000010658, 80.81828755692798438 ) ) ;
#33896=CARTESIAN_POINT ( 'NONE',  ( -126.6959734468149321, 1.749999999999997335, 120.8182875569279702 ) ) ;
#33900=CARTESIAN_POINT ( 'NONE',  ( -165.6708471809677974, -1.750000000000010436, 119.7931612910808781 ) ) ;
#33903=EDGE_CURVE ( 'NONE', #50159, #43847, #48283, .T. ) ;
#33904=CARTESIAN_POINT ( 'NONE',  ( -48.44597344681496054, -1.025126265847089657, -80.93171244307201562 ) ) ;
#33905=ORIENTED_EDGE ( 'NONE', *, *, #40902, .T. ) ;
#33907=CARTESIAN_POINT ( 'NONE',  ( 33.30402655318503946, -1.750000000000010658, 120.8182875569279702 ) ) ;
#33911=CARTESIAN_POINT ( 'NONE',  ( -8.445973446814976526, 0.000000000000000000, -80.93171244307204404 ) ) ;
#33912=( BOUNDED_CURVE ( )  B_SPLINE_CURVE ( 3, ( #25128, #37449, #21512, #21020 ),
 .UNSPECIFIED., .F., .F. ) 
 B_SPLINE_CURVE_WITH_KNOTS ( ( 4, 4 ),
 ( 3.141592653589793116, 4.712388980384689674 ),
 .UNSPECIFIED. ) 
 CURVE ( )  GEOMETRIC_REPRESENTATION_ITEM ( )  RATIONAL_B_SPLINE_CURVE ( ( 1.000000000000000000, 0.8047378541243649375, 0.8047378541243649375, 1.000000000000000000 ) ) 
 REPRESENTATION_ITEM ( '' )  );
#33914=LINE ( 'NONE', #30311, #36044 ) ;
#33918=DIRECTION ( 'NONE',  ( -1.000000000000000000, 0.000000000000000000, 0.000000000000000000 ) ) ;
#33922=VECTOR ( 'NONE', #43599, 1000.000000000000000 ) ;
#33923=ORIENTED_EDGE ( 'NONE', *, *, #13714, .T. ) ;
#33928=EDGE_CURVE ( 'NONE', #12513, #36229, #5726, .T. ) ;
#33936=CARTESIAN_POINT ( 'NONE',  ( -168.4459734468149747, -1.025126265847089657, -120.9317124430720440 ) ) ;
#33942=VECTOR ( 'NONE', #28682, 1000.000000000000000 ) ;
#33946=ORIENTED_EDGE ( 'NONE', *, *, #25726, .F. ) ;
#33947=DIRECTION ( 'NONE',  ( -1.000000000000000000, 0.000000000000000000, 0.000000000000000000 ) ) ;
#33948=LINE ( 'NONE', #6483, #17546 ) ;
#33949=DIRECTION ( 'NONE',  ( -1.000000000000000000, -0.000000000000000000, -0.000000000000000000 ) ) ;
#33950=EDGE_LOOP ( 'NONE', ( #45412, #40837, #11255, #8679, #40678, #45849 ) ) ;
#33958=ORIENTED_EDGE ( 'NONE', *, *, #24404, .F. ) ;
#33959=EDGE_LOOP ( 'NONE', ( #20694, #13826, #39380, #39476, #36746, #13076 ) ) ;
#33960=CARTESIAN_POINT ( 'NONE',  ( -208.4459734468149463, 0.000000000000000000, 162.5682875569279702 ) ) ;
#33961=AXIS2_PLACEMENT_3D ( 'NONE', #47187, #12084, #31848 ) ;
#33963=( BOUNDED_CURVE ( )  B_SPLINE_CURVE ( 3, ( #15713, #34992, #30612, #31385 ),
 .UNSPECIFIED., .F., .F. ) 
 B_SPLINE_CURVE_WITH_KNOTS ( ( 4, 4 ),
 ( 3.141592653589793116, 4.712388980384689674 ),
 .UNSPECIFIED. ) 
 CURVE ( )  GEOMETRIC_REPRESENTATION_ITEM ( )  RATIONAL_B_SPLINE_CURVE ( ( 1.000000000000000000, 0.8047378541243649375, 0.8047378541243649375, 1.000000000000000000 ) ) 
 REPRESENTATION_ITEM ( '' )  );
#33964=VERTEX_POINT ( 'NONE', #5473 ) ;
#33965=ORIENTED_EDGE ( 'NONE', *, *, #30104, .F. ) ;
#33970=CYLINDRICAL_SURFACE ( 'NONE', #27636, 1.750000000000008438 ) ;
#33972=EDGE_CURVE ( 'NONE', #21418, #14525, #35645, .T. ) ;
#33977=CARTESIAN_POINT ( 'NONE',  ( -48.44597344681496054, -1.025126265847089657, -120.9317124430720440 ) ) ;
#33981=VECTOR ( 'NONE', #34376, 1000.000000000000000 ) ;
#33982=CARTESIAN_POINT ( 'NONE',  ( 112.2789002873379758, -1.749999999999996669, 161.8434138227750907 ) ) ;
#33984=ORIENTED_EDGE ( 'NONE', *, *, #39968, .F. ) ;
#33987=EDGE_CURVE ( 'NONE', #21583, #18090, #13272, .T. ) ;
#33988=ORIENTED_EDGE ( 'NONE', *, *, #44672, .F. ) ;
#33990=DIRECTION ( 'NONE',  ( -1.000000000000000000, -0.000000000000000000, -0.000000000000000000 ) ) ;
#33991=ORIENTED_EDGE ( 'NONE', *, *, #35597, .T. ) ;
#33992=CARTESIAN_POINT ( 'NONE',  ( -47.72109971266203132, -1.750000000000010214, -78.15658617722490931 ) ) ;
#33993=ADVANCED_FACE ( 'NONE', ( #21374 ), #17285, .T. ) ;
#33998=AXIS2_PLACEMENT_3D ( 'NONE', #9849, #25502, #30114 ) ;
#33999=CARTESIAN_POINT ( 'NONE',  ( 31.55402655318503236, 1.025126265847089435, -77.43171244307200141 ) ) ;
#34002=EDGE_CURVE ( 'NONE', #37518, #10906, #7247, .T. ) ;
#34004=CYLINDRICAL_SURFACE ( 'NONE', #8085, 1.750000000000008438 ) ;
#34006=AXIS2_PLACEMENT_3D ( 'NONE', #18309, #13962, #22426 ) ;
#34008=FACE_OUTER_BOUND ( 'NONE', #33319, .T. ) ;
#34011=ADVANCED_FACE ( 'NONE', ( #2622 ), #18775, .T. ) ;
#34015=AXIS2_PLACEMENT_3D ( 'NONE', #37942, #2258, #5598 ) ;
#34016=ADVANCED_FACE ( 'NONE', ( #49287 ), #22890, .T. ) ;
#34017=ADVANCED_FACE ( 'NONE', ( #41637 ), #14439, .T. ) ;
#34018=CARTESIAN_POINT ( 'NONE',  ( -6.695973446814940111, -1.750000000000023759, 40.81828755692798438 ) ) ;
#34024=EDGE_LOOP ( 'NONE', ( #3896, #43722, #42472, #1099, #48803, #10900 ) ) ;
#34028=CARTESIAN_POINT ( 'NONE',  ( -48.44597344681496054, 1.025126265847089213, -0.9317124430720324924 ) ) ;
#34030=EDGE_LOOP ( 'NONE', ( #31980, #44657, #29248, #44519, #32852 ) ) ;
#34033=CARTESIAN_POINT ( 'NONE',  ( 32.27890028733795447, 1.750000000000009548, -0.2068387089191121020 ) ) ;
#34037=ORIENTED_EDGE ( 'NONE', *, *, #46296, .T. ) ;
#34041=CARTESIAN_POINT ( 'NONE',  ( 210.0000000000000568, 0.000000000000000000, 80.81828755692798438 ) ) ;
#34053=ORIENTED_EDGE ( 'NONE', *, *, #5264, .F. ) ;
#34054=CARTESIAN_POINT ( 'NONE',  ( -5.670847180967843570, -1.750000000000023315, -38.15658617722493062 ) ) ;
#34058=CYLINDRICAL_SURFACE ( 'NONE', #18639, 1.750000000000010214 ) ;
#34059=DIRECTION ( 'NONE',  ( -1.000000000000000000, 0.000000000000000000, 0.000000000000000000 ) ) ;
#34063=VERTEX_POINT ( 'NONE', #34209 ) ;
#34065=DIRECTION ( 'NONE',  ( 0.000000000000000000, 0.000000000000000000, -1.000000000000000000 ) ) ;
#34067=CARTESIAN_POINT ( 'NONE',  ( -45.67084718096785423, 1.750000000000009548, -160.2068387089191219 ) ) ;
#34080=ORIENTED_EDGE ( 'NONE', *, *, #247, .T. ) ;
#34081=DIRECTION ( 'NONE',  ( -1.000000000000000000, 0.000000000000000000, 0.000000000000000000 ) ) ;
#34088=DIRECTION ( 'NONE',  ( -1.000000000000000000, -0.000000000000000000, -0.000000000000000000 ) ) ;
#34101=ADVANCED_FACE ( 'NONE', ( #33698 ), #45453, .T. ) ;
#34103=ORIENTED_EDGE ( 'NONE', *, *, #40941, .T. ) ;
#34104=CYLINDRICAL_SURFACE ( 'NONE', #34676, 1.750000000000001554 ) ;
#34105=CARTESIAN_POINT ( 'NONE',  ( -128.4459734468149179, 0.000000000000000000, -40.93171244307202983 ) ) ;
#34108=CARTESIAN_POINT ( 'NONE',  ( 155.0540265531850537, 2.143131898507880377E-16, 165.0000000000000000 ) ) ;
#34110=ORIENTED_EDGE ( 'NONE', *, *, #39367, .T. ) ;
#34118=CARTESIAN_POINT ( 'NONE',  ( -208.4459734468148611, 1.025126265847089213, -0.9317124430720324924 ) ) ;
#34120=( BOUNDED_CURVE ( )  B_SPLINE_CURVE ( 3, ( #18943, #23053, #2794, #3815 ),
 .UNSPECIFIED., .F., .F. ) 
 B_SPLINE_CURVE_WITH_KNOTS ( ( 4, 4 ),
 ( 1.570796326794896558, 3.141592653589793116 ),
 .UNSPECIFIED. ) 
 CURVE ( )  GEOMETRIC_REPRESENTATION_ITEM ( )  RATIONAL_B_SPLINE_CURVE ( ( 1.000000000000000000, 0.8047378541243649375, 0.8047378541243649375, 1.000000000000000000 ) ) 
 REPRESENTATION_ITEM ( '' )  );
#34123=DIRECTION ( 'NONE',  ( 0.000000000000000000, 0.000000000000000000, 1.000000000000000000 ) ) ;
#34126=ORIENTED_EDGE ( 'NONE', *, *, #39339, .F. ) ;
#34128=( BOUNDED_CURVE ( )  B_SPLINE_CURVE ( 3, ( #6298, #10890, #13973, #21678 ),
 .UNSPECIFIED., .F., .F. ) 
 B_SPLINE_CURVE_WITH_KNOTS ( ( 4, 4 ),
 ( 1.570796326794896558, 3.141592653589793116 ),
 .UNSPECIFIED. ) 
 CURVE ( )  GEOMETRIC_REPRESENTATION_ITEM ( )  RATIONAL_B_SPLINE_CURVE ( ( 1.000000000000000000, 0.8047378541243649375, 0.8047378541243649375, 1.000000000000000000 ) ) 
 REPRESENTATION_ITEM ( '' )  );
#34129=ADVANCED_FACE ( 'NONE', ( #326 ), #31106, .T. ) ;
#34130=LINE ( 'NONE', #26152, #16630 ) ;
#34134=ADVANCED_FACE ( 'NONE', ( #31631 ), #47220, .T. ) ;
#34135=CARTESIAN_POINT ( 'NONE',  ( -204.9459734468149463, 2.143131898507880377E-16, -40.93171244307202983 ) ) ;
#34139=CARTESIAN_POINT ( 'NONE',  ( 111.5540265531850537, 1.025126265847081219, 2.568287556927973281 ) ) ;
#34140=VECTOR ( 'NONE', #9053, 1000.000000000000000 ) ;
#34147=( BOUNDED_CURVE ( )  B_SPLINE_CURVE ( 3, ( #28543, #6208, #1355, #13878 ),
 .UNSPECIFIED., .F., .F. ) 
 B_SPLINE_CURVE_WITH_KNOTS ( ( 4, 4 ),
 ( 4.712388980384689674, 6.283185307179586232 ),
 .UNSPECIFIED. ) 
 CURVE ( )  GEOMETRIC_REPRESENTATION_ITEM ( )  RATIONAL_B_SPLINE_CURVE ( ( 1.000000000000000000, 0.8047378541243649375, 0.8047378541243649375, 1.000000000000000000 ) ) 
 REPRESENTATION_ITEM ( '' )  );
#34150=CARTESIAN_POINT ( 'NONE',  ( 111.5540265531850537, 1.025126265847081664, 82.56828755692798438 ) ) ;
#34155=FACE_OUTER_BOUND ( 'NONE', #11596, .T. ) ;
#34157=VERTEX_POINT ( 'NONE', #11610 ) ;
#34159=CARTESIAN_POINT ( 'NONE',  ( 34.32915281903212446, 1.750000000000010214, -80.20683870891910772 ) ) ;
#34162=EDGE_LOOP ( 'NONE', ( #9523, #31963, #1546, #4038, #6417, #31720 ) ) ;
#34168=CARTESIAN_POINT ( 'NONE',  ( 191.5540265531851105, 0.000000000000000000, -157.4317124430720582 ) ) ;
#34169=VERTEX_POINT ( 'NONE', #39574 ) ;
#34178=CARTESIAN_POINT ( 'NONE',  ( -5.670847180967843570, -1.750000000000023315, 81.84341382277507648 ) ) ;
#34179=ORIENTED_EDGE ( 'NONE', *, *, #43986, .T. ) ;
#34183=CARTESIAN_POINT ( 'NONE',  ( -4.945973446814903696, 2.143131898507912917E-16, 165.0000000000000000 ) ) ;
#34184=EDGE_CURVE ( 'NONE', #5777, #16313, #43395, .T. ) ;
#34189=ORIENTED_EDGE ( 'NONE', *, *, #12176, .T. ) ;
#34192=EDGE_CURVE ( 'NONE', #45821, #14015, #7753, .T. ) ;
#34202=CARTESIAN_POINT ( 'NONE',  ( -165.6708471809677974, 1.750000000000009548, 1.843413822775065825 ) ) ;
#34204=LINE ( 'NONE', #49778, #6943 ) ;
#34205=VECTOR ( 'NONE', #10190, 1000.000000000000000 ) ;
#34208=ORIENTED_EDGE ( 'NONE', *, *, #39163, .F. ) ;
#34209=CARTESIAN_POINT ( 'NONE',  ( 113.3040265531850537, -1.749999999999996891, 160.8182875569279702 ) ) ;
#34210=DIRECTION ( 'NONE',  ( 0.000000000000000000, 0.000000000000000000, 1.000000000000000000 ) ) ;
#34211=CARTESIAN_POINT ( 'NONE',  ( -210.0000000000000568, 0.000000000000000000, 120.8182875569279702 ) ) ;
#34212=ORIENTED_EDGE ( 'NONE', *, *, #7513, .F. ) ;
#34213=DIRECTION ( 'NONE',  ( -0.000000000000000000, -0.000000000000000000, -1.000000000000000000 ) ) ;
#34215=DIRECTION ( 'NONE',  ( -0.000000000000000000, -0.000000000000000000, -1.000000000000000000 ) ) ;
#34216=( BOUNDED_CURVE ( )  B_SPLINE_CURVE ( 3, ( #6906, #26146, #37717, #49705 ),
 .UNSPECIFIED., .F., .F. ) 
 B_SPLINE_CURVE_WITH_KNOTS ( ( 4, 4 ),
 ( 0.000000000000000000, 1.570796326794896558 ),
 .UNSPECIFIED. ) 
 CURVE ( )  GEOMETRIC_REPRESENTATION_ITEM ( )  RATIONAL_B_SPLINE_CURVE ( ( 1.000000000000000000, 0.8047378541243649375, 0.8047378541243649375, 1.000000000000000000 ) ) 
 REPRESENTATION_ITEM ( '' )  );
#34217=CYLINDRICAL_SURFACE ( 'NONE', #17993, 1.750000000000001554 ) ;
#34228=CARTESIAN_POINT ( 'NONE',  ( -164.9459734468149463, 2.143131898507880377E-16, -157.4317124430720582 ) ) ;
#34231=ORIENTED_EDGE ( 'NONE', *, *, #32215, .F. ) ;
#34234=EDGE_LOOP ( 'NONE', ( #6177, #33481, #15159, #23024, #41385, #17089 ) ) ;
#34235=AXIS2_PLACEMENT_3D ( 'NONE', #11212, #38928, #26850 ) ;
#34241=ORIENTED_EDGE ( 'NONE', *, *, #1519, .T. ) ;
#34242=DIRECTION ( 'NONE',  ( 0.000000000000000000, 0.000000000000000000, 1.000000000000000000 ) ) ;
#34244=VERTEX_POINT ( 'NONE', #40820 ) ;
#34246=CARTESIAN_POINT ( 'NONE',  ( 115.0540265531850395, -1.025126265847081664, -37.43171244307203693 ) ) ;
#34252=CARTESIAN_POINT ( 'NONE',  ( 152.2789002873379900, -1.750000000000009548, -158.1565861772249377 ) ) ;
#34256=CARTESIAN_POINT ( 'NONE',  ( 71.55402655318505367, 0.000000000000000000, -117.4317124430720156 ) ) ;
#34263=( BOUNDED_CURVE ( )  B_SPLINE_CURVE ( 3, ( #20534, #47943, #31849, #12835 ),
 .UNSPECIFIED., .F., .F. ) 
 B_SPLINE_CURVE_WITH_KNOTS ( ( 4, 4 ),
 ( 4.712388980384689674, 6.283185307179586232 ),
 .UNSPECIFIED. ) 
 CURVE ( )  GEOMETRIC_REPRESENTATION_ITEM ( )  RATIONAL_B_SPLINE_CURVE ( ( 1.000000000000000000, 0.8047378541243649375, 0.8047378541243649375, 1.000000000000000000 ) ) 
 REPRESENTATION_ITEM ( '' )  );
#34264=VECTOR ( 'NONE', #37304, 1000.000000000000000 ) ;
#34269=( BOUNDED_CURVE ( )  B_SPLINE_CURVE ( 3, ( #29894, #45759, #49594, #10897 ),
 .UNSPECIFIED., .F., .F. ) 
 B_SPLINE_CURVE_WITH_KNOTS ( ( 4, 4 ),
 ( 0.000000000000000000, 1.570796326794896780 ),
 .UNSPECIFIED. ) 
 CURVE ( )  GEOMETRIC_REPRESENTATION_ITEM ( )  RATIONAL_B_SPLINE_CURVE ( ( 1.000000000000000000, 0.8047378541243649375, 0.8047378541243649375, 1.000000000000000000 ) ) 
 REPRESENTATION_ITEM ( '' )  );
#34270=ORIENTED_EDGE ( 'NONE', *, *, #12062, .F. ) ;
#34271=ADVANCED_FACE ( 'NONE', ( #32629 ), #5157, .T. ) ;
#34272=ORIENTED_EDGE ( 'NONE', *, *, #3111, .F. ) ;
#34275=EDGE_CURVE ( 'NONE', #40485, #24426, #5665, .T. ) ;
#34279=DIRECTION ( 'NONE',  ( -0.000000000000000000, -0.000000000000000000, -1.000000000000000000 ) ) ;
#34281=ORIENTED_EDGE ( 'NONE', *, *, #6200, .F. ) ;
#34285=CARTESIAN_POINT ( 'NONE',  ( -6.695973446814940111, 0.000000000000000000, 165.0000000000000000 ) ) ;
#34290=VERTEX_POINT ( 'NONE', #9514 ) ;
#34292=CARTESIAN_POINT ( 'NONE',  ( 210.0000000000000568, 0.000000000000000000, -39.18171244307202983 ) ) ;
#34293=DIRECTION ( 'NONE',  ( -1.000000000000000000, -0.000000000000000000, -0.000000000000000000 ) ) ;
#34297=EDGE_CURVE ( 'NONE', #45274, #29268, #37297, .T. ) ;
#34299=CARTESIAN_POINT ( 'NONE',  ( 33.30402655318503946, -1.750000000000010214, -39.18171244307202983 ) ) ;
#34301=ADVANCED_FACE ( 'NONE', ( #21318 ), #20564, .T. ) ;
#34311=DIRECTION ( 'NONE',  ( -1.000000000000000000, -0.000000000000000000, -0.000000000000000000 ) ) ;
#34313=CARTESIAN_POINT ( 'NONE',  ( -125.6708471809678542, 1.749999999999996891, -120.2068387089191219 ) ) ;
#34316=DIRECTION ( 'NONE',  ( 1.000000000000000000, 0.000000000000000000, 0.000000000000000000 ) ) ;
#34317=CARTESIAN_POINT ( 'NONE',  ( -4.945973446814917018, -1.025126265847097207, 39.06828755692796307 ) ) ;
#34318=ORIENTED_EDGE ( 'NONE', *, *, #15333, .F. ) ;
#34319=LINE ( 'NONE', #14812, #24006 ) ;
#34320=CARTESIAN_POINT ( 'NONE',  ( -164.9459734468149463, 2.143131898507880377E-16, -0.9317124430720247208 ) ) ;
#34323=CARTESIAN_POINT ( 'NONE',  ( -48.44597344681495343, 0.000000000000000000, 122.5682875569279702 ) ) ;
#34328=EDGE_CURVE ( 'NONE', #49797, #15554, #39532, .T. ) ;
#34329=EDGE_CURVE ( 'NONE', #35332, #15646, #12969, .T. ) ;
#34333=VECTOR ( 'NONE', #35588, 1000.000000000000000 ) ;
#34334=EDGE_CURVE ( 'NONE', #13192, #6245, #41152, .T. ) ;
#34339=CARTESIAN_POINT ( 'NONE',  ( 210.0000000000000568, 0.000000000000000000, 0.8182875569279768335 ) ) ;
#34343=EDGE_CURVE ( 'NONE', #42077, #30382, #48471, .T. ) ;
#34345=EDGE_CURVE ( 'NONE', #24452, #19705, #32034, .T. ) ;
#34348=ORIENTED_EDGE ( 'NONE', *, *, #482, .T. ) ;
#34349=CARTESIAN_POINT ( 'NONE',  ( -166.6959734468149463, 0.000000000000000000, 165.0000000000000000 ) ) ;
#34357=ORIENTED_EDGE ( 'NONE', *, *, #28495, .F. ) ;
#34359=ORIENTED_EDGE ( 'NONE', *, *, #47236, .T. ) ;
#34360=CARTESIAN_POINT ( 'NONE',  ( -5.670847180967843570, 1.750000000000022871, -158.1565861772249093 ) ) ;
#34365=CARTESIAN_POINT ( 'NONE',  ( -207.7210997126620384, 1.750000000000009548, 81.84341382277507648 ) ) ;
#34366=CARTESIAN_POINT ( 'NONE',  ( 155.0540265531850537, 2.143131898507880377E-16, -0.9317124430720247208 ) ) ;
#34367=EDGE_CURVE ( 'NONE', #28808, #19177, #13852, .T. ) ;
#34369=EDGE_CURVE ( 'NONE', #44745, #15868, #10280, .T. ) ;
#34373=ORIENTED_EDGE ( 'NONE', *, *, #12666, .F. ) ;
#34376=DIRECTION ( 'NONE',  ( -1.000000000000000000, -0.000000000000000000, -0.000000000000000000 ) ) ;
#34378=CARTESIAN_POINT ( 'NONE',  ( 111.5540265531850679, 0.000000000000000000, 42.56828755692795596 ) ) ;
#34379=CARTESIAN_POINT ( 'NONE',  ( 33.30402655318503946, 0.000000000000000000, 165.0000000000000000 ) ) ;
#34380=EDGE_LOOP ( 'NONE', ( #3155, #16481, #13743, #13199, #406, #34126 ) ) ;
#34383=EDGE_CURVE ( 'NONE', #14684, #45714, #8058, .T. ) ;
#34385=FACE_OUTER_BOUND ( 'NONE', #43034, .T. ) ;
#34390=ORIENTED_EDGE ( 'NONE', *, *, #34329, .F. ) ;
#34391=CARTESIAN_POINT ( 'NONE',  ( -206.6959734468149463, -1.750000000000009992, 0.8182875569279768335 ) ) ;
#34393=CARTESIAN_POINT ( 'NONE',  ( 75.05402655318509630, 2.143131898507880377E-16, -40.93171244307205825 ) ) ;
#34394=EDGE_CURVE ( 'NONE', #38096, #31646, #41795, .T. ) ;
#34395=VERTEX_POINT ( 'NONE', #29523 ) ;
#34397=CARTESIAN_POINT ( 'NONE',  ( 75.05402655318509630, 2.143131898507880377E-16, -37.43171244307200141 ) ) ;
#34399=DIRECTION ( 'NONE',  ( -0.000000000000000000, -0.000000000000000000, -1.000000000000000000 ) ) ;
#34400=VERTEX_POINT ( 'NONE', #26424 ) ;
#34408=CARTESIAN_POINT ( 'NONE',  ( -7.721099712662037540, -1.750000000000023537, -80.20683870891910772 ) ) ;
#34409=ORIENTED_EDGE ( 'NONE', *, *, #21983, .F. ) ;
#34416=EDGE_CURVE ( 'NONE', #18915, #8241, #17727, .T. ) ;
#34422=EDGE_LOOP ( 'NONE', ( #37411, #16708 ) ) ;
#34424=VECTOR ( 'NONE', #46104, 1000.000000000000000 ) ;
#34425=( BOUNDED_CURVE ( )  B_SPLINE_CURVE ( 3, ( #10889, #26545, #11398, #7050 ),
 .UNSPECIFIED., .F., .F. ) 
 B_SPLINE_CURVE_WITH_KNOTS ( ( 4, 4 ),
 ( 4.712388980384689674, 6.283185307179586232 ),
 .UNSPECIFIED. ) 
 CURVE ( )  GEOMETRIC_REPRESENTATION_ITEM ( )  RATIONAL_B_SPLINE_CURVE ( ( 1.000000000000000000, 0.8047378541243649375, 0.8047378541243649375, 1.000000000000000000 ) ) 
 REPRESENTATION_ITEM ( '' )  );
#34427=CARTESIAN_POINT ( 'NONE',  ( -168.4459734468149463, 0.000000000000000000, 79.06828755692797017 ) ) ;
#34430=CARTESIAN_POINT ( 'NONE',  ( -126.6959734468149321, -1.749999999999997335, -79.18171244307201562 ) ) ;
#34437=( BOUNDED_CURVE ( )  B_SPLINE_CURVE ( 3, ( #45565, #30451, #26603, #10945 ),
 .UNSPECIFIED., .F., .F. ) 
 B_SPLINE_CURVE_WITH_KNOTS ( ( 4, 4 ),
 ( 1.570796326794896558, 3.141592653589793116 ),
 .UNSPECIFIED. ) 
 CURVE ( )  GEOMETRIC_REPRESENTATION_ITEM ( )  RATIONAL_B_SPLINE_CURVE ( ( 1.000000000000000000, 0.8047378541243649375, 0.8047378541243649375, 1.000000000000000000 ) ) 
 REPRESENTATION_ITEM ( '' )  );
#34439=ORIENTED_EDGE ( 'NONE', *, *, #20329, .T. ) ;
#34451=VECTOR ( 'NONE', #49115, 1000.000000000000000 ) ;
#34453=VECTOR ( 'NONE', #30865, 1000.000000000000000 ) ;
#34461=VECTOR ( 'NONE', #27193, 1000.000000000000000 ) ;
#34462=CARTESIAN_POINT ( 'NONE',  ( 210.0000000000000568, 0.000000000000000000, 0.8182875569279768335 ) ) ;
#34465=EDGE_CURVE ( 'NONE', #2997, #21643, #6091, .T. ) ;
#34467=CARTESIAN_POINT ( 'NONE',  ( -164.9459734468149463, -1.025126265847088991, 2.568287556927986159 ) ) ;
#34479=FACE_OUTER_BOUND ( 'NONE', #16248, .T. ) ;
#34480=CARTESIAN_POINT ( 'NONE',  ( 210.0000000000000568, 2.143131898507881856E-16, -120.9317124430720582 ) ) ;
#34481=CARTESIAN_POINT ( 'NONE',  ( 193.3040265531851105, 0.000000000000000000, 165.0000000000000000 ) ) ;
#34485=VERTEX_POINT ( 'NONE', #18973 ) ;
#34487=CARTESIAN_POINT ( 'NONE',  ( -128.4459734468149463, -1.025126265847081886, -40.93171244307202272 ) ) ;
#34491=ORIENTED_EDGE ( 'NONE', *, *, #1448, .T. ) ;
#34494=FACE_OUTER_BOUND ( 'NONE', #8084, .T. ) ;
#34496=DIRECTION ( 'NONE',  ( 0.000000000000000000, 0.000000000000000000, 1.000000000000000000 ) ) ;
#34504=LINE ( 'NONE', #2676, #17231 ) ;
#34505=CARTESIAN_POINT ( 'NONE',  ( -164.9459734468149463, 2.143131898507880377E-16, -120.9317124430720156 ) ) ;
#34506=ORIENTED_EDGE ( 'NONE', *, *, #40715, .T. ) ;
#34509=CARTESIAN_POINT ( 'NONE',  ( 73.30402655318508209, -1.750000000000010214, -39.18171244307202983 ) ) ;
#34515=( BOUNDED_CURVE ( )  B_SPLINE_CURVE ( 3, ( #9791, #25456, #41104, #5947 ),
 .UNSPECIFIED., .F., .F. ) 
 B_SPLINE_CURVE_WITH_KNOTS ( ( 4, 4 ),
 ( 4.712388980384689674, 6.283185307179586232 ),
 .UNSPECIFIED. ) 
 CURVE ( )  GEOMETRIC_REPRESENTATION_ITEM ( )  RATIONAL_B_SPLINE_CURVE ( ( 1.000000000000000000, 0.8047378541243649375, 0.8047378541243649375, 1.000000000000000000 ) ) 
 REPRESENTATION_ITEM ( '' )  );
#34516=CARTESIAN_POINT ( 'NONE',  ( 193.3040265531851105, -1.750000000000010658, 80.81828755692798438 ) ) ;
#34520=AXIS2_PLACEMENT_3D ( 'NONE', #8307, #610, #360 ) ;
#34521=ORIENTED_EDGE ( 'NONE', *, *, #17552, .T. ) ;
#34535=CARTESIAN_POINT ( 'NONE',  ( 195.0540265531851105, -1.025126265847089213, -37.43171244307202272 ) ) ;
#34536=VERTEX_POINT ( 'NONE', #16158 ) ;
#34539=VERTEX_POINT ( 'NONE', #39515 ) ;
#34541=CARTESIAN_POINT ( 'NONE',  ( 210.0000000000000568, 0.000000000000000000, 80.81828755692798438 ) ) ;
#34543=ORIENTED_EDGE ( 'NONE', *, *, #47410, .F. ) ;
#34545=CARTESIAN_POINT ( 'NONE',  ( 74.32915281903215998, 1.750000000000009548, -40.20683870891912193 ) ) ;
#34550=CARTESIAN_POINT ( 'NONE',  ( -48.44597344681496054, 1.025126265847089213, 159.0682875569279418 ) ) ;
#34553=ORIENTED_EDGE ( 'NONE', *, *, #10513, .T. ) ;
#34554=ORIENTED_EDGE ( 'NONE', *, *, #42443, .F. ) ;
#34556=CYLINDRICAL_SURFACE ( 'NONE', #34620, 1.750000000000015543 ) ;
#34557=CARTESIAN_POINT ( 'NONE',  ( 35.05402655318504657, 1.025126265847089879, -117.4317124430720156 ) ) ;
#34559=VECTOR ( 'NONE', #45506, 1000.000000000000000 ) ;
#34565=AXIS2_PLACEMENT_3D ( 'NONE', #34462, #27520, #11349 ) ;
#34569=( BOUNDED_CURVE ( )  B_SPLINE_CURVE ( 3, ( #19447, #15606, #40730, #25080 ),
 .UNSPECIFIED., .F., .F. ) 
 B_SPLINE_CURVE_WITH_KNOTS ( ( 4, 4 ),
 ( 1.570796326794896558, 3.141592653589793116 ),
 .UNSPECIFIED. ) 
 CURVE ( )  GEOMETRIC_REPRESENTATION_ITEM ( )  RATIONAL_B_SPLINE_CURVE ( ( 1.000000000000000000, 0.8047378541243649375, 0.8047378541243649375, 1.000000000000000000 ) ) 
 REPRESENTATION_ITEM ( '' )  );
#34574=FACE_OUTER_BOUND ( 'NONE', #25347, .T. ) ;
#34577=DIRECTION ( 'NONE',  ( -0.000000000000000000, -0.000000000000000000, -1.000000000000000000 ) ) ;
#34582=CARTESIAN_POINT ( 'NONE',  ( -127.7210997126620242, 1.749999999999996669, -78.15658617722492352 ) ) ;
#34587=ORIENTED_EDGE ( 'NONE', *, *, #10891, .F. ) ;
#34588=CARTESIAN_POINT ( 'NONE',  ( 210.0000000000000568, 0.000000000000000000, -39.18171244307202983 ) ) ;
#34589=VERTEX_POINT ( 'NONE', #31314 ) ;
#34594=EDGE_CURVE ( 'NONE', #25029, #47864, #31817, .T. ) ;
#34599=DIRECTION ( 'NONE',  ( 0.000000000000000000, 0.000000000000000000, 1.000000000000000000 ) ) ;
#34601=CARTESIAN_POINT ( 'NONE',  ( -206.6959734468149463, -1.750000000000010658, 80.81828755692798438 ) ) ;
#34604=CARTESIAN_POINT ( 'NONE',  ( 191.5540265531851105, 0.000000000000000000, -40.93171244307202983 ) ) ;
#34609=ADVANCED_FACE ( 'NONE', ( #35424 ), #27451, .T. ) ;
#34610=AXIS2_PLACEMENT_3D ( 'NONE', #20138, #24259, #16552 ) ;
#34611=EDGE_CURVE ( 'NONE', #40582, #37522, #18213, .T. ) ;
#34614=CARTESIAN_POINT ( 'NONE',  ( 31.55402655318503236, -1.025126265847089213, 162.5682875569279133 ) ) ;
#34620=AXIS2_PLACEMENT_3D ( 'NONE', #50139, #39431, #32228 ) ;
#34621=CYLINDRICAL_SURFACE ( 'NONE', #38053, 1.749999999999987566 ) ;
#34623=AXIS2_PLACEMENT_3D ( 'NONE', #29313, #5956, #49264 ) ;
#34624=CARTESIAN_POINT ( 'NONE',  ( -168.4459734468149463, 0.000000000000000000, -40.93171244307202983 ) ) ;
#34626=EDGE_CURVE ( 'NONE', #6992, #36853, #23486, .T. ) ;
#34628=AXIS2_PLACEMENT_3D ( 'NONE', #35738, #16705, #11857 ) ;
#34631=DIRECTION ( 'NONE',  ( -0.000000000000000000, -0.000000000000000000, -1.000000000000000000 ) ) ;
#34637=ORIENTED_EDGE ( 'NONE', *, *, #27958, .T. ) ;
#34645=ORIENTED_EDGE ( 'NONE', *, *, #3267, .T. ) ;
#34646=DIRECTION ( 'NONE',  ( -1.000000000000000000, 0.000000000000000000, 0.000000000000000000 ) ) ;
#34648=CARTESIAN_POINT ( 'NONE',  ( 194.3291528190321742, -1.750000000000009548, 39.79316129108089228 ) ) ;
#34653=CARTESIAN_POINT ( 'NONE',  ( 153.3040265531850537, 1.750000000000009992, 160.8182875569279702 ) ) ;
#34659=DIRECTION ( 'NONE',  ( 0.000000000000000000, 0.000000000000000000, 1.000000000000000000 ) ) ;
#34663=ORIENTED_EDGE ( 'NONE', *, *, #25508, .T. ) ;
#34665=DIRECTION ( 'NONE',  ( -1.000000000000000000, -0.000000000000000000, -0.000000000000000000 ) ) ;
#34669=ORIENTED_EDGE ( 'NONE', *, *, #44613, .T. ) ;
#34673=ADVANCED_FACE ( 'NONE', ( #13295 ), #14557, .T. ) ;
#34674=DIRECTION ( 'NONE',  ( -1.000000000000000000, -0.000000000000000000, -0.000000000000000000 ) ) ;
#34676=AXIS2_PLACEMENT_3D ( 'NONE', #34349, #45841, #10727 ) ;
#34679=ORIENTED_EDGE ( 'NONE', *, *, #17032, .F. ) ;
#34680=DIRECTION ( 'NONE',  ( 1.000000000000000000, 0.000000000000000000, 0.000000000000000000 ) ) ;
#34681=LINE ( 'NONE', #6446, #30037 ) ;
#34685=DIRECTION ( 'NONE',  ( 0.000000000000000000, 0.000000000000000000, 1.000000000000000000 ) ) ;
#34686=CARTESIAN_POINT ( 'NONE',  ( 113.3040265531850537, 1.749999999999996891, 160.8182875569279702 ) ) ;
#34692=CARTESIAN_POINT ( 'NONE',  ( 111.5540265531850679, 0.000000000000000000, 2.568287556927950632 ) ) ;
#34697=CARTESIAN_POINT ( 'NONE',  ( 31.55402655318503236, 0.000000000000000000, -120.9317124430720725 ) ) ;
#34700=EDGE_CURVE ( 'NONE', #30887, #24424, #20176, .T. ) ;
#34701=EDGE_CURVE ( 'NONE', #44745, #35393, #25426, .T. ) ;
#34709=AXIS2_PLACEMENT_3D ( 'NONE', #18828, #29887, #10395 ) ;
#34711=CYLINDRICAL_SURFACE ( 'NONE', #22859, 1.750000000000001554 ) ;
#34716=VERTEX_POINT ( 'NONE', #34323 ) ;
#34718=CARTESIAN_POINT ( 'NONE',  ( -6.695973446814940111, 0.000000000000000000, -165.0000000000000000 ) ) ;
#34723=DIRECTION ( 'NONE',  ( -1.000000000000000000, -0.000000000000000000, -0.000000000000000000 ) ) ;
#34725=( BOUNDED_CURVE ( )  B_SPLINE_CURVE ( 3, ( #18717, #32014, #28155, #31764 ),
 .UNSPECIFIED., .F., .F. ) 
 B_SPLINE_CURVE_WITH_KNOTS ( ( 4, 4 ),
 ( 3.141592653589793116, 4.712388980384689674 ),
 .UNSPECIFIED. ) 
 CURVE ( )  GEOMETRIC_REPRESENTATION_ITEM ( )  RATIONAL_B_SPLINE_CURVE ( ( 1.000000000000000000, 0.8047378541243649375, 0.8047378541243649375, 1.000000000000000000 ) ) 
 REPRESENTATION_ITEM ( '' )  );
#34732=CARTESIAN_POINT ( 'NONE',  ( -206.6959734468149463, -1.750000000000009992, 0.8182875569279768335 ) ) ;
#34733=DIRECTION ( 'NONE',  ( -0.000000000000000000, -0.000000000000000000, -1.000000000000000000 ) ) ;
#34734=( BOUNDED_CURVE ( )  B_SPLINE_CURVE ( 3, ( #1566, #10270, #21305, #37734 ),
 .UNSPECIFIED., .F., .F. ) 
 B_SPLINE_CURVE_WITH_KNOTS ( ( 4, 4 ),
 ( 3.141592653589793116, 4.712388980384689674 ),
 .UNSPECIFIED. ) 
 CURVE ( )  GEOMETRIC_REPRESENTATION_ITEM ( )  RATIONAL_B_SPLINE_CURVE ( ( 1.000000000000000000, 0.8047378541243649375, 0.8047378541243649375, 1.000000000000000000 ) ) 
 REPRESENTATION_ITEM ( '' )  );
#34742=DIRECTION ( 'NONE',  ( -0.000000000000000000, -0.000000000000000000, -1.000000000000000000 ) ) ;
#34743=VECTOR ( 'NONE', #6189, 1000.000000000000000 ) ;
#34748=VERTEX_POINT ( 'NONE', #30213 ) ;
#34750=( BOUNDED_CURVE ( )  B_SPLINE_CURVE ( 3, ( #7591, #46792, #38907, #45787 ),
 .UNSPECIFIED., .F., .F. ) 
 B_SPLINE_CURVE_WITH_KNOTS ( ( 4, 4 ),
 ( 1.570796326794896558, 3.141592653589793116 ),
 .UNSPECIFIED. ) 
 CURVE ( )  GEOMETRIC_REPRESENTATION_ITEM ( )  RATIONAL_B_SPLINE_CURVE ( ( 1.000000000000000000, 0.8047378541243649375, 0.8047378541243649375, 1.000000000000000000 ) ) 
 REPRESENTATION_ITEM ( '' )  );
#34754=ORIENTED_EDGE ( 'NONE', *, *, #17032, .T. ) ;
#34756=ORIENTED_EDGE ( 'NONE', *, *, #27985, .T. ) ;
#34757=CARTESIAN_POINT ( 'NONE',  ( -8.445973446814914354, 0.000000000000000000, 162.5682875569279702 ) ) ;
#34765=CARTESIAN_POINT ( 'NONE',  ( 71.55402655318505367, 0.000000000000000000, 122.5682875569279844 ) ) ;
#34766=CARTESIAN_POINT ( 'NONE',  ( 73.30402655318508209, -1.750000000000010658, -119.1817124430720440 ) ) ;
#34767=CARTESIAN_POINT ( 'NONE',  ( -88.44597344681497475, 0.000000000000000000, -37.43171244307200141 ) ) ;
#34770=ADVANCED_FACE ( 'NONE', ( #9958 ), #6109, .T. ) ;
#34773=ORIENTED_EDGE ( 'NONE', *, *, #4909, .F. ) ;
#34778=CARTESIAN_POINT ( 'NONE',  ( 113.3040265531850537, 0.000000000000000000, 165.0000000000000000 ) ) ;
#34789=CYLINDRICAL_SURFACE ( 'NONE', #46746, 1.750000000000015543 ) ;
#34790=AXIS2_PLACEMENT_3D ( 'NONE', #3354, #18743, #33918 ) ;
#34792=CARTESIAN_POINT ( 'NONE',  ( 113.3040265531850537, -1.749999999999996891, -159.1817124430720298 ) ) ;
#34794=DIRECTION ( 'NONE',  ( -1.000000000000000000, -0.000000000000000000, -0.000000000000000000 ) ) ;
#34796=ORIENTED_EDGE ( 'NONE', *, *, #39324, .F. ) ;
#34797=CYLINDRICAL_SURFACE ( 'NONE', #46336, 1.750000000000001554 ) ;
#34798=CARTESIAN_POINT ( 'NONE',  ( 73.30402655318508209, -1.750000000000010658, 120.8182875569279702 ) ) ;
#34806=AXIS2_PLACEMENT_3D ( 'NONE', #23717, #27576, #43703 ) ;
#34809=EDGE_CURVE ( 'NONE', #9595, #36017, #568, .T. ) ;
#34811=CARTESIAN_POINT ( 'NONE',  ( -46.69597344681494633, -1.750000000000009992, -159.1817124430720298 ) ) ;
#34814=DIRECTION ( 'NONE',  ( -1.000000000000000000, 0.000000000000000000, 0.000000000000000000 ) ) ;
#34817=ORIENTED_EDGE ( 'NONE', *, *, #24668, .T. ) ;
#34819=CARTESIAN_POINT ( 'NONE',  ( 210.0000000000000568, 0.000000000000000000, 160.8182875569279702 ) ) ;
#34820=CARTESIAN_POINT ( 'NONE',  ( -128.4459734468149463, -1.025126265847081442, 162.5682875569279133 ) ) ;
#34823=ORIENTED_EDGE ( 'NONE', *, *, #852, .T. ) ;
#34824=VECTOR ( 'NONE', #20155, 1000.000000000000000 ) ;
#34825=CARTESIAN_POINT ( 'NONE',  ( 192.2789002873380184, 1.750000000000010436, 119.7931612910808781 ) ) ;
#34834=CARTESIAN_POINT ( 'NONE',  ( 210.0000000000000568, 0.000000000000000000, 0.8182875569279768335 ) ) ;
#34836=DIRECTION ( 'NONE',  ( -1.000000000000000000, 0.000000000000000000, 0.000000000000000000 ) ) ;
#34837=EDGE_CURVE ( 'NONE', #4803, #38537, #4151, .T. ) ;
#34838=AXIS2_PLACEMENT_3D ( 'NONE', #41124, #32677, #1135 ) ;
#34839=EDGE_LOOP ( 'NONE', ( #35043, #48306, #6072, #19878, #4250, #43279 ) ) ;
#34840=EDGE_CURVE ( 'NONE', #37272, #42411, #49943, .T. ) ;
#34842=CARTESIAN_POINT ( 'NONE',  ( 33.30402655318503946, -1.750000000000010658, 80.81828755692798438 ) ) ;
#34843=CARTESIAN_POINT ( 'NONE',  ( 153.3040265531850537, 1.750000000000010214, 40.81828755692798438 ) ) ;
#34844=EDGE_LOOP ( 'NONE', ( #4249, #40770, #4557, #7292, #49275 ) ) ;
#34855=VERTEX_POINT ( 'NONE', #4977 ) ;
#34861=CARTESIAN_POINT ( 'NONE',  ( 210.0000000000000568, 0.000000000000000000, -79.18171244307201562 ) ) ;
#34864=ORIENTED_EDGE ( 'NONE', *, *, #16278, .T. ) ;
#34866=PLANE ( 'NONE',  #29085 ) ;
#34871=CARTESIAN_POINT ( 'NONE',  ( 75.05402655318509630, 1.025126265847089657, -37.43171244307202272 ) ) ;
#34872=DIRECTION ( 'NONE',  ( -0.000000000000000000, -0.000000000000000000, -1.000000000000000000 ) ) ;
#34873=ORIENTED_EDGE ( 'NONE', *, *, #25535, .F. ) ;
#34881=CARTESIAN_POINT ( 'NONE',  ( -8.445973446814964092, 1.025126265847097429, -120.9317124430720440 ) ) ;
#34884=CARTESIAN_POINT ( 'NONE',  ( -48.44597344681496054, 1.025126265847089213, 42.56828755692799149 ) ) ;
#34885=CARTESIAN_POINT ( 'NONE',  ( 151.5540265531850537, -1.025126265847089879, 82.56828755692798438 ) ) ;
#34890=( BOUNDED_CURVE ( )  B_SPLINE_CURVE ( 3, ( #18175, #46098, #34871, #45352 ),
 .UNSPECIFIED., .F., .F. ) 
 B_SPLINE_CURVE_WITH_KNOTS ( ( 4, 4 ),
 ( 1.570796326794896558, 3.141592653589793116 ),
 .UNSPECIFIED. ) 
 CURVE ( )  GEOMETRIC_REPRESENTATION_ITEM ( )  RATIONAL_B_SPLINE_CURVE ( ( 1.000000000000000000, 0.8047378541243649375, 0.8047378541243649375, 1.000000000000000000 ) ) 
 REPRESENTATION_ITEM ( '' )  );
#34896=CARTESIAN_POINT ( 'NONE',  ( -44.94597344681493922, 2.143131898507880377E-16, 82.56828755692798438 ) ) ;
#34897=CARTESIAN_POINT ( 'NONE',  ( -125.6708471809678542, -1.749999999999996669, 121.8434138227750481 ) ) ;
#34902=CARTESIAN_POINT ( 'NONE',  ( -86.69597344681496054, 0.000000000000000000, 165.0000000000000000 ) ) ;
#34915=VECTOR ( 'NONE', #43071, 1000.000000000000000 ) ;
#34916=EDGE_LOOP ( 'NONE', ( #5001, #15431, #50052, #46755, #48969, #37379 ) ) ;
#34917=CYLINDRICAL_SURFACE ( 'NONE', #39645, 1.750000000000001554 ) ;
#34918=ORIENTED_EDGE ( 'NONE', *, *, #21171, .F. ) ;
#34924=CARTESIAN_POINT ( 'NONE',  ( 210.0000000000000568, 0.000000000000000000, -39.18171244307202983 ) ) ;
#34926=ORIENTED_EDGE ( 'NONE', *, *, #5314, .T. ) ;
#34929=DIRECTION ( 'NONE',  ( 0.000000000000000000, 0.000000000000000000, 1.000000000000000000 ) ) ;
#34931=CARTESIAN_POINT ( 'NONE',  ( -167.7210997126620384, -1.750000000000010214, 119.7931612910808781 ) ) ;
#34933=CARTESIAN_POINT ( 'NONE',  ( 193.3040265531851105, -1.750000000000009992, -159.1817124430720298 ) ) ;
#34945=ORIENTED_EDGE ( 'NONE', *, *, #19577, .F. ) ;
#34949=CARTESIAN_POINT ( 'NONE',  ( -84.94597344681493212, -1.025126265847088991, 2.568287556927986159 ) ) ;
#34955=CARTESIAN_POINT ( 'NONE',  ( -127.7210997126620242, -1.749999999999996669, -160.2068387089191219 ) ) ;
#34963=EDGE_CURVE ( 'NONE', #35915, #37221, #44464, .T. ) ;
#34966=CARTESIAN_POINT ( 'NONE',  ( -48.44597344681495343, 0.000000000000000000, 165.0000000000000000 ) ) ;
#34968=CYLINDRICAL_SURFACE ( 'NONE', #40390, 1.749999999999987566 ) ;
#34969=VERTEX_POINT ( 'NONE', #40648 ) ;
#34971=EDGE_CURVE ( 'NONE', #16197, #40485, #21518, .T. ) ;
#34973=CARTESIAN_POINT ( 'NONE',  ( 210.0000000000000568, 0.000000000000000000, -159.1817124430720298 ) ) ;
#34988=LINE ( 'NONE', #18275, #13114 ) ;
#34992=CARTESIAN_POINT ( 'NONE',  ( 155.0540265531850537, -1.025126265847089435, -77.43171244307200141 ) ) ;
#34993=CARTESIAN_POINT ( 'NONE',  ( 210.0000000000000568, 0.000000000000000000, -39.18171244307202983 ) ) ;
#34994=ORIENTED_EDGE ( 'NONE', *, *, #50578, .T. ) ;
#35001=EDGE_LOOP ( 'NONE', ( #28429, #41026 ) ) ;
#35003=CARTESIAN_POINT ( 'NONE',  ( 195.0540265531851105, 1.025126265847089657, -120.9317124430720440 ) ) ;
#35004=LINE ( 'NONE', #3922, #7090 ) ;
#35008=EDGE_CURVE ( 'NONE', #8469, #42421, #40854, .T. ) ;
#35010=EDGE_CURVE ( 'NONE', #38333, #10859, #46057, .T. ) ;
#35013=CARTESIAN_POINT ( 'NONE',  ( -167.7210997126620384, 1.750000000000010436, -80.20683870891910772 ) ) ;
#35022=CARTESIAN_POINT ( 'NONE',  ( 194.3291528190321742, 1.750000000000009548, 39.79316129108089228 ) ) ;
#35023=EDGE_LOOP ( 'NONE', ( #7785, #18494, #3476, #35551, #20015 ) ) ;
#35026=DIRECTION ( 'NONE',  ( 1.000000000000000000, 0.000000000000000000, 0.000000000000000000 ) ) ;
#35030=EDGE_CURVE ( 'NONE', #39708, #43597, #22150, .T. ) ;
#35032=DIRECTION ( 'NONE',  ( -1.000000000000000000, -0.000000000000000000, -0.000000000000000000 ) ) ;
#35037=CARTESIAN_POINT ( 'NONE',  ( 192.2789002873380184, -1.750000000000009548, 41.84341382277508359 ) ) ;
#35039=CYLINDRICAL_SURFACE ( 'NONE', #34806, 1.750000000000008438 ) ;
#35040=( BOUNDED_CURVE ( )  B_SPLINE_CURVE ( 3, ( #32742, #2446, #37115, #18085 ),
 .UNSPECIFIED., .F., .F. ) 
 B_SPLINE_CURVE_WITH_KNOTS ( ( 4, 4 ),
 ( 4.712388980384689674, 6.283185307179586232 ),
 .UNSPECIFIED. ) 
 CURVE ( )  GEOMETRIC_REPRESENTATION_ITEM ( )  RATIONAL_B_SPLINE_CURVE ( ( 1.000000000000000000, 0.8047378541243649375, 0.8047378541243649375, 1.000000000000000000 ) ) 
 REPRESENTATION_ITEM ( '' )  );
#35043=ORIENTED_EDGE ( 'NONE', *, *, #20620, .F. ) ;
#35046=( BOUNDED_CURVE ( )  B_SPLINE_CURVE ( 3, ( #27391, #19688, #19932, #8660 ),
 .UNSPECIFIED., .F., .F. ) 
 B_SPLINE_CURVE_WITH_KNOTS ( ( 4, 4 ),
 ( 0.000000000000000000, 1.570796326794896558 ),
 .UNSPECIFIED. ) 
 CURVE ( )  GEOMETRIC_REPRESENTATION_ITEM ( )  RATIONAL_B_SPLINE_CURVE ( ( 1.000000000000000000, 0.8047378541243649375, 0.8047378541243649375, 1.000000000000000000 ) ) 
 REPRESENTATION_ITEM ( '' )  );
#35047=CARTESIAN_POINT ( 'NONE',  ( -166.6959734468149463, 1.750000000000009992, -159.1817124430720298 ) ) ;
#35048=ORIENTED_EDGE ( 'NONE', *, *, #12770, .T. ) ;
#35050=ADVANCED_FACE ( 'NONE', ( #18536 ), #49294, .T. ) ;
#35053=( BOUNDED_CURVE ( )  B_SPLINE_CURVE ( 3, ( #42819, #12287, #46640, #46893 ),
 .UNSPECIFIED., .F., .F. ) 
 B_SPLINE_CURVE_WITH_KNOTS ( ( 4, 4 ),
 ( 3.141592653589793116, 4.712388980384689674 ),
 .UNSPECIFIED. ) 
 CURVE ( )  GEOMETRIC_REPRESENTATION_ITEM ( )  RATIONAL_B_SPLINE_CURVE ( ( 1.000000000000000000, 0.8047378541243649375, 0.8047378541243649375, 1.000000000000000000 ) ) 
 REPRESENTATION_ITEM ( '' )  );
#35054=ORIENTED_EDGE ( 'NONE', *, *, #11810, .F. ) ;
#35055=VERTEX_POINT ( 'NONE', #33709 ) ;
#35064=CARTESIAN_POINT ( 'NONE',  ( 111.5540265531850679, 0.000000000000000000, 39.06828755692798438 ) ) ;
#35066=ORIENTED_EDGE ( 'NONE', *, *, #43521, .T. ) ;
#35068=EDGE_CURVE ( 'NONE', #16975, #21335, #44734, .T. ) ;
#35069=EDGE_CURVE ( 'NONE', #16655, #32283, #41896, .T. ) ;
#35076=EDGE_LOOP ( 'NONE', ( #9792, #40416, #20917, #39657, #2971, #45417 ) ) ;
#35079=DIRECTION ( 'NONE',  ( -1.000000000000000000, 0.000000000000000000, 0.000000000000000000 ) ) ;
#35087=CARTESIAN_POINT ( 'NONE',  ( 115.0540265531850395, 2.143131898507847836E-16, 39.06828755692798438 ) ) ;
#35088=DIRECTION ( 'NONE',  ( -1.000000000000000000, -0.000000000000000000, -0.000000000000000000 ) ) ;
#35092=CARTESIAN_POINT ( 'NONE',  ( 192.2789002873380184, -1.750000000000009548, -160.2068387089191219 ) ) ;
#35094=CARTESIAN_POINT ( 'NONE',  ( 115.0540265531850395, 1.025126265847082108, 42.56828755692797017 ) ) ;
#35095=CARTESIAN_POINT ( 'NONE',  ( -126.6959734468149321, 0.000000000000000000, 165.0000000000000000 ) ) ;
#35110=FACE_OUTER_BOUND ( 'NONE', #44359, .T. ) ;
#35115=CARTESIAN_POINT ( 'NONE',  ( -124.9459734468149463, 2.143131898507847836E-16, 42.56828755692795596 ) ) ;
#35116=CARTESIAN_POINT ( 'NONE',  ( 194.3291528190321742, -1.750000000000009548, 121.8434138227750623 ) ) ;
#35121=CARTESIAN_POINT ( 'NONE',  ( -88.44597344681497475, 0.000000000000000000, 159.0682875569279418 ) ) ;
#35122=CARTESIAN_POINT ( 'NONE',  ( 75.05402655318509630, -1.025126265847089657, 79.06828755692797017 ) ) ;
#35123=VERTEX_POINT ( 'NONE', #39088 ) ;
#35124=DIRECTION ( 'NONE',  ( -0.000000000000000000, -0.000000000000000000, -1.000000000000000000 ) ) ;
#35125=EDGE_CURVE ( 'NONE', #22517, #12712, #42494, .T. ) ;
#35126=CARTESIAN_POINT ( 'NONE',  ( 210.0000000000000568, 0.000000000000000000, 40.81828755692798438 ) ) ;
#35128=CARTESIAN_POINT ( 'NONE',  ( 114.3291528190321173, 1.749999999999996669, 159.7931612910809065 ) ) ;
#35129=ORIENTED_EDGE ( 'NONE', *, *, #37535, .F. ) ;
#35133=ORIENTED_EDGE ( 'NONE', *, *, #34343, .T. ) ;
#35134=ORIENTED_EDGE ( 'NONE', *, *, #45528, .T. ) ;
#35144=DIRECTION ( 'NONE',  ( -0.000000000000000000, -0.000000000000000000, -1.000000000000000000 ) ) ;
#35145=CARTESIAN_POINT ( 'NONE',  ( 31.55402655318503236, -1.025126265847089657, -37.43171244307202272 ) ) ;
#35148=CARTESIAN_POINT ( 'NONE',  ( -5.670847180967843570, 1.750000000000023315, -0.2068387089191201234 ) ) ;
#35149=CARTESIAN_POINT ( 'NONE',  ( -168.4459734468149747, -1.025126265847089657, 119.0682875569279560 ) ) ;
#35153=CARTESIAN_POINT ( 'NONE',  ( -126.6959734468149321, -1.749999999999997335, 120.8182875569279702 ) ) ;
#35157=LINE ( 'NONE', #35910, #8127 ) ;
#35158=DIRECTION ( 'NONE',  ( 0.000000000000000000, 0.000000000000000000, 1.000000000000000000 ) ) ;
#35164=ORIENTED_EDGE ( 'NONE', *, *, #20827, .F. ) ;
#35169=FACE_OUTER_BOUND ( 'NONE', #4238, .T. ) ;
#35174=AXIS2_PLACEMENT_3D ( 'NONE', #41691, #45513, #14493 ) ;
#35176=CARTESIAN_POINT ( 'NONE',  ( 192.2789002873380184, 1.750000000000009548, 81.84341382277507648 ) ) ;
#35179=DIRECTION ( 'NONE',  ( -1.000000000000000000, 0.000000000000000000, 0.000000000000000000 ) ) ;
#35190=EDGE_CURVE ( 'NONE', #40604, #46387, #5790, .T. ) ;
#35191=( BOUNDED_CURVE ( )  B_SPLINE_CURVE ( 3, ( #18984, #46149, #25953, #30054 ),
 .UNSPECIFIED., .F., .F. ) 
 B_SPLINE_CURVE_WITH_KNOTS ( ( 4, 4 ),
 ( 0.000000000000000000, 1.570796326794896558 ),
 .UNSPECIFIED. ) 
 CURVE ( )  GEOMETRIC_REPRESENTATION_ITEM ( )  RATIONAL_B_SPLINE_CURVE ( ( 1.000000000000000000, 0.8047378541243649375, 0.8047378541243649375, 1.000000000000000000 ) ) 
 REPRESENTATION_ITEM ( '' )  );
#35193=ORIENTED_EDGE ( 'NONE', *, *, #27163, .T. ) ;
#35197=CARTESIAN_POINT ( 'NONE',  ( 75.05402655318509630, 2.143131898507880377E-16, -77.43171244307198720 ) ) ;
#35200=CARTESIAN_POINT ( 'NONE',  ( -86.69597344681494633, 1.750000000000009992, -159.1817124430720298 ) ) ;
#35203=AXIS2_PLACEMENT_3D ( 'NONE', #18142, #6603, #33817 ) ;
#35208=CARTESIAN_POINT ( 'NONE',  ( 33.30402655318503946, 1.750000000000010658, -119.1817124430720440 ) ) ;
#35215=DIRECTION ( 'NONE',  ( 0.000000000000000000, 0.000000000000000000, 1.000000000000000000 ) ) ;
#35220=CARTESIAN_POINT ( 'NONE',  ( 115.0540265531850395, 2.143131898507847836E-16, -160.9317124430720014 ) ) ;
#35223=CARTESIAN_POINT ( 'NONE',  ( -5.670847180967843570, 1.750000000000023315, 41.84341382277508359 ) ) ;
#35226=CYLINDRICAL_SURFACE ( 'NONE', #34565, 1.750000000000010214 ) ;
#35227=AXIS2_PLACEMENT_3D ( 'NONE', #17232, #21327, #32898 ) ;
#35231=CARTESIAN_POINT ( 'NONE',  ( 31.55402655318503236, 0.000000000000000000, 159.0682875569279702 ) ) ;
#35234=DIRECTION ( 'NONE',  ( -1.000000000000000000, 0.000000000000000000, 0.000000000000000000 ) ) ;
#35237=AXIS2_PLACEMENT_3D ( 'NONE', #25146, #48436, #39793 ) ;
#35240=CARTESIAN_POINT ( 'NONE',  ( -206.6959734468149463, -1.750000000000009992, 160.8182875569279702 ) ) ;
#35252=DIRECTION ( 'NONE',  ( -1.000000000000000000, -0.000000000000000000, -0.000000000000000000 ) ) ;
#35259=CARTESIAN_POINT ( 'NONE',  ( 153.3040265531850537, -1.750000000000010658, -79.18171244307201562 ) ) ;
#35266=VECTOR ( 'NONE', #5810, 1000.000000000000000 ) ;
#35267=ORIENTED_EDGE ( 'NONE', *, *, #17701, .T. ) ;
#35270=EDGE_LOOP ( 'NONE', ( #44255, #42515, #37261, #18525, #18498, #25615 ) ) ;
#35274=AXIS2_PLACEMENT_3D ( 'NONE', #24676, #5411, #9765 ) ;
#35287=EDGE_CURVE ( 'NONE', #26079, #27650, #32381, .T. ) ;
#35291=EDGE_CURVE ( 'NONE', #48865, #37507, #26777, .T. ) ;
#35292=ORIENTED_EDGE ( 'NONE', *, *, #1487, .F. ) ;
#35297=DIRECTION ( 'NONE',  ( -1.000000000000000000, 0.000000000000000000, 0.000000000000000000 ) ) ;
#35298=CARTESIAN_POINT ( 'NONE',  ( -126.6959734468149321, 1.749999999999997113, 40.81828755692798438 ) ) ;
#35299=CYLINDRICAL_SURFACE ( 'NONE', #27496, 1.750000000000015543 ) ;
#35302=EDGE_CURVE ( 'NONE', #39140, #34485, #37880, .T. ) ;
#35303=FACE_OUTER_BOUND ( 'NONE', #22146, .T. ) ;
#35306=VECTOR ( 'NONE', #49979, 1000.000000000000000 ) ;
#35308=ORIENTED_EDGE ( 'NONE', *, *, #2321, .F. ) ;
#35311=CARTESIAN_POINT ( 'NONE',  ( 195.0540265531851105, -1.025126265847088991, -157.4317124430720582 ) ) ;
#35314=CARTESIAN_POINT ( 'NONE',  ( -164.9459734468149463, 1.025126265847089879, 82.56828755692798438 ) ) ;
#35318=AXIS2_PLACEMENT_3D ( 'NONE', #28109, #23508, #39663 ) ;
#35321=CARTESIAN_POINT ( 'NONE',  ( -7.721099712662037540, -1.750000000000023537, 121.8434138227750623 ) ) ;
#35322=DIRECTION ( 'NONE',  ( -1.000000000000000000, -0.000000000000000000, -0.000000000000000000 ) ) ;
#35327=ORIENTED_EDGE ( 'NONE', *, *, #1502, .T. ) ;
#35329=CARTESIAN_POINT ( 'NONE',  ( -47.72109971266203132, 1.750000000000009548, 159.7931612910809065 ) ) ;
#35332=VERTEX_POINT ( 'NONE', #37015 ) ;
#35334=EDGE_CURVE ( 'NONE', #23855, #40582, #47705, .T. ) ;
#35338=( BOUNDED_CURVE ( )  B_SPLINE_CURVE ( 3, ( #48648, #48901, #5081, #44561 ),
 .UNSPECIFIED., .F., .F. ) 
 B_SPLINE_CURVE_WITH_KNOTS ( ( 4, 4 ),
 ( 0.000000000000000000, 1.570796326794896780 ),
 .UNSPECIFIED. ) 
 CURVE ( )  GEOMETRIC_REPRESENTATION_ITEM ( )  RATIONAL_B_SPLINE_CURVE ( ( 1.000000000000000000, 0.8047378541243649375, 0.8047378541243649375, 1.000000000000000000 ) ) 
 REPRESENTATION_ITEM ( '' )  );
#35342=EDGE_CURVE ( 'NONE', #9162, #47457, #5420, .T. ) ;
#35346=( BOUNDED_CURVE ( )  B_SPLINE_CURVE ( 3, ( #32515, #41188, #40192, #6043 ),
 .UNSPECIFIED., .F., .F. ) 
 B_SPLINE_CURVE_WITH_KNOTS ( ( 4, 4 ),
 ( 3.141592653589793116, 4.712388980384689674 ),
 .UNSPECIFIED. ) 
 CURVE ( )  GEOMETRIC_REPRESENTATION_ITEM ( )  RATIONAL_B_SPLINE_CURVE ( ( 1.000000000000000000, 0.8047378541243649375, 0.8047378541243649375, 1.000000000000000000 ) ) 
 REPRESENTATION_ITEM ( '' )  );
#35347=CARTESIAN_POINT ( 'NONE',  ( 210.0000000000000568, 0.000000000000000000, 160.8182875569279702 ) ) ;
#35350=LINE ( 'NONE', #43767, #47591 ) ;
#35352=ADVANCED_FACE ( 'NONE', ( #13626 ), #1586, .T. ) ;
#35354=CARTESIAN_POINT ( 'NONE',  ( 194.3291528190321742, -1.750000000000009548, -0.2068387089191121020 ) ) ;
#35356=DIRECTION ( 'NONE',  ( -0.000000000000000000, -0.000000000000000000, -1.000000000000000000 ) ) ;
#35358=CARTESIAN_POINT ( 'NONE',  ( 193.3040265531851105, 1.750000000000009992, -159.1817124430720298 ) ) ;
#35359=EDGE_CURVE ( 'NONE', #9213, #9513, #44647, .T. ) ;
#35361=ORIENTED_EDGE ( 'NONE', *, *, #9924, .T. ) ;
#35363=DIRECTION ( 'NONE',  ( 0.000000000000000000, 0.000000000000000000, 1.000000000000000000 ) ) ;
#35366=FACE_OUTER_BOUND ( 'NONE', #12132, .T. ) ;
#35372=LINE ( 'NONE', #16345, #15251 ) ;
#35379=CARTESIAN_POINT ( 'NONE',  ( 151.5540265531850537, 0.000000000000000000, 165.0000000000000000 ) ) ;
#35384=ORIENTED_EDGE ( 'NONE', *, *, #583, .T. ) ;
#35385=CARTESIAN_POINT ( 'NONE',  ( 210.0000000000000568, 0.000000000000000000, 120.8182875569279702 ) ) ;
#35387=EDGE_LOOP ( 'NONE', ( #44462, #3203, #9356, #8960, #2174, #8807 ) ) ;
#35391=CARTESIAN_POINT ( 'NONE',  ( 35.05402655318504657, -1.025126265847089657, 119.0682875569279560 ) ) ;
#35393=VERTEX_POINT ( 'NONE', #29789 ) ;
#35397=CARTESIAN_POINT ( 'NONE',  ( 33.30402655318503946, -1.750000000000010658, -79.18171244307201562 ) ) ;
#35398=CARTESIAN_POINT ( 'NONE',  ( 35.05402655318504657, 1.025126265847089213, -160.9317124430720014 ) ) ;
#35399=CARTESIAN_POINT ( 'NONE',  ( 153.3040265531850537, -1.750000000000010658, 80.81828755692798438 ) ) ;
#35400=CARTESIAN_POINT ( 'NONE',  ( -166.6959734468149463, 1.750000000000010658, -79.18171244307201562 ) ) ;
#35402=CYLINDRICAL_SURFACE ( 'NONE', #40415, 1.750000000000015543 ) ;
#35404=CARTESIAN_POINT ( 'NONE',  ( -126.6959734468149321, 1.749999999999997113, 40.81828755692798438 ) ) ;
#35410=CARTESIAN_POINT ( 'NONE',  ( -127.7210997126620242, 1.749999999999997113, -80.20683870891909351 ) ) ;
#35412=ADVANCED_FACE ( 'NONE', ( #49737 ), #46145, .T. ) ;
#35414=CARTESIAN_POINT ( 'NONE',  ( 194.3291528190321742, -1.750000000000010436, -120.2068387089191219 ) ) ;
#35415=CARTESIAN_POINT ( 'NONE',  ( 210.0000000000000568, 2.143131898507881116E-16, 39.06828755692797728 ) ) ;
#35416=EDGE_CURVE ( 'NONE', #6557, #49797, #48307, .T. ) ;
#35417=EDGE_CURVE ( 'NONE', #8857, #35947, #28727, .T. ) ;
#35419=CARTESIAN_POINT ( 'NONE',  ( 35.05402655318504657, 2.143131898507880377E-16, 165.0000000000000000 ) ) ;
#35420=EDGE_LOOP ( 'NONE', ( #12600, #38094, #38238, #35327, #41378, #26437 ) ) ;
#35424=FACE_OUTER_BOUND ( 'NONE', #17420, .T. ) ;
#35425=DIRECTION ( 'NONE',  ( -0.000000000000000000, -0.000000000000000000, -1.000000000000000000 ) ) ;
#35431=DIRECTION ( 'NONE',  ( 0.000000000000000000, 0.000000000000000000, 1.000000000000000000 ) ) ;
#35433=ORIENTED_EDGE ( 'NONE', *, *, #36676, .F. ) ;
#35435=CARTESIAN_POINT ( 'NONE',  ( 111.5540265531850679, 0.000000000000000000, -0.9317124430719969652 ) ) ;
#35438=DIRECTION ( 'NONE',  ( -1.000000000000000000, -0.000000000000000000, -0.000000000000000000 ) ) ;
#35444=ORIENTED_EDGE ( 'NONE', *, *, #22115, .F. ) ;
#35454=CARTESIAN_POINT ( 'NONE',  ( 73.30402655318508209, -1.750000000000010658, -119.1817124430720440 ) ) ;
#35459=DIRECTION ( 'NONE',  ( -1.000000000000000000, -0.000000000000000000, -0.000000000000000000 ) ) ;
#35460=EDGE_LOOP ( 'NONE', ( #13932, #7064 ) ) ;
#35463=DIRECTION ( 'NONE',  ( 1.000000000000000000, 0.000000000000000000, 0.000000000000000000 ) ) ;
#35465=CARTESIAN_POINT ( 'NONE',  ( 210.0000000000000568, 0.000000000000000000, 42.56828755692799149 ) ) ;
#35470=DIRECTION ( 'NONE',  ( 0.000000000000000000, 0.000000000000000000, 1.000000000000000000 ) ) ;
#35471=DIRECTION ( 'NONE',  ( -0.000000000000000000, -0.000000000000000000, -1.000000000000000000 ) ) ;
#35473=CARTESIAN_POINT ( 'NONE',  ( 113.3040265531850537, 1.749999999999997335, -119.1817124430720440 ) ) ;
#35477=EDGE_CURVE ( 'NONE', #44889, #8314, #2200, .T. ) ;
#35479=VECTOR ( 'NONE', #35459, 1000.000000000000000 ) ;
#35481=LINE ( 'NONE', #22892, #14886 ) ;
#35482=ORIENTED_EDGE ( 'NONE', *, *, #7810, .F. ) ;
#35485=AXIS2_PLACEMENT_3D ( 'NONE', #6470, #41626, #17521 ) ;
#35487=ORIENTED_EDGE ( 'NONE', *, *, #13316, .T. ) ;
#35492=( BOUNDED_CURVE ( )  B_SPLINE_CURVE ( 3, ( #44228, #911, #40154, #39411 ),
 .UNSPECIFIED., .F., .F. ) 
 B_SPLINE_CURVE_WITH_KNOTS ( ( 4, 4 ),
 ( 0.000000000000000000, 1.570796326794896780 ),
 .UNSPECIFIED. ) 
 CURVE ( )  GEOMETRIC_REPRESENTATION_ITEM ( )  RATIONAL_B_SPLINE_CURVE ( ( 1.000000000000000000, 0.8047378541243649375, 0.8047378541243649375, 1.000000000000000000 ) ) 
 REPRESENTATION_ITEM ( '' )  );
#35495=CARTESIAN_POINT ( 'NONE',  ( 154.3291528190321458, 1.750000000000009548, -40.20683870891912193 ) ) ;
#35496=ORIENTED_EDGE ( 'NONE', *, *, #9545, .F. ) ;
#35497=DIRECTION ( 'NONE',  ( -1.000000000000000000, -0.000000000000000000, -0.000000000000000000 ) ) ;
#35498=CARTESIAN_POINT ( 'NONE',  ( -165.6708471809677974, -1.750000000000009548, 39.79316129108089228 ) ) ;
#35502=LINE ( 'NONE', #8045, #44806 ) ;
#35509=EDGE_LOOP ( 'NONE', ( #29539, #32911 ) ) ;
#35512=ORIENTED_EDGE ( 'NONE', *, *, #7105, .T. ) ;
#35518=ORIENTED_EDGE ( 'NONE', *, *, #1092, .T. ) ;
#35519=DIRECTION ( 'NONE',  ( -0.000000000000000000, -0.000000000000000000, -1.000000000000000000 ) ) ;
#35524=DIRECTION ( 'NONE',  ( -1.000000000000000000, 0.000000000000000000, 0.000000000000000000 ) ) ;
#35526=CARTESIAN_POINT ( 'NONE',  ( -167.7210997126620384, 1.750000000000009548, -118.1565861772249519 ) ) ;
#35531=CARTESIAN_POINT ( 'NONE',  ( -6.695973446814940111, -1.750000000000024203, 80.81828755692798438 ) ) ;
#35533=DIRECTION ( 'NONE',  ( -0.000000000000000000, -0.000000000000000000, -1.000000000000000000 ) ) ;
#35534=CARTESIAN_POINT ( 'NONE',  ( 33.30402655318503946, 0.000000000000000000, 165.0000000000000000 ) ) ;
#35538=VERTEX_POINT ( 'NONE', #26191 ) ;
#35539=EDGE_CURVE ( 'NONE', #21654, #3325, #27376, .T. ) ;
#35543=CARTESIAN_POINT ( 'NONE',  ( 111.5540265531850679, 0.000000000000000000, 82.56828755692797017 ) ) ;
#35546=CYLINDRICAL_SURFACE ( 'NONE', #31616, 1.750000000000015543 ) ;
#35547=AXIS2_PLACEMENT_3D ( 'NONE', #45002, #48079, #12959 ) ;
#35551=ORIENTED_EDGE ( 'NONE', *, *, #1667, .F. ) ;
#35552=CARTESIAN_POINT ( 'NONE',  ( 210.0000000000000568, 0.000000000000000000, -157.4317124430720298 ) ) ;
#35557=ORIENTED_EDGE ( 'NONE', *, *, #39462, .F. ) ;
#35558=CARTESIAN_POINT ( 'NONE',  ( -84.94597344681494633, 2.143131898507880377E-16, 165.0000000000000000 ) ) ;
#35564=ORIENTED_EDGE ( 'NONE', *, *, #31490, .F. ) ;
#35565=EDGE_CURVE ( 'NONE', #12438, #7169, #17976, .T. ) ;
#35566=EDGE_CURVE ( 'NONE', #17256, #11190, #32631, .T. ) ;
#35570=EDGE_CURVE ( 'NONE', #16395, #2436, #23602, .T. ) ;
#35575=( BOUNDED_CURVE ( )  B_SPLINE_CURVE ( 3, ( #25762, #10855, #33721, #26018 ),
 .UNSPECIFIED., .F., .F. ) 
 B_SPLINE_CURVE_WITH_KNOTS ( ( 4, 4 ),
 ( 1.570796326794896558, 3.141592653589793116 ),
 .UNSPECIFIED. ) 
 CURVE ( )  GEOMETRIC_REPRESENTATION_ITEM ( )  RATIONAL_B_SPLINE_CURVE ( ( 1.000000000000000000, 0.8047378541243649375, 0.8047378541243649375, 1.000000000000000000 ) ) 
 REPRESENTATION_ITEM ( '' )  );
#35588=DIRECTION ( 'NONE',  ( -1.000000000000000000, -0.000000000000000000, -0.000000000000000000 ) ) ;
#35589=AXIS2_PLACEMENT_3D ( 'NONE', #15409, #22841, #18485 ) ;
#35590=AXIS2_PLACEMENT_3D ( 'NONE', #45835, #10227, #14062 ) ;
#35595=CARTESIAN_POINT ( 'NONE',  ( -48.44597344681495343, 0.000000000000000000, -80.93171244307204404 ) ) ;
#35597=EDGE_CURVE ( 'NONE', #35621, #12549, #2786, .T. ) ;
#35599=CARTESIAN_POINT ( 'NONE',  ( 155.0540265531850537, 2.143131898507880377E-16, -77.43171244307204404 ) ) ;
#35600=EDGE_CURVE ( 'NONE', #29055, #2997, #29024, .T. ) ;
#35601=ADVANCED_FACE ( 'NONE', ( #3849 ), #31829, .T. ) ;
#35610=DIRECTION ( 'NONE',  ( -0.000000000000000000, -0.000000000000000000, -1.000000000000000000 ) ) ;
#35612=CARTESIAN_POINT ( 'NONE',  ( 34.32915281903212446, -1.750000000000009548, 41.84341382277508359 ) ) ;
#35616=CARTESIAN_POINT ( 'NONE',  ( -164.9459734468149463, 2.143131898507880377E-16, -40.93171244307202983 ) ) ;
#35617=ORIENTED_EDGE ( 'NONE', *, *, #21202, .T. ) ;
#35620=DIRECTION ( 'NONE',  ( -1.000000000000000000, 0.000000000000000000, 0.000000000000000000 ) ) ;
#35621=VERTEX_POINT ( 'NONE', #46659 ) ;
#35623=CYLINDRICAL_SURFACE ( 'NONE', #7736, 1.750000000000015543 ) ;
#35626=EDGE_LOOP ( 'NONE', ( #8035, #46455, #1962, #14650, #21933, #38895 ) ) ;
#35627=VECTOR ( 'NONE', #17728, 1000.000000000000000 ) ;
#35628=DIRECTION ( 'NONE',  ( -1.000000000000000000, -0.000000000000000000, -0.000000000000000000 ) ) ;
#35634=( BOUNDED_CURVE ( )  B_SPLINE_CURVE ( 3, ( #532, #47417, #33338, #29727 ),
 .UNSPECIFIED., .F., .F. ) 
 B_SPLINE_CURVE_WITH_KNOTS ( ( 4, 4 ),
 ( 4.712388980384689674, 6.283185307179586232 ),
 .UNSPECIFIED. ) 
 CURVE ( )  GEOMETRIC_REPRESENTATION_ITEM ( )  RATIONAL_B_SPLINE_CURVE ( ( 1.000000000000000000, 0.8047378541243649375, 0.8047378541243649375, 1.000000000000000000 ) ) 
 REPRESENTATION_ITEM ( '' )  );
#35637=EDGE_CURVE ( 'NONE', #2259, #45927, #18521, .T. ) ;
#35642=ORIENTED_EDGE ( 'NONE', *, *, #20801, .T. ) ;
#35645=( BOUNDED_CURVE ( )  B_SPLINE_CURVE ( 3, ( #8833, #21127, #36805, #13423 ),
 .UNSPECIFIED., .F., .F. ) 
 B_SPLINE_CURVE_WITH_KNOTS ( ( 4, 4 ),
 ( 1.570796326794896558, 3.141592653589793116 ),
 .UNSPECIFIED. ) 
 CURVE ( )  GEOMETRIC_REPRESENTATION_ITEM ( )  RATIONAL_B_SPLINE_CURVE ( ( 1.000000000000000000, 0.8047378541243649375, 0.8047378541243649375, 1.000000000000000000 ) ) 
 REPRESENTATION_ITEM ( '' )  );
#35646=ADVANCED_FACE ( 'NONE', ( #23863 ), #4365, .T. ) ;
#35647=CARTESIAN_POINT ( 'NONE',  ( 154.3291528190321458, -1.750000000000009326, 1.843413822775066269 ) ) ;
#35652=FACE_OUTER_BOUND ( 'NONE', #49640, .T. ) ;
#35653=CARTESIAN_POINT ( 'NONE',  ( -47.72109971266203132, -1.750000000000009548, 159.7931612910809065 ) ) ;
#35659=LINE ( 'NONE', #8443, #20113 ) ;
#35665=EDGE_CURVE ( 'NONE', #23383, #34290, #23781, .T. ) ;
#35668=DIRECTION ( 'NONE',  ( -0.000000000000000000, -0.000000000000000000, -1.000000000000000000 ) ) ;
#35670=CARTESIAN_POINT ( 'NONE',  ( 210.0000000000000568, 0.000000000000000000, -159.1817124430720298 ) ) ;
#35675=ORIENTED_EDGE ( 'NONE', *, *, #30598, .T. ) ;
#35679=DIRECTION ( 'NONE',  ( -1.000000000000000000, -0.000000000000000000, -0.000000000000000000 ) ) ;
#35682=ORIENTED_EDGE ( 'NONE', *, *, #45727, .T. ) ;
#35684=ORIENTED_EDGE ( 'NONE', *, *, #1420, .F. ) ;
#35685=VECTOR ( 'NONE', #1955, 1000.000000000000000 ) ;
#35686=VERTEX_POINT ( 'NONE', #44342 ) ;
#35687=CARTESIAN_POINT ( 'NONE',  ( 113.3040265531850537, 0.000000000000000000, 165.0000000000000000 ) ) ;
#35689=AXIS2_PLACEMENT_3D ( 'NONE', #23071, #19213, #35158 ) ;
#35694=CARTESIAN_POINT ( 'NONE',  ( -86.69597344681494633, -1.750000000000009992, 160.8182875569279702 ) ) ;
#35695=CARTESIAN_POINT ( 'NONE',  ( 193.3040265531851105, -1.750000000000010658, 120.8182875569279702 ) ) ;
#35697=EDGE_CURVE ( 'NONE', #9233, #30056, #11339, .T. ) ;
#35707=DIRECTION ( 'NONE',  ( -1.000000000000000000, -0.000000000000000000, -0.000000000000000000 ) ) ;
#35710=AXIS2_PLACEMENT_3D ( 'NONE', #40239, #1992, #48637 ) ;
#35713=CARTESIAN_POINT ( 'NONE',  ( 35.05402655318504657, 2.143131898507880377E-16, -40.93171244307205825 ) ) ;
#35714=DIRECTION ( 'NONE',  ( -1.000000000000000000, -0.000000000000000000, -0.000000000000000000 ) ) ;
#35718=CARTESIAN_POINT ( 'NONE',  ( -6.695973446814940111, 0.000000000000000000, -165.0000000000000000 ) ) ;
#35722=ORIENTED_EDGE ( 'NONE', *, *, #50468, .T. ) ;
#35723=ORIENTED_EDGE ( 'NONE', *, *, #25967, .T. ) ;
#35725=CARTESIAN_POINT ( 'NONE',  ( 33.30402655318503946, -1.750000000000009992, -159.1817124430720298 ) ) ;
#35730=CARTESIAN_POINT ( 'NONE',  ( 195.0540265531851105, 2.143131898507880377E-16, -37.43171244307205825 ) ) ;
#35731=ORIENTED_EDGE ( 'NONE', *, *, #32922, .T. ) ;
#35732=DIRECTION ( 'NONE',  ( -1.000000000000000000, -0.000000000000000000, -0.000000000000000000 ) ) ;
#35738=CARTESIAN_POINT ( 'NONE',  ( -86.69597344681496054, 0.000000000000000000, -165.0000000000000000 ) ) ;
#35740=DIRECTION ( 'NONE',  ( -0.000000000000000000, -0.000000000000000000, -1.000000000000000000 ) ) ;
#35742=ORIENTED_EDGE ( 'NONE', *, *, #47179, .F. ) ;
#35744=CARTESIAN_POINT ( 'NONE',  ( 73.30402655318508209, -1.750000000000010214, 40.81828755692798438 ) ) ;
#35745=CARTESIAN_POINT ( 'NONE',  ( 195.0540265531851105, 2.143131898507880377E-16, 42.56828755692798438 ) ) ;
#35758=ORIENTED_EDGE ( 'NONE', *, *, #4220, .T. ) ;
#35766=DIRECTION ( 'NONE',  ( -0.000000000000000000, -0.000000000000000000, -1.000000000000000000 ) ) ;
#35771=CARTESIAN_POINT ( 'NONE',  ( 73.30402655318508209, 0.000000000000000000, 165.0000000000000000 ) ) ;
#35773=EDGE_CURVE ( 'NONE', #48958, #8816, #14571, .T. ) ;
#35775=VECTOR ( 'NONE', #22727, 1000.000000000000000 ) ;
#35782=CARTESIAN_POINT ( 'NONE',  ( -84.94597344681494633, 2.143131898507880377E-16, 159.0682875569279702 ) ) ;
#35787=CIRCLE ( 'NONE', #45573, 1.750000000000015543 ) ;
#35790=( BOUNDED_CURVE ( )  B_SPLINE_CURVE ( 3, ( #29195, #44812, #49142, #5834 ),
 .UNSPECIFIED., .F., .F. ) 
 B_SPLINE_CURVE_WITH_KNOTS ( ( 4, 4 ),
 ( 3.141592653589793116, 4.712388980384689674 ),
 .UNSPECIFIED. ) 
 CURVE ( )  GEOMETRIC_REPRESENTATION_ITEM ( )  RATIONAL_B_SPLINE_CURVE ( ( 1.000000000000000000, 0.8047378541243649375, 0.8047378541243649375, 1.000000000000000000 ) ) 
 REPRESENTATION_ITEM ( '' )  );
#35796=CARTESIAN_POINT ( 'NONE',  ( -128.4459734468149463, -1.025126265847081886, 79.06828755692797017 ) ) ;
#35799=CARTESIAN_POINT ( 'NONE',  ( -124.9459734468149463, 2.143131898507842906E-16, 165.0000000000000000 ) ) ;
#35800=( BOUNDED_CURVE ( )  B_SPLINE_CURVE ( 3, ( #13597, #48450, #17450, #44614 ),
 .UNSPECIFIED., .F., .F. ) 
 B_SPLINE_CURVE_WITH_KNOTS ( ( 4, 4 ),
 ( 1.570796326794896558, 3.141592653589793116 ),
 .UNSPECIFIED. ) 
 CURVE ( )  GEOMETRIC_REPRESENTATION_ITEM ( )  RATIONAL_B_SPLINE_CURVE ( ( 1.000000000000000000, 0.8047378541243649375, 0.8047378541243649375, 1.000000000000000000 ) ) 
 REPRESENTATION_ITEM ( '' )  );
#35804=CIRCLE ( 'NONE', #9538, 1.750000000000008438 ) ;
#35808=CARTESIAN_POINT ( 'NONE',  ( -166.6959734468149463, 1.750000000000009992, 0.8182875569279768335 ) ) ;
#35809=( BOUNDED_CURVE ( )  B_SPLINE_CURVE ( 3, ( #23236, #12203, #27354, #39669 ),
 .UNSPECIFIED., .F., .F. ) 
 B_SPLINE_CURVE_WITH_KNOTS ( ( 4, 4 ),
 ( 3.141592653589793116, 4.712388980384689674 ),
 .UNSPECIFIED. ) 
 CURVE ( )  GEOMETRIC_REPRESENTATION_ITEM ( )  RATIONAL_B_SPLINE_CURVE ( ( 1.000000000000000000, 0.8047378541243649375, 0.8047378541243649375, 1.000000000000000000 ) ) 
 REPRESENTATION_ITEM ( '' )  );
#35810=LINE ( 'NONE', #12917, #36186 ) ;
#35811=EDGE_CURVE ( 'NONE', #47399, #936, #4449, .T. ) ;
#35812=EDGE_LOOP ( 'NONE', ( #44578, #30479, #50328, #1373, #8708 ) ) ;
#35817=ORIENTED_EDGE ( 'NONE', *, *, #20959, .T. ) ;
#35827=CARTESIAN_POINT ( 'NONE',  ( -205.6708471809678827, -1.750000000000009548, 41.84341382277508359 ) ) ;
#35831=DIRECTION ( 'NONE',  ( -1.000000000000000000, -0.000000000000000000, -0.000000000000000000 ) ) ;
#35845=LINE ( 'NONE', #15810, #7522 ) ;
#35855=CARTESIAN_POINT ( 'NONE',  ( -48.44597344681495343, 0.000000000000000000, 79.06828755692797017 ) ) ;
#35856=CARTESIAN_POINT ( 'NONE',  ( -166.6959734468149463, 1.750000000000009992, 160.8182875569279702 ) ) ;
#35858=ORIENTED_EDGE ( 'NONE', *, *, #37611, .T. ) ;
#35860=CARTESIAN_POINT ( 'NONE',  ( 35.05402655318504657, 2.143131898507880377E-16, 39.06828755692798438 ) ) ;
#35861=VERTEX_POINT ( 'NONE', #3016 ) ;
#35862=CARTESIAN_POINT ( 'NONE',  ( -8.445973446814976526, 0.000000000000000000, -120.9317124430720725 ) ) ;
#35866=CARTESIAN_POINT ( 'NONE',  ( 113.3040265531850537, 1.749999999999997335, 80.81828755692798438 ) ) ;
#35867=ORIENTED_EDGE ( 'NONE', *, *, #28995, .F. ) ;
#35870=CARTESIAN_POINT ( 'NONE',  ( -8.445973446814976526, 0.000000000000000000, 79.06828755692795596 ) ) ;
#35874=( BOUNDED_CURVE ( )  B_SPLINE_CURVE ( 3, ( #12873, #1339, #49235, #9525 ),
 .UNSPECIFIED., .F., .F. ) 
 B_SPLINE_CURVE_WITH_KNOTS ( ( 4, 4 ),
 ( 4.712388980384689674, 6.283185307179586232 ),
 .UNSPECIFIED. ) 
 CURVE ( )  GEOMETRIC_REPRESENTATION_ITEM ( )  RATIONAL_B_SPLINE_CURVE ( ( 1.000000000000000000, 0.8047378541243649375, 0.8047378541243649375, 1.000000000000000000 ) ) 
 REPRESENTATION_ITEM ( '' )  );
#35875=ORIENTED_EDGE ( 'NONE', *, *, #32738, .F. ) ;
#35883=CARTESIAN_POINT ( 'NONE',  ( 75.05402655318509630, 2.143131898507880377E-16, -80.93171244307204404 ) ) ;
#35885=ORIENTED_EDGE ( 'NONE', *, *, #23285, .T. ) ;
#35888=CARTESIAN_POINT ( 'NONE',  ( -205.6708471809678827, -1.750000000000009548, 121.8434138227750623 ) ) ;
#35890=CARTESIAN_POINT ( 'NONE',  ( 33.30402655318503946, -1.750000000000010658, 120.8182875569279702 ) ) ;
#35894=CARTESIAN_POINT ( 'NONE',  ( -126.6959734468149321, 0.000000000000000000, -165.0000000000000000 ) ) ;
#35897=CARTESIAN_POINT ( 'NONE',  ( 111.5540265531850679, 0.000000000000000000, -157.4317124430720582 ) ) ;
#35900=CARTESIAN_POINT ( 'NONE',  ( 151.5540265531850537, 1.025126265847089213, 159.0682875569279418 ) ) ;
#35902=CARTESIAN_POINT ( 'NONE',  ( -84.94597344681494633, 2.143131898507880377E-16, 165.0000000000000000 ) ) ;
#35906=CARTESIAN_POINT ( 'NONE',  ( 210.0000000000000568, 2.143131898507880377E-16, -160.9317124430720298 ) ) ;
#35910=CARTESIAN_POINT ( 'NONE',  ( -128.4459734468149179, 0.000000000000000000, 165.0000000000000000 ) ) ;
#35911=CYLINDRICAL_SURFACE ( 'NONE', #8639, 1.750000000000010214 ) ;
#35912=EDGE_CURVE ( 'NONE', #20654, #37507, #16585, .T. ) ;
#35915=VERTEX_POINT ( 'NONE', #10226 ) ;
#35917=DIRECTION ( 'NONE',  ( 1.000000000000000000, 0.000000000000000000, 0.000000000000000000 ) ) ;
#35928=( BOUNDED_CURVE ( )  B_SPLINE_CURVE ( 3, ( #45376, #22052, #37730, #6159 ),
 .UNSPECIFIED., .F., .F. ) 
 B_SPLINE_CURVE_WITH_KNOTS ( ( 4, 4 ),
 ( 0.000000000000000000, 1.570796326794896558 ),
 .UNSPECIFIED. ) 
 CURVE ( )  GEOMETRIC_REPRESENTATION_ITEM ( )  RATIONAL_B_SPLINE_CURVE ( ( 1.000000000000000000, 0.8047378541243649375, 0.8047378541243649375, 1.000000000000000000 ) ) 
 REPRESENTATION_ITEM ( '' )  );
#35932=DIRECTION ( 'NONE',  ( 0.000000000000000000, 0.000000000000000000, 1.000000000000000000 ) ) ;
#35935=CARTESIAN_POINT ( 'NONE',  ( -206.6959734468149463, 0.000000000000000000, 165.0000000000000000 ) ) ;
#35936=CARTESIAN_POINT ( 'NONE',  ( 193.3040265531851105, 1.750000000000009992, 160.8182875569279702 ) ) ;
#35937=( BOUNDED_CURVE ( )  B_SPLINE_CURVE ( 3, ( #49534, #18526, #2867, #18269 ),
 .UNSPECIFIED., .F., .F. ) 
 B_SPLINE_CURVE_WITH_KNOTS ( ( 4, 4 ),
 ( 1.570796326794896558, 3.141592653589793116 ),
 .UNSPECIFIED. ) 
 CURVE ( )  GEOMETRIC_REPRESENTATION_ITEM ( )  RATIONAL_B_SPLINE_CURVE ( ( 1.000000000000000000, 0.8047378541243649375, 0.8047378541243649375, 1.000000000000000000 ) ) 
 REPRESENTATION_ITEM ( '' )  );
#35945=DIRECTION ( 'NONE',  ( 0.000000000000000000, 0.000000000000000000, -1.000000000000000000 ) ) ;
#35947=VERTEX_POINT ( 'NONE', #27145 ) ;
#35949=CARTESIAN_POINT ( 'NONE',  ( -88.44597344681494633, 1.025126265847089657, 119.0682875569279560 ) ) ;
#35953=CARTESIAN_POINT ( 'NONE',  ( 72.27890028733797578, 1.750000000000009548, 159.7931612910809065 ) ) ;
#35955=ORIENTED_EDGE ( 'NONE', *, *, #25315, .F. ) ;
#35956=CYLINDRICAL_SURFACE ( 'NONE', #41698, 1.750000000000001554 ) ;
#35961=ORIENTED_EDGE ( 'NONE', *, *, #18975, .F. ) ;
#35966=DIRECTION ( 'NONE',  ( -0.000000000000000000, -0.000000000000000000, -1.000000000000000000 ) ) ;
#35968=CARTESIAN_POINT ( 'NONE',  ( -84.94597344681493212, -1.025126265847089657, -80.93171244307201562 ) ) ;
#35969=DIRECTION ( 'NONE',  ( -0.000000000000000000, -0.000000000000000000, -1.000000000000000000 ) ) ;
#35978=EDGE_CURVE ( 'NONE', #35538, #14525, #12003, .T. ) ;
#35981=EDGE_LOOP ( 'NONE', ( #36769, #19168, #38347, #46466, #47352, #40430 ) ) ;
#35990=ADVANCED_FACE ( 'NONE', ( #23805 ), #11247, .T. ) ;
#35993=CARTESIAN_POINT ( 'NONE',  ( 153.3040265531850537, 1.750000000000010658, -79.18171244307201562 ) ) ;
#35994=ORIENTED_EDGE ( 'NONE', *, *, #34840, .F. ) ;
#35996=LINE ( 'NONE', #837, #1943 ) ;
#35997=LINE ( 'NONE', #32383, #49127 ) ;
#36000=ORIENTED_EDGE ( 'NONE', *, *, #23018, .T. ) ;
#36015=VECTOR ( 'NONE', #12189, 1000.000000000000000 ) ;
#36016=CARTESIAN_POINT ( 'NONE',  ( -205.6708471809678827, -1.750000000000010436, 119.7931612910808781 ) ) ;
#36017=VERTEX_POINT ( 'NONE', #31258 ) ;
#36021=CARTESIAN_POINT ( 'NONE',  ( -85.67084718096784002, -1.750000000000009326, 159.7931612910809065 ) ) ;
#36024=DIRECTION ( 'NONE',  ( 1.000000000000000000, 0.000000000000000000, 0.000000000000000000 ) ) ;
#36025=EDGE_LOOP ( 'NONE', ( #31625, #36066 ) ) ;
#36037=PLANE ( 'NONE',  #19322 ) ;
#36040=CARTESIAN_POINT ( 'NONE',  ( 210.0000000000000568, 0.000000000000000000, 80.81828755692798438 ) ) ;
#36044=VECTOR ( 'NONE', #45671, 1000.000000000000000 ) ;
#36047=CARTESIAN_POINT ( 'NONE',  ( -46.69597344681494633, 1.750000000000009992, 0.8182875569279768335 ) ) ;
#36052=CARTESIAN_POINT ( 'NONE',  ( 112.2789002873379758, -1.749999999999996891, 81.84341382277506227 ) ) ;
#36056=DIRECTION ( 'NONE',  ( 1.000000000000000000, 0.000000000000000000, 0.000000000000000000 ) ) ;
#36059=DIRECTION ( 'NONE',  ( -0.000000000000000000, -0.000000000000000000, -1.000000000000000000 ) ) ;
#36061=ORIENTED_EDGE ( 'NONE', *, *, #32849, .T. ) ;
#36066=ORIENTED_EDGE ( 'NONE', *, *, #25818, .T. ) ;
#36067=ORIENTED_EDGE ( 'NONE', *, *, #1547, .T. ) ;
#36069=CARTESIAN_POINT ( 'NONE',  ( -210.0000000000000568, 0.000000000000000000, 120.8182875569279702 ) ) ;
#36071=( BOUNDED_CURVE ( )  B_SPLINE_CURVE ( 3, ( #4212, #19845, #35526, #20858 ),
 .UNSPECIFIED., .F., .F. ) 
 B_SPLINE_CURVE_WITH_KNOTS ( ( 4, 4 ),
 ( 3.141592653589793116, 4.712388980384689674 ),
 .UNSPECIFIED. ) 
 CURVE ( )  GEOMETRIC_REPRESENTATION_ITEM ( )  RATIONAL_B_SPLINE_CURVE ( ( 1.000000000000000000, 0.8047378541243649375, 0.8047378541243649375, 1.000000000000000000 ) ) 
 REPRESENTATION_ITEM ( '' )  );
#36079=( BOUNDED_CURVE ( )  B_SPLINE_CURVE ( 3, ( #25971, #26459, #11061, #2349 ),
 .UNSPECIFIED., .F., .F. ) 
 B_SPLINE_CURVE_WITH_KNOTS ( ( 4, 4 ),
 ( 1.570796326794896558, 3.141592653589793116 ),
 .UNSPECIFIED. ) 
 CURVE ( )  GEOMETRIC_REPRESENTATION_ITEM ( )  RATIONAL_B_SPLINE_CURVE ( ( 1.000000000000000000, 0.8047378541243649375, 0.8047378541243649375, 1.000000000000000000 ) ) 
 REPRESENTATION_ITEM ( '' )  );
#36082=FACE_OUTER_BOUND ( 'NONE', #3143, .T. ) ;
#36084=EDGE_LOOP ( 'NONE', ( #13893, #5934, #1596, #47498, #43225, #43868 ) ) ;
#36090=FACE_OUTER_BOUND ( 'NONE', #36686, .T. ) ;
#36097=( BOUNDED_CURVE ( )  B_SPLINE_CURVE ( 3, ( #43142, #309, #1055, #8006 ),
 .UNSPECIFIED., .F., .F. ) 
 B_SPLINE_CURVE_WITH_KNOTS ( ( 4, 4 ),
 ( 4.712388980384689674, 6.283185307179586232 ),
 .UNSPECIFIED. ) 
 CURVE ( )  GEOMETRIC_REPRESENTATION_ITEM ( )  RATIONAL_B_SPLINE_CURVE ( ( 1.000000000000000000, 0.8047378541243649375, 0.8047378541243649375, 1.000000000000000000 ) ) 
 REPRESENTATION_ITEM ( '' )  );
#36098=DIRECTION ( 'NONE',  ( -1.000000000000000000, -0.000000000000000000, -0.000000000000000000 ) ) ;
#36100=CARTESIAN_POINT ( 'NONE',  ( -8.445973446814962315, 1.025126265847096763, 2.568287556927999926 ) ) ;
#36105=AXIS2_PLACEMENT_3D ( 'NONE', #9834, #29846, #6490 ) ;
#36107=DIRECTION ( 'NONE',  ( -0.000000000000000000, -0.000000000000000000, -1.000000000000000000 ) ) ;
#36108=AXIS2_PLACEMENT_3D ( 'NONE', #14625, #18211, #2320 ) ;
#36112=EDGE_CURVE ( 'NONE', #32609, #37650, #9688, .T. ) ;
#36118=ORIENTED_EDGE ( 'NONE', *, *, #21898, .F. ) ;
#36121=CARTESIAN_POINT ( 'NONE',  ( -168.4459734468149747, -1.025126265847089879, 122.5682875569280128 ) ) ;
#36124=CARTESIAN_POINT ( 'NONE',  ( -166.6959734468149463, -1.750000000000009992, 0.8182875569279768335 ) ) ;
#36128=FACE_OUTER_BOUND ( 'NONE', #26468, .T. ) ;
#36129=CARTESIAN_POINT ( 'NONE',  ( 155.0540265531850537, 1.025126265847088991, 162.5682875569279133 ) ) ;
#36131=ORIENTED_EDGE ( 'NONE', *, *, #45727, .F. ) ;
#36132=DIRECTION ( 'NONE',  ( 0.000000000000000000, 0.000000000000000000, 1.000000000000000000 ) ) ;
#36146=CARTESIAN_POINT ( 'NONE',  ( -126.6959734468149321, 1.749999999999997335, 80.81828755692798438 ) ) ;
#36160=CARTESIAN_POINT ( 'NONE',  ( -164.9459734468149463, -1.025126265847088991, 159.0682875569279418 ) ) ;
#36164=( BOUNDED_CURVE ( )  B_SPLINE_CURVE ( 3, ( #31342, #24405, #15937, #43125 ),
 .UNSPECIFIED., .F., .F. ) 
 B_SPLINE_CURVE_WITH_KNOTS ( ( 4, 4 ),
 ( 0.000000000000000000, 1.570796326794896558 ),
 .UNSPECIFIED. ) 
 CURVE ( )  GEOMETRIC_REPRESENTATION_ITEM ( )  RATIONAL_B_SPLINE_CURVE ( ( 1.000000000000000000, 0.8047378541243649375, 0.8047378541243649375, 1.000000000000000000 ) ) 
 REPRESENTATION_ITEM ( '' )  );
#36165=ORIENTED_EDGE ( 'NONE', *, *, #2771, .F. ) ;
#36170=EDGE_LOOP ( 'NONE', ( #9709, #28318, #1028, #25679, #44731 ) ) ;
#36174=ADVANCED_FACE ( 'NONE', ( #13243 ), #20440, .T. ) ;
#36183=EDGE_CURVE ( 'NONE', #5869, #41405, #27890, .T. ) ;
#36186=VECTOR ( 'NONE', #24487, 1000.000000000000000 ) ;
#36195=ORIENTED_EDGE ( 'NONE', *, *, #7057, .T. ) ;
#36198=ADVANCED_FACE ( 'NONE', ( #40208 ), #1715, .T. ) ;
#36199=ORIENTED_EDGE ( 'NONE', *, *, #24802, .F. ) ;
#36200=EDGE_CURVE ( 'NONE', #16946, #47659, #14936, .T. ) ;
#36206=EDGE_CURVE ( 'NONE', #33842, #39985, #33284, .T. ) ;
#36214=VERTEX_POINT ( 'NONE', #25563 ) ;
#36215=EDGE_LOOP ( 'NONE', ( #8557, #26529, #17401, #5989, #5866, #21152 ) ) ;
#36219=CARTESIAN_POINT ( 'NONE',  ( -86.69597344681494633, -1.750000000000010658, -79.18171244307201562 ) ) ;
#36222=CARTESIAN_POINT ( 'NONE',  ( 210.0000000000000568, 0.000000000000000000, -77.43171244307200141 ) ) ;
#36228=( BOUNDED_CURVE ( )  B_SPLINE_CURVE ( 3, ( #29541, #29799, #10046, #44905 ),
 .UNSPECIFIED., .F., .F. ) 
 B_SPLINE_CURVE_WITH_KNOTS ( ( 4, 4 ),
 ( 1.570796326794896558, 3.141592653589793116 ),
 .UNSPECIFIED. ) 
 CURVE ( )  GEOMETRIC_REPRESENTATION_ITEM ( )  RATIONAL_B_SPLINE_CURVE ( ( 1.000000000000000000, 0.8047378541243649375, 0.8047378541243649375, 1.000000000000000000 ) ) 
 REPRESENTATION_ITEM ( '' )  );
#36229=VERTEX_POINT ( 'NONE', #14768 ) ;
#36230=ADVANCED_FACE ( 'NONE', ( #18601 ), #48863, .T. ) ;
#36231=CARTESIAN_POINT ( 'NONE',  ( 115.0540265531850395, 2.143131898507847836E-16, -120.9317124430720156 ) ) ;
#36233=EDGE_CURVE ( 'NONE', #46718, #24760, #30675, .T. ) ;
#36238=( BOUNDED_CURVE ( )  B_SPLINE_CURVE ( 3, ( #45366, #41796, #5890, #37719 ),
 .UNSPECIFIED., .F., .F. ) 
 B_SPLINE_CURVE_WITH_KNOTS ( ( 4, 4 ),
 ( 1.570796326794896558, 3.141592653589793116 ),
 .UNSPECIFIED. ) 
 CURVE ( )  GEOMETRIC_REPRESENTATION_ITEM ( )  RATIONAL_B_SPLINE_CURVE ( ( 1.000000000000000000, 0.8047378541243649375, 0.8047378541243649375, 1.000000000000000000 ) ) 
 REPRESENTATION_ITEM ( '' )  );
#36239=DIRECTION ( 'NONE',  ( 0.000000000000000000, 0.000000000000000000, 1.000000000000000000 ) ) ;
#36240=DIRECTION ( 'NONE',  ( 0.000000000000000000, 0.000000000000000000, 1.000000000000000000 ) ) ;
#36242=EDGE_CURVE ( 'NONE', #23942, #41850, #9907, .T. ) ;
#36244=ORIENTED_EDGE ( 'NONE', *, *, #36436, .F. ) ;
#36245=CARTESIAN_POINT ( 'NONE',  ( -84.94597344681493212, 1.025126265847089213, -0.9317124430720324924 ) ) ;
#36247=CARTESIAN_POINT ( 'NONE',  ( 193.3040265531851105, 0.000000000000000000, 165.0000000000000000 ) ) ;
#36250=VERTEX_POINT ( 'NONE', #45282 ) ;
#36252=CARTESIAN_POINT ( 'NONE',  ( 193.3040265531851105, 1.750000000000009992, -159.1817124430720298 ) ) ;
#36255=ORIENTED_EDGE ( 'NONE', *, *, #41057, .T. ) ;
#36258=CARTESIAN_POINT ( 'NONE',  ( -88.44597344681494633, -1.025126265847089657, 42.56828755692799149 ) ) ;
#36260=EDGE_CURVE ( 'NONE', #13365, #3878, #22467, .T. ) ;
#36261=EDGE_LOOP ( 'NONE', ( #37511, #27749 ) ) ;
#36263=FACE_OUTER_BOUND ( 'NONE', #5243, .T. ) ;
#36266=DIRECTION ( 'NONE',  ( -1.000000000000000000, -0.000000000000000000, -0.000000000000000000 ) ) ;
#36268=EDGE_CURVE ( 'NONE', #22181, #10836, #21837, .T. ) ;
#36269=EDGE_CURVE ( 'NONE', #39985, #50479, #19879, .T. ) ;
#36270=ORIENTED_EDGE ( 'NONE', *, *, #14408, .T. ) ;
#36273=CARTESIAN_POINT ( 'NONE',  ( 191.5540265531851105, 0.000000000000000000, -120.9317124430720156 ) ) ;
#36277=CIRCLE ( 'NONE', #34610, 1.750000000000015543 ) ;
#36281=VERTEX_POINT ( 'NONE', #7080 ) ;
#36282=EDGE_CURVE ( 'NONE', #41447, #38146, #15533, .T. ) ;
#36287=DIRECTION ( 'NONE',  ( -0.000000000000000000, -0.000000000000000000, -1.000000000000000000 ) ) ;
#36300=VECTOR ( 'NONE', #10073, 1000.000000000000000 ) ;
#36307=CARTESIAN_POINT ( 'NONE',  ( 113.3040265531850537, -1.749999999999997335, 80.81828755692798438 ) ) ;
#36308=CARTESIAN_POINT ( 'NONE',  ( -208.4459734468148611, -1.025126265847089657, 42.56828755692799149 ) ) ;
#36311=EDGE_CURVE ( 'NONE', #18807, #36974, #32333, .T. ) ;
#36318=ORIENTED_EDGE ( 'NONE', *, *, #30292, .T. ) ;
#36320=CARTESIAN_POINT ( 'NONE',  ( -168.4459734468149463, 0.000000000000000000, 165.0000000000000000 ) ) ;
#36322=FACE_OUTER_BOUND ( 'NONE', #12266, .T. ) ;
#36323=VERTEX_POINT ( 'NONE', #30685 ) ;
#36325=AXIS2_PLACEMENT_3D ( 'NONE', #25598, #17638, #29200 ) ;
#36328=EDGE_CURVE ( 'NONE', #41828, #8682, #15778, .T. ) ;
#36333=ORIENTED_EDGE ( 'NONE', *, *, #5838, .F. ) ;
#36336=EDGE_CURVE ( 'NONE', #45355, #1022, #39227, .T. ) ;
#36340=CARTESIAN_POINT ( 'NONE',  ( 210.0000000000000568, 0.000000000000000000, -79.18171244307201562 ) ) ;
#36344=PLANE ( 'NONE',  #10664 ) ;
#36345=CARTESIAN_POINT ( 'NONE',  ( -48.44597344681496054, 1.025126265847089657, 119.0682875569279560 ) ) ;
#36347=DIRECTION ( 'NONE',  ( 0.000000000000000000, 0.000000000000000000, 1.000000000000000000 ) ) ;
#36355=DIRECTION ( 'NONE',  ( 0.000000000000000000, 0.000000000000000000, 1.000000000000000000 ) ) ;
#36358=CARTESIAN_POINT ( 'NONE',  ( -44.94597344681493922, 2.143131898507880377E-16, -80.93171244307204404 ) ) ;
#36361=ORIENTED_EDGE ( 'NONE', *, *, #30680, .T. ) ;
#36364=DIRECTION ( 'NONE',  ( -1.000000000000000000, -0.000000000000000000, -0.000000000000000000 ) ) ;
#36365=ORIENTED_EDGE ( 'NONE', *, *, #29939, .F. ) ;
#36366=FACE_OUTER_BOUND ( 'NONE', #1699, .T. ) ;
#36368=CARTESIAN_POINT ( 'NONE',  ( 32.27890028733795447, -1.750000000000010214, -78.15658617722490931 ) ) ;
#36372=ORIENTED_EDGE ( 'NONE', *, *, #34809, .T. ) ;
#36377=( BOUNDED_CURVE ( )  B_SPLINE_CURVE ( 3, ( #19106, #50369, #29655, #45276 ),
 .UNSPECIFIED., .F., .F. ) 
 B_SPLINE_CURVE_WITH_KNOTS ( ( 4, 4 ),
 ( 1.570796326794896558, 3.141592653589793116 ),
 .UNSPECIFIED. ) 
 CURVE ( )  GEOMETRIC_REPRESENTATION_ITEM ( )  RATIONAL_B_SPLINE_CURVE ( ( 1.000000000000000000, 0.8047378541243649375, 0.8047378541243649375, 1.000000000000000000 ) ) 
 REPRESENTATION_ITEM ( '' )  );
#36384=( BOUNDED_CURVE ( )  B_SPLINE_CURVE ( 3, ( #44424, #17501, #33423, #17757 ),
 .UNSPECIFIED., .F., .F. ) 
 B_SPLINE_CURVE_WITH_KNOTS ( ( 4, 4 ),
 ( 0.000000000000000000, 1.570796326794896780 ),
 .UNSPECIFIED. ) 
 CURVE ( )  GEOMETRIC_REPRESENTATION_ITEM ( )  RATIONAL_B_SPLINE_CURVE ( ( 1.000000000000000000, 0.8047378541243649375, 0.8047378541243649375, 1.000000000000000000 ) ) 
 REPRESENTATION_ITEM ( '' )  );
#36385=CARTESIAN_POINT ( 'NONE',  ( -48.44597344681495343, 0.000000000000000000, -77.43171244307198720 ) ) ;
#36386=ORIENTED_EDGE ( 'NONE', *, *, #34611, .T. ) ;
#36388=CARTESIAN_POINT ( 'NONE',  ( -126.6959734468149321, 0.000000000000000000, 165.0000000000000000 ) ) ;
#36389=CARTESIAN_POINT ( 'NONE',  ( 210.0000000000000568, 0.000000000000000000, 120.8182875569279702 ) ) ;
#36395=ORIENTED_EDGE ( 'NONE', *, *, #30880, .F. ) ;
#36397=CARTESIAN_POINT ( 'NONE',  ( -6.695973446814940111, -1.750000000000023315, 160.8182875569279702 ) ) ;
#36399=( BOUNDED_CURVE ( )  B_SPLINE_CURVE ( 3, ( #50181, #35128, #15358, #12255 ),
 .UNSPECIFIED., .F., .F. ) 
 B_SPLINE_CURVE_WITH_KNOTS ( ( 4, 4 ),
 ( 1.570796326794896558, 3.141592653589793116 ),
 .UNSPECIFIED. ) 
 CURVE ( )  GEOMETRIC_REPRESENTATION_ITEM ( )  RATIONAL_B_SPLINE_CURVE ( ( 1.000000000000000000, 0.8047378541243649375, 0.8047378541243649375, 1.000000000000000000 ) ) 
 REPRESENTATION_ITEM ( '' )  );
#36401=VERTEX_POINT ( 'NONE', #909 ) ;
#36404=VECTOR ( 'NONE', #3054, 1000.000000000000000 ) ;
#36406=CARTESIAN_POINT ( 'NONE',  ( -4.945973446814903696, 2.143131898507912917E-16, -0.9317124430720524764 ) ) ;
#36407=CARTESIAN_POINT ( 'NONE',  ( 111.5540265531850537, -1.025126265847081664, -157.4317124430720582 ) ) ;
#36411=CARTESIAN_POINT ( 'NONE',  ( -88.44597344681494633, 1.025126265847089435, -117.4317124430720156 ) ) ;
#36412=CARTESIAN_POINT ( 'NONE',  ( -207.7210997126620384, 1.750000000000009548, -160.2068387089191219 ) ) ;
#36413=DIRECTION ( 'NONE',  ( -0.000000000000000000, -0.000000000000000000, -1.000000000000000000 ) ) ;
#36414=DIRECTION ( 'NONE',  ( -0.000000000000000000, -0.000000000000000000, -1.000000000000000000 ) ) ;
#36418=ORIENTED_EDGE ( 'NONE', *, *, #46290, .T. ) ;
#36421=LINE ( 'NONE', #21000, #27500 ) ;
#36426=AXIS2_PLACEMENT_3D ( 'NONE', #28655, #28413, #9908 ) ;
#36427=ORIENTED_EDGE ( 'NONE', *, *, #5298, .T. ) ;
#36433=ORIENTED_EDGE ( 'NONE', *, *, #8625, .F. ) ;
#36435=AXIS2_PLACEMENT_3D ( 'NONE', #25651, #45620, #37226 ) ;
#36436=EDGE_CURVE ( 'NONE', #27396, #18807, #31742, .T. ) ;
#36438=CARTESIAN_POINT ( 'NONE',  ( 193.3040265531851105, -1.750000000000010658, 80.81828755692798438 ) ) ;
#36440=( BOUNDED_CURVE ( )  B_SPLINE_CURVE ( 3, ( #50275, #14925, #30846, #15433 ),
 .UNSPECIFIED., .F., .F. ) 
 B_SPLINE_CURVE_WITH_KNOTS ( ( 4, 4 ),
 ( 3.141592653589793116, 4.712388980384689674 ),
 .UNSPECIFIED. ) 
 CURVE ( )  GEOMETRIC_REPRESENTATION_ITEM ( )  RATIONAL_B_SPLINE_CURVE ( ( 1.000000000000000000, 0.8047378541243649375, 0.8047378541243649375, 1.000000000000000000 ) ) 
 REPRESENTATION_ITEM ( '' )  );
#36443=DIRECTION ( 'NONE',  ( 0.000000000000000000, 0.000000000000000000, 1.000000000000000000 ) ) ;
#36455=CARTESIAN_POINT ( 'NONE',  ( -4.945973446814916130, 1.025126265847097429, 79.06828755692792754 ) ) ;
#36456=CARTESIAN_POINT ( 'NONE',  ( -48.44597344681495343, 0.000000000000000000, 2.568287556927978166 ) ) ;
#36458=CYLINDRICAL_SURFACE ( 'NONE', #16916, 1.750000000000015543 ) ;
#36462=ORIENTED_EDGE ( 'NONE', *, *, #33903, .T. ) ;
#36464=LINE ( 'NONE', #16682, #5656 ) ;
#36465=CARTESIAN_POINT ( 'NONE',  ( -88.44597344681494633, 1.025126265847089657, -80.93171244307201562 ) ) ;
#36467=CARTESIAN_POINT ( 'NONE',  ( 151.5540265531850537, 1.025126265847089213, 162.5682875569279133 ) ) ;
#36469=AXIS2_PLACEMENT_3D ( 'NONE', #43812, #4809, #48380 ) ;
#36472=CARTESIAN_POINT ( 'NONE',  ( 35.05402655318504657, 2.143131898507880377E-16, -160.9317124430720582 ) ) ;
#36473=CARTESIAN_POINT ( 'NONE',  ( 115.0540265531850395, -1.025126265847081664, -77.43171244307201562 ) ) ;
#36474=CARTESIAN_POINT ( 'NONE',  ( -128.4459734468149179, 0.000000000000000000, 82.56828755692795596 ) ) ;
#36476=EDGE_LOOP ( 'NONE', ( #34637, #11994 ) ) ;
#36480=LINE ( 'NONE', #16965, #6139 ) ;
#36484=CARTESIAN_POINT ( 'NONE',  ( 192.2789002873380184, -1.750000000000010214, 119.7931612910808781 ) ) ;
#36487=AXIS2_PLACEMENT_3D ( 'NONE', #25225, #28571, #12910 ) ;
#36492=CARTESIAN_POINT ( 'NONE',  ( -204.9459734468149463, 2.143131898507880377E-16, -157.4317124430720582 ) ) ;
#36496=ADVANCED_FACE ( 'NONE', ( #48300 ), #40408, .T. ) ;
#36498=CARTESIAN_POINT ( 'NONE',  ( -126.6959734468149321, 1.749999999999996891, 0.8182875569279768335 ) ) ;
#36500=CARTESIAN_POINT ( 'NONE',  ( -166.6959734468149463, 1.750000000000010214, 40.81828755692798438 ) ) ;
#36501=AXIS2_PLACEMENT_3D ( 'NONE', #21207, #48615, #13506 ) ;
#36504=CARTESIAN_POINT ( 'NONE',  ( -128.4459734468149179, 0.000000000000000000, -117.4317124430720725 ) ) ;
#36514=DIRECTION ( 'NONE',  ( -1.000000000000000000, 0.000000000000000000, 0.000000000000000000 ) ) ;
#36515=EDGE_LOOP ( 'NONE', ( #45705, #49999, #3724, #18311, #47860, #14907 ) ) ;
#36522=VECTOR ( 'NONE', #40089, 1000.000000000000000 ) ;
#36530=EDGE_CURVE ( 'NONE', #21643, #21466, #267, .T. ) ;
#36533=CARTESIAN_POINT ( 'NONE',  ( 193.3040265531851105, 1.750000000000009992, 0.8182875569279768335 ) ) ;
#36534=EDGE_LOOP ( 'NONE', ( #8371, #11701, #22073, #37073, #1714, #24572 ) ) ;
#36541=CARTESIAN_POINT ( 'NONE',  ( -164.9459734468149463, 2.143131898507880377E-16, 165.0000000000000000 ) ) ;
#36542=CARTESIAN_POINT ( 'NONE',  ( 155.0540265531850537, 2.143131898507880377E-16, -157.4317124430720582 ) ) ;
#36544=CARTESIAN_POINT ( 'NONE',  ( -126.6959734468149321, 0.000000000000000000, 165.0000000000000000 ) ) ;
#36548=CARTESIAN_POINT ( 'NONE',  ( -48.44597344681495343, 0.000000000000000000, 2.568287556927978166 ) ) ;
#36549=( BOUNDED_CURVE ( )  B_SPLINE_CURVE ( 3, ( #24348, #13019, #47885, #17134 ),
 .UNSPECIFIED., .F., .F. ) 
 B_SPLINE_CURVE_WITH_KNOTS ( ( 4, 4 ),
 ( 3.141592653589793116, 4.712388980384689674 ),
 .UNSPECIFIED. ) 
 CURVE ( )  GEOMETRIC_REPRESENTATION_ITEM ( )  RATIONAL_B_SPLINE_CURVE ( ( 1.000000000000000000, 0.8047378541243649375, 0.8047378541243649375, 1.000000000000000000 ) ) 
 REPRESENTATION_ITEM ( '' )  );
#36550=CYLINDRICAL_SURFACE ( 'NONE', #36619, 1.750000000000036193 ) ;
#36551=FACE_OUTER_BOUND ( 'NONE', #50311, .T. ) ;
#36557=ORIENTED_EDGE ( 'NONE', *, *, #39649, .T. ) ;
#36559=LINE ( 'NONE', #1395, #12701 ) ;
#36564=ORIENTED_EDGE ( 'NONE', *, *, #21983, .T. ) ;
#36567=ADVANCED_FACE ( 'NONE', ( #40904 ), #17803, .T. ) ;
#36570=VECTOR ( 'NONE', #19119, 1000.000000000000000 ) ;
#36571=PLANE ( 'NONE',  #33583 ) ;
#36573=CYLINDRICAL_SURFACE ( 'NONE', #20121, 1.750000000000015543 ) ;
#36575=VECTOR ( 'NONE', #30401, 1000.000000000000000 ) ;
#36583=CARTESIAN_POINT ( 'NONE',  ( -86.69597344681496054, 0.000000000000000000, 165.0000000000000000 ) ) ;
#36589=VERTEX_POINT ( 'NONE', #33469 ) ;
#36592=DIRECTION ( 'NONE',  ( 1.000000000000000000, 0.000000000000000000, 0.000000000000000000 ) ) ;
#36594=EDGE_CURVE ( 'NONE', #37650, #17197, #48809, .T. ) ;
#36595=DIRECTION ( 'NONE',  ( -1.000000000000000000, -0.000000000000000000, -0.000000000000000000 ) ) ;
#36596=ORIENTED_EDGE ( 'NONE', *, *, #35665, .F. ) ;
#36603=FACE_OUTER_BOUND ( 'NONE', #38496, .T. ) ;
#36606=CYLINDRICAL_SURFACE ( 'NONE', #6848, 1.750000000000001554 ) ;
#36612=ORIENTED_EDGE ( 'NONE', *, *, #15637, .T. ) ;
#36615=CYLINDRICAL_SURFACE ( 'NONE', #9306, 1.750000000000036193 ) ;
#36618=VECTOR ( 'NONE', #22346, 1000.000000000000000 ) ;
#36619=AXIS2_PLACEMENT_3D ( 'NONE', #8696, #38987, #47131 ) ;
#36620=EDGE_CURVE ( 'NONE', #35055, #2039, #36695, .T. ) ;
#36622=CARTESIAN_POINT ( 'NONE',  ( -128.4459734468149463, 1.025126265847081886, 79.06828755692797017 ) ) ;
#36631=CARTESIAN_POINT ( 'NONE',  ( 155.0540265531850537, 1.025126265847089657, 42.56828755692799149 ) ) ;
#36632=ORIENTED_EDGE ( 'NONE', *, *, #20678, .T. ) ;
#36636=EDGE_CURVE ( 'NONE', #23942, #18077, #28432, .T. ) ;
#36637=ORIENTED_EDGE ( 'NONE', *, *, #2950, .F. ) ;
#36639=ORIENTED_EDGE ( 'NONE', *, *, #9948, .F. ) ;
#36642=DIRECTION ( 'NONE',  ( -1.000000000000000000, 0.000000000000000000, 0.000000000000000000 ) ) ;
#36647=CARTESIAN_POINT ( 'NONE',  ( 34.32915281903212446, 1.750000000000009548, 1.843413822775065825 ) ) ;
#36648=ORIENTED_EDGE ( 'NONE', *, *, #33741, .F. ) ;
#36649=ORIENTED_EDGE ( 'NONE', *, *, #9563, .T. ) ;
#36651=FACE_OUTER_BOUND ( 'NONE', #30638, .T. ) ;
#36656=ORIENTED_EDGE ( 'NONE', *, *, #12687, .F. ) ;
#36661=ORIENTED_EDGE ( 'NONE', *, *, #37764, .F. ) ;
#36663=CARTESIAN_POINT ( 'NONE',  ( 193.3040265531851105, 1.750000000000010658, -79.18171244307201562 ) ) ;
#36664=ORIENTED_EDGE ( 'NONE', *, *, #48073, .T. ) ;
#36676=EDGE_CURVE ( 'NONE', #38146, #45661, #6838, .T. ) ;
#36679=CARTESIAN_POINT ( 'NONE',  ( 114.3291528190321173, -1.749999999999996669, 161.8434138227750907 ) ) ;
#36684=CARTESIAN_POINT ( 'NONE',  ( -4.945973446814903696, 2.143131898507912917E-16, 165.0000000000000000 ) ) ;
#36685=( BOUNDED_CURVE ( )  B_SPLINE_CURVE ( 3, ( #21531, #34360, #29489, #6142 ),
 .UNSPECIFIED., .F., .F. ) 
 B_SPLINE_CURVE_WITH_KNOTS ( ( 4, 4 ),
 ( 1.570796326794896558, 3.141592653589793116 ),
 .UNSPECIFIED. ) 
 CURVE ( )  GEOMETRIC_REPRESENTATION_ITEM ( )  RATIONAL_B_SPLINE_CURVE ( ( 1.000000000000000000, 0.8047378541243649375, 0.8047378541243649375, 1.000000000000000000 ) ) 
 REPRESENTATION_ITEM ( '' )  );
#36686=EDGE_LOOP ( 'NONE', ( #34796, #13789, #11459, #21275, #24933, #23713 ) ) ;
#36687=DIRECTION ( 'NONE',  ( -1.000000000000000000, 0.000000000000000000, 0.000000000000000000 ) ) ;
#36689=EDGE_CURVE ( 'NONE', #6739, #28163, #8225, .T. ) ;
#36694=CARTESIAN_POINT ( 'NONE',  ( 113.3040265531850537, 1.749999999999997335, -119.1817124430720440 ) ) ;
#36695=( BOUNDED_CURVE ( )  B_SPLINE_CURVE ( 3, ( #21649, #5996, #37338, #2164 ),
 .UNSPECIFIED., .F., .F. ) 
 B_SPLINE_CURVE_WITH_KNOTS ( ( 4, 4 ),
 ( 1.570796326794896558, 3.141592653589793116 ),
 .UNSPECIFIED. ) 
 CURVE ( )  GEOMETRIC_REPRESENTATION_ITEM ( )  RATIONAL_B_SPLINE_CURVE ( ( 1.000000000000000000, 0.8047378541243649375, 0.8047378541243649375, 1.000000000000000000 ) ) 
 REPRESENTATION_ITEM ( '' )  );
#36697=CARTESIAN_POINT ( 'NONE',  ( -206.6959734468149463, -1.750000000000010658, 120.8182875569279702 ) ) ;
#36699=ORIENTED_EDGE ( 'NONE', *, *, #9578, .F. ) ;
#36700=ORIENTED_EDGE ( 'NONE', *, *, #18436, .F. ) ;
#36703=ORIENTED_EDGE ( 'NONE', *, *, #24340, .F. ) ;
#36705=CARTESIAN_POINT ( 'NONE',  ( 210.0000000000000568, 0.000000000000000000, -39.18171244307202983 ) ) ;
#36708=DIRECTION ( 'NONE',  ( -0.000000000000000000, -0.000000000000000000, -1.000000000000000000 ) ) ;
#36711=( BOUNDED_CURVE ( )  B_SPLINE_CURVE ( 3, ( #6328, #2715, #17364, #6066 ),
 .UNSPECIFIED., .F., .F. ) 
 B_SPLINE_CURVE_WITH_KNOTS ( ( 4, 4 ),
 ( 4.712388980384689674, 6.283185307179586232 ),
 .UNSPECIFIED. ) 
 CURVE ( )  GEOMETRIC_REPRESENTATION_ITEM ( )  RATIONAL_B_SPLINE_CURVE ( ( 1.000000000000000000, 0.8047378541243649375, 0.8047378541243649375, 1.000000000000000000 ) ) 
 REPRESENTATION_ITEM ( '' )  );
#36715=EDGE_LOOP ( 'NONE', ( #28854, #9014, #43855, #2844, #4496, #14136 ) ) ;
#36719=ORIENTED_EDGE ( 'NONE', *, *, #17194, .T. ) ;
#36738=DIRECTION ( 'NONE',  ( 0.000000000000000000, 0.000000000000000000, 1.000000000000000000 ) ) ;
#36741=CARTESIAN_POINT ( 'NONE',  ( 210.0000000000000568, 0.000000000000000000, -79.18171244307201562 ) ) ;
#36743=CYLINDRICAL_SURFACE ( 'NONE', #37646, 1.749999999999987566 ) ;
#36746=ORIENTED_EDGE ( 'NONE', *, *, #13930, .F. ) ;
#36751=ORIENTED_EDGE ( 'NONE', *, *, #41535, .F. ) ;
#36752=CARTESIAN_POINT ( 'NONE',  ( 210.0000000000000568, 0.000000000000000000, 42.56828755692799149 ) ) ;
#36754=CARTESIAN_POINT ( 'NONE',  ( -204.9459734468149463, 2.143131898507890731E-16, -165.0000000000000000 ) ) ;
#36756=ORIENTED_EDGE ( 'NONE', *, *, #23394, .F. ) ;
#36757=CARTESIAN_POINT ( 'NONE',  ( 153.3040265531850537, -1.750000000000009992, -159.1817124430720298 ) ) ;
#36760=CARTESIAN_POINT ( 'NONE',  ( -46.69597344681494633, -1.750000000000010214, -39.18171244307202983 ) ) ;
#36766=ORIENTED_EDGE ( 'NONE', *, *, #3769, .F. ) ;
#36769=ORIENTED_EDGE ( 'NONE', *, *, #48091, .F. ) ;
#36777=VERTEX_POINT ( 'NONE', #35695 ) ;
#36780=EDGE_LOOP ( 'NONE', ( #32229, #42126, #34270, #11916, #42398, #42930 ) ) ;
#36789=SHAPE_REPRESENTATION_RELATIONSHIP ( 'NONE' , 'NONE' ,  #50327, #37482 ) ;
#36793=CARTESIAN_POINT ( 'NONE',  ( 152.2789002873379900, 1.750000000000009548, -160.2068387089191219 ) ) ;
#36794=DIRECTION ( 'NONE',  ( 0.000000000000000000, 0.000000000000000000, 1.000000000000000000 ) ) ;
#36802=EDGE_LOOP ( 'NONE', ( #24078, #22409, #40879, #5563, #13257, #15800 ) ) ;
#36805=CARTESIAN_POINT ( 'NONE',  ( -4.945973446814916130, 1.025126265847097651, -77.43171244307197298 ) ) ;
#36815=VECTOR ( 'NONE', #9495, 1000.000000000000000 ) ;
#36816=AXIS2_PLACEMENT_3D ( 'NONE', #6637, #38469, #45847 ) ;
#36820=AXIS2_PLACEMENT_3D ( 'NONE', #12577, #32094, #16442 ) ;
#36821=VERTEX_POINT ( 'NONE', #4117 ) ;
#36831=CARTESIAN_POINT ( 'NONE',  ( -48.44597344681495343, 0.000000000000000000, -120.9317124430720725 ) ) ;
#36837=FACE_OUTER_BOUND ( 'NONE', #17652, .T. ) ;
#36841=VERTEX_POINT ( 'NONE', #28732 ) ;
#36843=CARTESIAN_POINT ( 'NONE',  ( 33.30402655318503946, -1.750000000000009992, 0.8182875569279768335 ) ) ;
#36844=( BOUNDED_CURVE ( )  B_SPLINE_CURVE ( 3, ( #10887, #33999, #14738, #14484 ),
 .UNSPECIFIED., .F., .F. ) 
 B_SPLINE_CURVE_WITH_KNOTS ( ( 4, 4 ),
 ( 3.141592653589793116, 4.712388980384689674 ),
 .UNSPECIFIED. ) 
 CURVE ( )  GEOMETRIC_REPRESENTATION_ITEM ( )  RATIONAL_B_SPLINE_CURVE ( ( 1.000000000000000000, 0.8047378541243649375, 0.8047378541243649375, 1.000000000000000000 ) ) 
 REPRESENTATION_ITEM ( '' )  );
#36845=CARTESIAN_POINT ( 'NONE',  ( -206.6959734468149463, -1.750000000000009992, 0.8182875569279768335 ) ) ;
#36848=ADVANCED_FACE ( 'NONE', ( #13810 ), #13569, .F. ) ;
#36853=VERTEX_POINT ( 'NONE', #29234 ) ;
#36856=CYLINDRICAL_SURFACE ( 'NONE', #18551, 1.750000000000001554 ) ;
#36857=DIRECTION ( 'NONE',  ( 0.000000000000000000, 0.000000000000000000, -1.000000000000000000 ) ) ;
#36861=CARTESIAN_POINT ( 'NONE',  ( -208.4459734468148611, 1.025126265847089435, -40.93171244307204404 ) ) ;
#36864=EDGE_CURVE ( 'NONE', #47416, #2022, #22307, .T. ) ;
#36882=CARTESIAN_POINT ( 'NONE',  ( 113.3040265531850537, 0.000000000000000000, 165.0000000000000000 ) ) ;
#36883=CARTESIAN_POINT ( 'NONE',  ( -127.7210997126620242, 1.749999999999996891, -40.20683870891911482 ) ) ;
#36884=DIRECTION ( 'NONE',  ( -1.000000000000000000, -0.000000000000000000, -0.000000000000000000 ) ) ;
#36887=ORIENTED_EDGE ( 'NONE', *, *, #36620, .F. ) ;
#36891=CARTESIAN_POINT ( 'NONE',  ( 31.55402655318503236, 0.000000000000000000, -120.9317124430720725 ) ) ;
#36895=CARTESIAN_POINT ( 'NONE',  ( -166.6959734468149463, 1.750000000000009992, -159.1817124430720298 ) ) ;
#36900=EDGE_CURVE ( 'NONE', #27168, #31470, #47686, .T. ) ;
#36902=CYLINDRICAL_SURFACE ( 'NONE', #29145, 1.750000000000015543 ) ;
#36903=CYLINDRICAL_SURFACE ( 'NONE', #5404, 1.750000000000015543 ) ;
#36908=EDGE_LOOP ( 'NONE', ( #33171, #25375, #39866, #48304, #37744, #27236 ) ) ;
#36915=CARTESIAN_POINT ( 'NONE',  ( -44.94597344681493922, -1.025126265847089435, 122.5682875569280128 ) ) ;
#36916=CARTESIAN_POINT ( 'NONE',  ( -206.6959734468149463, 0.000000000000000000, -165.0000000000000000 ) ) ;
#36917=ADVANCED_FACE ( 'NONE', ( #40038 ), #47930, .T. ) ;
#36925=DIRECTION ( 'NONE',  ( -1.000000000000000000, -0.000000000000000000, -0.000000000000000000 ) ) ;
#36935=CARTESIAN_POINT ( 'NONE',  ( -206.6959734468149463, -1.750000000000010658, 80.81828755692798438 ) ) ;
#36942=ADVANCED_FACE ( 'NONE', ( #30236 ), #34104, .T. ) ;
#36946=DIRECTION ( 'NONE',  ( -0.000000000000000000, -0.000000000000000000, -1.000000000000000000 ) ) ;
#36947=LINE ( 'NONE', #29715, #46267 ) ;
#36949=CARTESIAN_POINT ( 'NONE',  ( 151.5540265531850537, 0.000000000000000000, 122.5682875569279702 ) ) ;
#36950=ORIENTED_EDGE ( 'NONE', *, *, #14848, .F. ) ;
#36951=VERTEX_POINT ( 'NONE', #41273 ) ;
#36956=ORIENTED_EDGE ( 'NONE', *, *, #2704, .F. ) ;
#36958=CARTESIAN_POINT ( 'NONE',  ( -44.94597344681493922, 2.143131898507880377E-16, -120.9317124430720725 ) ) ;
#36969=VERTEX_POINT ( 'NONE', #25637 ) ;
#36970=ORIENTED_EDGE ( 'NONE', *, *, #19577, .T. ) ;
#36972=CARTESIAN_POINT ( 'NONE',  ( 210.0000000000000568, 0.000000000000000000, -79.18171244307201562 ) ) ;
#36974=VERTEX_POINT ( 'NONE', #6630 ) ;
#36975=CYLINDRICAL_SURFACE ( 'NONE', #19178, 1.750000000000008438 ) ;
#36978=EDGE_CURVE ( 'NONE', #48741, #8469, #22530, .T. ) ;
#36980=ORIENTED_EDGE ( 'NONE', *, *, #45375, .F. ) ;
#36981=DIRECTION ( 'NONE',  ( -1.000000000000000000, -0.000000000000000000, -0.000000000000000000 ) ) ;
#36989=CARTESIAN_POINT ( 'NONE',  ( 210.0000000000000568, 0.000000000000000000, -157.4317124430720298 ) ) ;
#36990=( BOUNDED_CURVE ( )  B_SPLINE_CURVE ( 3, ( #15583, #689, #4540, #11991 ),
 .UNSPECIFIED., .F., .F. ) 
 B_SPLINE_CURVE_WITH_KNOTS ( ( 4, 4 ),
 ( 4.712388980384689674, 6.283185307179586232 ),
 .UNSPECIFIED. ) 
 CURVE ( )  GEOMETRIC_REPRESENTATION_ITEM ( )  RATIONAL_B_SPLINE_CURVE ( ( 1.000000000000000000, 0.8047378541243649375, 0.8047378541243649375, 1.000000000000000000 ) ) 
 REPRESENTATION_ITEM ( '' )  );
#36994=ORIENTED_EDGE ( 'NONE', *, *, #40212, .T. ) ;
#36995=DIRECTION ( 'NONE',  ( -0.000000000000000000, -0.000000000000000000, -1.000000000000000000 ) ) ;
#36997=( BOUNDED_CURVE ( )  B_SPLINE_CURVE ( 3, ( #13854, #22078, #45142, #41580 ),
 .UNSPECIFIED., .F., .F. ) 
 B_SPLINE_CURVE_WITH_KNOTS ( ( 4, 4 ),
 ( 0.000000000000000000, 1.570796326794896558 ),
 .UNSPECIFIED. ) 
 CURVE ( )  GEOMETRIC_REPRESENTATION_ITEM ( )  RATIONAL_B_SPLINE_CURVE ( ( 1.000000000000000000, 0.8047378541243649375, 0.8047378541243649375, 1.000000000000000000 ) ) 
 REPRESENTATION_ITEM ( '' )  );
#37000=DIRECTION ( 'NONE',  ( -0.000000000000000000, -0.000000000000000000, -1.000000000000000000 ) ) ;
#37007=ORIENTED_EDGE ( 'NONE', *, *, #41420, .F. ) ;
#37008=CARTESIAN_POINT ( 'NONE',  ( 75.05402655318509630, 1.025126265847089435, -157.4317124430720582 ) ) ;
#37009=VECTOR ( 'NONE', #1590, 1000.000000000000000 ) ;
#37010=DIRECTION ( 'NONE',  ( 0.000000000000000000, 0.000000000000000000, 1.000000000000000000 ) ) ;
#37011=( BOUNDED_CURVE ( )  B_SPLINE_CURVE ( 3, ( #48647, #24852, #29208, #39759 ),
 .UNSPECIFIED., .F., .F. ) 
 B_SPLINE_CURVE_WITH_KNOTS ( ( 4, 4 ),
 ( 1.570796326794896558, 3.141592653589793116 ),
 .UNSPECIFIED. ) 
 CURVE ( )  GEOMETRIC_REPRESENTATION_ITEM ( )  RATIONAL_B_SPLINE_CURVE ( ( 1.000000000000000000, 0.8047378541243649375, 0.8047378541243649375, 1.000000000000000000 ) ) 
 REPRESENTATION_ITEM ( '' )  );
#37015=CARTESIAN_POINT ( 'NONE',  ( 73.30402655318508209, 1.750000000000009992, -159.1817124430720298 ) ) ;
#37018=CARTESIAN_POINT ( 'NONE',  ( 74.32915281903215998, -1.750000000000009326, 159.7931612910809065 ) ) ;
#37020=ORIENTED_EDGE ( 'NONE', *, *, #38475, .F. ) ;
#37021=ORIENTED_EDGE ( 'NONE', *, *, #16957, .T. ) ;
#37025=DIRECTION ( 'NONE',  ( 1.000000000000000000, 0.000000000000000000, 0.000000000000000000 ) ) ;
#37026=CARTESIAN_POINT ( 'NONE',  ( 210.0000000000000568, 0.000000000000000000, -117.4317124430720298 ) ) ;
#37027=ORIENTED_EDGE ( 'NONE', *, *, #17326, .F. ) ;
#37037=ORIENTED_EDGE ( 'NONE', *, *, #8552, .F. ) ;
#37042=AXIS2_PLACEMENT_3D ( 'NONE', #26001, #33949, #41641 ) ;
#37044=DIRECTION ( 'NONE',  ( -1.000000000000000000, -0.000000000000000000, -0.000000000000000000 ) ) ;
#37045=ORIENTED_EDGE ( 'NONE', *, *, #19286, .T. ) ;
#37046=DIRECTION ( 'NONE',  ( -1.000000000000000000, -0.000000000000000000, -0.000000000000000000 ) ) ;
#37048=CARTESIAN_POINT ( 'NONE',  ( 154.3291528190321458, -1.750000000000009326, -158.1565861772249377 ) ) ;
#37049=CYLINDRICAL_SURFACE ( 'NONE', #16013, 1.750000000000015543 ) ;
#37050=CARTESIAN_POINT ( 'NONE',  ( 113.3040265531850537, 1.749999999999997335, 120.8182875569279702 ) ) ;
#37055=CARTESIAN_POINT ( 'NONE',  ( 210.0000000000000568, 0.000000000000000000, 160.8182875569279702 ) ) ;
#37056=LINE ( 'NONE', #1882, #39744 ) ;
#37059=PLANE ( 'NONE',  #47442 ) ;
#37061=CARTESIAN_POINT ( 'NONE',  ( 73.30402655318508209, -1.750000000000010658, -79.18171244307201562 ) ) ;
#37065=ORIENTED_EDGE ( 'NONE', *, *, #39511, .F. ) ;
#37071=CARTESIAN_POINT ( 'NONE',  ( -164.9459734468149463, 2.143131898507880377E-16, 82.56828755692798438 ) ) ;
#37073=ORIENTED_EDGE ( 'NONE', *, *, #16472, .F. ) ;
#37074=CARTESIAN_POINT ( 'NONE',  ( -46.69597344681494633, 0.000000000000000000, 165.0000000000000000 ) ) ;
#37078=ORIENTED_EDGE ( 'NONE', *, *, #46290, .F. ) ;
#37079=DIRECTION ( 'NONE',  ( -1.000000000000000000, 0.000000000000000000, 0.000000000000000000 ) ) ;
#37080=CARTESIAN_POINT ( 'NONE',  ( 34.32915281903212446, 1.750000000000009548, 41.84341382277508359 ) ) ;
#37082=LINE ( 'NONE', #1910, #11672 ) ;
#37085=ORIENTED_EDGE ( 'NONE', *, *, #17474, .F. ) ;
#37086=VECTOR ( 'NONE', #48051, 1000.000000000000000 ) ;
#37087=CARTESIAN_POINT ( 'NONE',  ( -8.445973446814964092, -1.025126265847097207, -40.93171244307204404 ) ) ;
#37088=DIRECTION ( 'NONE',  ( -1.000000000000000000, -0.000000000000000000, -0.000000000000000000 ) ) ;
#37095=ORIENTED_EDGE ( 'NONE', *, *, #16831, .T. ) ;
#37096=ORIENTED_EDGE ( 'NONE', *, *, #30711, .T. ) ;
#37099=CYLINDRICAL_SURFACE ( 'NONE', #22301, 1.750000000000008438 ) ;
#37100=ORIENTED_EDGE ( 'NONE', *, *, #47411, .T. ) ;
#37102=CARTESIAN_POINT ( 'NONE',  ( -204.9459734468149463, 2.143131898507880377E-16, 165.0000000000000000 ) ) ;
#37108=EDGE_CURVE ( 'NONE', #45829, #829, #8803, .T. ) ;
#37115=CARTESIAN_POINT ( 'NONE',  ( 111.5540265531850537, 1.025126265847081886, 119.0682875569279702 ) ) ;
#37119=EDGE_CURVE ( 'NONE', #26888, #9206, #32428, .T. ) ;
#37122=ORIENTED_EDGE ( 'NONE', *, *, #41613, .F. ) ;
#37130=DIRECTION ( 'NONE',  ( -0.000000000000000000, -0.000000000000000000, -1.000000000000000000 ) ) ;
#37134=CARTESIAN_POINT ( 'NONE',  ( 210.0000000000000568, 0.000000000000000000, 0.8182875569279768335 ) ) ;
#37145=( BOUNDED_CURVE ( )  B_SPLINE_CURVE ( 3, ( #45463, #10359, #44961, #2155 ),
 .UNSPECIFIED., .F., .F. ) 
 B_SPLINE_CURVE_WITH_KNOTS ( ( 4, 4 ),
 ( 3.141592653589793116, 4.712388980384689674 ),
 .UNSPECIFIED. ) 
 CURVE ( )  GEOMETRIC_REPRESENTATION_ITEM ( )  RATIONAL_B_SPLINE_CURVE ( ( 1.000000000000000000, 0.8047378541243649375, 0.8047378541243649375, 1.000000000000000000 ) ) 
 REPRESENTATION_ITEM ( '' )  );
#37146=CARTESIAN_POINT ( 'NONE',  ( 191.5540265531851105, 0.000000000000000000, 122.5682875569279702 ) ) ;
#37153=ORIENTED_EDGE ( 'NONE', *, *, #30487, .F. ) ;
#37162=FACE_OUTER_BOUND ( 'NONE', #24574, .T. ) ;
#37164=EDGE_CURVE ( 'NONE', #27926, #31866, #3842, .T. ) ;
#37168=CARTESIAN_POINT ( 'NONE',  ( 194.3291528190321742, 1.750000000000009548, 1.843413822775065825 ) ) ;
#37169=EDGE_CURVE ( 'NONE', #11965, #44183, #9811, .T. ) ;
#37175=ADVANCED_FACE ( 'NONE', ( #37551 ), #25988, .T. ) ;
#37185=CARTESIAN_POINT ( 'NONE',  ( -87.72109971266203843, 1.750000000000010436, -120.2068387089191219 ) ) ;
#37195=VERTEX_POINT ( 'NONE', #48781 ) ;
#37198=EDGE_CURVE ( 'NONE', #20525, #8314, #13903, .T. ) ;
#37202=CARTESIAN_POINT ( 'NONE',  ( -6.695973446814940111, -1.750000000000024203, -79.18171244307201562 ) ) ;
#37203=AXIS2_PLACEMENT_3D ( 'NONE', #36705, #17669, #16930 ) ;
#37204=VERTEX_POINT ( 'NONE', #41120 ) ;
#37207=EDGE_CURVE ( 'NONE', #4486, #43884, #41900, .T. ) ;
#37212=ORIENTED_EDGE ( 'NONE', *, *, #3999, .F. ) ;
#37215=CIRCLE ( 'NONE', #2776, 1.750000000000036193 ) ;
#37218=CARTESIAN_POINT ( 'NONE',  ( -164.9459734468149463, 2.143131898507880377E-16, -37.43171244307205825 ) ) ;
#37220=ORIENTED_EDGE ( 'NONE', *, *, #29078, .T. ) ;
#37221=VERTEX_POINT ( 'NONE', #6234 ) ;
#37223=CARTESIAN_POINT ( 'NONE',  ( 210.0000000000000568, 0.000000000000000000, 122.5682875569279844 ) ) ;
#37225=ORIENTED_EDGE ( 'NONE', *, *, #19223, .T. ) ;
#37226=DIRECTION ( 'NONE',  ( 0.000000000000000000, 0.000000000000000000, 1.000000000000000000 ) ) ;
#37227=DIRECTION ( 'NONE',  ( -0.000000000000000000, -0.000000000000000000, -1.000000000000000000 ) ) ;
#37229=FACE_OUTER_BOUND ( 'NONE', #14079, .T. ) ;
#37230=EDGE_CURVE ( 'NONE', #32429, #32609, #17328, .T. ) ;
#37234=DIRECTION ( 'NONE',  ( -0.000000000000000000, -0.000000000000000000, -1.000000000000000000 ) ) ;
#37235=CARTESIAN_POINT ( 'NONE',  ( 151.5540265531850537, 0.000000000000000000, 162.5682875569279702 ) ) ;
#37237=CARTESIAN_POINT ( 'NONE',  ( 71.55402655318505367, 0.000000000000000000, -77.43171244307198720 ) ) ;
#37244=CARTESIAN_POINT ( 'NONE',  ( -8.445973446814976526, 0.000000000000000000, 122.5682875569279986 ) ) ;
#37245=AXIS2_PLACEMENT_3D ( 'NONE', #6935, #3070, #2816 ) ;
#37248=CYLINDRICAL_SURFACE ( 'NONE', #28581, 1.750000000000015543 ) ;
#37249=FACE_OUTER_BOUND ( 'NONE', #33714, .T. ) ;
#37253=CARTESIAN_POINT ( 'NONE',  ( -168.4459734468149747, 1.025126265847088991, 2.568287556927986159 ) ) ;
#37256=EDGE_CURVE ( 'NONE', #40596, #20412, #32943, .T. ) ;
#37257=ORIENTED_EDGE ( 'NONE', *, *, #44118, .F. ) ;
#37261=ORIENTED_EDGE ( 'NONE', *, *, #34809, .F. ) ;
#37263=VECTOR ( 'NONE', #13407, 1000.000000000000000 ) ;
#37265=EDGE_CURVE ( 'NONE', #46038, #18302, #47405, .T. ) ;
#37269=CARTESIAN_POINT ( 'NONE',  ( -164.9459734468149463, 1.025126265847089879, -77.43171244307200141 ) ) ;
#37271=FACE_OUTER_BOUND ( 'NONE', #36534, .T. ) ;
#37272=VERTEX_POINT ( 'NONE', #25732 ) ;
#37276=EDGE_CURVE ( 'NONE', #30495, #27396, #50533, .T. ) ;
#37277=ADVANCED_FACE ( 'NONE', ( #19276 ), #34968, .T. ) ;
#37278=ORIENTED_EDGE ( 'NONE', *, *, #29967, .F. ) ;
#37282=ORIENTED_EDGE ( 'NONE', *, *, #26230, .T. ) ;
#37288=DIRECTION ( 'NONE',  ( -1.000000000000000000, -0.000000000000000000, -0.000000000000000000 ) ) ;
#37289=CARTESIAN_POINT ( 'NONE',  ( -88.44597344681497475, 0.000000000000000000, 79.06828755692795596 ) ) ;
#37290=( BOUNDED_CURVE ( )  B_SPLINE_CURVE ( 3, ( #19100, #31949, #46770, #30938 ),
 .UNSPECIFIED., .F., .F. ) 
 B_SPLINE_CURVE_WITH_KNOTS ( ( 4, 4 ),
 ( 3.141592653589793116, 4.712388980384689674 ),
 .UNSPECIFIED. ) 
 CURVE ( )  GEOMETRIC_REPRESENTATION_ITEM ( )  RATIONAL_B_SPLINE_CURVE ( ( 1.000000000000000000, 0.8047378541243649375, 0.8047378541243649375, 1.000000000000000000 ) ) 
 REPRESENTATION_ITEM ( '' )  );
#37294=DIRECTION ( 'NONE',  ( 0.000000000000000000, 0.000000000000000000, 1.000000000000000000 ) ) ;
#37295=CARTESIAN_POINT ( 'NONE',  ( -47.72109971266203132, 1.750000000000009548, 41.84341382277508359 ) ) ;
#37296=CARTESIAN_POINT ( 'NONE',  ( -46.69597344681494633, 1.750000000000010658, 80.81828755692798438 ) ) ;
#37297=( BOUNDED_CURVE ( )  B_SPLINE_CURVE ( 3, ( #20309, #4902, #8781, #44639 ),
 .UNSPECIFIED., .F., .F. ) 
 B_SPLINE_CURVE_WITH_KNOTS ( ( 4, 4 ),
 ( 0.000000000000000000, 1.570796326794896558 ),
 .UNSPECIFIED. ) 
 CURVE ( )  GEOMETRIC_REPRESENTATION_ITEM ( )  RATIONAL_B_SPLINE_CURVE ( ( 1.000000000000000000, 0.8047378541243649375, 0.8047378541243649375, 1.000000000000000000 ) ) 
 REPRESENTATION_ITEM ( '' )  );
#37299=CARTESIAN_POINT ( 'NONE',  ( -45.67084718096785423, 1.750000000000010214, -80.20683870891910772 ) ) ;
#37303=CARTESIAN_POINT ( 'NONE',  ( 193.3040265531851105, -1.750000000000010658, -119.1817124430720440 ) ) ;
#37304=DIRECTION ( 'NONE',  ( -0.000000000000000000, -0.000000000000000000, -1.000000000000000000 ) ) ;
#37305=CARTESIAN_POINT ( 'NONE',  ( 193.3040265531851105, 0.000000000000000000, 165.0000000000000000 ) ) ;
#37306=DIRECTION ( 'NONE',  ( 0.000000000000000000, 0.000000000000000000, 1.000000000000000000 ) ) ;
#37310=CARTESIAN_POINT ( 'NONE',  ( 195.0540265531851105, -1.025126265847089435, -40.93171244307204404 ) ) ;
#37313=EDGE_CURVE ( 'NONE', #16019, #36974, #6723, .T. ) ;
#37315=EDGE_LOOP ( 'NONE', ( #6326, #11804, #44576, #27004, #8357, #38264 ) ) ;
#37318=ORIENTED_EDGE ( 'NONE', *, *, #44118, .T. ) ;
#37337=ORIENTED_EDGE ( 'NONE', *, *, #1859, .T. ) ;
#37338=CARTESIAN_POINT ( 'NONE',  ( 155.0540265531850537, 1.025126265847089879, -77.43171244307200141 ) ) ;
#37340=CARTESIAN_POINT ( 'NONE',  ( 210.0000000000000568, 0.000000000000000000, -37.43171244307202272 ) ) ;
#37343=VERTEX_POINT ( 'NONE', #26480 ) ;
#37344=EDGE_CURVE ( 'NONE', #20584, #18366, #23172, .T. ) ;
#37349=VECTOR ( 'NONE', #9809, 1000.000000000000000 ) ;
#37351=ORIENTED_EDGE ( 'NONE', *, *, #31803, .F. ) ;
#37352=VECTOR ( 'NONE', #1735, 1000.000000000000000 ) ;
#37362=ORIENTED_EDGE ( 'NONE', *, *, #20797, .F. ) ;
#37366=CARTESIAN_POINT ( 'NONE',  ( 115.0540265531850395, 2.143131898507847836E-16, 165.0000000000000000 ) ) ;
#37368=LINE ( 'NONE', #2191, #34559 ) ;
#37379=ORIENTED_EDGE ( 'NONE', *, *, #31834, .T. ) ;
#37380=CARTESIAN_POINT ( 'NONE',  ( 111.5540265531850537, 1.025126265847081664, 122.5682875569279702 ) ) ;
#37387=LINE ( 'NONE', #17346, #13522 ) ;
#37388=EDGE_LOOP ( 'NONE', ( #4299, #48876, #21755, #35267, #8376, #3899 ) ) ;
#37390=CARTESIAN_POINT ( 'NONE',  ( -167.7210997126620384, 1.750000000000009548, -38.15658617722494483 ) ) ;
#37398=ORIENTED_EDGE ( 'NONE', *, *, #40106, .T. ) ;
#37406=EDGE_LOOP ( 'NONE', ( #38794, #34318, #7533, #8454, #26762, #27124 ) ) ;
#37407=VECTOR ( 'NONE', #20339, 1000.000000000000000 ) ;
#37410=CARTESIAN_POINT ( 'NONE',  ( 111.5540265531850679, 0.000000000000000000, 122.5682875569279560 ) ) ;
#37411=ORIENTED_EDGE ( 'NONE', *, *, #49136, .T. ) ;
#37412=CARTESIAN_POINT ( 'NONE',  ( -164.9459734468149463, 2.143131898507890731E-16, 165.0000000000000000 ) ) ;
#37419=LINE ( 'NONE', #26091, #22599 ) ;
#37424=( BOUNDED_CURVE ( )  B_SPLINE_CURVE ( 3, ( #48384, #41491, #6342, #2982 ),
 .UNSPECIFIED., .F., .F. ) 
 B_SPLINE_CURVE_WITH_KNOTS ( ( 4, 4 ),
 ( 3.141592653589793116, 4.712388980384689674 ),
 .UNSPECIFIED. ) 
 CURVE ( )  GEOMETRIC_REPRESENTATION_ITEM ( )  RATIONAL_B_SPLINE_CURVE ( ( 1.000000000000000000, 0.8047378541243649375, 0.8047378541243649375, 1.000000000000000000 ) ) 
 REPRESENTATION_ITEM ( '' )  );
#37426=ORIENTED_EDGE ( 'NONE', *, *, #14179, .F. ) ;
#37429=CARTESIAN_POINT ( 'NONE',  ( -85.67084718096784002, 1.750000000000009548, -158.1565861772249377 ) ) ;
#37430=ORIENTED_EDGE ( 'NONE', *, *, #30288, .F. ) ;
#37432=AXIS2_PLACEMENT_3D ( 'NONE', #5819, #33033, #40976 ) ;
#37433=CARTESIAN_POINT ( 'NONE',  ( 193.3040265531851105, 0.000000000000000000, 165.0000000000000000 ) ) ;
#37434=VECTOR ( 'NONE', #29368, 1000.000000000000000 ) ;
#37437=CARTESIAN_POINT ( 'NONE',  ( -8.445973446814964092, -1.025126265847097429, 119.0682875569279133 ) ) ;
#37438=CARTESIAN_POINT ( 'NONE',  ( -126.6959734468149321, 1.749999999999996891, 0.8182875569279768335 ) ) ;
#37440=( BOUNDED_CURVE ( )  B_SPLINE_CURVE ( 3, ( #13219, #1684, #44757, #25277 ),
 .UNSPECIFIED., .F., .F. ) 
 B_SPLINE_CURVE_WITH_KNOTS ( ( 4, 4 ),
 ( 1.570796326794896558, 3.141592653589793116 ),
 .UNSPECIFIED. ) 
 CURVE ( )  GEOMETRIC_REPRESENTATION_ITEM ( )  RATIONAL_B_SPLINE_CURVE ( ( 1.000000000000000000, 0.8047378541243649375, 0.8047378541243649375, 1.000000000000000000 ) ) 
 REPRESENTATION_ITEM ( '' )  );
#37441=ORIENTED_EDGE ( 'NONE', *, *, #23360, .F. ) ;
#37442=DIRECTION ( 'NONE',  ( -1.000000000000000000, -0.000000000000000000, -0.000000000000000000 ) ) ;
#37445=CARTESIAN_POINT ( 'NONE',  ( -86.69597344681494633, -1.750000000000010214, -39.18171244307202983 ) ) ;
#37449=CARTESIAN_POINT ( 'NONE',  ( -88.44597344681494633, 1.025126265847089435, 122.5682875569280128 ) ) ;
#37452=EDGE_CURVE ( 'NONE', #23796, #35947, #31865, .T. ) ;
#37453=LINE ( 'NONE', #5365, #43758 ) ;
#37455=ORIENTED_EDGE ( 'NONE', *, *, #33389, .T. ) ;
#37456=EDGE_CURVE ( 'NONE', #14077, #28486, #40064, .T. ) ;
#37459=DIRECTION ( 'NONE',  ( -0.000000000000000000, -0.000000000000000000, -1.000000000000000000 ) ) ;
#37460=EDGE_CURVE ( 'NONE', #16730, #48110, #33024, .T. ) ;
#37465=ORIENTED_EDGE ( 'NONE', *, *, #17538, .F. ) ;
#37466=VERTEX_POINT ( 'NONE', #16693 ) ;
#37471=CARTESIAN_POINT ( 'NONE',  ( -207.7210997126620384, 1.750000000000009548, -0.2068387089191121020 ) ) ;
#37474=CARTESIAN_POINT ( 'NONE',  ( 193.3040265531851105, -1.750000000000010658, 80.81828755692798438 ) ) ;
#37476=VERTEX_POINT ( 'NONE', #35730 ) ;
#37478=CARTESIAN_POINT ( 'NONE',  ( -86.69597344681494633, 1.750000000000010658, -79.18171244307201562 ) ) ;
#37481=EDGE_CURVE ( 'NONE', #7355, #22572, #12678, .T. ) ;
#37482=ADVANCED_BREP_SHAPE_REPRESENTATION ( '', ( #5787, #45486 ), #43870 ) ;
#37488=EDGE_CURVE ( 'NONE', #31049, #29572, #27994, .T. ) ;
#37490=CARTESIAN_POINT ( 'NONE',  ( 210.0000000000000568, 0.000000000000000000, -119.1817124430720440 ) ) ;
#37492=EDGE_CURVE ( 'NONE', #25713, #38146, #12092, .T. ) ;
#37498=EDGE_LOOP ( 'NONE', ( #19128, #47048, #20503, #8776, #28714, #26697 ) ) ;
#37501=CARTESIAN_POINT ( 'NONE',  ( -4.945973446814903696, 2.143131898507912917E-16, 42.56828755692802702 ) ) ;
#37502=EDGE_LOOP ( 'NONE', ( #38925, #1679, #20439, #35617, #3571 ) ) ;
#37503=DIRECTION ( 'NONE',  ( -0.000000000000000000, -0.000000000000000000, -1.000000000000000000 ) ) ;
#37504=FACE_OUTER_BOUND ( 'NONE', #37315, .T. ) ;
#37507=VERTEX_POINT ( 'NONE', #27501 ) ;
#37511=ORIENTED_EDGE ( 'NONE', *, *, #32922, .F. ) ;
#37512=CARTESIAN_POINT ( 'NONE',  ( 194.3291528190321742, 1.750000000000009326, 161.8434138227750907 ) ) ;
#37513=CARTESIAN_POINT ( 'NONE',  ( 210.0000000000000568, 0.000000000000000000, 2.568287556927987048 ) ) ;
#37514=CARTESIAN_POINT ( 'NONE',  ( -48.44597344681495343, 0.000000000000000000, -40.93171244307205825 ) ) ;
#37516=VERTEX_POINT ( 'NONE', #47206 ) ;
#37518=VERTEX_POINT ( 'NONE', #23897 ) ;
#37519=DIRECTION ( 'NONE',  ( 0.000000000000000000, 0.000000000000000000, 1.000000000000000000 ) ) ;
#37521=( BOUNDED_CURVE ( )  B_SPLINE_CURVE ( 3, ( #43030, #19698, #28162, #27146 ),
 .UNSPECIFIED., .F., .F. ) 
 B_SPLINE_CURVE_WITH_KNOTS ( ( 4, 4 ),
 ( 0.000000000000000000, 1.570796326794896558 ),
 .UNSPECIFIED. ) 
 CURVE ( )  GEOMETRIC_REPRESENTATION_ITEM ( )  RATIONAL_B_SPLINE_CURVE ( ( 1.000000000000000000, 0.8047378541243649375, 0.8047378541243649375, 1.000000000000000000 ) ) 
 REPRESENTATION_ITEM ( '' )  );
#37522=VERTEX_POINT ( 'NONE', #39562 ) ;
#37529=CARTESIAN_POINT ( 'NONE',  ( 210.0000000000000568, 0.000000000000000000, 120.8182875569279702 ) ) ;
#37531=CARTESIAN_POINT ( 'NONE',  ( -206.6959734468149463, 1.750000000000009992, 160.8182875569279702 ) ) ;
#37532=CARTESIAN_POINT ( 'NONE',  ( 210.0000000000000568, 2.143131898507881856E-16, -120.9317124430720582 ) ) ;
#37533=ORIENTED_EDGE ( 'NONE', *, *, #42158, .F. ) ;
#37535=EDGE_CURVE ( 'NONE', #9801, #8676, #33380, .T. ) ;
#37538=FACE_OUTER_BOUND ( 'NONE', #33959, .T. ) ;
#37541=CARTESIAN_POINT ( 'NONE',  ( 113.3040265531850537, 1.749999999999997113, 40.81828755692798438 ) ) ;
#37543=CARTESIAN_POINT ( 'NONE',  ( 75.05402655318509630, 2.143131898507880377E-16, -160.9317124430720582 ) ) ;
#37544=DIRECTION ( 'NONE',  ( -1.000000000000000000, -0.000000000000000000, -0.000000000000000000 ) ) ;
#37545=CARTESIAN_POINT ( 'NONE',  ( 153.3040265531850537, 1.750000000000009992, 0.8182875569279768335 ) ) ;
#37549=CARTESIAN_POINT ( 'NONE',  ( 210.0000000000000568, 0.000000000000000000, -79.18171244307201562 ) ) ;
#37550=DIRECTION ( 'NONE',  ( -0.000000000000000000, -0.000000000000000000, -1.000000000000000000 ) ) ;
#37551=FACE_OUTER_BOUND ( 'NONE', #44155, .T. ) ;
#37554=ADVANCED_FACE ( 'NONE', ( #17456 ), #9748, .T. ) ;
#37555=CARTESIAN_POINT ( 'NONE',  ( 115.0540265531850395, 2.143131898507847836E-16, -37.43171244307205825 ) ) ;
#37557=ADVANCED_FACE ( 'NONE', ( #9499 ), #1814, .T. ) ;
#37558=ADVANCED_FACE ( 'NONE', ( #2064 ), #44874, .T. ) ;
#37562=ORIENTED_EDGE ( 'NONE', *, *, #2894, .F. ) ;
#37566=CARTESIAN_POINT ( 'NONE',  ( -208.4459734468149463, 0.000000000000000000, -77.43171244307204404 ) ) ;
#37571=CARTESIAN_POINT ( 'NONE',  ( 195.0540265531851105, 2.143131898507880377E-16, 159.0682875569279702 ) ) ;
#37573=ORIENTED_EDGE ( 'NONE', *, *, #3061, .F. ) ;
#37575=LINE ( 'NONE', #14453, #12784 ) ;
#37577=( BOUNDED_CURVE ( )  B_SPLINE_CURVE ( 3, ( #29693, #45315, #13779, #9437 ),
 .UNSPECIFIED., .F., .F. ) 
 B_SPLINE_CURVE_WITH_KNOTS ( ( 4, 4 ),
 ( 4.712388980384689674, 6.283185307179586232 ),
 .UNSPECIFIED. ) 
 CURVE ( )  GEOMETRIC_REPRESENTATION_ITEM ( )  RATIONAL_B_SPLINE_CURVE ( ( 1.000000000000000000, 0.8047378541243649375, 0.8047378541243649375, 1.000000000000000000 ) ) 
 REPRESENTATION_ITEM ( '' )  );
#37578=AXIS2_PLACEMENT_3D ( 'NONE', #43702, #35533, #16268 ) ;
#37579=ORIENTED_EDGE ( 'NONE', *, *, #21460, .T. ) ;
#37582=CARTESIAN_POINT ( 'NONE',  ( -46.69597344681494633, 1.750000000000010658, -119.1817124430720440 ) ) ;
#37584=ORIENTED_EDGE ( 'NONE', *, *, #5322, .T. ) ;
#37586=VERTEX_POINT ( 'NONE', #5143 ) ;
#37587=( BOUNDED_CURVE ( )  B_SPLINE_CURVE ( 3, ( #13281, #26306, #33062, #6797 ),
 .UNSPECIFIED., .F., .F. ) 
 B_SPLINE_CURVE_WITH_KNOTS ( ( 4, 4 ),
 ( 3.141592653589793116, 4.712388980384689674 ),
 .UNSPECIFIED. ) 
 CURVE ( )  GEOMETRIC_REPRESENTATION_ITEM ( )  RATIONAL_B_SPLINE_CURVE ( ( 1.000000000000000000, 0.8047378541243649375, 0.8047378541243649375, 1.000000000000000000 ) ) 
 REPRESENTATION_ITEM ( '' )  );
#37591=EDGE_LOOP ( 'NONE', ( #33329, #41121, #34945, #33032, #3533, #50301 ) ) ;
#37592=CARTESIAN_POINT ( 'NONE',  ( -47.72109971266203132, -1.750000000000009548, -38.15658617722494483 ) ) ;
#37593=DIRECTION ( 'NONE',  ( -1.000000000000000000, -0.000000000000000000, -0.000000000000000000 ) ) ;
#37597=CARTESIAN_POINT ( 'NONE',  ( -48.44597344681495343, 0.000000000000000000, 165.0000000000000000 ) ) ;
#37600=CARTESIAN_POINT ( 'NONE',  ( 115.0540265531850395, 2.143131898507847836E-16, -80.93171244307201562 ) ) ;
#37601=CARTESIAN_POINT ( 'NONE',  ( -128.4459734468149179, 0.000000000000000000, 165.0000000000000000 ) ) ;
#37603=ADVANCED_FACE ( 'NONE', ( #9255 ), #16961, .T. ) ;
#37605=ORIENTED_EDGE ( 'NONE', *, *, #25600, .F. ) ;
#37609=CARTESIAN_POINT ( 'NONE',  ( -46.69597344681494633, 1.750000000000010658, -119.1817124430720440 ) ) ;
#37611=EDGE_CURVE ( 'NONE', #24770, #16975, #26171, .T. ) ;
#37615=CARTESIAN_POINT ( 'NONE',  ( 210.0000000000000568, 0.000000000000000000, 40.81828755692798438 ) ) ;
#37616=DIRECTION ( 'NONE',  ( -0.000000000000000000, -0.000000000000000000, -1.000000000000000000 ) ) ;
#37623=ORIENTED_EDGE ( 'NONE', *, *, #23723, .T. ) ;
#37625=AXIS2_PLACEMENT_3D ( 'NONE', #31114, #3651, #7252 ) ;
#37629=DIRECTION ( 'NONE',  ( 0.000000000000000000, 0.000000000000000000, 1.000000000000000000 ) ) ;
#37630=ORIENTED_EDGE ( 'NONE', *, *, #18145, .T. ) ;
#37635=ORIENTED_EDGE ( 'NONE', *, *, #43073, .F. ) ;
#37642=CARTESIAN_POINT ( 'NONE',  ( -87.72109971266203843, -1.750000000000009548, 1.843413822775065825 ) ) ;
#37644=DIRECTION ( 'NONE',  ( -1.000000000000000000, -0.000000000000000000, -0.000000000000000000 ) ) ;
#37645=ORIENTED_EDGE ( 'NONE', *, *, #29143, .T. ) ;
#37646=AXIS2_PLACEMENT_3D ( 'NONE', #6414, #21307, #9754 ) ;
#37647=FACE_OUTER_BOUND ( 'NONE', #38822, .T. ) ;
#37650=VERTEX_POINT ( 'NONE', #49468 ) ;
#37655=CARTESIAN_POINT ( 'NONE',  ( 210.0000000000000568, 2.143131898507881116E-16, -40.93171244307203693 ) ) ;
#37660=DIRECTION ( 'NONE',  ( 0.000000000000000000, 0.000000000000000000, 1.000000000000000000 ) ) ;
#37679=CARTESIAN_POINT ( 'NONE',  ( 155.0540265531850537, 1.025126265847089657, -37.43171244307202272 ) ) ;
#37686=CARTESIAN_POINT ( 'NONE',  ( 210.0000000000000568, 2.143131898507880377E-16, -0.9317124430720331585 ) ) ;
#37691=EDGE_LOOP ( 'NONE', ( #35994, #22066, #22777, #112, #29910, #5371 ) ) ;
#37695=CARTESIAN_POINT ( 'NONE',  ( -46.69597344681494633, -1.750000000000010658, 120.8182875569279702 ) ) ;
#37708=VERTEX_POINT ( 'NONE', #23063 ) ;
#37710=CYLINDRICAL_SURFACE ( 'NONE', #47935, 1.750000000000008438 ) ;
#37711=ORIENTED_EDGE ( 'NONE', *, *, #20903, .F. ) ;
#37714=CARTESIAN_POINT ( 'NONE',  ( 33.30402655318503946, -1.750000000000009992, 160.8182875569279702 ) ) ;
#37717=CARTESIAN_POINT ( 'NONE',  ( -87.72109971266203843, -1.750000000000010214, 119.7931612910808781 ) ) ;
#37719=CARTESIAN_POINT ( 'NONE',  ( -4.945973446814903696, 2.143131898507912917E-16, 82.56828755692801280 ) ) ;
#37721=CARTESIAN_POINT ( 'NONE',  ( 34.32915281903212446, 1.750000000000009548, -0.2068387089191121020 ) ) ;
#37722=DIRECTION ( 'NONE',  ( 1.000000000000000000, 0.000000000000000000, 0.000000000000000000 ) ) ;
#37723=AXIS2_PLACEMENT_3D ( 'NONE', #34292, #23511, #3997 ) ;
#37724=( BOUNDED_CURVE ( )  B_SPLINE_CURVE ( 3, ( #40487, #1738, #40230, #39736 ),
 .UNSPECIFIED., .F., .F. ) 
 B_SPLINE_CURVE_WITH_KNOTS ( ( 4, 4 ),
 ( 0.000000000000000000, 1.570796326794896558 ),
 .UNSPECIFIED. ) 
 CURVE ( )  GEOMETRIC_REPRESENTATION_ITEM ( )  RATIONAL_B_SPLINE_CURVE ( ( 1.000000000000000000, 0.8047378541243649375, 0.8047378541243649375, 1.000000000000000000 ) ) 
 REPRESENTATION_ITEM ( '' )  );
#37725=CIRCLE ( 'NONE', #31168, 1.749999999999987566 ) ;
#37727=ORIENTED_EDGE ( 'NONE', *, *, #40714, .F. ) ;
#37729=AXIS2_PLACEMENT_3D ( 'NONE', #9772, #33646, #25693 ) ;
#37730=CARTESIAN_POINT ( 'NONE',  ( 192.2789002873380184, -1.750000000000009548, -40.20683870891912193 ) ) ;
#37734=CARTESIAN_POINT ( 'NONE',  ( 193.3040265531851105, -1.750000000000010214, 40.81828755692798438 ) ) ;
#37735=ADVANCED_FACE ( 'NONE', ( #38738 ), #50478, .T. ) ;
#37736=FACE_OUTER_BOUND ( 'NONE', #50051, .T. ) ;
#37739=DIRECTION ( 'NONE',  ( 0.000000000000000000, 0.000000000000000000, 1.000000000000000000 ) ) ;
#37741=CARTESIAN_POINT ( 'NONE',  ( 112.2789002873379758, 1.749999999999996669, 81.84341382277506227 ) ) ;
#37742=ORIENTED_EDGE ( 'NONE', *, *, #24341, .T. ) ;
#37744=ORIENTED_EDGE ( 'NONE', *, *, #27216, .T. ) ;
#37748=CARTESIAN_POINT ( 'NONE',  ( -124.9459734468149321, -1.025126265847081664, 162.5682875569279133 ) ) ;
#37753=EDGE_CURVE ( 'NONE', #48199, #7390, #38933, .T. ) ;
#37757=CARTESIAN_POINT ( 'NONE',  ( 191.5540265531850537, -1.025126265847089657, -80.93171244307201562 ) ) ;
#37764=EDGE_CURVE ( 'NONE', #41270, #4446, #26165, .T. ) ;
#37765=ORIENTED_EDGE ( 'NONE', *, *, #10442, .F. ) ;
#37767=EDGE_CURVE ( 'NONE', #43082, #19505, #37985, .T. ) ;
#37769=EDGE_CURVE ( 'NONE', #14566, #50334, #38626, .T. ) ;
#37772=CARTESIAN_POINT ( 'NONE',  ( 31.55402655318503236, 1.025126265847088991, -157.4317124430720582 ) ) ;
#37773=ORIENTED_EDGE ( 'NONE', *, *, #22749, .T. ) ;
#37774=CARTESIAN_POINT ( 'NONE',  ( 151.5540265531850537, 0.000000000000000000, -120.9317124430720156 ) ) ;
#37779=CARTESIAN_POINT ( 'NONE',  ( -6.695973446814940111, -1.750000000000023315, 160.8182875569279702 ) ) ;
#37781=DIRECTION ( 'NONE',  ( -0.000000000000000000, -0.000000000000000000, -1.000000000000000000 ) ) ;
#37783=EDGE_LOOP ( 'NONE', ( #33874, #36970, #4291, #28759, #46962, #41428 ) ) ;
#37786=ORIENTED_EDGE ( 'NONE', *, *, #31661, .F. ) ;
#37790=EDGE_LOOP ( 'NONE', ( #38748, #45498, #3195, #21032, #5748, #15999 ) ) ;
#37793=DIRECTION ( 'NONE',  ( 1.000000000000000000, 0.000000000000000000, 0.000000000000000000 ) ) ;
#37796=EDGE_CURVE ( 'NONE', #29268, #42490, #14322, .T. ) ;
#37797=DIRECTION ( 'NONE',  ( -0.000000000000000000, -0.000000000000000000, -1.000000000000000000 ) ) ;
#37798=CARTESIAN_POINT ( 'NONE',  ( 210.0000000000000568, 0.000000000000000000, 80.81828755692798438 ) ) ;
#37801=CARTESIAN_POINT ( 'NONE',  ( -8.445973446814976526, 0.000000000000000000, 39.06828755692792754 ) ) ;
#37809=ORIENTED_EDGE ( 'NONE', *, *, #35008, .T. ) ;
#37814=CARTESIAN_POINT ( 'NONE',  ( -208.4459734468148611, -1.025126265847089879, -77.43171244307200141 ) ) ;
#37820=( BOUNDED_CURVE ( )  B_SPLINE_CURVE ( 3, ( #17444, #47944, #12836, #5129 ),
 .UNSPECIFIED., .F., .F. ) 
 B_SPLINE_CURVE_WITH_KNOTS ( ( 4, 4 ),
 ( 1.570796326794896558, 3.141592653589793116 ),
 .UNSPECIFIED. ) 
 CURVE ( )  GEOMETRIC_REPRESENTATION_ITEM ( )  RATIONAL_B_SPLINE_CURVE ( ( 1.000000000000000000, 0.8047378541243649375, 0.8047378541243649375, 1.000000000000000000 ) ) 
 REPRESENTATION_ITEM ( '' )  );
#37823=ORIENTED_EDGE ( 'NONE', *, *, #48630, .F. ) ;
#37828=ADVANCED_FACE ( 'NONE', ( #27434 ), #42813, .T. ) ;
#37831=ORIENTED_EDGE ( 'NONE', *, *, #43377, .F. ) ;
#37839=EDGE_CURVE ( 'NONE', #23935, #36821, #8484, .T. ) ;
#37850=EDGE_LOOP ( 'NONE', ( #44598, #12718, #11589, #47617, #5881, #47430 ) ) ;
#37851=CARTESIAN_POINT ( 'NONE',  ( 191.5540265531851105, 0.000000000000000000, -165.0000000000000000 ) ) ;
#37857=CARTESIAN_POINT ( 'NONE',  ( 73.30402655318508209, 1.750000000000010658, 80.81828755692798438 ) ) ;
#37863=CYLINDRICAL_SURFACE ( 'NONE', #30591, 1.749999999999987566 ) ;
#37864=CARTESIAN_POINT ( 'NONE',  ( -167.7210997126620384, 1.750000000000009326, -158.1565861772249377 ) ) ;
#37867=DIRECTION ( 'NONE',  ( -0.000000000000000000, -0.000000000000000000, -1.000000000000000000 ) ) ;
#37873=ORIENTED_EDGE ( 'NONE', *, *, #26864, .T. ) ;
#37875=( BOUNDED_CURVE ( )  B_SPLINE_CURVE ( 3, ( #2271, #17908, #35314, #27338 ),
 .UNSPECIFIED., .F., .F. ) 
 B_SPLINE_CURVE_WITH_KNOTS ( ( 4, 4 ),
 ( 1.570796326794896558, 3.141592653589793116 ),
 .UNSPECIFIED. ) 
 CURVE ( )  GEOMETRIC_REPRESENTATION_ITEM ( )  RATIONAL_B_SPLINE_CURVE ( ( 1.000000000000000000, 0.8047378541243649375, 0.8047378541243649375, 1.000000000000000000 ) ) 
 REPRESENTATION_ITEM ( '' )  );
#37880=( BOUNDED_CURVE ( )  B_SPLINE_CURVE ( 3, ( #40086, #36245, #28530, #17479 ),
 .UNSPECIFIED., .F., .F. ) 
 B_SPLINE_CURVE_WITH_KNOTS ( ( 4, 4 ),
 ( 0.000000000000000000, 1.570796326794896780 ),
 .UNSPECIFIED. ) 
 CURVE ( )  GEOMETRIC_REPRESENTATION_ITEM ( )  RATIONAL_B_SPLINE_CURVE ( ( 1.000000000000000000, 0.8047378541243649375, 0.8047378541243649375, 1.000000000000000000 ) ) 
 REPRESENTATION_ITEM ( '' )  );
#37884=DIRECTION ( 'NONE',  ( -0.000000000000000000, -0.000000000000000000, -1.000000000000000000 ) ) ;
#37889=CARTESIAN_POINT ( 'NONE',  ( -208.4459734468149463, 0.000000000000000000, -117.4317124430720725 ) ) ;
#37895=ADVANCED_FACE ( 'NONE', ( #45757 ), #14228, .T. ) ;
#37903=CARTESIAN_POINT ( 'NONE',  ( -206.6959734468149463, -1.750000000000010658, 80.81828755692798438 ) ) ;
#37909=LINE ( 'NONE', #2725, #27049 ) ;
#37913=CARTESIAN_POINT ( 'NONE',  ( 192.2789002873380184, 1.750000000000009548, 41.84341382277508359 ) ) ;
#37916=FACE_OUTER_BOUND ( 'NONE', #20563, .T. ) ;
#37918=EDGE_LOOP ( 'NONE', ( #20343, #2338, #38039, #37282, #42885, #29238 ) ) ;
#37925=CARTESIAN_POINT ( 'NONE',  ( -124.9459734468149463, 2.143131898507847836E-16, -120.9317124430720156 ) ) ;
#37927=ORIENTED_EDGE ( 'NONE', *, *, #36206, .F. ) ;
#37930=CARTESIAN_POINT ( 'NONE',  ( 71.55402655318505367, 0.000000000000000000, -117.4317124430720156 ) ) ;
#37932=AXIS2_PLACEMENT_3D ( 'NONE', #28203, #23852, #27445 ) ;
#37935=CARTESIAN_POINT ( 'NONE',  ( -168.4459734468149463, 0.000000000000000000, 119.0682875569279702 ) ) ;
#37942=CARTESIAN_POINT ( 'NONE',  ( 210.0000000000000568, 0.000000000000000000, 40.81828755692798438 ) ) ;
#37946=ORIENTED_EDGE ( 'NONE', *, *, #4805, .T. ) ;
#37949=VERTEX_POINT ( 'NONE', #33756 ) ;
#37954=DIRECTION ( 'NONE',  ( -1.000000000000000000, 0.000000000000000000, 0.000000000000000000 ) ) ;
#37955=EDGE_LOOP ( 'NONE', ( #22356, #37426, #43253, #12351, #41570, #37278 ) ) ;
#37958=ADVANCED_FACE ( 'NONE', ( #41690 ), #2686, .T. ) ;
#37959=ADVANCED_FACE ( 'NONE', ( #6795 ), #9885, .T. ) ;
#37961=ORIENTED_EDGE ( 'NONE', *, *, #27406, .T. ) ;
#37967=ORIENTED_EDGE ( 'NONE', *, *, #47434, .T. ) ;
#37969=ADVANCED_FACE ( 'NONE', ( #30147 ), #48843, .T. ) ;
#37976=CARTESIAN_POINT ( 'NONE',  ( 115.0540265531850395, 1.025126265847081886, 119.0682875569279702 ) ) ;
#37985=LINE ( 'NONE', #12281, #48567 ) ;
#37988=FACE_OUTER_BOUND ( 'NONE', #33950, .T. ) ;
#37990=CARTESIAN_POINT ( 'NONE',  ( 71.55402655318505367, 1.025126265847089213, 162.5682875569279133 ) ) ;
#37991=CARTESIAN_POINT ( 'NONE',  ( -88.44597344681491791, 0.000000000000000000, 162.5682875569279702 ) ) ;
#37996=DIRECTION ( 'NONE',  ( 0.000000000000000000, 0.000000000000000000, 1.000000000000000000 ) ) ;
#37997=AXIS2_PLACEMENT_3D ( 'NONE', #20574, #28279, #35234 ) ;
#37998=ORIENTED_EDGE ( 'NONE', *, *, #15135, .T. ) ;
#38002=CARTESIAN_POINT ( 'NONE',  ( 210.0000000000000568, 2.143131898507881116E-16, 39.06828755692797728 ) ) ;
#38005=ORIENTED_EDGE ( 'NONE', *, *, #12723, .F. ) ;
#38006=CARTESIAN_POINT ( 'NONE',  ( 191.5540265531851105, 0.000000000000000000, -80.93171244307201562 ) ) ;
#38010=CARTESIAN_POINT ( 'NONE',  ( -88.44597344681494633, -1.025126265847089879, -117.4317124430720156 ) ) ;
#38013=ORIENTED_EDGE ( 'NONE', *, *, #50683, .F. ) ;
#38015=( BOUNDED_CURVE ( )  B_SPLINE_CURVE ( 3, ( #8984, #40289, #8744, #16426 ),
 .UNSPECIFIED., .F., .F. ) 
 B_SPLINE_CURVE_WITH_KNOTS ( ( 4, 4 ),
 ( 1.570796326794896558, 3.141592653589793116 ),
 .UNSPECIFIED. ) 
 CURVE ( )  GEOMETRIC_REPRESENTATION_ITEM ( )  RATIONAL_B_SPLINE_CURVE ( ( 1.000000000000000000, 0.8047378541243649375, 0.8047378541243649375, 1.000000000000000000 ) ) 
 REPRESENTATION_ITEM ( '' )  );
#38023=( BOUNDED_CURVE ( )  B_SPLINE_CURVE ( 3, ( #45059, #42249, #41744, #18384 ),
 .UNSPECIFIED., .F., .F. ) 
 B_SPLINE_CURVE_WITH_KNOTS ( ( 4, 4 ),
 ( 1.570796326794896558, 3.141592653589793116 ),
 .UNSPECIFIED. ) 
 CURVE ( )  GEOMETRIC_REPRESENTATION_ITEM ( )  RATIONAL_B_SPLINE_CURVE ( ( 1.000000000000000000, 0.8047378541243649375, 0.8047378541243649375, 1.000000000000000000 ) ) 
 REPRESENTATION_ITEM ( '' )  );
#38024=CYLINDRICAL_SURFACE ( 'NONE', #21017, 1.750000000000001554 ) ;
#38037=ORIENTED_EDGE ( 'NONE', *, *, #41003, .F. ) ;
#38039=ORIENTED_EDGE ( 'NONE', *, *, #43521, .F. ) ;
#38043=DIRECTION ( 'NONE',  ( -0.000000000000000000, -0.000000000000000000, -1.000000000000000000 ) ) ;
#38046=CARTESIAN_POINT ( 'NONE',  ( 73.30402655318508209, -1.750000000000010214, 40.81828755692798438 ) ) ;
#38053=AXIS2_PLACEMENT_3D ( 'NONE', #6221, #45427, #41364 ) ;
#38057=ORIENTED_EDGE ( 'NONE', *, *, #11198, .F. ) ;
#38058=DIRECTION ( 'NONE',  ( -0.000000000000000000, -0.000000000000000000, -1.000000000000000000 ) ) ;
#38061=VERTEX_POINT ( 'NONE', #23472 ) ;
#38062=CARTESIAN_POINT ( 'NONE',  ( -4.945973446814903696, 2.143131898507912917E-16, 165.0000000000000000 ) ) ;
#38063=ORIENTED_EDGE ( 'NONE', *, *, #25263, .F. ) ;
#38069=ORIENTED_EDGE ( 'NONE', *, *, #41930, .T. ) ;
#38070=VERTEX_POINT ( 'NONE', #39134 ) ;
#38088=AXIS2_PLACEMENT_3D ( 'NONE', #36544, #1380, #21113 ) ;
#38094=ORIENTED_EDGE ( 'NONE', *, *, #28505, .T. ) ;
#38096=VERTEX_POINT ( 'NONE', #47019 ) ;
#38099=EDGE_LOOP ( 'NONE', ( #26071, #864, #39291, #36365, #31722, #43557 ) ) ;
#38107=CARTESIAN_POINT ( 'NONE',  ( 210.0000000000000568, 0.000000000000000000, -119.1817124430720440 ) ) ;
#38115=( BOUNDED_CURVE ( )  B_SPLINE_CURVE ( 3, ( #30633, #33977, #49564, #38343 ),
 .UNSPECIFIED., .F., .F. ) 
 B_SPLINE_CURVE_WITH_KNOTS ( ( 4, 4 ),
 ( 0.000000000000000000, 1.570796326794896558 ),
 .UNSPECIFIED. ) 
 CURVE ( )  GEOMETRIC_REPRESENTATION_ITEM ( )  RATIONAL_B_SPLINE_CURVE ( ( 1.000000000000000000, 0.8047378541243649375, 0.8047378541243649375, 1.000000000000000000 ) ) 
 REPRESENTATION_ITEM ( '' )  );
#38116=CARTESIAN_POINT ( 'NONE',  ( 113.3040265531850537, -1.749999999999996891, 0.8182875569279768335 ) ) ;
#38132=ORIENTED_EDGE ( 'NONE', *, *, #807, .T. ) ;
#38140=CARTESIAN_POINT ( 'NONE',  ( 210.0000000000000568, 0.000000000000000000, -37.43171244307202272 ) ) ;
#38142=CARTESIAN_POINT ( 'NONE',  ( 195.0540265531851105, 2.143131898507880377E-16, -37.43171244307205825 ) ) ;
#38145=VERTEX_POINT ( 'NONE', #48278 ) ;
#38146=VERTEX_POINT ( 'NONE', #4467 ) ;
#38150=CARTESIAN_POINT ( 'NONE',  ( 111.5540265531850679, 0.000000000000000000, -37.43171244307205825 ) ) ;
#38154=DIRECTION ( 'NONE',  ( -0.000000000000000000, -0.000000000000000000, -1.000000000000000000 ) ) ;
#38159=ADVANCED_FACE ( 'NONE', ( #630 ), #40135, .T. ) ;
#38167=CARTESIAN_POINT ( 'NONE',  ( 210.0000000000000568, 0.000000000000000000, 40.81828755692798438 ) ) ;
#38171=CIRCLE ( 'NONE', #29948, 1.750000000000001554 ) ;
#38174=DIRECTION ( 'NONE',  ( 1.000000000000000000, 0.000000000000000000, 0.000000000000000000 ) ) ;
#38175=CARTESIAN_POINT ( 'NONE',  ( -86.69597344681494633, -1.750000000000010658, -119.1817124430720440 ) ) ;
#38178=CARTESIAN_POINT ( 'NONE',  ( 210.0000000000000568, 0.000000000000000000, -119.1817124430720440 ) ) ;
#38179=( BOUNDED_CURVE ( )  B_SPLINE_CURVE ( 3, ( #46118, #7942, #12040, #46627 ),
 .UNSPECIFIED., .F., .F. ) 
 B_SPLINE_CURVE_WITH_KNOTS ( ( 4, 4 ),
 ( 3.141592653589793116, 4.712388980384689674 ),
 .UNSPECIFIED. ) 
 CURVE ( )  GEOMETRIC_REPRESENTATION_ITEM ( )  RATIONAL_B_SPLINE_CURVE ( ( 1.000000000000000000, 0.8047378541243649375, 0.8047378541243649375, 1.000000000000000000 ) ) 
 REPRESENTATION_ITEM ( '' )  );
#38186=( BOUNDED_CURVE ( )  B_SPLINE_CURVE ( 3, ( #12109, #569, #32617, #5147 ),
 .UNSPECIFIED., .F., .F. ) 
 B_SPLINE_CURVE_WITH_KNOTS ( ( 4, 4 ),
 ( 1.570796326794896558, 3.141592653589793116 ),
 .UNSPECIFIED. ) 
 CURVE ( )  GEOMETRIC_REPRESENTATION_ITEM ( )  RATIONAL_B_SPLINE_CURVE ( ( 1.000000000000000000, 0.8047378541243649375, 0.8047378541243649375, 1.000000000000000000 ) ) 
 REPRESENTATION_ITEM ( '' )  );
#38188=DIRECTION ( 'NONE',  ( -0.000000000000000000, -0.000000000000000000, -1.000000000000000000 ) ) ;
#38194=EDGE_LOOP ( 'NONE', ( #35054, #23436, #9991, #41651, #50596, #14469 ) ) ;
#38195=ORIENTED_EDGE ( 'NONE', *, *, #46586, .T. ) ;
#38197=DIRECTION ( 'NONE',  ( -1.000000000000000000, 0.000000000000000000, 0.000000000000000000 ) ) ;
#38199=CARTESIAN_POINT ( 'NONE',  ( -88.44597344681497475, 0.000000000000000000, -40.93171244307205825 ) ) ;
#38202=CYLINDRICAL_SURFACE ( 'NONE', #49437, 1.750000000000001554 ) ;
#38204=ORIENTED_EDGE ( 'NONE', *, *, #49663, .T. ) ;
#38205=FACE_OUTER_BOUND ( 'NONE', #18841, .T. ) ;
#38208=CARTESIAN_POINT ( 'NONE',  ( -127.7210997126620242, 1.749999999999996891, 39.79316129108089228 ) ) ;
#38211=CARTESIAN_POINT ( 'NONE',  ( 210.0000000000000568, 0.000000000000000000, 42.56828755692799149 ) ) ;
#38216=CARTESIAN_POINT ( 'NONE',  ( -88.44597344681494633, 1.025126265847089435, 82.56828755692798438 ) ) ;
#38220=VERTEX_POINT ( 'NONE', #14164 ) ;
#38221=CARTESIAN_POINT ( 'NONE',  ( -8.445973446814964092, -1.025126265847097429, 79.06828755692792754 ) ) ;
#38223=ORIENTED_EDGE ( 'NONE', *, *, #3704, .T. ) ;
#38224=VECTOR ( 'NONE', #43062, 1000.000000000000000 ) ;
#38225=ORIENTED_EDGE ( 'NONE', *, *, #49310, .T. ) ;
#38234=CARTESIAN_POINT ( 'NONE',  ( -46.69597344681494633, 1.750000000000010214, 40.81828755692798438 ) ) ;
#38236=CARTESIAN_POINT ( 'NONE',  ( 193.3040265531851105, 0.000000000000000000, 165.0000000000000000 ) ) ;
#38237=DIRECTION ( 'NONE',  ( -0.000000000000000000, -0.000000000000000000, -1.000000000000000000 ) ) ;
#38238=ORIENTED_EDGE ( 'NONE', *, *, #38410, .T. ) ;
#38243=VECTOR ( 'NONE', #30622, 1000.000000000000000 ) ;
#38245=AXIS2_PLACEMENT_3D ( 'NONE', #5191, #37288, #25708 ) ;
#38248=CARTESIAN_POINT ( 'NONE',  ( -164.9459734468149463, 1.025126265847089657, 119.0682875569279560 ) ) ;
#38252=DIRECTION ( 'NONE',  ( -0.000000000000000000, -0.000000000000000000, -1.000000000000000000 ) ) ;
#38253=ADVANCED_FACE ( 'NONE', ( #41382 ), #25740, .T. ) ;
#38256=EDGE_LOOP ( 'NONE', ( #50511, #44051, #17506, #22002, #15977, #1343 ) ) ;
#38257=ORIENTED_EDGE ( 'NONE', *, *, #11088, .F. ) ;
#38258=CARTESIAN_POINT ( 'NONE',  ( -6.695973446814940111, 1.750000000000023315, 160.8182875569279702 ) ) ;
#38263=CYLINDRICAL_SURFACE ( 'NONE', #37245, 1.750000000000001554 ) ;
#38264=ORIENTED_EDGE ( 'NONE', *, *, #7621, .F. ) ;
#38265=CYLINDRICAL_SURFACE ( 'NONE', #28138, 1.750000000000015543 ) ;
#38266=ORIENTED_EDGE ( 'NONE', *, *, #18323, .F. ) ;
#38270=CARTESIAN_POINT ( 'NONE',  ( 71.55402655318505367, 0.000000000000000000, -37.43171244307200141 ) ) ;
#38275=CYLINDRICAL_SURFACE ( 'NONE', #48620, 1.750000000000001554 ) ;
#38280=ORIENTED_EDGE ( 'NONE', *, *, #23609, .F. ) ;
#38284=FACE_OUTER_BOUND ( 'NONE', #10854, .T. ) ;
#38285=ORIENTED_EDGE ( 'NONE', *, *, #39131, .F. ) ;
#38287=EDGE_CURVE ( 'NONE', #40841, #41782, #12382, .T. ) ;
#38288=CARTESIAN_POINT ( 'NONE',  ( -208.4459734468148611, 1.025126265847089435, -77.43171244307200141 ) ) ;
#38307=LINE ( 'NONE', #11079, #15958 ) ;
#38312=DIRECTION ( 'NONE',  ( -0.000000000000000000, -0.000000000000000000, -1.000000000000000000 ) ) ;
#38316=EDGE_LOOP ( 'NONE', ( #43612, #21676, #22290, #19797, #41073, #22655 ) ) ;
#38322=( BOUNDED_CURVE ( )  B_SPLINE_CURVE ( 3, ( #1486, #28924, #35888, #20457 ),
 .UNSPECIFIED., .F., .F. ) 
 B_SPLINE_CURVE_WITH_KNOTS ( ( 4, 4 ),
 ( 3.141592653589793116, 4.712388980384689674 ),
 .UNSPECIFIED. ) 
 CURVE ( )  GEOMETRIC_REPRESENTATION_ITEM ( )  RATIONAL_B_SPLINE_CURVE ( ( 1.000000000000000000, 0.8047378541243649375, 0.8047378541243649375, 1.000000000000000000 ) ) 
 REPRESENTATION_ITEM ( '' )  );
#38324=ORIENTED_EDGE ( 'NONE', *, *, #35334, .T. ) ;
#38326=CARTESIAN_POINT ( 'NONE',  ( 210.0000000000000568, 0.000000000000000000, -39.18171244307202983 ) ) ;
#38329=ORIENTED_EDGE ( 'NONE', *, *, #41582, .F. ) ;
#38333=VERTEX_POINT ( 'NONE', #49780 ) ;
#38335=CARTESIAN_POINT ( 'NONE',  ( 34.32915281903212446, 1.750000000000010214, -120.2068387089191219 ) ) ;
#38340=ORIENTED_EDGE ( 'NONE', *, *, #36436, .T. ) ;
#38341=( BOUNDED_CURVE ( )  B_SPLINE_CURVE ( 3, ( #18869, #34550, #35329, #46306 ),
 .UNSPECIFIED., .F., .F. ) 
 B_SPLINE_CURVE_WITH_KNOTS ( ( 4, 4 ),
 ( 0.000000000000000000, 1.570796326794896558 ),
 .UNSPECIFIED. ) 
 CURVE ( )  GEOMETRIC_REPRESENTATION_ITEM ( )  RATIONAL_B_SPLINE_CURVE ( ( 1.000000000000000000, 0.8047378541243649375, 0.8047378541243649375, 1.000000000000000000 ) ) 
 REPRESENTATION_ITEM ( '' )  );
#38343=CARTESIAN_POINT ( 'NONE',  ( -46.69597344681494633, -1.750000000000010658, -119.1817124430720440 ) ) ;
#38345=AXIS2_PLACEMENT_3D ( 'NONE', #29377, #48579, #36857 ) ;
#38346=ORIENTED_EDGE ( 'NONE', *, *, #47904, .T. ) ;
#38347=ORIENTED_EDGE ( 'NONE', *, *, #22132, .F. ) ;
#38350=ORIENTED_EDGE ( 'NONE', *, *, #42108, .T. ) ;
#38358=DIRECTION ( 'NONE',  ( -0.000000000000000000, -0.000000000000000000, -1.000000000000000000 ) ) ;
#38363=FACE_OUTER_BOUND ( 'NONE', #9624, .T. ) ;
#38370=CARTESIAN_POINT ( 'NONE',  ( -88.44597344681497475, 0.000000000000000000, 165.0000000000000000 ) ) ;
#38373=ORIENTED_EDGE ( 'NONE', *, *, #30351, .F. ) ;
#38380=EDGE_CURVE ( 'NONE', #11761, #35393, #5487, .T. ) ;
#38383=ORIENTED_EDGE ( 'NONE', *, *, #27069, .T. ) ;
#38385=EDGE_CURVE ( 'NONE', #26183, #36777, #27832, .T. ) ;
#38387=ORIENTED_EDGE ( 'NONE', *, *, #48675, .T. ) ;
#38389=DIRECTION ( 'NONE',  ( 0.000000000000000000, 0.000000000000000000, 1.000000000000000000 ) ) ;
#38394=ADVANCED_FACE ( 'NONE', ( #9015 ), #16210, .F. ) ;
#38395=ADVANCED_FACE ( 'NONE', ( #40319 ), #32370, .T. ) ;
#38399=EDGE_CURVE ( 'NONE', #5180, #13146, #31433, .T. ) ;
#38403=CARTESIAN_POINT ( 'NONE',  ( 113.3040265531850537, 0.000000000000000000, -165.0000000000000000 ) ) ;
#38410=EDGE_CURVE ( 'NONE', #41166, #35123, #47101, .T. ) ;
#38412=ORIENTED_EDGE ( 'NONE', *, *, #25887, .T. ) ;
#38417=AXIS2_PLACEMENT_3D ( 'NONE', #45508, #41945, #30145 ) ;
#38418=DIRECTION ( 'NONE',  ( -1.000000000000000000, -0.000000000000000000, -0.000000000000000000 ) ) ;
#38420=CARTESIAN_POINT ( 'NONE',  ( 111.5540265531850679, 0.000000000000000000, 165.0000000000000000 ) ) ;
#38424=EDGE_CURVE ( 'NONE', #7516, #16448, #49349, .T. ) ;
#38426=EDGE_CURVE ( 'NONE', #43884, #13365, #8777, .T. ) ;
#38431=DIRECTION ( 'NONE',  ( -0.000000000000000000, -0.000000000000000000, -1.000000000000000000 ) ) ;
#38433=EDGE_CURVE ( 'NONE', #20298, #5511, #24425, .T. ) ;
#38439=CARTESIAN_POINT ( 'NONE',  ( -7.721099712662037540, 1.750000000000022871, 159.7931612910808781 ) ) ;
#38441=CARTESIAN_POINT ( 'NONE',  ( 75.05402655318509630, 2.143131898507880377E-16, 2.568287556928006143 ) ) ;
#38442=VERTEX_POINT ( 'NONE', #4158 ) ;
#38451=VERTEX_POINT ( 'NONE', #27758 ) ;
#38455=CARTESIAN_POINT ( 'NONE',  ( -206.6959734468149463, 1.750000000000010658, -119.1817124430720440 ) ) ;
#38456=CIRCLE ( 'NONE', #24528, 1.750000000000015543 ) ;
#38457=AXIS2_PLACEMENT_3D ( 'NONE', #20017, #12078, #24392 ) ;
#38460=ORIENTED_EDGE ( 'NONE', *, *, #36636, .T. ) ;
#38461=DIRECTION ( 'NONE',  ( 0.000000000000000000, 0.000000000000000000, 1.000000000000000000 ) ) ;
#38462=CARTESIAN_POINT ( 'NONE',  ( 32.27890028733795447, 1.750000000000009548, 161.8434138227750907 ) ) ;
#38466=VERTEX_POINT ( 'NONE', #44633 ) ;
#38467=EDGE_CURVE ( 'NONE', #19269, #40908, #2314, .T. ) ;
#38469=DIRECTION ( 'NONE',  ( -1.000000000000000000, -0.000000000000000000, -0.000000000000000000 ) ) ;
#38475=EDGE_CURVE ( 'NONE', #23653, #23447, #45763, .T. ) ;
#38478=EDGE_LOOP ( 'NONE', ( #39366, #40291 ) ) ;
#38491=DIRECTION ( 'NONE',  ( -1.000000000000000000, -0.000000000000000000, -0.000000000000000000 ) ) ;
#38494=CARTESIAN_POINT ( 'NONE',  ( -126.6959734468149321, -1.749999999999997335, -119.1817124430720440 ) ) ;
#38496=EDGE_LOOP ( 'NONE', ( #10248, #37465, #31271, #20486, #33724, #8046 ) ) ;
#38500=DIRECTION ( 'NONE',  ( 0.000000000000000000, 0.000000000000000000, 1.000000000000000000 ) ) ;
#38502=DIRECTION ( 'NONE',  ( -1.000000000000000000, -0.000000000000000000, -0.000000000000000000 ) ) ;
#38504=AXIS2_PLACEMENT_3D ( 'NONE', #12740, #24545, #9647 ) ;
#38505=ORIENTED_EDGE ( 'NONE', *, *, #43417, .T. ) ;
#38506=ORIENTED_EDGE ( 'NONE', *, *, #29030, .T. ) ;
#38509=CARTESIAN_POINT ( 'NONE',  ( 155.0540265531850537, 2.143131898507880377E-16, -160.9317124430720014 ) ) ;
#38511=FACE_OUTER_BOUND ( 'NONE', #32656, .T. ) ;
#38513=ORIENTED_EDGE ( 'NONE', *, *, #49310, .F. ) ;
#38516=VERTEX_POINT ( 'NONE', #40815 ) ;
#38519=CARTESIAN_POINT ( 'NONE',  ( -6.695973446814940111, -1.750000000000024203, -79.18171244307201562 ) ) ;
#38524=CARTESIAN_POINT ( 'NONE',  ( 153.3040265531850537, 1.750000000000009992, 0.8182875569279768335 ) ) ;
#38530=FACE_OUTER_BOUND ( 'NONE', #40214, .T. ) ;
#38532=ORIENTED_EDGE ( 'NONE', *, *, #39811, .T. ) ;
#38535=EDGE_CURVE ( 'NONE', #25164, #3012, #13612, .T. ) ;
#38537=VERTEX_POINT ( 'NONE', #13104 ) ;
#38539=EDGE_CURVE ( 'NONE', #21304, #41284, #22068, .T. ) ;
#38540=CARTESIAN_POINT ( 'NONE',  ( -47.72109971266203132, -1.750000000000009548, -158.1565861772249377 ) ) ;
#38544=DIRECTION ( 'NONE',  ( 0.000000000000000000, 0.000000000000000000, -1.000000000000000000 ) ) ;
#38557=CARTESIAN_POINT ( 'NONE',  ( -166.6959734468149463, -1.750000000000010658, -119.1817124430720440 ) ) ;
#38559=CARTESIAN_POINT ( 'NONE',  ( 155.0540265531850537, 2.143131898507880377E-16, 39.06828755692798438 ) ) ;
#38561=CARTESIAN_POINT ( 'NONE',  ( 32.27890028733795447, -1.750000000000009548, -158.1565861772249377 ) ) ;
#38566=CARTESIAN_POINT ( 'NONE',  ( 71.55402655318505367, -1.025126265847089213, 159.0682875569279418 ) ) ;
#38568=VERTEX_POINT ( 'NONE', #21062 ) ;
#38569=AXIS2_PLACEMENT_3D ( 'NONE', #25582, #8112, #7600 ) ;
#38570=CARTESIAN_POINT ( 'NONE',  ( -206.6959734468149463, 0.000000000000000000, 165.0000000000000000 ) ) ;
#38574=DIRECTION ( 'NONE',  ( 0.000000000000000000, 0.000000000000000000, 1.000000000000000000 ) ) ;
#38581=CARTESIAN_POINT ( 'NONE',  ( 35.05402655318504657, 2.143131898507880377E-16, 82.56828755692798438 ) ) ;
#38582=CYLINDRICAL_SURFACE ( 'NONE', #22570, 1.750000000000001554 ) ;
#38584=ORIENTED_EDGE ( 'NONE', *, *, #19903, .F. ) ;
#38588=ORIENTED_EDGE ( 'NONE', *, *, #25580, .T. ) ;
#38590=CARTESIAN_POINT ( 'NONE',  ( 35.05402655318504657, 2.143131898507880377E-16, 42.56828755692798438 ) ) ;
#38595=CARTESIAN_POINT ( 'NONE',  ( 194.3291528190321742, -1.750000000000009548, 81.84341382277507648 ) ) ;
#38596=AXIS2_PLACEMENT_3D ( 'NONE', #43405, #19547, #23663 ) ;
#38602=CARTESIAN_POINT ( 'NONE',  ( -6.695973446814940111, 1.750000000000023315, 160.8182875569279702 ) ) ;
#38603=ADVANCED_FACE ( 'NONE', ( #33387 ), #41321, .T. ) ;
#38609=VERTEX_POINT ( 'NONE', #34391 ) ;
#38615=CARTESIAN_POINT ( 'NONE',  ( 210.0000000000000568, 2.143131898507881856E-16, 79.06828755692797017 ) ) ;
#38620=DIRECTION ( 'NONE',  ( 0.000000000000000000, 0.000000000000000000, -1.000000000000000000 ) ) ;
#38621=( BOUNDED_CURVE ( )  B_SPLINE_CURVE ( 3, ( #903, #21386, #32967, #40897 ),
 .UNSPECIFIED., .F., .F. ) 
 B_SPLINE_CURVE_WITH_KNOTS ( ( 4, 4 ),
 ( 1.570796326794896558, 3.141592653589793116 ),
 .UNSPECIFIED. ) 
 CURVE ( )  GEOMETRIC_REPRESENTATION_ITEM ( )  RATIONAL_B_SPLINE_CURVE ( ( 1.000000000000000000, 0.8047378541243649375, 0.8047378541243649375, 1.000000000000000000 ) ) 
 REPRESENTATION_ITEM ( '' )  );
#38626=( BOUNDED_CURVE ( )  B_SPLINE_CURVE ( 3, ( #44505, #11537, #3826, #252 ),
 .UNSPECIFIED., .F., .F. ) 
 B_SPLINE_CURVE_WITH_KNOTS ( ( 4, 4 ),
 ( 0.000000000000000000, 1.570796326794896780 ),
 .UNSPECIFIED. ) 
 CURVE ( )  GEOMETRIC_REPRESENTATION_ITEM ( )  RATIONAL_B_SPLINE_CURVE ( ( 1.000000000000000000, 0.8047378541243649375, 0.8047378541243649375, 1.000000000000000000 ) ) 
 REPRESENTATION_ITEM ( '' )  );
#38627=CARTESIAN_POINT ( 'NONE',  ( 193.3040265531851105, 0.000000000000000000, 165.0000000000000000 ) ) ;
#38629=VECTOR ( 'NONE', #31147, 1000.000000000000000 ) ;
#38634=( BOUNDED_CURVE ( )  B_SPLINE_CURVE ( 3, ( #44742, #37592, #33737, #9617 ),
 .UNSPECIFIED., .F., .F. ) 
 B_SPLINE_CURVE_WITH_KNOTS ( ( 4, 4 ),
 ( 1.570796326794896558, 3.141592653589793116 ),
 .UNSPECIFIED. ) 
 CURVE ( )  GEOMETRIC_REPRESENTATION_ITEM ( )  RATIONAL_B_SPLINE_CURVE ( ( 1.000000000000000000, 0.8047378541243649375, 0.8047378541243649375, 1.000000000000000000 ) ) 
 REPRESENTATION_ITEM ( '' )  );
#38637=ORIENTED_EDGE ( 'NONE', *, *, #40912, .T. ) ;
#38638=CARTESIAN_POINT ( 'NONE',  ( 210.0000000000000568, 0.000000000000000000, -159.1817124430720298 ) ) ;
#38642=CARTESIAN_POINT ( 'NONE',  ( -44.94597344681493922, 1.025126265847089657, -37.43171244307202272 ) ) ;
#38643=CARTESIAN_POINT ( 'NONE',  ( -124.9459734468149321, -1.025126265847081219, -157.4317124430720582 ) ) ;
#38646=VERTEX_POINT ( 'NONE', #14619 ) ;
#38649=CARTESIAN_POINT ( 'NONE',  ( -85.67084718096784002, 1.750000000000009548, 159.7931612910809065 ) ) ;
#38655=FACE_OUTER_BOUND ( 'NONE', #47309, .T. ) ;
#38657=CARTESIAN_POINT ( 'NONE',  ( -125.6708471809678542, -1.749999999999997113, -120.2068387089191219 ) ) ;
#38659=CYLINDRICAL_SURFACE ( 'NONE', #3560, 1.750000000000010214 ) ;
#38661=VERTEX_POINT ( 'NONE', #41820 ) ;
#38663=CYLINDRICAL_SURFACE ( 'NONE', #30123, 1.750000000000015543 ) ;
#38669=EDGE_CURVE ( 'NONE', #43847, #45334, #17909, .T. ) ;
#38674=ADVANCED_FACE ( 'NONE', ( #26931 ), #46130, .T. ) ;
#38675=DIRECTION ( 'NONE',  ( -0.000000000000000000, -0.000000000000000000, -1.000000000000000000 ) ) ;
#38677=ORIENTED_EDGE ( 'NONE', *, *, #44014, .T. ) ;
#38681=EDGE_CURVE ( 'NONE', #48612, #34716, #9094, .T. ) ;
#38685=ADVANCED_FACE ( 'NONE', ( #18207 ), #33886, .T. ) ;
#38688=DIRECTION ( 'NONE',  ( 0.000000000000000000, 0.000000000000000000, 1.000000000000000000 ) ) ;
#38693=DIRECTION ( 'NONE',  ( -1.000000000000000000, -0.000000000000000000, -0.000000000000000000 ) ) ;
#38702=DIRECTION ( 'NONE',  ( -0.000000000000000000, -0.000000000000000000, -1.000000000000000000 ) ) ;
#38703=EDGE_CURVE ( 'NONE', #2781, #50360, #7455, .T. ) ;
#38704=EDGE_LOOP ( 'NONE', ( #2712, #25131, #9500, #27756, #12995 ) ) ;
#38716=ADVANCED_FACE ( 'NONE', ( #20247 ), #12052, .T. ) ;
#38721=CARTESIAN_POINT ( 'NONE',  ( -164.9459734468149463, -1.025126265847089435, -77.43171244307200141 ) ) ;
#38724=DIRECTION ( 'NONE',  ( -1.000000000000000000, 0.000000000000000000, 0.000000000000000000 ) ) ;
#38725=DIRECTION ( 'NONE',  ( -1.000000000000000000, -0.000000000000000000, -0.000000000000000000 ) ) ;
#38726=CARTESIAN_POINT ( 'NONE',  ( -166.6959734468149463, -1.750000000000010658, 80.81828755692798438 ) ) ;
#38727=CARTESIAN_POINT ( 'NONE',  ( 33.30402655318503946, -1.750000000000010658, 120.8182875569279702 ) ) ;
#38732=ORIENTED_EDGE ( 'NONE', *, *, #42487, .F. ) ;
#38736=ADVANCED_FACE ( 'NONE', ( #4 ), #16393, .F. ) ;
#38738=FACE_OUTER_BOUND ( 'NONE', #22523, .T. ) ;
#38739=ORIENTED_EDGE ( 'NONE', *, *, #25244, .F. ) ;
#38745=LINE ( 'NONE', #35415, #19727 ) ;
#38747=ADVANCED_FACE ( 'NONE', ( #511 ), #28461, .T. ) ;
#38748=ORIENTED_EDGE ( 'NONE', *, *, #46586, .F. ) ;
#38749=DIRECTION ( 'NONE',  ( -1.000000000000000000, 0.000000000000000000, 0.000000000000000000 ) ) ;
#38751=EDGE_LOOP ( 'NONE', ( #46097, #45034, #13866, #5825, #2089, #8620 ) ) ;
#38753=EDGE_CURVE ( 'NONE', #4361, #11473, #19740, .T. ) ;
#38759=CARTESIAN_POINT ( 'NONE',  ( 193.3040265531851105, 0.000000000000000000, 165.0000000000000000 ) ) ;
#38763=FACE_OUTER_BOUND ( 'NONE', #42608, .T. ) ;
#38774=EDGE_LOOP ( 'NONE', ( #3455, #39766, #10730, #82, #24974, #925 ) ) ;
#38777=CARTESIAN_POINT ( 'NONE',  ( -7.721099712662037540, 1.750000000000023981, -80.20683870891910772 ) ) ;
#38780=( BOUNDED_CURVE ( )  B_SPLINE_CURVE ( 3, ( #40410, #4744, #48050, #5247 ),
 .UNSPECIFIED., .F., .F. ) 
 B_SPLINE_CURVE_WITH_KNOTS ( ( 4, 4 ),
 ( 1.570796326794896558, 3.141592653589793116 ),
 .UNSPECIFIED. ) 
 CURVE ( )  GEOMETRIC_REPRESENTATION_ITEM ( )  RATIONAL_B_SPLINE_CURVE ( ( 1.000000000000000000, 0.8047378541243649375, 0.8047378541243649375, 1.000000000000000000 ) ) 
 REPRESENTATION_ITEM ( '' )  );
#38781=DIRECTION ( 'NONE',  ( -1.000000000000000000, -0.000000000000000000, -0.000000000000000000 ) ) ;
#38783=PRODUCT_DEFINITION ( 'UNKNOWN', '', #38952, #24211 ) ;
#38786=CARTESIAN_POINT ( 'NONE',  ( -208.4459734468149463, 0.000000000000000000, 42.56828755692798438 ) ) ;
#38787=CARTESIAN_POINT ( 'NONE',  ( 210.0000000000000568, 2.143131898507881856E-16, -80.93171244307202983 ) ) ;
#38788=LINE ( 'NONE', #10551, #41942 ) ;
#38794=ORIENTED_EDGE ( 'NONE', *, *, #28338, .F. ) ;
#38806=VECTOR ( 'NONE', #48583, 1000.000000000000000 ) ;
#38809=VECTOR ( 'NONE', #44089, 1000.000000000000000 ) ;
#38810=CARTESIAN_POINT ( 'NONE',  ( 191.5540265531850537, -1.025126265847089879, -117.4317124430720156 ) ) ;
#38815=DIRECTION ( 'NONE',  ( 1.000000000000000000, 0.000000000000000000, -0.000000000000000000 ) ) ;
#38817=EDGE_LOOP ( 'NONE', ( #3006, #14003, #9877, #9793, #15212, #13166 ) ) ;
#38822=EDGE_LOOP ( 'NONE', ( #32469, #44443, #23943, #41774, #8585, #1854 ) ) ;
#38823=EDGE_CURVE ( 'NONE', #6064, #13712, #1603, .T. ) ;
#38824=ADVANCED_FACE ( 'NONE', ( #5853 ), #48403, .T. ) ;
#38835=ORIENTED_EDGE ( 'NONE', *, *, #46926, .F. ) ;
#38838=CARTESIAN_POINT ( 'NONE',  ( 112.2789002873379758, -1.749999999999996891, -78.15658617722492352 ) ) ;
#38841=LINE ( 'NONE', #19560, #3656 ) ;
#38844=CARTESIAN_POINT ( 'NONE',  ( 33.30402655318503946, 1.750000000000010214, 40.81828755692798438 ) ) ;
#38845=ORIENTED_EDGE ( 'NONE', *, *, #26570, .T. ) ;
#38851=VECTOR ( 'NONE', #33124, 1000.000000000000000 ) ;
#38853=ORIENTED_EDGE ( 'NONE', *, *, #30351, .T. ) ;
#38862=CARTESIAN_POINT ( 'NONE',  ( -165.6708471809677974, 1.750000000000009548, 41.84341382277508359 ) ) ;
#38863=EDGE_LOOP ( 'NONE', ( #22149, #3001, #32030, #38132, #31350, #19031 ) ) ;
#38865=CARTESIAN_POINT ( 'NONE',  ( -86.69597344681494633, -1.750000000000010658, 120.8182875569279702 ) ) ;
#38868=( BOUNDED_CURVE ( )  B_SPLINE_CURVE ( 3, ( #41406, #29860, #38335, #41658 ),
 .UNSPECIFIED., .F., .F. ) 
 B_SPLINE_CURVE_WITH_KNOTS ( ( 4, 4 ),
 ( 0.000000000000000000, 1.570796326794896558 ),
 .UNSPECIFIED. ) 
 CURVE ( )  GEOMETRIC_REPRESENTATION_ITEM ( )  RATIONAL_B_SPLINE_CURVE ( ( 1.000000000000000000, 0.8047378541243649375, 0.8047378541243649375, 1.000000000000000000 ) ) 
 REPRESENTATION_ITEM ( '' )  );
#38871=ORIENTED_EDGE ( 'NONE', *, *, #1385, .F. ) ;
#38876=EDGE_CURVE ( 'NONE', #16166, #38061, #33673, .T. ) ;
#38882=VERTEX_POINT ( 'NONE', #6103 ) ;
#38884=CARTESIAN_POINT ( 'NONE',  ( -164.9459734468149463, 1.025126265847089213, -0.9317124430720324924 ) ) ;
#38887=ADVANCED_FACE ( 'NONE', ( #28705 ), #17402, .T. ) ;
#38889=CARTESIAN_POINT ( 'NONE',  ( -164.9459734468149463, 2.143131898507880377E-16, 42.56828755692798438 ) ) ;
#38890=CARTESIAN_POINT ( 'NONE',  ( -126.6959734468149321, -1.749999999999997335, 120.8182875569279702 ) ) ;
#38891=EDGE_CURVE ( 'NONE', #25713, #36323, #19568, .T. ) ;
#38893=VERTEX_POINT ( 'NONE', #44563 ) ;
#38895=ORIENTED_EDGE ( 'NONE', *, *, #47586, .T. ) ;
#38896=CARTESIAN_POINT ( 'NONE',  ( -208.4459734468149463, 0.000000000000000000, 82.56828755692798438 ) ) ;
#38907=CARTESIAN_POINT ( 'NONE',  ( 191.5540265531850537, -1.025126265847089657, -37.43171244307202272 ) ) ;
#38912=CARTESIAN_POINT ( 'NONE',  ( 210.0000000000000568, 0.000000000000000000, 2.568287556927987048 ) ) ;
#38915=DIRECTION ( 'NONE',  ( -1.000000000000000000, 0.000000000000000000, 0.000000000000000000 ) ) ;
#38924=CARTESIAN_POINT ( 'NONE',  ( -164.9459734468149463, 2.143131898507880377E-16, -80.93171244307201562 ) ) ;
#38925=ORIENTED_EDGE ( 'NONE', *, *, #25798, .F. ) ;
#38926=( BOUNDED_CURVE ( )  B_SPLINE_CURVE ( 3, ( #16277, #47538, #12418, #28076 ),
 .UNSPECIFIED., .F., .F. ) 
 B_SPLINE_CURVE_WITH_KNOTS ( ( 4, 4 ),
 ( 4.712388980384689674, 6.283185307179586232 ),
 .UNSPECIFIED. ) 
 CURVE ( )  GEOMETRIC_REPRESENTATION_ITEM ( )  RATIONAL_B_SPLINE_CURVE ( ( 1.000000000000000000, 0.8047378541243649375, 0.8047378541243649375, 1.000000000000000000 ) ) 
 REPRESENTATION_ITEM ( '' )  );
#38927=FACE_OUTER_BOUND ( 'NONE', #36476, .T. ) ;
#38928=DIRECTION ( 'NONE',  ( -0.000000000000000000, -0.000000000000000000, -1.000000000000000000 ) ) ;
#38930=CARTESIAN_POINT ( 'NONE',  ( -166.6959734468149463, -1.750000000000010658, 80.81828755692798438 ) ) ;
#38933=( BOUNDED_CURVE ( )  B_SPLINE_CURVE ( 3, ( #45380, #10268, #25926, #22056 ),
 .UNSPECIFIED., .F., .F. ) 
 B_SPLINE_CURVE_WITH_KNOTS ( ( 4, 4 ),
 ( 1.570796326794896558, 3.141592653589793116 ),
 .UNSPECIFIED. ) 
 CURVE ( )  GEOMETRIC_REPRESENTATION_ITEM ( )  RATIONAL_B_SPLINE_CURVE ( ( 1.000000000000000000, 0.8047378541243649375, 0.8047378541243649375, 1.000000000000000000 ) ) 
 REPRESENTATION_ITEM ( '' )  );
#38934=FACE_OUTER_BOUND ( 'NONE', #46202, .T. ) ;
#38935=CARTESIAN_POINT ( 'NONE',  ( 210.0000000000000568, 0.000000000000000000, -39.18171244307202983 ) ) ;
#38936=DIRECTION ( 'NONE',  ( 0.000000000000000000, 0.000000000000000000, 1.000000000000000000 ) ) ;
#38938=AXIS2_PLACEMENT_3D ( 'NONE', #24666, #17217, #20799 ) ;
#38939=VERTEX_POINT ( 'NONE', #6865 ) ;
#38948=EDGE_CURVE ( 'NONE', #39145, #47361, #34319, .T. ) ;
#38951=EDGE_LOOP ( 'NONE', ( #45234, #23564, #4625, #35758, #687, #3845 ) ) ;
#38952=PRODUCT_DEFINITION_FORMATION_WITH_SPECIFIED_SOURCE ( 'ANY', '', #9324, .NOT_KNOWN. ) ;
#38956=AXIS2_PLACEMENT_3D ( 'NONE', #45992, #22680, #26792 ) ;
#38962=ORIENTED_EDGE ( 'NONE', *, *, #20171, .F. ) ;
#38966=EDGE_LOOP ( 'NONE', ( #3223, #5230, #15901, #40218, #47115, #6459 ) ) ;
#38981=FACE_OUTER_BOUND ( 'NONE', #6920, .T. ) ;
#38987=DIRECTION ( 'NONE',  ( -0.000000000000000000, -0.000000000000000000, -1.000000000000000000 ) ) ;
#38988=CARTESIAN_POINT ( 'NONE',  ( 32.27890028733795447, -1.750000000000009548, -160.2068387089191219 ) ) ;
#38989=CARTESIAN_POINT ( 'NONE',  ( -126.6959734468149321, -1.749999999999997113, 40.81828755692798438 ) ) ;
#38994=CARTESIAN_POINT ( 'NONE',  ( -8.445973446814976526, 0.000000000000000000, -37.43171244307200141 ) ) ;
#38995=DIRECTION ( 'NONE',  ( -1.000000000000000000, -0.000000000000000000, -0.000000000000000000 ) ) ;
#38997=VERTEX_POINT ( 'NONE', #37935 ) ;
#38999=CARTESIAN_POINT ( 'NONE',  ( 113.3040265531850537, -1.749999999999996891, -159.1817124430720298 ) ) ;
#39001=CARTESIAN_POINT ( 'NONE',  ( -44.94597344681493922, 2.143131898507880377E-16, -77.43171244307198720 ) ) ;
#39002=ORIENTED_EDGE ( 'NONE', *, *, #31490, .T. ) ;
#39004=DIRECTION ( 'NONE',  ( -0.000000000000000000, -0.000000000000000000, -1.000000000000000000 ) ) ;
#39016=ADVANCED_FACE ( 'NONE', ( #2508 ), #23007, .T. ) ;
#39017=ADVANCED_FACE ( 'NONE', ( #10705 ), #42011, .T. ) ;
#39019=EDGE_LOOP ( 'NONE', ( #4836, #22720, #6949, #28502, #38266, #21852 ) ) ;
#39020=CARTESIAN_POINT ( 'NONE',  ( 71.55402655318505367, 0.000000000000000000, 79.06828755692797017 ) ) ;
#39024=CYLINDRICAL_SURFACE ( 'NONE', #19657, 1.750000000000001554 ) ;
#39025=CARTESIAN_POINT ( 'NONE',  ( 112.2789002873379758, 1.749999999999996669, -0.2068387089191042749 ) ) ;
#39027=ORIENTED_EDGE ( 'NONE', *, *, #28731, .F. ) ;
#39035=CARTESIAN_POINT ( 'NONE',  ( 210.0000000000000568, 2.143131898507881116E-16, 39.06828755692797728 ) ) ;
#39037=EDGE_CURVE ( 'NONE', #20525, #24506, #15677, .T. ) ;
#39042=CARTESIAN_POINT ( 'NONE',  ( -210.0000000000000568, 0.000000000000000000, -39.18171244307202983 ) ) ;
#39044=ADVANCED_FACE ( 'NONE', ( #42264 ), #22762, .T. ) ;
#39047=VECTOR ( 'NONE', #39279, 1000.000000000000000 ) ;
#39050=EDGE_CURVE ( 'NONE', #7869, #43947, #11988, .T. ) ;
#39051=CARTESIAN_POINT ( 'NONE',  ( 111.5540265531850537, -1.025126265847081664, 2.568287556927973281 ) ) ;
#39055=VERTEX_POINT ( 'NONE', #192 ) ;
#39059=CARTESIAN_POINT ( 'NONE',  ( -124.9459734468149321, -1.025126265847081886, -40.93171244307202272 ) ) ;
#39061=CARTESIAN_POINT ( 'NONE',  ( -205.6708471809678827, -1.750000000000009326, -158.1565861772249377 ) ) ;
#39062=VECTOR ( 'NONE', #39494, 1000.000000000000000 ) ;
#39063=DIRECTION ( 'NONE',  ( -1.000000000000000000, -0.000000000000000000, -0.000000000000000000 ) ) ;
#39064=ORIENTED_EDGE ( 'NONE', *, *, #11750, .F. ) ;
#39069=VECTOR ( 'NONE', #44163, 1000.000000000000000 ) ;
#39070=( BOUNDED_CURVE ( )  B_SPLINE_CURVE ( 3, ( #4952, #32423, #48017, #12902 ),
 .UNSPECIFIED., .F., .F. ) 
 B_SPLINE_CURVE_WITH_KNOTS ( ( 4, 4 ),
 ( 1.570796326794896558, 3.141592653589793116 ),
 .UNSPECIFIED. ) 
 CURVE ( )  GEOMETRIC_REPRESENTATION_ITEM ( )  RATIONAL_B_SPLINE_CURVE ( ( 1.000000000000000000, 0.8047378541243649375, 0.8047378541243649375, 1.000000000000000000 ) ) 
 REPRESENTATION_ITEM ( '' )  );
#39084=EDGE_CURVE ( 'NONE', #21262, #40406, #5187, .T. ) ;
#39088=CARTESIAN_POINT ( 'NONE',  ( 113.3040265531850537, 1.749999999999997335, -119.1817124430720440 ) ) ;
#39090=LINE ( 'NONE', #4424, #31172 ) ;
#39092=( BOUNDED_CURVE ( )  B_SPLINE_CURVE ( 3, ( #23485, #26316, #22456, #6807 ),
 .UNSPECIFIED., .F., .F. ) 
 B_SPLINE_CURVE_WITH_KNOTS ( ( 4, 4 ),
 ( 4.712388980384689674, 6.283185307179586232 ),
 .UNSPECIFIED. ) 
 CURVE ( )  GEOMETRIC_REPRESENTATION_ITEM ( )  RATIONAL_B_SPLINE_CURVE ( ( 1.000000000000000000, 0.8047378541243649375, 0.8047378541243649375, 1.000000000000000000 ) ) 
 REPRESENTATION_ITEM ( '' )  );
#39094=ORIENTED_EDGE ( 'NONE', *, *, #33487, .F. ) ;
#39098=CARTESIAN_POINT ( 'NONE',  ( 195.0540265531851105, 2.143131898507880377E-16, -120.9317124430720156 ) ) ;
#39105=VECTOR ( 'NONE', #11751, 1000.000000000000000 ) ;
#39108=EDGE_CURVE ( 'NONE', #41145, #19783, #39699, .T. ) ;
#39114=CYLINDRICAL_SURFACE ( 'NONE', #8497, 1.750000000000001554 ) ;
#39117=CARTESIAN_POINT ( 'NONE',  ( 33.30402655318503946, 1.750000000000010658, 120.8182875569279702 ) ) ;
#39119=EDGE_CURVE ( 'NONE', #34716, #23271, #24831, .T. ) ;
#39123=CARTESIAN_POINT ( 'NONE',  ( 210.0000000000000568, 2.143131898507881856E-16, -80.93171244307202983 ) ) ;
#39125=CARTESIAN_POINT ( 'NONE',  ( 193.3040265531851105, 1.750000000000010658, -79.18171244307201562 ) ) ;
#39129=ORIENTED_EDGE ( 'NONE', *, *, #41420, .T. ) ;
#39131=EDGE_CURVE ( 'NONE', #5910, #15638, #30078, .T. ) ;
#39133=CARTESIAN_POINT ( 'NONE',  ( 115.0540265531850395, 2.143131898507847836E-16, 42.56828755692795596 ) ) ;
#39134=CARTESIAN_POINT ( 'NONE',  ( -46.69597344681494633, -1.750000000000010658, 80.81828755692798438 ) ) ;
#39135=EDGE_CURVE ( 'NONE', #25919, #43433, #35346, .T. ) ;
#39140=VERTEX_POINT ( 'NONE', #48596 ) ;
#39142=CARTESIAN_POINT ( 'NONE',  ( -167.7210997126620384, 1.750000000000009548, 39.79316129108089228 ) ) ;
#39145=VERTEX_POINT ( 'NONE', #40704 ) ;
#39146=CARTESIAN_POINT ( 'NONE',  ( 193.3040265531851105, -1.750000000000010658, -79.18171244307201562 ) ) ;
#39148=AXIS2_PLACEMENT_3D ( 'NONE', #6341, #21986, #37660 ) ;
#39150=ORIENTED_EDGE ( 'NONE', *, *, #17136, .F. ) ;
#39157=ORIENTED_EDGE ( 'NONE', *, *, #32148, .T. ) ;
#39158=CARTESIAN_POINT ( 'NONE',  ( -8.445973446814976526, 0.000000000000000000, 122.5682875569279986 ) ) ;
#39163=EDGE_CURVE ( 'NONE', #39985, #26096, #28128, .T. ) ;
#39165=FACE_OUTER_BOUND ( 'NONE', #40541, .T. ) ;
#39167=( BOUNDED_CURVE ( )  B_SPLINE_CURVE ( 3, ( #41717, #18352, #10662, #26325 ),
 .UNSPECIFIED., .F., .F. ) 
 B_SPLINE_CURVE_WITH_KNOTS ( ( 4, 4 ),
 ( 1.570796326794896558, 3.141592653589793116 ),
 .UNSPECIFIED. ) 
 CURVE ( )  GEOMETRIC_REPRESENTATION_ITEM ( )  RATIONAL_B_SPLINE_CURVE ( ( 1.000000000000000000, 0.8047378541243649375, 0.8047378541243649375, 1.000000000000000000 ) ) 
 REPRESENTATION_ITEM ( '' )  );
#39179=ADVANCED_FACE ( 'NONE', ( #25053 ), #1951, .T. ) ;
#39186=CARTESIAN_POINT ( 'NONE',  ( 210.0000000000000568, 2.143131898507880377E-16, 159.0682875569279702 ) ) ;
#39189=CARTESIAN_POINT ( 'NONE',  ( 35.05402655318504657, 2.143131898507880377E-16, 165.0000000000000000 ) ) ;
#39195=ORIENTED_EDGE ( 'NONE', *, *, #22425, .T. ) ;
#39196=CARTESIAN_POINT ( 'NONE',  ( -48.44597344681495343, 0.000000000000000000, 122.5682875569279702 ) ) ;
#39198=ORIENTED_EDGE ( 'NONE', *, *, #14215, .F. ) ;
#39201=CARTESIAN_POINT ( 'NONE',  ( -44.94597344681493922, 1.025126265847089879, 122.5682875569280128 ) ) ;
#39203=DIRECTION ( 'NONE',  ( -1.000000000000000000, -0.000000000000000000, -0.000000000000000000 ) ) ;
#39209=FACE_OUTER_BOUND ( 'NONE', #44162, .T. ) ;
#39211=DIRECTION ( 'NONE',  ( -1.000000000000000000, 0.000000000000000000, 0.000000000000000000 ) ) ;
#39212=FACE_OUTER_BOUND ( 'NONE', #33179, .T. ) ;
#39218=( BOUNDED_CURVE ( )  B_SPLINE_CURVE ( 3, ( #2331, #45148, #2093, #10036 ),
 .UNSPECIFIED., .F., .F. ) 
 B_SPLINE_CURVE_WITH_KNOTS ( ( 4, 4 ),
 ( 1.570796326794896558, 3.141592653589793116 ),
 .UNSPECIFIED. ) 
 CURVE ( )  GEOMETRIC_REPRESENTATION_ITEM ( )  RATIONAL_B_SPLINE_CURVE ( ( 1.000000000000000000, 0.8047378541243649375, 0.8047378541243649375, 1.000000000000000000 ) ) 
 REPRESENTATION_ITEM ( '' )  );
#39219=ORIENTED_EDGE ( 'NONE', *, *, #30680, .F. ) ;
#39227=( BOUNDED_CURVE ( )  B_SPLINE_CURVE ( 3, ( #42708, #11944, #47041, #27602 ),
 .UNSPECIFIED., .F., .F. ) 
 B_SPLINE_CURVE_WITH_KNOTS ( ( 4, 4 ),
 ( 4.712388980384689674, 6.283185307179586232 ),
 .UNSPECIFIED. ) 
 CURVE ( )  GEOMETRIC_REPRESENTATION_ITEM ( )  RATIONAL_B_SPLINE_CURVE ( ( 1.000000000000000000, 0.8047378541243649375, 0.8047378541243649375, 1.000000000000000000 ) ) 
 REPRESENTATION_ITEM ( '' )  );
#39229=ORIENTED_EDGE ( 'NONE', *, *, #14890, .T. ) ;
#39231=CARTESIAN_POINT ( 'NONE',  ( 32.27890028733795447, -1.750000000000009548, 161.8434138227750907 ) ) ;
#39232=CYLINDRICAL_SURFACE ( 'NONE', #13125, 1.749999999999987566 ) ;
#39235=FACE_OUTER_BOUND ( 'NONE', #21279, .T. ) ;
#39236=CARTESIAN_POINT ( 'NONE',  ( 71.55402655318505367, 0.000000000000000000, 82.56828755692799859 ) ) ;
#39242=CYLINDRICAL_SURFACE ( 'NONE', #28935, 1.750000000000001554 ) ;
#39248=CYLINDRICAL_SURFACE ( 'NONE', #42526, 1.750000000000036193 ) ;
#39249=CARTESIAN_POINT ( 'NONE',  ( 114.3291528190321173, -1.749999999999996225, 159.7931612910809065 ) ) ;
#39252=VECTOR ( 'NONE', #2432, 1000.000000000000000 ) ;
#39255=AXIS2_PLACEMENT_3D ( 'NONE', #49473, #46126, #30034 ) ;
#39264=DIRECTION ( 'NONE',  ( -0.000000000000000000, -0.000000000000000000, -1.000000000000000000 ) ) ;
#39265=CIRCLE ( 'NONE', #14666, 1.750000000000036193 ) ;
#39266=EDGE_LOOP ( 'NONE', ( #41106, #37946, #46854, #32164, #18161, #15281 ) ) ;
#39272=ORIENTED_EDGE ( 'NONE', *, *, #34383, .F. ) ;
#39275=ORIENTED_EDGE ( 'NONE', *, *, #18348, .F. ) ;
#39278=ORIENTED_EDGE ( 'NONE', *, *, #21484, .T. ) ;
#39279=DIRECTION ( 'NONE',  ( -1.000000000000000000, -0.000000000000000000, -0.000000000000000000 ) ) ;
#39280=CARTESIAN_POINT ( 'NONE',  ( 153.3040265531850537, -1.750000000000010214, 40.81828755692798438 ) ) ;
#39283=DIRECTION ( 'NONE',  ( -0.000000000000000000, -0.000000000000000000, -1.000000000000000000 ) ) ;
#39291=ORIENTED_EDGE ( 'NONE', *, *, #2358, .F. ) ;
#39293=AXIS2_PLACEMENT_3D ( 'NONE', #43298, #47112, #47364 ) ;
#39296=LINE ( 'NONE', #19779, #35479 ) ;
#39301=CARTESIAN_POINT ( 'NONE',  ( 31.55402655318503236, 1.025126265847089657, -120.9317124430720440 ) ) ;
#39304=DIRECTION ( 'NONE',  ( -0.000000000000000000, -0.000000000000000000, -1.000000000000000000 ) ) ;
#39312=CARTESIAN_POINT ( 'NONE',  ( 210.0000000000000568, 0.000000000000000000, 0.8182875569279768335 ) ) ;
#39316=CARTESIAN_POINT ( 'NONE',  ( 114.3291528190321173, 1.749999999999996891, -120.2068387089191219 ) ) ;
#39318=FACE_OUTER_BOUND ( 'NONE', #18361, .T. ) ;
#39322=EDGE_CURVE ( 'NONE', #47604, #24955, #40562, .T. ) ;
#39324=EDGE_CURVE ( 'NONE', #41657, #13983, #10723, .T. ) ;
#39330=AXIS2_PLACEMENT_3D ( 'NONE', #42383, #30602, #45957 ) ;
#39339=EDGE_CURVE ( 'NONE', #15022, #24864, #24532, .T. ) ;
#39340=ORIENTED_EDGE ( 'NONE', *, *, #1295, .T. ) ;
#39345=CARTESIAN_POINT ( 'NONE',  ( 193.3040265531851105, 1.750000000000010658, -119.1817124430720440 ) ) ;
#39348=ORIENTED_EDGE ( 'NONE', *, *, #38753, .T. ) ;
#39350=ORIENTED_EDGE ( 'NONE', *, *, #2083, .T. ) ;
#39352=EDGE_CURVE ( 'NONE', #18302, #35538, #28013, .T. ) ;
#39355=ADVANCED_FACE ( 'NONE', ( #43647 ), #44150, .T. ) ;
#39356=ORIENTED_EDGE ( 'NONE', *, *, #23018, .F. ) ;
#39357=EDGE_CURVE ( 'NONE', #20835, #25904, #21223, .T. ) ;
#39364=CARTESIAN_POINT ( 'NONE',  ( -44.94597344681493922, 2.143131898507880377E-16, -80.93171244307204404 ) ) ;
#39366=ORIENTED_EDGE ( 'NONE', *, *, #42053, .T. ) ;
#39367=EDGE_CURVE ( 'NONE', #37516, #15344, #48593, .T. ) ;
#39370=VERTEX_POINT ( 'NONE', #40078 ) ;
#39372=( BOUNDED_CURVE ( )  B_SPLINE_CURVE ( 3, ( #24585, #27675, #31792, #43569 ),
 .UNSPECIFIED., .F., .F. ) 
 B_SPLINE_CURVE_WITH_KNOTS ( ( 4, 4 ),
 ( 3.141592653589793116, 4.712388980384689674 ),
 .UNSPECIFIED. ) 
 CURVE ( )  GEOMETRIC_REPRESENTATION_ITEM ( )  RATIONAL_B_SPLINE_CURVE ( ( 1.000000000000000000, 0.8047378541243649375, 0.8047378541243649375, 1.000000000000000000 ) ) 
 REPRESENTATION_ITEM ( '' )  );
#39373=CARTESIAN_POINT ( 'NONE',  ( 33.30402655318503946, 0.000000000000000000, 165.0000000000000000 ) ) ;
#39377=DIRECTION ( 'NONE',  ( -0.000000000000000000, -0.000000000000000000, -1.000000000000000000 ) ) ;
#39380=ORIENTED_EDGE ( 'NONE', *, *, #8363, .F. ) ;
#39383=( BOUNDED_CURVE ( )  B_SPLINE_CURVE ( 3, ( #16454, #24661, #22942, #3698 ),
 .UNSPECIFIED., .F., .F. ) 
 B_SPLINE_CURVE_WITH_KNOTS ( ( 4, 4 ),
 ( 0.000000000000000000, 1.570796326794896558 ),
 .UNSPECIFIED. ) 
 CURVE ( )  GEOMETRIC_REPRESENTATION_ITEM ( )  RATIONAL_B_SPLINE_CURVE ( ( 1.000000000000000000, 0.8047378541243649375, 0.8047378541243649375, 1.000000000000000000 ) ) 
 REPRESENTATION_ITEM ( '' )  );
#39385=CARTESIAN_POINT ( 'NONE',  ( 71.55402655318505367, -1.025126265847089879, -117.4317124430720156 ) ) ;
#39386=CYLINDRICAL_SURFACE ( 'NONE', #25773, 1.750000000000008438 ) ;
#39392=( BOUNDED_CURVE ( )  B_SPLINE_CURVE ( 3, ( #7604, #50649, #4001, #19651 ),
 .UNSPECIFIED., .F., .F. ) 
 B_SPLINE_CURVE_WITH_KNOTS ( ( 4, 4 ),
 ( 0.000000000000000000, 1.570796326794896780 ),
 .UNSPECIFIED. ) 
 CURVE ( )  GEOMETRIC_REPRESENTATION_ITEM ( )  RATIONAL_B_SPLINE_CURVE ( ( 1.000000000000000000, 0.8047378541243649375, 0.8047378541243649375, 1.000000000000000000 ) ) 
 REPRESENTATION_ITEM ( '' )  );
#39393=DIRECTION ( 'NONE',  ( -0.000000000000000000, -0.000000000000000000, -1.000000000000000000 ) ) ;
#39398=CARTESIAN_POINT ( 'NONE',  ( -168.4459734468149463, 0.000000000000000000, 39.06828755692798438 ) ) ;
#39401=EDGE_CURVE ( 'NONE', #41447, #1049, #26466, .T. ) ;
#39403=ORIENTED_EDGE ( 'NONE', *, *, #15864, .F. ) ;
#39410=DIRECTION ( 'NONE',  ( -1.000000000000000000, 0.000000000000000000, 0.000000000000000000 ) ) ;
#39411=CARTESIAN_POINT ( 'NONE',  ( -206.6959734468149463, 1.750000000000009992, 0.8182875569279768335 ) ) ;
#39412=ORIENTED_EDGE ( 'NONE', *, *, #11238, .T. ) ;
#39417=FACE_OUTER_BOUND ( 'NONE', #28482, .T. ) ;
#39425=CYLINDRICAL_SURFACE ( 'NONE', #14774, 1.750000000000036193 ) ;
#39427=DIRECTION ( 'NONE',  ( -1.000000000000000000, -0.000000000000000000, -0.000000000000000000 ) ) ;
#39429=ORIENTED_EDGE ( 'NONE', *, *, #8410, .F. ) ;
#39431=DIRECTION ( 'NONE',  ( -1.000000000000000000, -0.000000000000000000, -0.000000000000000000 ) ) ;
#39433=CARTESIAN_POINT ( 'NONE',  ( -6.695973446814940111, 0.000000000000000000, 165.0000000000000000 ) ) ;
#39440=DIRECTION ( 'NONE',  ( -0.000000000000000000, -0.000000000000000000, -1.000000000000000000 ) ) ;
#39442=CARTESIAN_POINT ( 'NONE',  ( -7.721099712662037540, 1.750000000000022427, 1.843413822775074040 ) ) ;
#39458=CARTESIAN_POINT ( 'NONE',  ( -124.9459734468149321, -1.025126265847081664, -37.43171244307203693 ) ) ;
#39462=EDGE_CURVE ( 'NONE', #29622, #2364, #36997, .T. ) ;
#39464=EDGE_CURVE ( 'NONE', #11195, #21418, #15990, .T. ) ;
#39465=VERTEX_POINT ( 'NONE', #36754 ) ;
#39468=( BOUNDED_CURVE ( )  B_SPLINE_CURVE ( 3, ( #14719, #42160, #22669, #16746 ),
 .UNSPECIFIED., .F., .F. ) 
 B_SPLINE_CURVE_WITH_KNOTS ( ( 4, 4 ),
 ( 4.712388980384689674, 6.283185307179586232 ),
 .UNSPECIFIED. ) 
 CURVE ( )  GEOMETRIC_REPRESENTATION_ITEM ( )  RATIONAL_B_SPLINE_CURVE ( ( 1.000000000000000000, 0.8047378541243649375, 0.8047378541243649375, 1.000000000000000000 ) ) 
 REPRESENTATION_ITEM ( '' )  );
#39469=EDGE_CURVE ( 'NONE', #37195, #32609, #42195, .T. ) ;
#39473=FACE_OUTER_BOUND ( 'NONE', #23179, .T. ) ;
#39476=ORIENTED_EDGE ( 'NONE', *, *, #22067, .T. ) ;
#39477=CARTESIAN_POINT ( 'NONE',  ( 210.0000000000000568, 0.000000000000000000, -39.18171244307202983 ) ) ;
#39489=LINE ( 'NONE', #19717, #22269 ) ;
#39494=DIRECTION ( 'NONE',  ( -0.000000000000000000, -0.000000000000000000, -1.000000000000000000 ) ) ;
#39496=DIRECTION ( 'NONE',  ( -0.000000000000000000, -0.000000000000000000, -1.000000000000000000 ) ) ;
#39498=EDGE_CURVE ( 'NONE', #20980, #19783, #1899, .T. ) ;
#39501=CARTESIAN_POINT ( 'NONE',  ( -204.9459734468148895, -1.025126265847089435, 39.06828755692797728 ) ) ;
#39509=ORIENTED_EDGE ( 'NONE', *, *, #15787, .T. ) ;
#39511=EDGE_CURVE ( 'NONE', #2812, #38442, #7142, .T. ) ;
#39513=LINE ( 'NONE', #43086, #46626 ) ;
#39514=ORIENTED_EDGE ( 'NONE', *, *, #25089, .T. ) ;
#39515=CARTESIAN_POINT ( 'NONE',  ( 193.3040265531851105, -1.750000000000009992, 0.8182875569279768335 ) ) ;
#39521=ADVANCED_FACE ( 'NONE', ( #38511 ), #34917, .T. ) ;
#39522=( BOUNDED_CURVE ( )  B_SPLINE_CURVE ( 3, ( #30768, #46379, #34881, #26904 ),
 .UNSPECIFIED., .F., .F. ) 
 B_SPLINE_CURVE_WITH_KNOTS ( ( 4, 4 ),
 ( 4.712388980384689674, 6.283185307179586232 ),
 .UNSPECIFIED. ) 
 CURVE ( )  GEOMETRIC_REPRESENTATION_ITEM ( )  RATIONAL_B_SPLINE_CURVE ( ( 1.000000000000000000, 0.8047378541243649375, 0.8047378541243649375, 1.000000000000000000 ) ) 
 REPRESENTATION_ITEM ( '' )  );
#39527=CARTESIAN_POINT ( 'NONE',  ( 31.55402655318503236, 0.000000000000000000, -117.4317124430720156 ) ) ;
#39529=EDGE_CURVE ( 'NONE', #28572, #37476, #14629, .T. ) ;
#39532=( BOUNDED_CURVE ( )  B_SPLINE_CURVE ( 3, ( #17224, #28523, #29022, #824 ),
 .UNSPECIFIED., .F., .F. ) 
 B_SPLINE_CURVE_WITH_KNOTS ( ( 4, 4 ),
 ( 4.712388980384689674, 6.283185307179586232 ),
 .UNSPECIFIED. ) 
 CURVE ( )  GEOMETRIC_REPRESENTATION_ITEM ( )  RATIONAL_B_SPLINE_CURVE ( ( 1.000000000000000000, 0.8047378541243649375, 0.8047378541243649375, 1.000000000000000000 ) ) 
 REPRESENTATION_ITEM ( '' )  );
#39533=CARTESIAN_POINT ( 'NONE',  ( -88.44597344681491791, 0.000000000000000000, 162.5682875569279702 ) ) ;
#39536=CARTESIAN_POINT ( 'NONE',  ( 151.5540265531850537, 1.025126265847089435, 82.56828755692798438 ) ) ;
#39541=VECTOR ( 'NONE', #1246, 1000.000000000000000 ) ;
#39545=CYLINDRICAL_SURFACE ( 'NONE', #2153, 1.750000000000015543 ) ;
#39562=CARTESIAN_POINT ( 'NONE',  ( 155.0540265531850537, 2.143131898507880377E-16, -160.9317124430720014 ) ) ;
#39563=EDGE_LOOP ( 'NONE', ( #37873, #31237, #30284, #49268, #19938, #38069 ) ) ;
#39566=CARTESIAN_POINT ( 'NONE',  ( -167.7210997126620384, 1.750000000000009548, -78.15658617722490931 ) ) ;
#39570=ORIENTED_EDGE ( 'NONE', *, *, #23345, .T. ) ;
#39574=CARTESIAN_POINT ( 'NONE',  ( -124.9459734468149463, 2.143131898507847836E-16, -0.9317124430719969652 ) ) ;
#39577=CARTESIAN_POINT ( 'NONE',  ( 75.05402655318509630, -1.025126265847089213, 42.56828755692799149 ) ) ;
#39578=CARTESIAN_POINT ( 'NONE',  ( 210.0000000000000568, 0.000000000000000000, -79.18171244307201562 ) ) ;
#39580=AXIS2_PLACEMENT_3D ( 'NONE', #43329, #4097, #12540 ) ;
#39584=ORIENTED_EDGE ( 'NONE', *, *, #7076, .F. ) ;
#39587=DIRECTION ( 'NONE',  ( -1.000000000000000000, -0.000000000000000000, -0.000000000000000000 ) ) ;
#39590=EDGE_LOOP ( 'NONE', ( #25196, #3305, #25083, #15151, #26327, #46485 ) ) ;
#39592=DIRECTION ( 'NONE',  ( 1.000000000000000000, 0.000000000000000000, 0.000000000000000000 ) ) ;
#39594=CARTESIAN_POINT ( 'NONE',  ( 153.3040265531850537, -1.750000000000010658, 80.81828755692798438 ) ) ;
#39595=CARTESIAN_POINT ( 'NONE',  ( 210.0000000000000568, 0.000000000000000000, 82.56828755692799859 ) ) ;
#39608=CARTESIAN_POINT ( 'NONE',  ( 114.3291528190321173, -1.749999999999996669, -118.1565861772249661 ) ) ;
#39625=FACE_OUTER_BOUND ( 'NONE', #42850, .T. ) ;
#39627=DIRECTION ( 'NONE',  ( -0.000000000000000000, -0.000000000000000000, -1.000000000000000000 ) ) ;
#39632=CARTESIAN_POINT ( 'NONE',  ( -168.4459734468149747, 1.025126265847089657, 119.0682875569279560 ) ) ;
#39634=EDGE_CURVE ( 'NONE', #1914, #26837, #46905, .T. ) ;
#39635=ADVANCED_FACE ( 'NONE', ( #18476 ), #38265, .T. ) ;
#39643=ORIENTED_EDGE ( 'NONE', *, *, #35566, .T. ) ;
#39645=AXIS2_PLACEMENT_3D ( 'NONE', #38759, #45895, #3844 ) ;
#39646=EDGE_CURVE ( 'NONE', #48914, #39055, #26694, .T. ) ;
#39649=EDGE_CURVE ( 'NONE', #7223, #13192, #16922, .T. ) ;
#39652=CARTESIAN_POINT ( 'NONE',  ( 195.0540265531851105, 2.143131898507880377E-16, -117.4317124430720725 ) ) ;
#39656=CARTESIAN_POINT ( 'NONE',  ( -126.6959734468149321, 1.749999999999996891, -159.1817124430720298 ) ) ;
#39657=ORIENTED_EDGE ( 'NONE', *, *, #21247, .T. ) ;
#39661=( BOUNDED_CURVE ( )  B_SPLINE_CURVE ( 3, ( #34792, #11670, #7836, #27323 ),
 .UNSPECIFIED., .F., .F. ) 
 B_SPLINE_CURVE_WITH_KNOTS ( ( 4, 4 ),
 ( 4.712388980384689674, 6.283185307179586232 ),
 .UNSPECIFIED. ) 
 CURVE ( )  GEOMETRIC_REPRESENTATION_ITEM ( )  RATIONAL_B_SPLINE_CURVE ( ( 1.000000000000000000, 0.8047378541243649375, 0.8047378541243649375, 1.000000000000000000 ) ) 
 REPRESENTATION_ITEM ( '' )  );
#39662=ORIENTED_EDGE ( 'NONE', *, *, #20610, .F. ) ;
#39663=DIRECTION ( 'NONE',  ( -1.000000000000000000, 0.000000000000000000, 0.000000000000000000 ) ) ;
#39665=ORIENTED_EDGE ( 'NONE', *, *, #30598, .F. ) ;
#39667=( BOUNDED_CURVE ( )  B_SPLINE_CURVE ( 3, ( #9813, #10571, #25476, #38046 ),
 .UNSPECIFIED., .F., .F. ) 
 B_SPLINE_CURVE_WITH_KNOTS ( ( 4, 4 ),
 ( 0.000000000000000000, 1.570796326794896558 ),
 .UNSPECIFIED. ) 
 CURVE ( )  GEOMETRIC_REPRESENTATION_ITEM ( )  RATIONAL_B_SPLINE_CURVE ( ( 1.000000000000000000, 0.8047378541243649375, 0.8047378541243649375, 1.000000000000000000 ) ) 
 REPRESENTATION_ITEM ( '' )  );
#39669=CARTESIAN_POINT ( 'NONE',  ( 193.3040265531851105, 1.750000000000010658, -119.1817124430720440 ) ) ;
#39672=EDGE_CURVE ( 'NONE', #6245, #46611, #17625, .T. ) ;
#39673=ORIENTED_EDGE ( 'NONE', *, *, #48073, .F. ) ;
#39674=CARTESIAN_POINT ( 'NONE',  ( 210.0000000000000568, 0.000000000000000000, 122.5682875569279844 ) ) ;
#39686=AXIS2_PLACEMENT_3D ( 'NONE', #13362, #1581, #41077 ) ;
#39689=DIRECTION ( 'NONE',  ( -1.000000000000000000, -0.000000000000000000, -0.000000000000000000 ) ) ;
#39690=( BOUNDED_CURVE ( )  B_SPLINE_CURVE ( 3, ( #46166, #45416, #34178, #15165 ),
 .UNSPECIFIED., .F., .F. ) 
 B_SPLINE_CURVE_WITH_KNOTS ( ( 4, 4 ),
 ( 3.141592653589793116, 4.712388980384689674 ),
 .UNSPECIFIED. ) 
 CURVE ( )  GEOMETRIC_REPRESENTATION_ITEM ( )  RATIONAL_B_SPLINE_CURVE ( ( 1.000000000000000000, 0.8047378541243649375, 0.8047378541243649375, 1.000000000000000000 ) ) 
 REPRESENTATION_ITEM ( '' )  );
#39696=EDGE_CURVE ( 'NONE', #33331, #47564, #23598, .T. ) ;
#39699=LINE ( 'NONE', #31242, #18264 ) ;
#39700=AXIS2_PLACEMENT_3D ( 'NONE', #7166, #29312, #2119 ) ;
#39703=CARTESIAN_POINT ( 'NONE',  ( -88.44597344681497475, 0.000000000000000000, -0.9317124430720524764 ) ) ;
#39704=ORIENTED_EDGE ( 'NONE', *, *, #43987, .T. ) ;
#39708=VERTEX_POINT ( 'NONE', #39771 ) ;
#39709=DIRECTION ( 'NONE',  ( -1.000000000000000000, 0.000000000000000000, 0.000000000000000000 ) ) ;
#39711=ORIENTED_EDGE ( 'NONE', *, *, #3045, .F. ) ;
#39714=EDGE_LOOP ( 'NONE', ( #9229, #28145, #30555, #3324, #44759, #14983 ) ) ;
#39717=VECTOR ( 'NONE', #35497, 1000.000000000000000 ) ;
#39720=ADVANCED_FACE ( 'NONE', ( #4615 ), #16401, .T. ) ;
#39721=CYLINDRICAL_SURFACE ( 'NONE', #11221, 1.750000000000015543 ) ;
#39722=ORIENTED_EDGE ( 'NONE', *, *, #19614, .T. ) ;
#39727=VERTEX_POINT ( 'NONE', #36949 ) ;
#39731=EDGE_CURVE ( 'NONE', #43884, #14506, #49168, .T. ) ;
#39733=ORIENTED_EDGE ( 'NONE', *, *, #8467, .F. ) ;
#39735=ORIENTED_EDGE ( 'NONE', *, *, #31867, .T. ) ;
#39736=CARTESIAN_POINT ( 'NONE',  ( -86.69597344681494633, -1.750000000000010658, -119.1817124430720440 ) ) ;
#39739=EDGE_CURVE ( 'NONE', #34855, #8918, #22866, .T. ) ;
#39741=CARTESIAN_POINT ( 'NONE',  ( -44.94597344681493922, 1.025126265847089657, 42.56828755692799149 ) ) ;
#39744=VECTOR ( 'NONE', #38312, 1000.000000000000000 ) ;
#39746=CARTESIAN_POINT ( 'NONE',  ( 191.5540265531850537, 1.025126265847089213, -37.43171244307202272 ) ) ;
#39752=LINE ( 'NONE', #35906, #10737 ) ;
#39755=VERTEX_POINT ( 'NONE', #2020 ) ;
#39757=ADVANCED_FACE ( 'NONE', ( #2260 ), #18157, .T. ) ;
#39759=CARTESIAN_POINT ( 'NONE',  ( -168.4459734468149463, 0.000000000000000000, 2.568287556927978166 ) ) ;
#39764=DIRECTION ( 'NONE',  ( -0.000000000000000000, -0.000000000000000000, -1.000000000000000000 ) ) ;
#39765=( BOUNDED_CURVE ( )  B_SPLINE_CURVE ( 3, ( #4944, #31919, #27805, #1114 ),
 .UNSPECIFIED., .F., .F. ) 
 B_SPLINE_CURVE_WITH_KNOTS ( ( 4, 4 ),
 ( 0.000000000000000000, 1.570796326794896780 ),
 .UNSPECIFIED. ) 
 CURVE ( )  GEOMETRIC_REPRESENTATION_ITEM ( )  RATIONAL_B_SPLINE_CURVE ( ( 1.000000000000000000, 0.8047378541243649375, 0.8047378541243649375, 1.000000000000000000 ) ) 
 REPRESENTATION_ITEM ( '' )  );
#39766=ORIENTED_EDGE ( 'NONE', *, *, #24322, .T. ) ;
#39771=CARTESIAN_POINT ( 'NONE',  ( 71.55402655318505367, 0.000000000000000000, -120.9317124430720725 ) ) ;
#39772=ORIENTED_EDGE ( 'NONE', *, *, #25580, .F. ) ;
#39774=CARTESIAN_POINT ( 'NONE',  ( 113.3040265531850537, 0.000000000000000000, 165.0000000000000000 ) ) ;
#39775=LINE ( 'NONE', #43853, #48588 ) ;
#39778=CARTESIAN_POINT ( 'NONE',  ( 210.0000000000000568, 0.000000000000000000, 0.8182875569279768335 ) ) ;
#39783=ORIENTED_EDGE ( 'NONE', *, *, #36282, .F. ) ;
#39785=CARTESIAN_POINT ( 'NONE',  ( 210.0000000000000568, 2.143131898507880377E-16, -160.9317124430720298 ) ) ;
#39788=DIRECTION ( 'NONE',  ( 0.000000000000000000, 0.000000000000000000, 1.000000000000000000 ) ) ;
#39790=CARTESIAN_POINT ( 'NONE',  ( 154.3291528190321458, -1.750000000000009548, 39.79316129108089228 ) ) ;
#39791=AXIS2_PLACEMENT_3D ( 'NONE', #36972, #30765, #22036 ) ;
#39792=ORIENTED_EDGE ( 'NONE', *, *, #16180, .T. ) ;
#39793=DIRECTION ( 'NONE',  ( -1.000000000000000000, 0.000000000000000000, 0.000000000000000000 ) ) ;
#39798=CARTESIAN_POINT ( 'NONE',  ( 35.05402655318504657, 2.143131898507880377E-16, 2.568287556927978166 ) ) ;
#39803=EDGE_LOOP ( 'NONE', ( #37623, #19804, #21895, #36372, #13359, #42089 ) ) ;
#39805=EDGE_CURVE ( 'NONE', #20580, #1904, #43845, .T. ) ;
#39811=EDGE_CURVE ( 'NONE', #43082, #16057, #49045, .T. ) ;
#39814=AXIS2_PLACEMENT_3D ( 'NONE', #43409, #1085, #32384 ) ;
#39818=VECTOR ( 'NONE', #15478, 1000.000000000000000 ) ;
#39823=CARTESIAN_POINT ( 'NONE',  ( -6.695973446814940111, 0.000000000000000000, 165.0000000000000000 ) ) ;
#39827=( BOUNDED_CURVE ( )  B_SPLINE_CURVE ( 3, ( #32707, #1165, #32467, #39656 ),
 .UNSPECIFIED., .F., .F. ) 
 B_SPLINE_CURVE_WITH_KNOTS ( ( 4, 4 ),
 ( 0.000000000000000000, 1.570796326794896558 ),
 .UNSPECIFIED. ) 
 CURVE ( )  GEOMETRIC_REPRESENTATION_ITEM ( )  RATIONAL_B_SPLINE_CURVE ( ( 1.000000000000000000, 0.8047378541243649375, 0.8047378541243649375, 1.000000000000000000 ) ) 
 REPRESENTATION_ITEM ( '' )  );
#39831=ORIENTED_EDGE ( 'NONE', *, *, #15792, .F. ) ;
#39837=( BOUNDED_CURVE ( )  B_SPLINE_CURVE ( 3, ( #42497, #30720, #35094, #184 ),
 .UNSPECIFIED., .F., .F. ) 
 B_SPLINE_CURVE_WITH_KNOTS ( ( 4, 4 ),
 ( 1.570796326794896558, 3.141592653589793116 ),
 .UNSPECIFIED. ) 
 CURVE ( )  GEOMETRIC_REPRESENTATION_ITEM ( )  RATIONAL_B_SPLINE_CURVE ( ( 1.000000000000000000, 0.8047378541243649375, 0.8047378541243649375, 1.000000000000000000 ) ) 
 REPRESENTATION_ITEM ( '' )  );
#39838=CARTESIAN_POINT ( 'NONE',  ( -205.6708471809678827, -1.750000000000009548, -38.15658617722494483 ) ) ;
#39839=CARTESIAN_POINT ( 'NONE',  ( -124.9459734468149321, -1.025126265847081664, -77.43171244307201562 ) ) ;
#39849=CARTESIAN_POINT ( 'NONE',  ( 33.30402655318503946, 1.750000000000010658, -119.1817124430720440 ) ) ;
#39850=EDGE_CURVE ( 'NONE', #4897, #27926, #18411, .T. ) ;
#39851=ORIENTED_EDGE ( 'NONE', *, *, #28374, .T. ) ;
#39854=EDGE_CURVE ( 'NONE', #40520, #27700, #3521, .T. ) ;
#39859=CARTESIAN_POINT ( 'NONE',  ( -86.69597344681494633, -1.750000000000010214, 40.81828755692798438 ) ) ;
#39860=CARTESIAN_POINT ( 'NONE',  ( -166.6959734468149463, 0.000000000000000000, 165.0000000000000000 ) ) ;
#39861=ORIENTED_EDGE ( 'NONE', *, *, #1512, .T. ) ;
#39866=ORIENTED_EDGE ( 'NONE', *, *, #46155, .T. ) ;
#39867=ORIENTED_EDGE ( 'NONE', *, *, #19863, .T. ) ;
#39872=CARTESIAN_POINT ( 'NONE',  ( -8.445973446814964092, -1.025126265847097651, 82.56828755692798438 ) ) ;
#39874=CARTESIAN_POINT ( 'NONE',  ( -46.69597344681494633, 0.000000000000000000, 165.0000000000000000 ) ) ;
#39881=CARTESIAN_POINT ( 'NONE',  ( -87.72109971266203843, -1.750000000000009548, -160.2068387089191219 ) ) ;
#39886=ORIENTED_EDGE ( 'NONE', *, *, #8906, .F. ) ;
#39887=ORIENTED_EDGE ( 'NONE', *, *, #34626, .T. ) ;
#39888=ADVANCED_FACE ( 'NONE', ( #23270 ), #38202, .T. ) ;
#39891=CARTESIAN_POINT ( 'NONE',  ( 31.55402655318503236, -1.025126265847089435, -40.93171244307204404 ) ) ;
#39897=CARTESIAN_POINT ( 'NONE',  ( 75.05402655318509630, 2.143131898507880377E-16, -0.9317124430720524764 ) ) ;
#39899=ORIENTED_EDGE ( 'NONE', *, *, #17666, .T. ) ;
#39901=CARTESIAN_POINT ( 'NONE',  ( 73.30402655318508209, 1.750000000000010214, 40.81828755692798438 ) ) ;
#39911=ORIENTED_EDGE ( 'NONE', *, *, #16714, .F. ) ;
#39918=ORIENTED_EDGE ( 'NONE', *, *, #38539, .T. ) ;
#39920=CARTESIAN_POINT ( 'NONE',  ( 72.27890028733797578, -1.750000000000009548, 41.84341382277508359 ) ) ;
#39922=LINE ( 'NONE', #38912, #11527 ) ;
#39925=CARTESIAN_POINT ( 'NONE',  ( -8.445973446814914354, 2.143131898507880377E-16, -160.9317124430720298 ) ) ;
#39926=CARTESIAN_POINT ( 'NONE',  ( 210.0000000000000568, 0.000000000000000000, -159.1817124430720298 ) ) ;
#39928=EDGE_LOOP ( 'NONE', ( #48866, #1464, #2789, #50169, #16675, #547 ) ) ;
#39936=DIRECTION ( 'NONE',  ( -0.000000000000000000, -0.000000000000000000, -1.000000000000000000 ) ) ;
#39937=ORIENTED_EDGE ( 'NONE', *, *, #49636, .F. ) ;
#39944=EDGE_CURVE ( 'NONE', #10841, #21654, #10470, .T. ) ;
#39946=EDGE_CURVE ( 'NONE', #43746, #7277, #45590, .T. ) ;
#39947=EDGE_CURVE ( 'NONE', #10849, #18366, #14017, .T. ) ;
#39953=FACE_OUTER_BOUND ( 'NONE', #24544, .T. ) ;
#39959=CARTESIAN_POINT ( 'NONE',  ( -164.9459734468149463, -1.025126265847089435, -117.4317124430720156 ) ) ;
#39961=EDGE_CURVE ( 'NONE', #31607, #12842, #19265, .T. ) ;
#39962=ORIENTED_EDGE ( 'NONE', *, *, #39634, .T. ) ;
#39967=ADVANCED_FACE ( 'NONE', ( #35110 ), #50685, .T. ) ;
#39968=EDGE_CURVE ( 'NONE', #13126, #9081, #29767, .T. ) ;
#39971=ORIENTED_EDGE ( 'NONE', *, *, #45272, .F. ) ;
#39972=ADVANCED_FACE ( 'NONE', ( #28406 ), #47602, .T. ) ;
#39973=( BOUNDED_CURVE ( )  B_SPLINE_CURVE ( 3, ( #37801, #48783, #6472, #14159 ),
 .UNSPECIFIED., .F., .F. ) 
 B_SPLINE_CURVE_WITH_KNOTS ( ( 4, 4 ),
 ( 0.000000000000000000, 1.570796326794896558 ),
 .UNSPECIFIED. ) 
 CURVE ( )  GEOMETRIC_REPRESENTATION_ITEM ( )  RATIONAL_B_SPLINE_CURVE ( ( 1.000000000000000000, 0.8047378541243649375, 0.8047378541243649375, 1.000000000000000000 ) ) 
 REPRESENTATION_ITEM ( '' )  );
#39974=EDGE_CURVE ( 'NONE', #50130, #24506, #35046, .T. ) ;
#39976=ORIENTED_EDGE ( 'NONE', *, *, #1093, .F. ) ;
#39978=CARTESIAN_POINT ( 'NONE',  ( -8.445973446814976526, 0.000000000000000000, -157.4317124430720014 ) ) ;
#39980=VERTEX_POINT ( 'NONE', #35866 ) ;
#39981=CARTESIAN_POINT ( 'NONE',  ( 210.0000000000000568, 0.000000000000000000, 40.81828755692798438 ) ) ;
#39985=VERTEX_POINT ( 'NONE', #20190 ) ;
#39987=( BOUNDED_CURVE ( )  B_SPLINE_CURVE ( 3, ( #47954, #36473, #1313, #16960 ),
 .UNSPECIFIED., .F., .F. ) 
 B_SPLINE_CURVE_WITH_KNOTS ( ( 4, 4 ),
 ( 3.141592653589793116, 4.712388980384689674 ),
 .UNSPECIFIED. ) 
 CURVE ( )  GEOMETRIC_REPRESENTATION_ITEM ( )  RATIONAL_B_SPLINE_CURVE ( ( 1.000000000000000000, 0.8047378541243649375, 0.8047378541243649375, 1.000000000000000000 ) ) 
 REPRESENTATION_ITEM ( '' )  );
#39993=DIRECTION ( 'NONE',  ( -0.000000000000000000, -0.000000000000000000, -1.000000000000000000 ) ) ;
#39995=CARTESIAN_POINT ( 'NONE',  ( 35.05402655318504657, 2.143131898507880377E-16, -160.9317124430720582 ) ) ;
#39998=CARTESIAN_POINT ( 'NONE',  ( -85.67084718096784002, -1.750000000000009548, 39.79316129108089228 ) ) ;
#40000=EDGE_CURVE ( 'NONE', #44684, #46959, #40261, .T. ) ;
#40001=DIRECTION ( 'NONE',  ( 0.000000000000000000, 0.000000000000000000, 1.000000000000000000 ) ) ;
#40005=UNCERTAINTY_MEASURE_WITH_UNIT (LENGTH_MEASURE( 1.000000000000000082E-05 ), #7757, 'distance_accuracy_value', 'NONE');
#40007=VERTEX_POINT ( 'NONE', #16342 ) ;
#40012=ORIENTED_EDGE ( 'NONE', *, *, #36260, .F. ) ;
#40016=ORIENTED_EDGE ( 'NONE', *, *, #30073, .F. ) ;
#40026=ORIENTED_EDGE ( 'NONE', *, *, #26556, .T. ) ;
#40027=CARTESIAN_POINT ( 'NONE',  ( -166.6959734468149463, -1.750000000000010214, 40.81828755692798438 ) ) ;
#40028=CARTESIAN_POINT ( 'NONE',  ( -46.69597344681494633, -1.750000000000010658, 120.8182875569279702 ) ) ;
#40030=CARTESIAN_POINT ( 'NONE',  ( 73.30402655318508209, -1.750000000000010214, -39.18171244307202983 ) ) ;
#40031=CARTESIAN_POINT ( 'NONE',  ( 113.3040265531850537, 1.749999999999996891, 0.8182875569279768335 ) ) ;
#40032=EDGE_CURVE ( 'NONE', #44427, #48473, #13495, .T. ) ;
#40033=LINE ( 'NONE', #43349, #1189 ) ;
#40034=ADVANCED_FACE ( 'NONE', ( #33277 ), #1212, .T. ) ;
#40036=VERTEX_POINT ( 'NONE', #48100 ) ;
#40038=FACE_OUTER_BOUND ( 'NONE', #23614, .T. ) ;
#40044=CYLINDRICAL_SURFACE ( 'NONE', #9553, 1.750000000000015543 ) ;
#40049=DIRECTION ( 'NONE',  ( -1.000000000000000000, -0.000000000000000000, -0.000000000000000000 ) ) ;
#40051=EDGE_CURVE ( 'NONE', #38609, #31049, #45464, .T. ) ;
#40064=LINE ( 'NONE', #35465, #9238 ) ;
#40068=CARTESIAN_POINT ( 'NONE',  ( 191.5540265531851105, 0.000000000000000000, 165.0000000000000000 ) ) ;
#40070=DIRECTION ( 'NONE',  ( -1.000000000000000000, 0.000000000000000000, 0.000000000000000000 ) ) ;
#40071=ORIENTED_EDGE ( 'NONE', *, *, #17474, .T. ) ;
#40076=CARTESIAN_POINT ( 'NONE',  ( 75.05402655318509630, 2.143131898507880377E-16, -157.4317124430720014 ) ) ;
#40078=CARTESIAN_POINT ( 'NONE',  ( -128.4459734468149179, 0.000000000000000000, 42.56828755692794175 ) ) ;
#40082=CARTESIAN_POINT ( 'NONE',  ( -8.445973446814964092, 1.025126265847097207, 39.06828755692796307 ) ) ;
#40086=CARTESIAN_POINT ( 'NONE',  ( -84.94597344681494633, 2.143131898507880377E-16, -0.9317124430720247208 ) ) ;
#40089=DIRECTION ( 'NONE',  ( -0.000000000000000000, -0.000000000000000000, -1.000000000000000000 ) ) ;
#40090=ORIENTED_EDGE ( 'NONE', *, *, #1295, .F. ) ;
#40093=CARTESIAN_POINT ( 'NONE',  ( 195.0540265531851105, 2.143131898507880377E-16, -157.4317124430720582 ) ) ;
#40094=EDGE_CURVE ( 'NONE', #960, #9715, #48604, .T. ) ;
#40098=EDGE_LOOP ( 'NONE', ( #24461, #36564, #17522, #22869, #42149, #32673 ) ) ;
#40102=ORIENTED_EDGE ( 'NONE', *, *, #30711, .F. ) ;
#40106=EDGE_CURVE ( 'NONE', #37522, #10041, #50391, .T. ) ;
#40107=CARTESIAN_POINT ( 'NONE',  ( 210.0000000000000568, 0.000000000000000000, -39.18171244307202983 ) ) ;
#40108=DIRECTION ( 'NONE',  ( -1.000000000000000000, 0.000000000000000000, 0.000000000000000000 ) ) ;
#40111=ORIENTED_EDGE ( 'NONE', *, *, #45596, .F. ) ;
#40113=ORIENTED_EDGE ( 'NONE', *, *, #2602, .F. ) ;
#40117=ORIENTED_EDGE ( 'NONE', *, *, #9276, .T. ) ;
#40118=CARTESIAN_POINT ( 'NONE',  ( -164.9459734468149463, 2.143131898507880377E-16, 165.0000000000000000 ) ) ;
#40119=ORIENTED_EDGE ( 'NONE', *, *, #3966, .T. ) ;
#40123=CARTESIAN_POINT ( 'NONE',  ( -88.44597344681494633, -1.025126265847089213, -160.9317124430720014 ) ) ;
#40128=( BOUNDED_CURVE ( )  B_SPLINE_CURVE ( 3, ( #32577, #24616, #9201, #8722 ),
 .UNSPECIFIED., .F., .F. ) 
 B_SPLINE_CURVE_WITH_KNOTS ( ( 4, 4 ),
 ( 0.000000000000000000, 1.570796326794896558 ),
 .UNSPECIFIED. ) 
 CURVE ( )  GEOMETRIC_REPRESENTATION_ITEM ( )  RATIONAL_B_SPLINE_CURVE ( ( 1.000000000000000000, 0.8047378541243649375, 0.8047378541243649375, 1.000000000000000000 ) ) 
 REPRESENTATION_ITEM ( '' )  );
#40129=CARTESIAN_POINT ( 'NONE',  ( 153.3040265531850537, -1.750000000000009992, 160.8182875569279702 ) ) ;
#40135=CYLINDRICAL_SURFACE ( 'NONE', #24779, 1.750000000000015543 ) ;
#40136=ORIENTED_EDGE ( 'NONE', *, *, #17382, .F. ) ;
#40138=VERTEX_POINT ( 'NONE', #3472 ) ;
#40141=CARTESIAN_POINT ( 'NONE',  ( -210.0000000000000568, 0.000000000000000000, -117.4317124430720298 ) ) ;
#40144=CARTESIAN_POINT ( 'NONE',  ( 73.30402655318508209, 0.000000000000000000, 165.0000000000000000 ) ) ;
#40154=CARTESIAN_POINT ( 'NONE',  ( -205.6708471809678827, 1.750000000000009548, -0.2068387089191121020 ) ) ;
#40161=CARTESIAN_POINT ( 'NONE',  ( -44.94597344681493922, 2.143131898507880377E-16, 165.0000000000000000 ) ) ;
#40166=ORIENTED_EDGE ( 'NONE', *, *, #10431, .T. ) ;
#40169=VECTOR ( 'NONE', #40049, 1000.000000000000000 ) ;
#40173=FACE_OUTER_BOUND ( 'NONE', #13613, .T. ) ;
#40177=CARTESIAN_POINT ( 'NONE',  ( -166.6959734468149463, 0.000000000000000000, 165.0000000000000000 ) ) ;
#40180=DIRECTION ( 'NONE',  ( 1.000000000000000000, 0.000000000000000000, 0.000000000000000000 ) ) ;
#40181=ORIENTED_EDGE ( 'NONE', *, *, #2920, .F. ) ;
#40183=DIRECTION ( 'NONE',  ( 0.000000000000000000, 0.000000000000000000, 1.000000000000000000 ) ) ;
#40184=CARTESIAN_POINT ( 'NONE',  ( -165.6708471809677974, 1.750000000000010214, -118.1565861772249519 ) ) ;
#40187=CARTESIAN_POINT ( 'NONE',  ( 31.55402655318503236, 0.000000000000000000, 119.0682875569279702 ) ) ;
#40189=CARTESIAN_POINT ( 'NONE',  ( 154.3291528190321458, 1.750000000000009548, -160.2068387089191219 ) ) ;
#40192=CARTESIAN_POINT ( 'NONE',  ( 32.27890028733795447, 1.750000000000009548, 121.8434138227750623 ) ) ;
#40197=CARTESIAN_POINT ( 'NONE',  ( 155.0540265531850537, 2.143131898507880377E-16, 39.06828755692798438 ) ) ;
#40206=DIRECTION ( 'NONE',  ( -1.000000000000000000, -0.000000000000000000, -0.000000000000000000 ) ) ;
#40208=FACE_OUTER_BOUND ( 'NONE', #3686, .T. ) ;
#40209=LINE ( 'NONE', #28910, #13435 ) ;
#40211=ORIENTED_EDGE ( 'NONE', *, *, #858, .F. ) ;
#40212=EDGE_CURVE ( 'NONE', #40007, #37708, #46505, .T. ) ;
#40213=FACE_OUTER_BOUND ( 'NONE', #18382, .T. ) ;
#40214=EDGE_LOOP ( 'NONE', ( #13251, #12911, #11895, #16659, #14257, #38460 ) ) ;
#40216=CARTESIAN_POINT ( 'NONE',  ( 153.3040265531850537, 1.750000000000009992, 160.8182875569279702 ) ) ;
#40218=ORIENTED_EDGE ( 'NONE', *, *, #45272, .T. ) ;
#40221=ORIENTED_EDGE ( 'NONE', *, *, #9536, .T. ) ;
#40222=VERTEX_POINT ( 'NONE', #11958 ) ;
#40225=ADVANCED_FACE ( 'NONE', ( #30697 ), #11693, .T. ) ;
#40227=EDGE_LOOP ( 'NONE', ( #39094, #10957 ) ) ;
#40229=AXIS2_PLACEMENT_3D ( 'NONE', #32261, #32015, #36642 ) ;
#40230=CARTESIAN_POINT ( 'NONE',  ( -87.72109971266203843, -1.750000000000010214, -120.2068387089191219 ) ) ;
#40233=LINE ( 'NONE', #44304, #39541 ) ;
#40239=CARTESIAN_POINT ( 'NONE',  ( 113.3040265531850537, 0.000000000000000000, 165.0000000000000000 ) ) ;
#40240=CARTESIAN_POINT ( 'NONE',  ( -87.72109971266203843, -1.750000000000009548, -158.1565861772249377 ) ) ;
#40242=EDGE_CURVE ( 'NONE', #45334, #32429, #30825, .T. ) ;
#40244=EDGE_CURVE ( 'NONE', #47433, #13085, #48448, .T. ) ;
#40246=EDGE_CURVE ( 'NONE', #47361, #22212, #8584, .T. ) ;
#40249=CYLINDRICAL_SURFACE ( 'NONE', #16353, 1.750000000000001554 ) ;
#40253=( BOUNDED_CURVE ( )  B_SPLINE_CURVE ( 3, ( #7764, #22887, #38566, #11344 ),
 .UNSPECIFIED., .F., .F. ) 
 B_SPLINE_CURVE_WITH_KNOTS ( ( 4, 4 ),
 ( 4.712388980384689674, 6.283185307179586232 ),
 .UNSPECIFIED. ) 
 CURVE ( )  GEOMETRIC_REPRESENTATION_ITEM ( )  RATIONAL_B_SPLINE_CURVE ( ( 1.000000000000000000, 0.8047378541243649375, 0.8047378541243649375, 1.000000000000000000 ) ) 
 REPRESENTATION_ITEM ( '' )  );
#40255=DIRECTION ( 'NONE',  ( -1.000000000000000000, 0.000000000000000000, 0.000000000000000000 ) ) ;
#40256=CARTESIAN_POINT ( 'NONE',  ( -210.0000000000000568, 0.000000000000000000, 0.8182875569279768335 ) ) ;
#40261=( BOUNDED_CURVE ( )  B_SPLINE_CURVE ( 3, ( #16597, #32256, #4297, #35616 ),
 .UNSPECIFIED., .F., .F. ) 
 B_SPLINE_CURVE_WITH_KNOTS ( ( 4, 4 ),
 ( 4.712388980384689674, 6.283185307179586232 ),
 .UNSPECIFIED. ) 
 CURVE ( )  GEOMETRIC_REPRESENTATION_ITEM ( )  RATIONAL_B_SPLINE_CURVE ( ( 1.000000000000000000, 0.8047378541243649375, 0.8047378541243649375, 1.000000000000000000 ) ) 
 REPRESENTATION_ITEM ( '' )  );
#40262=EDGE_LOOP ( 'NONE', ( #30076, #1911, #22233, #27083, #36756 ) ) ;
#40264=EDGE_CURVE ( 'NONE', #20298, #40360, #43242, .T. ) ;
#40268=EDGE_CURVE ( 'NONE', #40908, #40762, #43247, .T. ) ;
#40273=ORIENTED_EDGE ( 'NONE', *, *, #41003, .T. ) ;
#40276=EDGE_CURVE ( 'NONE', #41270, #27700, #36384, .T. ) ;
#40278=( BOUNDED_CURVE ( )  B_SPLINE_CURVE ( 3, ( #26593, #15802, #47060, #42237 ),
 .UNSPECIFIED., .F., .F. ) 
 B_SPLINE_CURVE_WITH_KNOTS ( ( 4, 4 ),
 ( 0.000000000000000000, 1.570796326794896558 ),
 .UNSPECIFIED. ) 
 CURVE ( )  GEOMETRIC_REPRESENTATION_ITEM ( )  RATIONAL_B_SPLINE_CURVE ( ( 1.000000000000000000, 0.8047378541243649375, 0.8047378541243649375, 1.000000000000000000 ) ) 
 REPRESENTATION_ITEM ( '' )  );
#40282=ADVANCED_FACE ( 'NONE', ( #44179 ), #41103, .T. ) ;
#40289=CARTESIAN_POINT ( 'NONE',  ( 194.3291528190321742, 1.750000000000010214, 81.84341382277507648 ) ) ;
#40291=ORIENTED_EDGE ( 'NONE', *, *, #23730, .T. ) ;
#40292=CARTESIAN_POINT ( 'NONE',  ( -166.6959734468149463, -1.750000000000009992, 160.8182875569279702 ) ) ;
#40298=CARTESIAN_POINT ( 'NONE',  ( 74.32915281903215998, 1.750000000000010214, 79.79316129108087807 ) ) ;
#40305=DIRECTION ( 'NONE',  ( -1.000000000000000000, -0.000000000000000000, -0.000000000000000000 ) ) ;
#40310=CARTESIAN_POINT ( 'NONE',  ( -164.9459734468149463, 1.025126265847089657, -120.9317124430720440 ) ) ;
#40319=FACE_OUTER_BOUND ( 'NONE', #38704, .T. ) ;
#40320=ORIENTED_EDGE ( 'NONE', *, *, #27163, .F. ) ;
#40321=CARTESIAN_POINT ( 'NONE',  ( 115.0540265531850395, -1.025126265847081886, -40.93171244307202272 ) ) ;
#40325=DIRECTION ( 'NONE',  ( 1.000000000000000000, 0.000000000000000000, 0.000000000000000000 ) ) ;
#40327=VERTEX_POINT ( 'NONE', #37289 ) ;
#40329=CARTESIAN_POINT ( 'NONE',  ( -124.9459734468149321, 1.025126265847081442, -0.9317124430720195027 ) ) ;
#40332=CARTESIAN_POINT ( 'NONE',  ( 152.2789002873379900, -1.750000000000009548, -160.2068387089191219 ) ) ;
#40333=CARTESIAN_POINT ( 'NONE',  ( 33.30402655318503946, 0.000000000000000000, 165.0000000000000000 ) ) ;
#40335=CARTESIAN_POINT ( 'NONE',  ( 75.05402655318509630, -1.025126265847088991, 159.0682875569279418 ) ) ;
#40337=LINE ( 'NONE', #10039, #43517 ) ;
#40343=EDGE_LOOP ( 'NONE', ( #7857, #46462, #31461, #43796, #44537 ) ) ;
#40346=CARTESIAN_POINT ( 'NONE',  ( -208.4459734468148611, -1.025126265847089657, -120.9317124430720440 ) ) ;
#40347=CARTESIAN_POINT ( 'NONE',  ( 35.05402655318504657, 2.143131898507880377E-16, -120.9317124430720725 ) ) ;
#40351=CARTESIAN_POINT ( 'NONE',  ( -166.6959734468149463, 0.000000000000000000, 165.0000000000000000 ) ) ;
#40358=VERTEX_POINT ( 'NONE', #34686 ) ;
#40359=EDGE_CURVE ( 'NONE', #4058, #22032, #36079, .T. ) ;
#40360=VERTEX_POINT ( 'NONE', #2591 ) ;
#40362=CARTESIAN_POINT ( 'NONE',  ( -4.945973446814903696, 2.143131898507912917E-16, 122.5682875569279986 ) ) ;
#40365=DIRECTION ( 'NONE',  ( 0.000000000000000000, 0.000000000000000000, 1.000000000000000000 ) ) ;
#40373=ADVANCED_FACE ( 'NONE', ( #6212 ), #19000, .T. ) ;
#40374=EDGE_CURVE ( 'NONE', #8918, #27492, #11483, .T. ) ;
#40375=CARTESIAN_POINT ( 'NONE',  ( -166.6959734468149463, 1.750000000000009992, 160.8182875569279702 ) ) ;
#40382=EDGE_CURVE ( 'NONE', #29172, #4462, #44866, .T. ) ;
#40385=VECTOR ( 'NONE', #44389, 1000.000000000000000 ) ;
#40386=EDGE_CURVE ( 'NONE', #20063, #35915, #1307, .T. ) ;
#40390=AXIS2_PLACEMENT_3D ( 'NONE', #19017, #45691, #7498 ) ;
#40391=CARTESIAN_POINT ( 'NONE',  ( -88.44597344681497475, 0.000000000000000000, 165.0000000000000000 ) ) ;
#40392=EDGE_LOOP ( 'NONE', ( #29049, #33017, #37441, #21599, #30221, #24079 ) ) ;
#40394=EDGE_CURVE ( 'NONE', #20584, #17646, #21866, .T. ) ;
#40395=CARTESIAN_POINT ( 'NONE',  ( 193.3040265531851105, 1.750000000000009992, 0.8182875569279768335 ) ) ;
#40396=ORIENTED_EDGE ( 'NONE', *, *, #18689, .F. ) ;
#40401=FACE_OUTER_BOUND ( 'NONE', #34916, .T. ) ;
#40402=ORIENTED_EDGE ( 'NONE', *, *, #31852, .T. ) ;
#40403=VERTEX_POINT ( 'NONE', #10805 ) ;
#40406=VERTEX_POINT ( 'NONE', #37779 ) ;
#40408=CYLINDRICAL_SURFACE ( 'NONE', #45201, 1.749999999999973799 ) ;
#40410=CARTESIAN_POINT ( 'NONE',  ( 193.3040265531851105, -1.750000000000010658, -79.18171244307201562 ) ) ;
#40411=CARTESIAN_POINT ( 'NONE',  ( 71.55402655318505367, 0.000000000000000000, 119.0682875569279560 ) ) ;
#40412=ORIENTED_EDGE ( 'NONE', *, *, #47660, .T. ) ;
#40415=AXIS2_PLACEMENT_3D ( 'NONE', #15880, #47133, #12036 ) ;
#40416=ORIENTED_EDGE ( 'NONE', *, *, #2916, .T. ) ;
#40418=ADVANCED_FACE ( 'NONE', ( #17991 ), #41606, .T. ) ;
#40424=( BOUNDED_CURVE ( )  B_SPLINE_CURVE ( 3, ( #5015, #48329, #36861, #20671 ),
 .UNSPECIFIED., .F., .F. ) 
 B_SPLINE_CURVE_WITH_KNOTS ( ( 4, 4 ),
 ( 4.712388980384689674, 6.283185307179586232 ),
 .UNSPECIFIED. ) 
 CURVE ( )  GEOMETRIC_REPRESENTATION_ITEM ( )  RATIONAL_B_SPLINE_CURVE ( ( 1.000000000000000000, 0.8047378541243649375, 0.8047378541243649375, 1.000000000000000000 ) ) 
 REPRESENTATION_ITEM ( '' )  );
#40425=CARTESIAN_POINT ( 'NONE',  ( 115.0540265531850395, 2.143131898507847836E-16, 119.0682875569279844 ) ) ;
#40426=VERTEX_POINT ( 'NONE', #30072 ) ;
#40430=ORIENTED_EDGE ( 'NONE', *, *, #26827, .F. ) ;
#40446=CARTESIAN_POINT ( 'NONE',  ( -210.0000000000000568, 0.000000000000000000, 40.81828755692798438 ) ) ;
#40448=CARTESIAN_POINT ( 'NONE',  ( -44.94597344681493922, 2.143131898507880377E-16, 79.06828755692797017 ) ) ;
#40456=DIRECTION ( 'NONE',  ( -1.000000000000000000, -0.000000000000000000, -0.000000000000000000 ) ) ;
#40457=DIRECTION ( 'NONE',  ( -1.000000000000000000, -0.000000000000000000, -0.000000000000000000 ) ) ;
#40459=DIRECTION ( 'NONE',  ( -1.000000000000000000, -0.000000000000000000, -0.000000000000000000 ) ) ;
#40466=DIRECTION ( 'NONE',  ( -0.000000000000000000, -0.000000000000000000, -1.000000000000000000 ) ) ;
#40469=VERTEX_POINT ( 'NONE', #46431 ) ;
#40472=EDGE_CURVE ( 'NONE', #19269, #44210, #6536, .T. ) ;
#40479=AXIS2_PLACEMENT_3D ( 'NONE', #25884, #46088, #42282 ) ;
#40483=DIRECTION ( 'NONE',  ( -1.000000000000000000, -0.000000000000000000, -0.000000000000000000 ) ) ;
#40485=VERTEX_POINT ( 'NONE', #38786 ) ;
#40486=VECTOR ( 'NONE', #40459, 1000.000000000000000 ) ;
#40487=CARTESIAN_POINT ( 'NONE',  ( -88.44597344681497475, 0.000000000000000000, -120.9317124430720725 ) ) ;
#40490=DIRECTION ( 'NONE',  ( -1.000000000000000000, 0.000000000000000000, 0.000000000000000000 ) ) ;
#40492=CARTESIAN_POINT ( 'NONE',  ( 210.0000000000000568, 2.143131898507876926E-16, -120.9317124430720582 ) ) ;
#40496=CYLINDRICAL_SURFACE ( 'NONE', #36325, 1.750000000000008438 ) ;
#40500=( BOUNDED_CURVE ( )  B_SPLINE_CURVE ( 3, ( #42225, #19196, #19721, #38726 ),
 .UNSPECIFIED., .F., .F. ) 
 B_SPLINE_CURVE_WITH_KNOTS ( ( 4, 4 ),
 ( 0.000000000000000000, 1.570796326794896558 ),
 .UNSPECIFIED. ) 
 CURVE ( )  GEOMETRIC_REPRESENTATION_ITEM ( )  RATIONAL_B_SPLINE_CURVE ( ( 1.000000000000000000, 0.8047378541243649375, 0.8047378541243649375, 1.000000000000000000 ) ) 
 REPRESENTATION_ITEM ( '' )  );
#40502=VERTEX_POINT ( 'NONE', #35713 ) ;
#40510=CARTESIAN_POINT ( 'NONE',  ( -48.44597344681492501, 2.143131898507880377E-16, -160.9317124430720298 ) ) ;
#40515=CARTESIAN_POINT ( 'NONE',  ( 31.55402655318503236, 0.000000000000000000, -157.4317124430720014 ) ) ;
#40520=VERTEX_POINT ( 'NONE', #39798 ) ;
#40521=EDGE_LOOP ( 'NONE', ( #44618, #44848, #34212, #11780, #20639, #15051 ) ) ;
#40527=DIRECTION ( 'NONE',  ( -0.000000000000000000, -0.000000000000000000, -1.000000000000000000 ) ) ;
#40532=ORIENTED_EDGE ( 'NONE', *, *, #39854, .F. ) ;
#40538=ORIENTED_EDGE ( 'NONE', *, *, #4877, .T. ) ;
#40541=EDGE_LOOP ( 'NONE', ( #15953, #48923, #10610, #6823, #39272, #24324 ) ) ;
#40545=ORIENTED_EDGE ( 'NONE', *, *, #29517, .T. ) ;
#40551=ORIENTED_EDGE ( 'NONE', *, *, #46595, .T. ) ;
#40553=CARTESIAN_POINT ( 'NONE',  ( 114.3291528190321173, -1.749999999999996669, 121.8434138227750481 ) ) ;
#40554=( BOUNDED_CURVE ( )  B_SPLINE_CURVE ( 3, ( #10764, #49219, #14616, #37991 ),
 .UNSPECIFIED., .F., .F. ) 
 B_SPLINE_CURVE_WITH_KNOTS ( ( 4, 4 ),
 ( 4.712388980384689674, 6.283185307179586232 ),
 .UNSPECIFIED. ) 
 CURVE ( )  GEOMETRIC_REPRESENTATION_ITEM ( )  RATIONAL_B_SPLINE_CURVE ( ( 1.000000000000000000, 0.8047378541243649375, 0.8047378541243649375, 1.000000000000000000 ) ) 
 REPRESENTATION_ITEM ( '' )  );
#40556=ADVANCED_FACE ( 'NONE', ( #23113 ), #42857, .T. ) ;
#40560=LINE ( 'NONE', #10012, #41901 ) ;
#40562=( BOUNDED_CURVE ( )  B_SPLINE_CURVE ( 3, ( #24680, #1075, #48225, #36492 ),
 .UNSPECIFIED., .F., .F. ) 
 B_SPLINE_CURVE_WITH_KNOTS ( ( 4, 4 ),
 ( 1.570796326794896558, 3.141592653589793116 ),
 .UNSPECIFIED. ) 
 CURVE ( )  GEOMETRIC_REPRESENTATION_ITEM ( )  RATIONAL_B_SPLINE_CURVE ( ( 1.000000000000000000, 0.8047378541243649375, 0.8047378541243649375, 1.000000000000000000 ) ) 
 REPRESENTATION_ITEM ( '' )  );
#40571=ORIENTED_EDGE ( 'NONE', *, *, #21838, .T. ) ;
#40574=ORIENTED_EDGE ( 'NONE', *, *, #33903, .F. ) ;
#40576=CARTESIAN_POINT ( 'NONE',  ( 210.0000000000000568, 0.000000000000000000, 160.8182875569279702 ) ) ;
#40578=CARTESIAN_POINT ( 'NONE',  ( -86.69597344681494633, 1.750000000000010658, -79.18171244307201562 ) ) ;
#40579=EDGE_LOOP ( 'NONE', ( #47370, #12919 ) ) ;
#40582=VERTEX_POINT ( 'NONE', #21040 ) ;
#40588=ORIENTED_EDGE ( 'NONE', *, *, #44865, .F. ) ;
#40590=ORIENTED_EDGE ( 'NONE', *, *, #23345, .F. ) ;
#40594=ADVANCED_FACE ( 'NONE', ( #32090 ), #36975, .T. ) ;
#40596=VERTEX_POINT ( 'NONE', #1548 ) ;
#40600=CARTESIAN_POINT ( 'NONE',  ( -128.4459734468149179, 0.000000000000000000, 162.5682875569279702 ) ) ;
#40604=VERTEX_POINT ( 'NONE', #16677 ) ;
#40607=CYLINDRICAL_SURFACE ( 'NONE', #8369, 1.749999999999987566 ) ;
#40611=VERTEX_POINT ( 'NONE', #25395 ) ;
#40617=CARTESIAN_POINT ( 'NONE',  ( 73.30402655318508209, 1.750000000000010658, -79.18171244307201562 ) ) ;
#40620=CARTESIAN_POINT ( 'NONE',  ( -126.6959734468149321, -1.749999999999996891, 0.8182875569279768335 ) ) ;
#40634=FACE_OUTER_BOUND ( 'NONE', #8473, .T. ) ;
#40636=EDGE_CURVE ( 'NONE', #48865, #38333, #48186, .T. ) ;
#40645=ORIENTED_EDGE ( 'NONE', *, *, #18331, .T. ) ;
#40648=CARTESIAN_POINT ( 'NONE',  ( -126.6959734468149321, 1.749999999999996891, 160.8182875569279702 ) ) ;
#40657=CIRCLE ( 'NONE', #16927, 1.750000000000036193 ) ;
#40658=EDGE_CURVE ( 'NONE', #40007, #41009, #16726, .T. ) ;
#40659=EDGE_CURVE ( 'NONE', #34244, #38646, #29747, .T. ) ;
#40660=ORIENTED_EDGE ( 'NONE', *, *, #49340, .T. ) ;
#40662=CARTESIAN_POINT ( 'NONE',  ( -48.44597344681496054, 1.025126265847089213, -37.43171244307202272 ) ) ;
#40664=CARTESIAN_POINT ( 'NONE',  ( -48.44597344681496054, 1.025126265847089657, -120.9317124430720440 ) ) ;
#40665=CARTESIAN_POINT ( 'NONE',  ( 32.27890028733795447, 1.750000000000009548, 159.7931612910809065 ) ) ;
#40668=ORIENTED_EDGE ( 'NONE', *, *, #41853, .F. ) ;
#40669=EDGE_LOOP ( 'NONE', ( #21211, #12990, #25389, #38853, #34373, #32686 ) ) ;
#40670=ADVANCED_FACE ( 'NONE', ( #18184 ), #41547, .T. ) ;
#40673=CARTESIAN_POINT ( 'NONE',  ( 195.0540265531851105, 2.143131898507880377E-16, 119.0682875569279702 ) ) ;
#40678=ORIENTED_EDGE ( 'NONE', *, *, #14838, .T. ) ;
#40679=EDGE_LOOP ( 'NONE', ( #37605, #41466, #14074, #3682, #44642, #10790 ) ) ;
#40684=FACE_OUTER_BOUND ( 'NONE', #1591, .T. ) ;
#40685=FACE_OUTER_BOUND ( 'NONE', #42379, .T. ) ;
#40688=EDGE_CURVE ( 'NONE', #28309, #5743, #3039, .T. ) ;
#40700=CARTESIAN_POINT ( 'NONE',  ( -127.7210997126620242, 1.749999999999997113, 79.79316129108087807 ) ) ;
#40702=VECTOR ( 'NONE', #11498, 1000.000000000000000 ) ;
#40704=CARTESIAN_POINT ( 'NONE',  ( 115.0540265531850395, 2.143131898507847836E-16, -160.9317124430720014 ) ) ;
#40706=DIRECTION ( 'NONE',  ( -1.000000000000000000, -0.000000000000000000, -0.000000000000000000 ) ) ;
#40707=CARTESIAN_POINT ( 'NONE',  ( -126.6959734468149321, 1.749999999999997113, -39.18171244307202983 ) ) ;
#40710=DIRECTION ( 'NONE',  ( 0.000000000000000000, 0.000000000000000000, 1.000000000000000000 ) ) ;
#40711=EDGE_LOOP ( 'NONE', ( #29726, #44093, #25016, #17464, #29471, #33232 ) ) ;
#40713=LINE ( 'NONE', #31765, #41832 ) ;
#40714=EDGE_CURVE ( 'NONE', #10095, #5769, #15077, .T. ) ;
#40715=EDGE_CURVE ( 'NONE', #26837, #21965, #14852, .T. ) ;
#40718=DIRECTION ( 'NONE',  ( -1.000000000000000000, 0.000000000000000000, 0.000000000000000000 ) ) ;
#40719=CARTESIAN_POINT ( 'NONE',  ( -168.4459734468149463, 0.000000000000000000, -77.43171244307204404 ) ) ;
#40722=( BOUNDED_CURVE ( )  B_SPLINE_CURVE ( 3, ( #28540, #40346, #31393, #27542 ),
 .UNSPECIFIED., .F., .F. ) 
 B_SPLINE_CURVE_WITH_KNOTS ( ( 4, 4 ),
 ( 0.000000000000000000, 1.570796326794896558 ),
 .UNSPECIFIED. ) 
 CURVE ( )  GEOMETRIC_REPRESENTATION_ITEM ( )  RATIONAL_B_SPLINE_CURVE ( ( 1.000000000000000000, 0.8047378541243649375, 0.8047378541243649375, 1.000000000000000000 ) ) 
 REPRESENTATION_ITEM ( '' )  );
#40723=ADVANCED_FACE ( 'NONE', ( #14339 ), #7159, .T. ) ;
#40724=FACE_OUTER_BOUND ( 'NONE', #46950, .T. ) ;
#40726=ADVANCED_FACE ( 'NONE', ( #49199 ), #18437, .T. ) ;
#40727=CYLINDRICAL_SURFACE ( 'NONE', #6266, 1.750000000000015543 ) ;
#40729=DIRECTION ( 'NONE',  ( 0.000000000000000000, 0.000000000000000000, 1.000000000000000000 ) ) ;
#40730=CARTESIAN_POINT ( 'NONE',  ( -84.94597344681493212, 1.025126265847089435, 2.568287556927986159 ) ) ;
#40731=EDGE_LOOP ( 'NONE', ( #28275, #23009, #44800, #42672, #14451, #33073 ) ) ;
#40735=EDGE_CURVE ( 'NONE', #50479, #44495, #18958, .T. ) ;
#40740=CARTESIAN_POINT ( 'NONE',  ( 151.5540265531850537, 0.000000000000000000, 42.56828755692798438 ) ) ;
#40741=CARTESIAN_POINT ( 'NONE',  ( 73.30402655318508209, 1.750000000000009992, 160.8182875569279702 ) ) ;
#40744=APPLICATION_CONTEXT ( 'automotive_design' ) ;
#40748=FACE_OUTER_BOUND ( 'NONE', #46787, .T. ) ;
#40757=CARTESIAN_POINT ( 'NONE',  ( -166.6959734468149463, -1.750000000000009992, 160.8182875569279702 ) ) ;
#40758=EDGE_CURVE ( 'NONE', #9269, #31049, #13822, .T. ) ;
#40762=VERTEX_POINT ( 'NONE', #37714 ) ;
#40765=CARTESIAN_POINT ( 'NONE',  ( 210.0000000000000568, 0.000000000000000000, 0.8182875569279768335 ) ) ;
#40767=CARTESIAN_POINT ( 'NONE',  ( -207.7210997126620384, -1.750000000000010214, 121.8434138227750623 ) ) ;
#40770=ORIENTED_EDGE ( 'NONE', *, *, #33414, .T. ) ;
#40778=CARTESIAN_POINT ( 'NONE',  ( -167.7210997126620384, -1.750000000000009548, 159.7931612910809065 ) ) ;
#40780=DIRECTION ( 'NONE',  ( 1.000000000000000000, 0.000000000000000000, 0.000000000000000000 ) ) ;
#40781=ORIENTED_EDGE ( 'NONE', *, *, #30292, .F. ) ;
#40787=VERTEX_POINT ( 'NONE', #21799 ) ;
#40791=PLANE ( 'NONE',  #39791 ) ;
#40797=( BOUNDED_CURVE ( )  B_SPLINE_CURVE ( 3, ( #50704, #47614, #15601, #7918 ),
 .UNSPECIFIED., .F., .F. ) 
 B_SPLINE_CURVE_WITH_KNOTS ( ( 4, 4 ),
 ( 0.000000000000000000, 1.570796326794896558 ),
 .UNSPECIFIED. ) 
 CURVE ( )  GEOMETRIC_REPRESENTATION_ITEM ( )  RATIONAL_B_SPLINE_CURVE ( ( 1.000000000000000000, 0.8047378541243649375, 0.8047378541243649375, 1.000000000000000000 ) ) 
 REPRESENTATION_ITEM ( '' )  );
#40799=CARTESIAN_POINT ( 'NONE',  ( 151.5540265531850537, 0.000000000000000000, -80.93171244307201562 ) ) ;
#40801=DIRECTION ( 'NONE',  ( 0.000000000000000000, 0.000000000000000000, 1.000000000000000000 ) ) ;
#40803=VERTEX_POINT ( 'NONE', #27670 ) ;
#40808=ORIENTED_EDGE ( 'NONE', *, *, #41387, .T. ) ;
#40814=VERTEX_POINT ( 'NONE', #27170 ) ;
#40815=CARTESIAN_POINT ( 'NONE',  ( -208.4459734468149463, 0.000000000000000000, -157.4317124430720582 ) ) ;
#40820=CARTESIAN_POINT ( 'NONE',  ( 191.5540265531851105, 0.000000000000000000, -37.43171244307205825 ) ) ;
#40821=CARTESIAN_POINT ( 'NONE',  ( -208.4459734468149179, 2.143131898507880377E-16, -160.9317124430720298 ) ) ;
#40824=CARTESIAN_POINT ( 'NONE',  ( -7.721099712662037540, 1.750000000000023315, -78.15658617722490931 ) ) ;
#40825=ORIENTED_EDGE ( 'NONE', *, *, #37481, .F. ) ;
#40826=DIRECTION ( 'NONE',  ( -0.000000000000000000, -0.000000000000000000, -1.000000000000000000 ) ) ;
#40827=CARTESIAN_POINT ( 'NONE',  ( -126.6959734468149321, 1.749999999999997335, -119.1817124430720440 ) ) ;
#40828=DIRECTION ( 'NONE',  ( -0.000000000000000000, -0.000000000000000000, -1.000000000000000000 ) ) ;
#40837=ORIENTED_EDGE ( 'NONE', *, *, #14215, .T. ) ;
#40839=EDGE_CURVE ( 'NONE', #47564, #40762, #41301, .T. ) ;
#40840=CARTESIAN_POINT ( 'NONE',  ( 152.2789002873379900, -1.750000000000010214, 79.79316129108087807 ) ) ;
#40841=VERTEX_POINT ( 'NONE', #23569 ) ;
#40845=( BOUNDED_CURVE ( )  B_SPLINE_CURVE ( 3, ( #17421, #22279, #14064, #6125 ),
 .UNSPECIFIED., .F., .F. ) 
 B_SPLINE_CURVE_WITH_KNOTS ( ( 4, 4 ),
 ( 4.712388980384689674, 6.283185307179586232 ),
 .UNSPECIFIED. ) 
 CURVE ( )  GEOMETRIC_REPRESENTATION_ITEM ( )  RATIONAL_B_SPLINE_CURVE ( ( 1.000000000000000000, 0.8047378541243649375, 0.8047378541243649375, 1.000000000000000000 ) ) 
 REPRESENTATION_ITEM ( '' )  );
#40846=CARTESIAN_POINT ( 'NONE',  ( -8.445973446814976526, 0.000000000000000000, 165.0000000000000000 ) ) ;
#40854=( BOUNDED_CURVE ( )  B_SPLINE_CURVE ( 3, ( #37571, #29848, #3391, #7255 ),
 .UNSPECIFIED., .F., .F. ) 
 B_SPLINE_CURVE_WITH_KNOTS ( ( 4, 4 ),
 ( 3.141592653589793116, 4.712388980384689674 ),
 .UNSPECIFIED. ) 
 CURVE ( )  GEOMETRIC_REPRESENTATION_ITEM ( )  RATIONAL_B_SPLINE_CURVE ( ( 1.000000000000000000, 0.8047378541243649375, 0.8047378541243649375, 1.000000000000000000 ) ) 
 REPRESENTATION_ITEM ( '' )  );
#40860=ORIENTED_EDGE ( 'NONE', *, *, #21433, .F. ) ;
#40864=LINE ( 'NONE', #32668, #34264 ) ;
#40865=CARTESIAN_POINT ( 'NONE',  ( -4.945973446814903696, 2.143131898507912917E-16, 119.0682875569279418 ) ) ;
#40866=DIRECTION ( 'NONE',  ( 0.000000000000000000, 0.000000000000000000, -1.000000000000000000 ) ) ;
#40874=EDGE_CURVE ( 'NONE', #34536, #46541, #13424, .T. ) ;
#40878=CARTESIAN_POINT ( 'NONE',  ( 31.55402655318503236, 0.000000000000000000, 165.0000000000000000 ) ) ;
#40879=ORIENTED_EDGE ( 'NONE', *, *, #48957, .F. ) ;
#40880=CARTESIAN_POINT ( 'NONE',  ( -44.94597344681493922, 2.143131898507880377E-16, 82.56828755692798438 ) ) ;
#40897=CARTESIAN_POINT ( 'NONE',  ( 151.5540265531850537, 0.000000000000000000, -117.4317124430720725 ) ) ;
#40902=EDGE_CURVE ( 'NONE', #41828, #6375, #50396, .T. ) ;
#40904=FACE_OUTER_BOUND ( 'NONE', #10209, .T. ) ;
#40906=CARTESIAN_POINT ( 'NONE',  ( 35.05402655318504657, 1.025126265847089435, 159.0682875569279418 ) ) ;
#40908=VERTEX_POINT ( 'NONE', #25090 ) ;
#40910=EDGE_CURVE ( 'NONE', #5910, #26020, #13264, .T. ) ;
#40911=ORIENTED_EDGE ( 'NONE', *, *, #10506, .F. ) ;
#40912=EDGE_CURVE ( 'NONE', #7079, #7012, #24835, .T. ) ;
#40914=DIRECTION ( 'NONE',  ( -1.000000000000000000, -0.000000000000000000, -0.000000000000000000 ) ) ;
#40915=ORIENTED_EDGE ( 'NONE', *, *, #47606, .F. ) ;
#40916=ORIENTED_EDGE ( 'NONE', *, *, #2008, .T. ) ;
#40921=CARTESIAN_POINT ( 'NONE',  ( -124.9459734468149463, 2.143131898507847836E-16, 39.06828755692798438 ) ) ;
#40927=CARTESIAN_POINT ( 'NONE',  ( -44.94597344681493922, 2.143131898507880377E-16, 165.0000000000000000 ) ) ;
#40930=EDGE_CURVE ( 'NONE', #6064, #40611, #48147, .T. ) ;
#40934=CARTESIAN_POINT ( 'NONE',  ( 151.5540265531850537, 0.000000000000000000, -157.4317124430720582 ) ) ;
#40939=EDGE_CURVE ( 'NONE', #26375, #48612, #46804, .T. ) ;
#40940=ADVANCED_FACE ( 'NONE', ( #48127 ), #32038, .T. ) ;
#40941=EDGE_CURVE ( 'NONE', #36323, #45661, #37724, .T. ) ;
#40942=DIRECTION ( 'NONE',  ( -1.000000000000000000, 0.000000000000000000, 0.000000000000000000 ) ) ;
#40943=CARTESIAN_POINT ( 'NONE',  ( -204.9459734468149463, 2.143131898507880377E-16, -117.4317124430720725 ) ) ;
#40953=CARTESIAN_POINT ( 'NONE',  ( -206.6959734468149463, 0.000000000000000000, 165.0000000000000000 ) ) ;
#40969=ORIENTED_EDGE ( 'NONE', *, *, #21484, .F. ) ;
#40976=DIRECTION ( 'NONE',  ( 1.000000000000000000, 0.000000000000000000, -0.000000000000000000 ) ) ;
#40985=CARTESIAN_POINT ( 'NONE',  ( -208.4459734468148611, -1.025126265847089879, -117.4317124430720156 ) ) ;
#40987=LINE ( 'NONE', #13771, #6319 ) ;
#40991=CARTESIAN_POINT ( 'NONE',  ( 31.55402655318503236, 0.000000000000000000, 42.56828755692798438 ) ) ;
#40992=CARTESIAN_POINT ( 'NONE',  ( 210.0000000000000568, 0.000000000000000000, -119.1817124430720440 ) ) ;
#40996=( BOUNDED_CURVE ( )  B_SPLINE_CURVE ( 3, ( #45820, #17404, #29457, #14043 ),
 .UNSPECIFIED., .F., .F. ) 
 B_SPLINE_CURVE_WITH_KNOTS ( ( 4, 4 ),
 ( 4.712388980384689674, 6.283185307179586232 ),
 .UNSPECIFIED. ) 
 CURVE ( )  GEOMETRIC_REPRESENTATION_ITEM ( )  RATIONAL_B_SPLINE_CURVE ( ( 1.000000000000000000, 0.8047378541243649375, 0.8047378541243649375, 1.000000000000000000 ) ) 
 REPRESENTATION_ITEM ( '' )  );
#40997=ADVANCED_FACE ( 'NONE', ( #1244 ), #28183, .T. ) ;
#41003=EDGE_CURVE ( 'NONE', #44183, #38646, #985, .T. ) ;
#41008=EDGE_CURVE ( 'NONE', #36841, #44023, #23922, .T. ) ;
#41009=VERTEX_POINT ( 'NONE', #2729 ) ;
#41016=EDGE_CURVE ( 'NONE', #2518, #7079, #2623, .T. ) ;
#41017=( BOUNDED_CURVE ( )  B_SPLINE_CURVE ( 3, ( #731, #16133, #27425, #31030 ),
 .UNSPECIFIED., .F., .F. ) 
 B_SPLINE_CURVE_WITH_KNOTS ( ( 4, 4 ),
 ( 0.000000000000000000, 1.570796326794896558 ),
 .UNSPECIFIED. ) 
 CURVE ( )  GEOMETRIC_REPRESENTATION_ITEM ( )  RATIONAL_B_SPLINE_CURVE ( ( 1.000000000000000000, 0.8047378541243649375, 0.8047378541243649375, 1.000000000000000000 ) ) 
 REPRESENTATION_ITEM ( '' )  );
#41025=DIRECTION ( 'NONE',  ( -1.000000000000000000, 0.000000000000000000, 0.000000000000000000 ) ) ;
#41026=ORIENTED_EDGE ( 'NONE', *, *, #2626, .T. ) ;
#41039=ORIENTED_EDGE ( 'NONE', *, *, #595, .T. ) ;
#41045=ADVANCED_FACE ( 'NONE', ( #29434 ), #18626, .T. ) ;
#41049=CARTESIAN_POINT ( 'NONE',  ( -166.6959734468149463, 1.750000000000010214, -39.18171244307202983 ) ) ;
#41050=ORIENTED_EDGE ( 'NONE', *, *, #4825, .T. ) ;
#41055=CARTESIAN_POINT ( 'NONE',  ( 114.3291528190321173, 1.749999999999996891, -118.1565861772249661 ) ) ;
#41057=EDGE_CURVE ( 'NONE', #45408, #47482, #18376, .T. ) ;
#41058=EDGE_CURVE ( 'NONE', #45409, #6771, #27534, .T. ) ;
#41063=CARTESIAN_POINT ( 'NONE',  ( 210.0000000000000568, 0.000000000000000000, -119.1817124430720440 ) ) ;
#41065=LINE ( 'NONE', #28516, #28743 ) ;
#41070=DIRECTION ( 'NONE',  ( -1.000000000000000000, -0.000000000000000000, -0.000000000000000000 ) ) ;
#41071=ORIENTED_EDGE ( 'NONE', *, *, #48189, .T. ) ;
#41073=ORIENTED_EDGE ( 'NONE', *, *, #13650, .F. ) ;
#41077=DIRECTION ( 'NONE',  ( -1.000000000000000000, 0.000000000000000000, 0.000000000000000000 ) ) ;
#41083=ORIENTED_EDGE ( 'NONE', *, *, #25875, .T. ) ;
#41084=CARTESIAN_POINT ( 'NONE',  ( -165.6708471809677974, 1.750000000000009548, 39.79316129108089228 ) ) ;
#41091=ORIENTED_EDGE ( 'NONE', *, *, #30649, .F. ) ;
#41094=( BOUNDED_CURVE ( )  B_SPLINE_CURVE ( 3, ( #17049, #47803, #32705, #28351 ),
 .UNSPECIFIED., .F., .F. ) 
 B_SPLINE_CURVE_WITH_KNOTS ( ( 4, 4 ),
 ( 3.141592653589793116, 4.712388980384689674 ),
 .UNSPECIFIED. ) 
 CURVE ( )  GEOMETRIC_REPRESENTATION_ITEM ( )  RATIONAL_B_SPLINE_CURVE ( ( 1.000000000000000000, 0.8047378541243649375, 0.8047378541243649375, 1.000000000000000000 ) ) 
 REPRESENTATION_ITEM ( '' )  );
#41098=CARTESIAN_POINT ( 'NONE',  ( 153.3040265531850537, -1.750000000000010658, 80.81828755692798438 ) ) ;
#41103=CYLINDRICAL_SURFACE ( 'NONE', #47834, 1.750000000000001554 ) ;
#41104=CARTESIAN_POINT ( 'NONE',  ( 115.0540265531850395, -1.025126265847081886, 39.06828755692799149 ) ) ;
#41106=ORIENTED_EDGE ( 'NONE', *, *, #21797, .T. ) ;
#41113=CARTESIAN_POINT ( 'NONE',  ( 111.5540265531850679, 0.000000000000000000, 42.56828755692795596 ) ) ;
#41118=CARTESIAN_POINT ( 'NONE',  ( 210.0000000000000568, 0.000000000000000000, -79.18171244307201562 ) ) ;
#41120=CARTESIAN_POINT ( 'NONE',  ( -126.6959734468149321, -1.749999999999996891, -159.1817124430720298 ) ) ;
#41121=ORIENTED_EDGE ( 'NONE', *, *, #41265, .F. ) ;
#41124=CARTESIAN_POINT ( 'NONE',  ( -6.695973446814940111, 0.000000000000000000, 165.0000000000000000 ) ) ;
#41126=ORIENTED_EDGE ( 'NONE', *, *, #7416, .T. ) ;
#41127=DIRECTION ( 'NONE',  ( -1.000000000000000000, 0.000000000000000000, 0.000000000000000000 ) ) ;
#41128=ORIENTED_EDGE ( 'NONE', *, *, #15627, .F. ) ;
#41129=EDGE_CURVE ( 'NONE', #23318, #35686, #45557, .T. ) ;
#41130=DIRECTION ( 'NONE',  ( -1.000000000000000000, -0.000000000000000000, -0.000000000000000000 ) ) ;
#41139=ORIENTED_EDGE ( 'NONE', *, *, #26331, .T. ) ;
#41143=( BOUNDED_CURVE ( )  B_SPLINE_CURVE ( 3, ( #33549, #17872, #44809, #48883 ),
 .UNSPECIFIED., .F., .F. ) 
 B_SPLINE_CURVE_WITH_KNOTS ( ( 4, 4 ),
 ( 0.000000000000000000, 1.570796326794896558 ),
 .UNSPECIFIED. ) 
 CURVE ( )  GEOMETRIC_REPRESENTATION_ITEM ( )  RATIONAL_B_SPLINE_CURVE ( ( 1.000000000000000000, 0.8047378541243649375, 0.8047378541243649375, 1.000000000000000000 ) ) 
 REPRESENTATION_ITEM ( '' )  );
#41144=EDGE_LOOP ( 'NONE', ( #24281, #4429, #5649, #38637, #16864 ) ) ;
#41145=VERTEX_POINT ( 'NONE', #37412 ) ;
#41149=CARTESIAN_POINT ( 'NONE',  ( -84.94597344681494633, 2.143131898507880377E-16, 42.56828755692798438 ) ) ;
#41151=VERTEX_POINT ( 'NONE', #14276 ) ;
#41152=( BOUNDED_CURVE ( )  B_SPLINE_CURVE ( 3, ( #9270, #13108, #28271, #43905 ),
 .UNSPECIFIED., .F., .F. ) 
 B_SPLINE_CURVE_WITH_KNOTS ( ( 4, 4 ),
 ( 0.000000000000000000, 1.570796326794896558 ),
 .UNSPECIFIED. ) 
 CURVE ( )  GEOMETRIC_REPRESENTATION_ITEM ( )  RATIONAL_B_SPLINE_CURVE ( ( 1.000000000000000000, 0.8047378541243649375, 0.8047378541243649375, 1.000000000000000000 ) ) 
 REPRESENTATION_ITEM ( '' )  );
#41154=CARTESIAN_POINT ( 'NONE',  ( -7.721099712662037540, -1.750000000000023315, -40.20683870891912903 ) ) ;
#41160=DIRECTION ( 'NONE',  ( -0.000000000000000000, -0.000000000000000000, -1.000000000000000000 ) ) ;
#41164=CARTESIAN_POINT ( 'NONE',  ( 210.0000000000000568, 0.000000000000000000, 2.568287556927987048 ) ) ;
#41165=LINE ( 'NONE', #5517, #9187 ) ;
#41166=VERTEX_POINT ( 'NONE', #33304 ) ;
#41169=DIRECTION ( 'NONE',  ( -0.000000000000000000, -0.000000000000000000, -1.000000000000000000 ) ) ;
#41172=CARTESIAN_POINT ( 'NONE',  ( -165.6708471809677974, -1.750000000000010436, 79.79316129108087807 ) ) ;
#41173=ORIENTED_EDGE ( 'NONE', *, *, #4553, .T. ) ;
#41174=CARTESIAN_POINT ( 'NONE',  ( -208.4459734468148611, -1.025126265847089657, -80.93171244307201562 ) ) ;
#41178=EDGE_CURVE ( 'NONE', #21466, #20141, #29942, .T. ) ;
#41180=CARTESIAN_POINT ( 'NONE',  ( 71.55402655318505367, -1.025126265847089879, 122.5682875569280128 ) ) ;
#41182=EDGE_CURVE ( 'NONE', #42453, #46337, #2923, .T. ) ;
#41188=CARTESIAN_POINT ( 'NONE',  ( 31.55402655318503236, 1.025126265847089435, 122.5682875569280128 ) ) ;
#41189=DIRECTION ( 'NONE',  ( -0.000000000000000000, -0.000000000000000000, -1.000000000000000000 ) ) ;
#41190=AXIS2_PLACEMENT_3D ( 'NONE', #19531, #35471, #40070 ) ;
#41195=ORIENTED_EDGE ( 'NONE', *, *, #35570, .F. ) ;
#41198=CARTESIAN_POINT ( 'NONE',  ( -168.4459734468149747, 1.025126265847089213, -37.43171244307202272 ) ) ;
#41200=CARTESIAN_POINT ( 'NONE',  ( 112.2789002873379758, -1.749999999999996891, 119.7931612910809065 ) ) ;
#41201=EDGE_LOOP ( 'NONE', ( #40668, #50006, #32755, #38871, #6645, #33225 ) ) ;
#41204=CYLINDRICAL_SURFACE ( 'NONE', #50264, 1.749999999999973799 ) ;
#41209=ADVANCED_FACE ( 'NONE', ( #30447 ), #46312, .F. ) ;
#41211=FACE_OUTER_BOUND ( 'NONE', #10279, .T. ) ;
#41212=DIRECTION ( 'NONE',  ( 1.000000000000000000, 0.000000000000000000, 0.000000000000000000 ) ) ;
#41215=EDGE_CURVE ( 'NONE', #28163, #35332, #10131, .T. ) ;
#41219=VERTEX_POINT ( 'NONE', #46556 ) ;
#41221=DIRECTION ( 'NONE',  ( 0.000000000000000000, 0.000000000000000000, 1.000000000000000000 ) ) ;
#41223=CARTESIAN_POINT ( 'NONE',  ( 111.5540265531850537, -1.025126265847082108, 122.5682875569279702 ) ) ;
#41224=EDGE_CURVE ( 'NONE', #40403, #26183, #45161, .T. ) ;
#41225=CARTESIAN_POINT ( 'NONE',  ( 115.0540265531850395, 2.143131898507847836E-16, -37.43171244307205825 ) ) ;
#41233=CARTESIAN_POINT ( 'NONE',  ( -47.72109971266203132, -1.750000000000009548, -0.2068387089191121020 ) ) ;
#41235=CARTESIAN_POINT ( 'NONE',  ( -164.9459734468149463, -1.025126265847089213, -37.43171244307202272 ) ) ;
#41236=CARTESIAN_POINT ( 'NONE',  ( 210.0000000000000568, 0.000000000000000000, -79.18171244307201562 ) ) ;
#41237=CARTESIAN_POINT ( 'NONE',  ( 210.0000000000000568, 0.000000000000000000, 80.81828755692798438 ) ) ;
#41242=VECTOR ( 'NONE', #6655, 1000.000000000000000 ) ;
#41243=CARTESIAN_POINT ( 'NONE',  ( -166.6959734468149463, -1.750000000000010658, -79.18171244307201562 ) ) ;
#41245=CYLINDRICAL_SURFACE ( 'NONE', #35203, 1.750000000000001554 ) ;
#41246=FACE_OUTER_BOUND ( 'NONE', #25513, .T. ) ;
#41247=CARTESIAN_POINT ( 'NONE',  ( -4.945973446814903696, 2.143131898507912917E-16, 39.06828755692792754 ) ) ;
#41255=CARTESIAN_POINT ( 'NONE',  ( -125.6708471809678542, 1.749999999999996669, 1.843413822775057609 ) ) ;
#41261=ORIENTED_EDGE ( 'NONE', *, *, #50266, .T. ) ;
#41265=EDGE_CURVE ( 'NONE', #45334, #37195, #1001, .T. ) ;
#41270=VERTEX_POINT ( 'NONE', #47321 ) ;
#41273=CARTESIAN_POINT ( 'NONE',  ( -44.94597344681493922, 2.143131898507880377E-16, -77.43171244307198720 ) ) ;
#41275=AXIS2_PLACEMENT_3D ( 'NONE', #1810, #17453, #5644 ) ;
#41280=CARTESIAN_POINT ( 'NONE',  ( -48.44597344681495343, 0.000000000000000000, -120.9317124430720725 ) ) ;
#41284=VERTEX_POINT ( 'NONE', #32486 ) ;
#41293=EDGE_CURVE ( 'NONE', #34716, #48470, #24020, .T. ) ;
#41294=( BOUNDED_CURVE ( )  B_SPLINE_CURVE ( 3, ( #29882, #45502, #26040, #45745 ),
 .UNSPECIFIED., .F., .F. ) 
 B_SPLINE_CURVE_WITH_KNOTS ( ( 4, 4 ),
 ( 4.712388980384689674, 6.283185307179586232 ),
 .UNSPECIFIED. ) 
 CURVE ( )  GEOMETRIC_REPRESENTATION_ITEM ( )  RATIONAL_B_SPLINE_CURVE ( ( 1.000000000000000000, 0.8047378541243649375, 0.8047378541243649375, 1.000000000000000000 ) ) 
 REPRESENTATION_ITEM ( '' )  );
#41295=FACE_OUTER_BOUND ( 'NONE', #26612, .T. ) ;
#41301=( BOUNDED_CURVE ( )  B_SPLINE_CURVE ( 3, ( #43565, #34614, #39231, #19191 ),
 .UNSPECIFIED., .F., .F. ) 
 B_SPLINE_CURVE_WITH_KNOTS ( ( 4, 4 ),
 ( 0.000000000000000000, 1.570796326794896558 ),
 .UNSPECIFIED. ) 
 CURVE ( )  GEOMETRIC_REPRESENTATION_ITEM ( )  RATIONAL_B_SPLINE_CURVE ( ( 1.000000000000000000, 0.8047378541243649375, 0.8047378541243649375, 1.000000000000000000 ) ) 
 REPRESENTATION_ITEM ( '' )  );
#41309=CIRCLE ( 'NONE', #19172, 1.750000000000001554 ) ;
#41316=( BOUNDED_CURVE ( )  B_SPLINE_CURVE ( 3, ( #23642, #15951, #32360, #19787 ),
 .UNSPECIFIED., .F., .F. ) 
 B_SPLINE_CURVE_WITH_KNOTS ( ( 4, 4 ),
 ( 0.000000000000000000, 1.570796326794896558 ),
 .UNSPECIFIED. ) 
 CURVE ( )  GEOMETRIC_REPRESENTATION_ITEM ( )  RATIONAL_B_SPLINE_CURVE ( ( 1.000000000000000000, 0.8047378541243649375, 0.8047378541243649375, 1.000000000000000000 ) ) 
 REPRESENTATION_ITEM ( '' )  );
#41321=CYLINDRICAL_SURFACE ( 'NONE', #9234, 1.750000000000001554 ) ;
#41328=CARTESIAN_POINT ( 'NONE',  ( -6.695973446814940111, 1.750000000000024203, -79.18171244307201562 ) ) ;
#41329=ORIENTED_EDGE ( 'NONE', *, *, #16314, .T. ) ;
#41331=DIRECTION ( 'NONE',  ( -1.000000000000000000, 0.000000000000000000, 0.000000000000000000 ) ) ;
#41333=LINE ( 'NONE', #29531, #45339 ) ;
#41335=CARTESIAN_POINT ( 'NONE',  ( -164.9459734468149463, 2.143131898507880377E-16, -77.43171244307204404 ) ) ;
#41336=DIRECTION ( 'NONE',  ( -1.000000000000000000, -0.000000000000000000, -0.000000000000000000 ) ) ;
#41341=ADVANCED_FACE ( 'NONE', ( #40173 ), #5009, .T. ) ;
#41348=ADVANCED_FACE ( 'NONE', ( #25270 ), #49326, .T. ) ;
#41349=DIRECTION ( 'NONE',  ( 0.000000000000000000, 0.000000000000000000, 1.000000000000000000 ) ) ;
#41350=VERTEX_POINT ( 'NONE', #21410 ) ;
#41353=FACE_OUTER_BOUND ( 'NONE', #16257, .T. ) ;
#41355=CARTESIAN_POINT ( 'NONE',  ( -48.44597344681495343, 0.000000000000000000, -157.4317124430720014 ) ) ;
#41356=CARTESIAN_POINT ( 'NONE',  ( -204.9459734468149747, 0.000000000000000000, 162.5682875569279702 ) ) ;
#41357=EDGE_CURVE ( 'NONE', #3215, #5399, #6288, .T. ) ;
#41358=DIRECTION ( 'NONE',  ( -0.000000000000000000, -0.000000000000000000, -1.000000000000000000 ) ) ;
#41359=ORIENTED_EDGE ( 'NONE', *, *, #32456, .F. ) ;
#41364=DIRECTION ( 'NONE',  ( -1.000000000000000000, 0.000000000000000000, 0.000000000000000000 ) ) ;
#41369=ORIENTED_EDGE ( 'NONE', *, *, #14430, .T. ) ;
#41370=CARTESIAN_POINT ( 'NONE',  ( -126.6959734468149321, -1.749999999999996891, 160.8182875569279702 ) ) ;
#41372=CARTESIAN_POINT ( 'NONE',  ( 111.5540265531850679, 0.000000000000000000, 165.0000000000000000 ) ) ;
#41373=AXIS2_PLACEMENT_3D ( 'NONE', #32254, #32008, #20693 ) ;
#41377=CARTESIAN_POINT ( 'NONE',  ( -128.4459734468149179, 0.000000000000000000, -0.9317124430719969652 ) ) ;
#41378=ORIENTED_EDGE ( 'NONE', *, *, #3558, .F. ) ;
#41379=CARTESIAN_POINT ( 'NONE',  ( 75.05402655318509630, 2.143131898507880377E-16, 39.06828755692795596 ) ) ;
#41381=CARTESIAN_POINT ( 'NONE',  ( 31.55402655318503236, -1.025126265847089435, -157.4317124430720582 ) ) ;
#41382=FACE_OUTER_BOUND ( 'NONE', #7151, .T. ) ;
#41385=ORIENTED_EDGE ( 'NONE', *, *, #34963, .F. ) ;
#41387=EDGE_CURVE ( 'NONE', #33331, #13763, #15980, .T. ) ;
#41395=CARTESIAN_POINT ( 'NONE',  ( 210.0000000000000568, 0.000000000000000000, -157.4317124430720298 ) ) ;
#41396=( BOUNDED_CURVE ( )  B_SPLINE_CURVE ( 3, ( #21716, #21214, #26077, #26337 ),
 .UNSPECIFIED., .F., .F. ) 
 B_SPLINE_CURVE_WITH_KNOTS ( ( 4, 4 ),
 ( 0.000000000000000000, 1.570796326794896558 ),
 .UNSPECIFIED. ) 
 CURVE ( )  GEOMETRIC_REPRESENTATION_ITEM ( )  RATIONAL_B_SPLINE_CURVE ( ( 1.000000000000000000, 0.8047378541243649375, 0.8047378541243649375, 1.000000000000000000 ) ) 
 REPRESENTATION_ITEM ( '' )  );
#41398=DIRECTION ( 'NONE',  ( -1.000000000000000000, -0.000000000000000000, -0.000000000000000000 ) ) ;
#41399=EDGE_LOOP ( 'NONE', ( #48059, #21774, #36433, #43750, #37078, #43245 ) ) ;
#41400=ORIENTED_EDGE ( 'NONE', *, *, #19048, .T. ) ;
#41401=CARTESIAN_POINT ( 'NONE',  ( -126.6959734468149321, 0.000000000000000000, -165.0000000000000000 ) ) ;
#41404=ORIENTED_EDGE ( 'NONE', *, *, #43268, .F. ) ;
#41405=VERTEX_POINT ( 'NONE', #37851 ) ;
#41406=CARTESIAN_POINT ( 'NONE',  ( 35.05402655318504657, 2.143131898507880377E-16, -120.9317124430720725 ) ) ;
#41407=CARTESIAN_POINT ( 'NONE',  ( -85.67084718096784002, -1.750000000000009548, 41.84341382277508359 ) ) ;
#41409=EDGE_LOOP ( 'NONE', ( #30159, #40402 ) ) ;
#41413=CARTESIAN_POINT ( 'NONE',  ( -126.6959734468149321, -1.749999999999997113, -39.18171244307202983 ) ) ;
#41419=ORIENTED_EDGE ( 'NONE', *, *, #39050, .F. ) ;
#41420=EDGE_CURVE ( 'NONE', #26020, #559, #44748, .T. ) ;
#41421=CARTESIAN_POINT ( 'NONE',  ( -8.445973446814976526, 0.000000000000000000, 122.5682875569279986 ) ) ;
#41425=ORIENTED_EDGE ( 'NONE', *, *, #9613, .F. ) ;
#41428=ORIENTED_EDGE ( 'NONE', *, *, #42554, .T. ) ;
#41429=CARTESIAN_POINT ( 'NONE',  ( 31.55402655318503236, -1.025126265847089213, 159.0682875569279418 ) ) ;
#41430=CARTESIAN_POINT ( 'NONE',  ( 114.3291528190321173, -1.749999999999996669, -38.15658617722495194 ) ) ;
#41432=DIRECTION ( 'NONE',  ( 0.000000000000000000, 0.000000000000000000, 1.000000000000000000 ) ) ;
#41439=VECTOR ( 'NONE', #46028, 1000.000000000000000 ) ;
#41441=CARTESIAN_POINT ( 'NONE',  ( -206.6959734468149463, 1.750000000000010658, -119.1817124430720440 ) ) ;
#41444=VECTOR ( 'NONE', #42558, 1000.000000000000000 ) ;
#41446=EDGE_CURVE ( 'NONE', #26878, #23932, #13465, .T. ) ;
#41447=VERTEX_POINT ( 'NONE', #9622 ) ;
#41449=( BOUNDED_CURVE ( )  B_SPLINE_CURVE ( 3, ( #41149, #5999, #41407, #6272 ),
 .UNSPECIFIED., .F., .F. ) 
 B_SPLINE_CURVE_WITH_KNOTS ( ( 4, 4 ),
 ( 3.141592653589793116, 4.712388980384689674 ),
 .UNSPECIFIED. ) 
 CURVE ( )  GEOMETRIC_REPRESENTATION_ITEM ( )  RATIONAL_B_SPLINE_CURVE ( ( 1.000000000000000000, 0.8047378541243649375, 0.8047378541243649375, 1.000000000000000000 ) ) 
 REPRESENTATION_ITEM ( '' )  );
#41454=CARTESIAN_POINT ( 'NONE',  ( -124.9459734468149463, 2.143131898507847836E-16, 42.56828755692795596 ) ) ;
#41456=( BOUNDED_CURVE ( )  B_SPLINE_CURVE ( 3, ( #50081, #2918, #26539, #34766 ),
 .UNSPECIFIED., .F., .F. ) 
 B_SPLINE_CURVE_WITH_KNOTS ( ( 4, 4 ),
 ( 3.141592653589793116, 4.712388980384689674 ),
 .UNSPECIFIED. ) 
 CURVE ( )  GEOMETRIC_REPRESENTATION_ITEM ( )  RATIONAL_B_SPLINE_CURVE ( ( 1.000000000000000000, 0.8047378541243649375, 0.8047378541243649375, 1.000000000000000000 ) ) 
 REPRESENTATION_ITEM ( '' )  );
#41461=AXIS2_PLACEMENT_3D ( 'NONE', #41401, #26265, #49048 ) ;
#41465=FACE_OUTER_BOUND ( 'NONE', #7789, .T. ) ;
#41466=ORIENTED_EDGE ( 'NONE', *, *, #46511, .F. ) ;
#41475=CARTESIAN_POINT ( 'NONE',  ( 115.0540265531850395, 2.143131898507847836E-16, 39.06828755692798438 ) ) ;
#41480=CARTESIAN_POINT ( 'NONE',  ( 155.0540265531850537, -1.025126265847088991, 159.0682875569279418 ) ) ;
#41487=CARTESIAN_POINT ( 'NONE',  ( 210.0000000000000568, 0.000000000000000000, -157.4317124430720298 ) ) ;
#41488=EDGE_CURVE ( 'NONE', #1022, #47399, #8200, .T. ) ;
#41491=CARTESIAN_POINT ( 'NONE',  ( -88.44597344681494633, 1.025126265847088991, -157.4317124430720582 ) ) ;
#41492=AXIS2_PLACEMENT_3D ( 'NONE', #13595, #29250, #13087 ) ;
#41498=ADVANCED_FACE ( 'NONE', ( #30912 ), #7041, .T. ) ;
#41503=CARTESIAN_POINT ( 'NONE',  ( 151.5540265531850537, 0.000000000000000000, 165.0000000000000000 ) ) ;
#41504=ADVANCED_FACE ( 'NONE', ( #11905 ), #15252, .T. ) ;
#41508=EDGE_LOOP ( 'NONE', ( #23950, #4288, #14708, #45954, #7413 ) ) ;
#41510=ADVANCED_FACE ( 'NONE', ( #27036 ), #42174, .T. ) ;
#41512=CARTESIAN_POINT ( 'NONE',  ( 154.3291528190321458, 1.750000000000009548, -38.15658617722494483 ) ) ;
#41517=FACE_OUTER_BOUND ( 'NONE', #32527, .T. ) ;
#41519=EDGE_LOOP ( 'NONE', ( #10345, #8350, #49801, #34669, #3555, #46502 ) ) ;
#41521=EDGE_LOOP ( 'NONE', ( #8758, #25562, #14923, #20623, #6781, #24722 ) ) ;
#41523=ORIENTED_EDGE ( 'NONE', *, *, #46982, .F. ) ;
#41531=AXIS2_PLACEMENT_3D ( 'NONE', #5047, #32771, #13942 ) ;
#41533=FACE_OUTER_BOUND ( 'NONE', #20825, .T. ) ;
#41535=EDGE_CURVE ( 'NONE', #37507, #15868, #11789, .T. ) ;
#41539=ORIENTED_EDGE ( 'NONE', *, *, #4904, .T. ) ;
#41541=VERTEX_POINT ( 'NONE', #18815 ) ;
#41544=FACE_OUTER_BOUND ( 'NONE', #18990, .T. ) ;
#41547=CYLINDRICAL_SURFACE ( 'NONE', #36435, 1.750000000000001554 ) ;
#41550=DIRECTION ( 'NONE',  ( -0.000000000000000000, -0.000000000000000000, -1.000000000000000000 ) ) ;
#41552=ORIENTED_EDGE ( 'NONE', *, *, #21144, .T. ) ;
#41554=CARTESIAN_POINT ( 'NONE',  ( -125.6708471809678542, -1.749999999999997113, 79.79316129108087807 ) ) ;
#41556=EDGE_CURVE ( 'NONE', #29610, #11124, #9829, .T. ) ;
#41563=ORIENTED_EDGE ( 'NONE', *, *, #5835, .T. ) ;
#41566=FACE_OUTER_BOUND ( 'NONE', #37388, .T. ) ;
#41567=DIRECTION ( 'NONE',  ( -1.000000000000000000, -0.000000000000000000, -0.000000000000000000 ) ) ;
#41568=CARTESIAN_POINT ( 'NONE',  ( 111.5540265531850679, 0.000000000000000000, 82.56828755692797017 ) ) ;
#41570=ORIENTED_EDGE ( 'NONE', *, *, #49121, .F. ) ;
#41578=CARTESIAN_POINT ( 'NONE',  ( 193.3040265531851105, -1.750000000000010214, 40.81828755692798438 ) ) ;
#41580=CARTESIAN_POINT ( 'NONE',  ( 73.30402655318508209, 1.750000000000010658, 120.8182875569279702 ) ) ;
#41581=ORIENTED_EDGE ( 'NONE', *, *, #37753, .T. ) ;
#41582=EDGE_CURVE ( 'NONE', #18090, #38070, #17028, .T. ) ;
#41586=CARTESIAN_POINT ( 'NONE',  ( 71.55402655318505367, -1.025126265847089657, -37.43171244307202272 ) ) ;
#41587=CARTESIAN_POINT ( 'NONE',  ( -8.445973446814976526, 0.000000000000000000, 42.56828755692802702 ) ) ;
#41592=CARTESIAN_POINT ( 'NONE',  ( 35.05402655318504657, 2.143131898507880377E-16, 122.5682875569279702 ) ) ;
#41593=( BOUNDED_CURVE ( )  B_SPLINE_CURVE ( 3, ( #27843, #8594, #47036, #39146 ),
 .UNSPECIFIED., .F., .F. ) 
 B_SPLINE_CURVE_WITH_KNOTS ( ( 4, 4 ),
 ( 3.141592653589793116, 4.712388980384689674 ),
 .UNSPECIFIED. ) 
 CURVE ( )  GEOMETRIC_REPRESENTATION_ITEM ( )  RATIONAL_B_SPLINE_CURVE ( ( 1.000000000000000000, 0.8047378541243649375, 0.8047378541243649375, 1.000000000000000000 ) ) 
 REPRESENTATION_ITEM ( '' )  );
#41601=( BOUNDED_CURVE ( )  B_SPLINE_CURVE ( 3, ( #8132, #3486, #35092, #23249 ),
 .UNSPECIFIED., .F., .F. ) 
 B_SPLINE_CURVE_WITH_KNOTS ( ( 4, 4 ),
 ( 0.000000000000000000, 1.570796326794896558 ),
 .UNSPECIFIED. ) 
 CURVE ( )  GEOMETRIC_REPRESENTATION_ITEM ( )  RATIONAL_B_SPLINE_CURVE ( ( 1.000000000000000000, 0.8047378541243649375, 0.8047378541243649375, 1.000000000000000000 ) ) 
 REPRESENTATION_ITEM ( '' )  );
#41605=CARTESIAN_POINT ( 'NONE',  ( -125.6708471809678542, -1.749999999999996669, -118.1565861772249661 ) ) ;
#41606=CYLINDRICAL_SURFACE ( 'NONE', #46221, 1.750000000000015543 ) ;
#41607=CARTESIAN_POINT ( 'NONE',  ( 210.0000000000000568, 2.143131898507880377E-16, -160.9317124430720298 ) ) ;
#41608=CARTESIAN_POINT ( 'NONE',  ( 35.05402655318504657, 2.143131898507880377E-16, 82.56828755692798438 ) ) ;
#41609=ORIENTED_EDGE ( 'NONE', *, *, #27518, .F. ) ;
#41610=ORIENTED_EDGE ( 'NONE', *, *, #45870, .T. ) ;
#41613=EDGE_CURVE ( 'NONE', #7107, #40469, #24469, .T. ) ;
#41614=( BOUNDED_CURVE ( )  B_SPLINE_CURVE ( 3, ( #10617, #21407, #6010, #9864 ),
 .UNSPECIFIED., .F., .F. ) 
 B_SPLINE_CURVE_WITH_KNOTS ( ( 4, 4 ),
 ( 3.141592653589793116, 4.712388980384689674 ),
 .UNSPECIFIED. ) 
 CURVE ( )  GEOMETRIC_REPRESENTATION_ITEM ( )  RATIONAL_B_SPLINE_CURVE ( ( 1.000000000000000000, 0.8047378541243649375, 0.8047378541243649375, 1.000000000000000000 ) ) 
 REPRESENTATION_ITEM ( '' )  );
#41622=LINE ( 'NONE', #41372, #16840 ) ;
#41623=AXIS2_PLACEMENT_3D ( 'NONE', #45184, #10069, #25729 ) ;
#41624=CARTESIAN_POINT ( 'NONE',  ( 151.5540265531850537, 2.143131898507880377E-16, -160.9317124430720298 ) ) ;
#41626=DIRECTION ( 'NONE',  ( -0.000000000000000000, -0.000000000000000000, -1.000000000000000000 ) ) ;
#41633=EDGE_CURVE ( 'NONE', #43082, #10600, #43687, .T. ) ;
#41636=ORIENTED_EDGE ( 'NONE', *, *, #32456, .T. ) ;
#41637=FACE_OUTER_BOUND ( 'NONE', #46707, .T. ) ;
#41641=DIRECTION ( 'NONE',  ( 0.000000000000000000, 0.000000000000000000, 1.000000000000000000 ) ) ;
#41642=ORIENTED_EDGE ( 'NONE', *, *, #8363, .T. ) ;
#41644=EDGE_CURVE ( 'NONE', #29991, #38466, #6247, .T. ) ;
#41647=CARTESIAN_POINT ( 'NONE',  ( -44.94597344681493922, 2.143131898507880377E-16, 39.06828755692798438 ) ) ;
#41649=CYLINDRICAL_SURFACE ( 'NONE', #5358, 1.750000000000008438 ) ;
#41651=ORIENTED_EDGE ( 'NONE', *, *, #30342, .T. ) ;
#41652=VERTEX_POINT ( 'NONE', #9802 ) ;
#41657=VERTEX_POINT ( 'NONE', #25213 ) ;
#41658=CARTESIAN_POINT ( 'NONE',  ( 33.30402655318503946, 1.750000000000010658, -119.1817124430720440 ) ) ;
#41660=CARTESIAN_POINT ( 'NONE',  ( 111.5540265531850679, 0.000000000000000000, 79.06828755692798438 ) ) ;
#41661=( BOUNDED_CURVE ( )  B_SPLINE_CURVE ( 3, ( #7495, #23125, #23894, #19519 ),
 .UNSPECIFIED., .F., .F. ) 
 B_SPLINE_CURVE_WITH_KNOTS ( ( 4, 4 ),
 ( 4.712388980384689674, 6.283185307179586232 ),
 .UNSPECIFIED. ) 
 CURVE ( )  GEOMETRIC_REPRESENTATION_ITEM ( )  RATIONAL_B_SPLINE_CURVE ( ( 1.000000000000000000, 0.8047378541243649375, 0.8047378541243649375, 1.000000000000000000 ) ) 
 REPRESENTATION_ITEM ( '' )  );
#41663=FACE_OUTER_BOUND ( 'NONE', #11291, .T. ) ;
#41664=ORIENTED_EDGE ( 'NONE', *, *, #40264, .F. ) ;
#41666=CARTESIAN_POINT ( 'NONE',  ( -127.7210997126620242, -1.749999999999996669, -38.15658617722495194 ) ) ;
#41670=CARTESIAN_POINT ( 'NONE',  ( 113.3040265531850537, -1.749999999999996891, 160.8182875569279702 ) ) ;
#41671=CARTESIAN_POINT ( 'NONE',  ( 193.3040265531851105, -1.750000000000009992, 0.8182875569279768335 ) ) ;
#41672=ORIENTED_EDGE ( 'NONE', *, *, #15529, .F. ) ;
#41679=CYLINDRICAL_SURFACE ( 'NONE', #22770, 1.750000000000015543 ) ;
#41680=CARTESIAN_POINT ( 'NONE',  ( 115.0540265531850395, -1.025126265847081886, -80.93171244307201562 ) ) ;
#41682=DIRECTION ( 'NONE',  ( 0.000000000000000000, 0.000000000000000000, 1.000000000000000000 ) ) ;
#41685=DIRECTION ( 'NONE',  ( -1.000000000000000000, -0.000000000000000000, -0.000000000000000000 ) ) ;
#41690=FACE_OUTER_BOUND ( 'NONE', #18848, .T. ) ;
#41691=CARTESIAN_POINT ( 'NONE',  ( 210.0000000000000568, 0.000000000000000000, 160.8182875569279702 ) ) ;
#41693=( BOUNDED_CURVE ( )  B_SPLINE_CURVE ( 3, ( #49512, #6706, #19002, #7486 ),
 .UNSPECIFIED., .F., .F. ) 
 B_SPLINE_CURVE_WITH_KNOTS ( ( 4, 4 ),
 ( 4.712388980384689674, 6.283185307179586232 ),
 .UNSPECIFIED. ) 
 CURVE ( )  GEOMETRIC_REPRESENTATION_ITEM ( )  RATIONAL_B_SPLINE_CURVE ( ( 1.000000000000000000, 0.8047378541243649375, 0.8047378541243649375, 1.000000000000000000 ) ) 
 REPRESENTATION_ITEM ( '' )  );
#41698=AXIS2_PLACEMENT_3D ( 'NONE', #555, #28247, #43880 ) ;
#41702=EDGE_LOOP ( 'NONE', ( #37831, #13536, #7599, #29863, #3443, #21039 ) ) ;
#41710=ORIENTED_EDGE ( 'NONE', *, *, #42134, .T. ) ;
#41716=DIRECTION ( 'NONE',  ( -1.000000000000000000, 0.000000000000000000, 0.000000000000000000 ) ) ;
#41717=CARTESIAN_POINT ( 'NONE',  ( 193.3040265531851105, -1.750000000000009992, 0.8182875569279768335 ) ) ;
#41719=VERTEX_POINT ( 'NONE', #44687 ) ;
#41723=CARTESIAN_POINT ( 'NONE',  ( -46.69597344681494633, 1.750000000000010658, 120.8182875569279702 ) ) ;
#41728=EDGE_LOOP ( 'NONE', ( #18287, #45250, #49019, #22951, #21334, #11956 ) ) ;
#41730=DIRECTION ( 'NONE',  ( 1.000000000000000000, 0.000000000000000000, -0.000000000000000000 ) ) ;
#41733=CARTESIAN_POINT ( 'NONE',  ( -5.670847180967843570, -1.750000000000023315, -40.20683870891912903 ) ) ;
#41741=CARTESIAN_POINT ( 'NONE',  ( 210.0000000000000568, 2.143131898507881116E-16, -40.93171244307203693 ) ) ;
#41742=ORIENTED_EDGE ( 'NONE', *, *, #38380, .T. ) ;
#41743=LINE ( 'NONE', #22247, #443 ) ;
#41744=CARTESIAN_POINT ( 'NONE',  ( -84.94597344681493212, 1.025126265847089657, 42.56828755692799149 ) ) ;
#41746=CYLINDRICAL_SURFACE ( 'NONE', #18679, 1.750000000000015543 ) ;
#41747=( BOUNDED_CURVE ( )  B_SPLINE_CURVE ( 3, ( #13966, #18313, #14480, #14734 ),
 .UNSPECIFIED., .F., .F. ) 
 B_SPLINE_CURVE_WITH_KNOTS ( ( 4, 4 ),
 ( 4.712388980384689674, 6.283185307179586232 ),
 .UNSPECIFIED. ) 
 CURVE ( )  GEOMETRIC_REPRESENTATION_ITEM ( )  RATIONAL_B_SPLINE_CURVE ( ( 1.000000000000000000, 0.8047378541243649375, 0.8047378541243649375, 1.000000000000000000 ) ) 
 REPRESENTATION_ITEM ( '' )  );
#41751=( BOUNDED_CURVE ( )  B_SPLINE_CURVE ( 3, ( #14226, #13974, #10636, #29384 ),
 .UNSPECIFIED., .F., .F. ) 
 B_SPLINE_CURVE_WITH_KNOTS ( ( 4, 4 ),
 ( 3.141592653589793116, 4.712388980384689674 ),
 .UNSPECIFIED. ) 
 CURVE ( )  GEOMETRIC_REPRESENTATION_ITEM ( )  RATIONAL_B_SPLINE_CURVE ( ( 1.000000000000000000, 0.8047378541243649375, 0.8047378541243649375, 1.000000000000000000 ) ) 
 REPRESENTATION_ITEM ( '' )  );
#41757=ORIENTED_EDGE ( 'NONE', *, *, #45434, .F. ) ;
#41761=FACE_OUTER_BOUND ( 'NONE', #39590, .T. ) ;
#41763=ORIENTED_EDGE ( 'NONE', *, *, #27720, .T. ) ;
#41764=CARTESIAN_POINT ( 'NONE',  ( -8.445973446814976526, 0.000000000000000000, 165.0000000000000000 ) ) ;
#41771=EDGE_CURVE ( 'NONE', #17646, #24955, #32934, .T. ) ;
#41772=CARTESIAN_POINT ( 'NONE',  ( 210.0000000000000568, 2.143131898507881116E-16, 39.06828755692797728 ) ) ;
#41773=CARTESIAN_POINT ( 'NONE',  ( 33.30402655318503946, 0.000000000000000000, 165.0000000000000000 ) ) ;
#41774=ORIENTED_EDGE ( 'NONE', *, *, #36242, .T. ) ;
#41775=EDGE_CURVE ( 'NONE', #46337, #19548, #32770, .T. ) ;
#41777=CARTESIAN_POINT ( 'NONE',  ( 71.55402655318505367, 0.000000000000000000, 119.0682875569279560 ) ) ;
#41782=VERTEX_POINT ( 'NONE', #40620 ) ;
#41786=CARTESIAN_POINT ( 'NONE',  ( -206.6959734468149463, -1.750000000000010658, -79.18171244307201562 ) ) ;
#41791=CARTESIAN_POINT ( 'NONE',  ( 73.30402655318508209, -1.750000000000010658, 120.8182875569279702 ) ) ;
#41795=CIRCLE ( 'NONE', #36108, 1.750000000000036193 ) ;
#41796=CARTESIAN_POINT ( 'NONE',  ( -5.670847180967843570, 1.750000000000023537, 81.84341382277507648 ) ) ;
#41797=VECTOR ( 'NONE', #17576, 1000.000000000000000 ) ;
#41798=EDGE_LOOP ( 'NONE', ( #16956, #11295, #39198, #25326, #18267, #11168 ) ) ;
#41806=CARTESIAN_POINT ( 'NONE',  ( 73.30402655318508209, 1.750000000000010658, -79.18171244307201562 ) ) ;
#41808=DIRECTION ( 'NONE',  ( -0.000000000000000000, -0.000000000000000000, -1.000000000000000000 ) ) ;
#41809=CARTESIAN_POINT ( 'NONE',  ( 31.55402655318503236, 0.000000000000000000, 165.0000000000000000 ) ) ;
#41817=LINE ( 'NONE', #18203, #9866 ) ;
#41820=CARTESIAN_POINT ( 'NONE',  ( -210.0000000000000568, 2.143131898507876926E-16, -120.9317124430720582 ) ) ;
#41825=CARTESIAN_POINT ( 'NONE',  ( -84.94597344681493212, -1.025126265847089213, -37.43171244307202272 ) ) ;
#41827=CARTESIAN_POINT ( 'NONE',  ( 210.0000000000000568, 0.000000000000000000, 82.56828755692799859 ) ) ;
#41828=VERTEX_POINT ( 'NONE', #20233 ) ;
#41832=VECTOR ( 'NONE', #40206, 1000.000000000000000 ) ;
#41833=AXIS2_PLACEMENT_3D ( 'NONE', #17657, #2255, #38197 ) ;
#41836=CARTESIAN_POINT ( 'NONE',  ( 74.32915281903215998, 1.750000000000010214, -78.15658617722490931 ) ) ;
#41839=CARTESIAN_POINT ( 'NONE',  ( -45.67084718096785423, -1.750000000000009326, 1.843413822775066269 ) ) ;
#41848=DIRECTION ( 'NONE',  ( 0.000000000000000000, 0.000000000000000000, -1.000000000000000000 ) ) ;
#41850=VERTEX_POINT ( 'NONE', #16378 ) ;
#41851=DIRECTION ( 'NONE',  ( 0.000000000000000000, 0.000000000000000000, -1.000000000000000000 ) ) ;
#41853=EDGE_CURVE ( 'NONE', #29317, #22517, #42942, .T. ) ;
#41855=EDGE_CURVE ( 'NONE', #34244, #4629, #21967, .T. ) ;
#41856=CARTESIAN_POINT ( 'NONE',  ( -126.6959734468149321, -1.749999999999997335, -119.1817124430720440 ) ) ;
#41857=CARTESIAN_POINT ( 'NONE',  ( -127.7210997126620242, -1.749999999999996891, -78.15658617722492352 ) ) ;
#41876=DIRECTION ( 'NONE',  ( -1.000000000000000000, -0.000000000000000000, -0.000000000000000000 ) ) ;
#41878=CARTESIAN_POINT ( 'NONE',  ( 73.30402655318508209, -1.750000000000010214, 40.81828755692798438 ) ) ;
#41881=CARTESIAN_POINT ( 'NONE',  ( 31.55402655318503236, 0.000000000000000000, -157.4317124430720014 ) ) ;
#41883=EDGE_CURVE ( 'NONE', #20298, #29366, #31123, .T. ) ;
#41886=EDGE_CURVE ( 'NONE', #45654, #41447, #35659, .T. ) ;
#41887=DIRECTION ( 'NONE',  ( -0.000000000000000000, -0.000000000000000000, -1.000000000000000000 ) ) ;
#41890=CARTESIAN_POINT ( 'NONE',  ( 210.0000000000000568, 2.143131898507890731E-16, -160.9317124430720298 ) ) ;
#41893=( BOUNDED_CURVE ( )  B_SPLINE_CURVE ( 3, ( #14786, #27617, #22734, #50132 ),
 .UNSPECIFIED., .F., .F. ) 
 B_SPLINE_CURVE_WITH_KNOTS ( ( 4, 4 ),
 ( 0.000000000000000000, 1.570796326794896558 ),
 .UNSPECIFIED. ) 
 CURVE ( )  GEOMETRIC_REPRESENTATION_ITEM ( )  RATIONAL_B_SPLINE_CURVE ( ( 1.000000000000000000, 0.8047378541243649375, 0.8047378541243649375, 1.000000000000000000 ) ) 
 REPRESENTATION_ITEM ( '' )  );
#41894=FACE_OUTER_BOUND ( 'NONE', #18431, .T. ) ;
#41896=LINE ( 'NONE', #19045, #27121 ) ;
#41898=CARTESIAN_POINT ( 'NONE',  ( -6.695973446814940111, 1.750000000000023315, 160.8182875569279702 ) ) ;
#41900=( BOUNDED_CURVE ( )  B_SPLINE_CURVE ( 3, ( #17017, #33194, #48269, #41377 ),
 .UNSPECIFIED., .F., .F. ) 
 B_SPLINE_CURVE_WITH_KNOTS ( ( 4, 4 ),
 ( 4.712388980384689674, 6.283185307179586232 ),
 .UNSPECIFIED. ) 
 CURVE ( )  GEOMETRIC_REPRESENTATION_ITEM ( )  RATIONAL_B_SPLINE_CURVE ( ( 1.000000000000000000, 0.8047378541243649375, 0.8047378541243649375, 1.000000000000000000 ) ) 
 REPRESENTATION_ITEM ( '' )  );
#41901=VECTOR ( 'NONE', #9752, 1000.000000000000000 ) ;
#41908=EDGE_LOOP ( 'NONE', ( #40808, #25015 ) ) ;
#41911=DIRECTION ( 'NONE',  ( 0.000000000000000000, 0.000000000000000000, 1.000000000000000000 ) ) ;
#41916=( BOUNDED_CURVE ( )  B_SPLINE_CURVE ( 3, ( #33181, #49003, #13889, #6220 ),
 .UNSPECIFIED., .F., .F. ) 
 B_SPLINE_CURVE_WITH_KNOTS ( ( 4, 4 ),
 ( 3.141592653589793116, 4.712388980384689674 ),
 .UNSPECIFIED. ) 
 CURVE ( )  GEOMETRIC_REPRESENTATION_ITEM ( )  RATIONAL_B_SPLINE_CURVE ( ( 1.000000000000000000, 0.8047378541243649375, 0.8047378541243649375, 1.000000000000000000 ) ) 
 REPRESENTATION_ITEM ( '' )  );
#41921=ORIENTED_EDGE ( 'NONE', *, *, #27708, .T. ) ;
#41922=ORIENTED_EDGE ( 'NONE', *, *, #20221, .F. ) ;
#41925=CARTESIAN_POINT ( 'NONE',  ( 155.0540265531850537, 2.143131898507880377E-16, -0.9317124430720247208 ) ) ;
#41928=PLANE ( 'NONE',  #4295 ) ;
#41929=ORIENTED_EDGE ( 'NONE', *, *, #25848, .T. ) ;
#41930=EDGE_CURVE ( 'NONE', #42224, #46895, #22268, .T. ) ;
#41932=CARTESIAN_POINT ( 'NONE',  ( 210.0000000000000568, 2.143131898507880377E-16, -0.9317124430720331585 ) ) ;
#41936=CARTESIAN_POINT ( 'NONE',  ( -86.69597344681496054, 0.000000000000000000, 165.0000000000000000 ) ) ;
#41941=CARTESIAN_POINT ( 'NONE',  ( -206.6959734468149463, 1.750000000000010214, 40.81828755692798438 ) ) ;
#41942=VECTOR ( 'NONE', #18243, 1000.000000000000000 ) ;
#41945=DIRECTION ( 'NONE',  ( 0.000000000000000000, 0.000000000000000000, 1.000000000000000000 ) ) ;
#41949=CARTESIAN_POINT ( 'NONE',  ( 35.05402655318504657, 2.143131898507880377E-16, -80.93171244307204404 ) ) ;
#41951=CARTESIAN_POINT ( 'NONE',  ( -168.4459734468149463, 0.000000000000000000, 122.5682875569279702 ) ) ;
#41975=ORIENTED_EDGE ( 'NONE', *, *, #44048, .F. ) ;
#41977=LINE ( 'NONE', #26585, #7944 ) ;
#41980=CYLINDRICAL_SURFACE ( 'NONE', #7521, 1.750000000000015543 ) ;
#41982=ORIENTED_EDGE ( 'NONE', *, *, #1170, .F. ) ;
#41985=DIRECTION ( 'NONE',  ( -0.000000000000000000, -0.000000000000000000, -1.000000000000000000 ) ) ;
#41987=EDGE_CURVE ( 'NONE', #33640, #25713, #15388, .T. ) ;
#41989=ORIENTED_EDGE ( 'NONE', *, *, #35302, .T. ) ;
#41990=ADVANCED_FACE ( 'NONE', ( #24352 ), #9687, .T. ) ;
#41991=CARTESIAN_POINT ( 'NONE',  ( 191.5540265531851105, 0.000000000000000000, 42.56828755692798438 ) ) ;
#41995=CARTESIAN_POINT ( 'NONE',  ( -84.94597344681494633, 2.143131898507880377E-16, 165.0000000000000000 ) ) ;
#41996=CARTESIAN_POINT ( 'NONE',  ( 210.0000000000000568, 0.000000000000000000, -157.4317124430720298 ) ) ;
#41998=CARTESIAN_POINT ( 'NONE',  ( 195.0540265531851105, 2.143131898507880377E-16, -157.4317124430720582 ) ) ;
#42001=CARTESIAN_POINT ( 'NONE',  ( -48.44597344681496054, 1.025126265847089435, -117.4317124430720156 ) ) ;
#42003=FACE_OUTER_BOUND ( 'NONE', #4908, .T. ) ;
#42005=ORIENTED_EDGE ( 'NONE', *, *, #4896, .T. ) ;
#42010=ORIENTED_EDGE ( 'NONE', *, *, #50388, .T. ) ;
#42011=CYLINDRICAL_SURFACE ( 'NONE', #46108, 1.749999999999973799 ) ;
#42013=DIRECTION ( 'NONE',  ( 0.000000000000000000, 0.000000000000000000, 1.000000000000000000 ) ) ;
#42015=CARTESIAN_POINT ( 'NONE',  ( 33.30402655318503946, 0.000000000000000000, 165.0000000000000000 ) ) ;
#42022=ADVANCED_FACE ( 'NONE', ( #44549 ), #991, .F. ) ;
#42023=CARTESIAN_POINT ( 'NONE',  ( -88.44597344681494633, -1.025126265847089657, -37.43171244307202272 ) ) ;
#42033=CARTESIAN_POINT ( 'NONE',  ( -127.7210997126620242, -1.749999999999996669, -158.1565861772249377 ) ) ;
#42035=ORIENTED_EDGE ( 'NONE', *, *, #9441, .F. ) ;
#42044=EDGE_LOOP ( 'NONE', ( #35557, #4546, #38057, #38513, #2305, #20127 ) ) ;
#42045=VECTOR ( 'NONE', #36107, 1000.000000000000000 ) ;
#42051=LINE ( 'NONE', #3548, #23365 ) ;
#42053=EDGE_CURVE ( 'NONE', #41350, #41145, #16054, .T. ) ;
#42054=( BOUNDED_CURVE ( )  B_SPLINE_CURVE ( 3, ( #47600, #36368, #8890, #20429 ),
 .UNSPECIFIED., .F., .F. ) 
 B_SPLINE_CURVE_WITH_KNOTS ( ( 4, 4 ),
 ( 1.570796326794896558, 3.141592653589793116 ),
 .UNSPECIFIED. ) 
 CURVE ( )  GEOMETRIC_REPRESENTATION_ITEM ( )  RATIONAL_B_SPLINE_CURVE ( ( 1.000000000000000000, 0.8047378541243649375, 0.8047378541243649375, 1.000000000000000000 ) ) 
 REPRESENTATION_ITEM ( '' )  );
#42062=LINE ( 'NONE', #2805, #9156 ) ;
#42067=ORIENTED_EDGE ( 'NONE', *, *, #45859, .F. ) ;
#42068=CARTESIAN_POINT ( 'NONE',  ( -126.6959734468149321, -1.749999999999997335, -119.1817124430720440 ) ) ;
#42075=VECTOR ( 'NONE', #34399, 1000.000000000000000 ) ;
#42076=CARTESIAN_POINT ( 'NONE',  ( 33.30402655318503946, -1.750000000000010214, 40.81828755692798438 ) ) ;
#42077=VERTEX_POINT ( 'NONE', #22497 ) ;
#42081=FACE_OUTER_BOUND ( 'NONE', #27640, .T. ) ;
#42085=ORIENTED_EDGE ( 'NONE', *, *, #35416, .F. ) ;
#42088=AXIS2_PLACEMENT_3D ( 'NONE', #8370, #28366, #44489 ) ;
#42089=ORIENTED_EDGE ( 'NONE', *, *, #48665, .T. ) ;
#42093=CARTESIAN_POINT ( 'NONE',  ( -206.6959734468149463, 1.750000000000010658, -79.18171244307201562 ) ) ;
#42098=DIRECTION ( 'NONE',  ( -0.000000000000000000, -0.000000000000000000, -1.000000000000000000 ) ) ;
#42104=AXIS2_PLACEMENT_3D ( 'NONE', #18058, #40914, #49315 ) ;
#42108=EDGE_CURVE ( 'NONE', #13712, #8918, #37419, .T. ) ;
#42111=CYLINDRICAL_SURFACE ( 'NONE', #23684, 1.749999999999973799 ) ;
#42117=ORIENTED_EDGE ( 'NONE', *, *, #17390, .F. ) ;
#42119=EDGE_CURVE ( 'NONE', #7169, #34395, #45807, .T. ) ;
#42122=CARTESIAN_POINT ( 'NONE',  ( -168.4459734468149463, 0.000000000000000000, -77.43171244307204404 ) ) ;
#42123=EDGE_CURVE ( 'NONE', #3878, #44684, #29464, .T. ) ;
#42124=ORIENTED_EDGE ( 'NONE', *, *, #1188, .F. ) ;
#42125=LINE ( 'NONE', #30863, #11439 ) ;
#42126=ORIENTED_EDGE ( 'NONE', *, *, #12042, .T. ) ;
#42131=EDGE_CURVE ( 'NONE', #41850, #5763, #25567, .T. ) ;
#42134=EDGE_CURVE ( 'NONE', #13983, #18505, #38023, .T. ) ;
#42135=LINE ( 'NONE', #38062, #1666 ) ;
#42141=CARTESIAN_POINT ( 'NONE',  ( -126.6959734468149321, -1.749999999999996891, 0.8182875569279768335 ) ) ;
#42143=EDGE_CURVE ( 'NONE', #23855, #39145, #49648, .T. ) ;
#42149=ORIENTED_EDGE ( 'NONE', *, *, #19283, .F. ) ;
#42150=ORIENTED_EDGE ( 'NONE', *, *, #36864, .T. ) ;
#42155=CYLINDRICAL_SURFACE ( 'NONE', #46410, 1.750000000000001554 ) ;
#42158=EDGE_CURVE ( 'NONE', #32209, #17157, #46333, .T. ) ;
#42159=CARTESIAN_POINT ( 'NONE',  ( -168.4459734468149463, 0.000000000000000000, -80.93171244307201562 ) ) ;
#42160=CARTESIAN_POINT ( 'NONE',  ( 152.2789002873379900, 1.750000000000010436, -80.20683870891910772 ) ) ;
#42161=VECTOR ( 'NONE', #2435, 1000.000000000000000 ) ;
#42163=ORIENTED_EDGE ( 'NONE', *, *, #7993, .T. ) ;
#42167=AXIS2_PLACEMENT_3D ( 'NONE', #39312, #8257, #35470 ) ;
#42172=ORIENTED_EDGE ( 'NONE', *, *, #28728, .T. ) ;
#42174=CYLINDRICAL_SURFACE ( 'NONE', #4547, 1.750000000000015543 ) ;
#42178=CARTESIAN_POINT ( 'NONE',  ( 111.5540265531850679, 0.000000000000000000, 39.06828755692798438 ) ) ;
#42181=CARTESIAN_POINT ( 'NONE',  ( 210.0000000000000568, 0.000000000000000000, 162.5682875569279702 ) ) ;
#42189=EDGE_CURVE ( 'NONE', #49578, #10836, #41601, .T. ) ;
#42190=( BOUNDED_CURVE ( )  B_SPLINE_CURVE ( 3, ( #10464, #6358, #6612, #7127 ),
 .UNSPECIFIED., .F., .F. ) 
 B_SPLINE_CURVE_WITH_KNOTS ( ( 4, 4 ),
 ( 4.712388980384689674, 6.283185307179586232 ),
 .UNSPECIFIED. ) 
 CURVE ( )  GEOMETRIC_REPRESENTATION_ITEM ( )  RATIONAL_B_SPLINE_CURVE ( ( 1.000000000000000000, 0.8047378541243649375, 0.8047378541243649375, 1.000000000000000000 ) ) 
 REPRESENTATION_ITEM ( '' )  );
#42195=( BOUNDED_CURVE ( )  B_SPLINE_CURVE ( 3, ( #44891, #18215, #1582, #33893 ),
 .UNSPECIFIED., .F., .F. ) 
 B_SPLINE_CURVE_WITH_KNOTS ( ( 4, 4 ),
 ( 0.000000000000000000, 1.570796326794896558 ),
 .UNSPECIFIED. ) 
 CURVE ( )  GEOMETRIC_REPRESENTATION_ITEM ( )  RATIONAL_B_SPLINE_CURVE ( ( 1.000000000000000000, 0.8047378541243649375, 0.8047378541243649375, 1.000000000000000000 ) ) 
 REPRESENTATION_ITEM ( '' )  );
#42196=CARTESIAN_POINT ( 'NONE',  ( 115.0540265531850395, 2.143131898507847836E-16, 165.0000000000000000 ) ) ;
#42197=VERTEX_POINT ( 'NONE', #43511 ) ;
#42201=CARTESIAN_POINT ( 'NONE',  ( -166.6959734468149463, -1.750000000000010214, 40.81828755692798438 ) ) ;
#42202=AXIS2_PLACEMENT_3D ( 'NONE', #50215, #47144, #12049 ) ;
#42204=CARTESIAN_POINT ( 'NONE',  ( 193.3040265531851105, 0.000000000000000000, 165.0000000000000000 ) ) ;
#42208=( BOUNDED_CURVE ( )  B_SPLINE_CURVE ( 3, ( #41413, #41666, #44979, #22166 ),
 .UNSPECIFIED., .F., .F. ) 
 B_SPLINE_CURVE_WITH_KNOTS ( ( 4, 4 ),
 ( 1.570796326794896558, 3.141592653589793116 ),
 .UNSPECIFIED. ) 
 CURVE ( )  GEOMETRIC_REPRESENTATION_ITEM ( )  RATIONAL_B_SPLINE_CURVE ( ( 1.000000000000000000, 0.8047378541243649375, 0.8047378541243649375, 1.000000000000000000 ) ) 
 REPRESENTATION_ITEM ( '' )  );
#42211=DIRECTION ( 'NONE',  ( -1.000000000000000000, -0.000000000000000000, -0.000000000000000000 ) ) ;
#42212=EDGE_CURVE ( 'NONE', #5114, #2259, #7617, .T. ) ;
#42213=DIRECTION ( 'NONE',  ( -1.000000000000000000, 0.000000000000000000, 0.000000000000000000 ) ) ;
#42222=ORIENTED_EDGE ( 'NONE', *, *, #23634, .F. ) ;
#42224=VERTEX_POINT ( 'NONE', #43001 ) ;
#42225=CARTESIAN_POINT ( 'NONE',  ( -168.4459734468149463, 0.000000000000000000, 79.06828755692797017 ) ) ;
#42229=CARTESIAN_POINT ( 'NONE',  ( -47.72109971266203132, -1.750000000000009548, -160.2068387089191219 ) ) ;
#42231=CARTESIAN_POINT ( 'NONE',  ( 31.55402655318503236, 0.000000000000000000, 39.06828755692798438 ) ) ;
#42234=ORIENTED_EDGE ( 'NONE', *, *, #12642, .T. ) ;
#42237=CARTESIAN_POINT ( 'NONE',  ( -46.69597344681494633, 1.750000000000010214, -39.18171244307202983 ) ) ;
#42238=CARTESIAN_POINT ( 'NONE',  ( 71.55402655318505367, -1.025126265847089657, 79.06828755692797017 ) ) ;
#42241=CARTESIAN_POINT ( 'NONE',  ( 75.05402655318509630, 1.025126265847089213, -160.9317124430720014 ) ) ;
#42244=CARTESIAN_POINT ( 'NONE',  ( 34.32915281903212446, -1.750000000000009548, -38.15658617722494483 ) ) ;
#42249=CARTESIAN_POINT ( 'NONE',  ( -85.67084718096784002, 1.750000000000009548, 41.84341382277508359 ) ) ;
#42254=DIRECTION ( 'NONE',  ( -1.000000000000000000, 0.000000000000000000, 0.000000000000000000 ) ) ;
#42257=EDGE_LOOP ( 'NONE', ( #11069, #16878, #33984, #8792, #31630, #49007 ) ) ;
#42264=FACE_OUTER_BOUND ( 'NONE', #47776, .T. ) ;
#42271=CARTESIAN_POINT ( 'NONE',  ( 33.30402655318503946, 0.000000000000000000, 165.0000000000000000 ) ) ;
#42272=EDGE_CURVE ( 'NONE', #28163, #11666, #3759, .T. ) ;
#42277=DIRECTION ( 'NONE',  ( -1.000000000000000000, -0.000000000000000000, -0.000000000000000000 ) ) ;
#42280=ORIENTED_EDGE ( 'NONE', *, *, #26521, .F. ) ;
#42282=DIRECTION ( 'NONE',  ( 0.000000000000000000, 0.000000000000000000, 1.000000000000000000 ) ) ;
#42284=CARTESIAN_POINT ( 'NONE',  ( 113.3040265531850537, -1.749999999999997335, -79.18171244307201562 ) ) ;
#42288=DIRECTION ( 'NONE',  ( 1.000000000000000000, 0.000000000000000000, -0.000000000000000000 ) ) ;
#42291=AXIS2_PLACEMENT_3D ( 'NONE', #33417, #13642, #41349 ) ;
#42298=ORIENTED_EDGE ( 'NONE', *, *, #1410, .T. ) ;
#42301=EDGE_LOOP ( 'NONE', ( #2169, #3632, #24226, #23238, #5749 ) ) ;
#42304=CARTESIAN_POINT ( 'NONE',  ( 111.5540265531850537, 1.025126265847081886, 79.06828755692797017 ) ) ;
#42312=EDGE_LOOP ( 'NONE', ( #23059, #24442, #37021, #10614, #50017 ) ) ;
#42314=CARTESIAN_POINT ( 'NONE',  ( -7.721099712662037540, -1.750000000000023315, -38.15658617722493062 ) ) ;
#42328=ORIENTED_EDGE ( 'NONE', *, *, #9041, .T. ) ;
#42329=DIRECTION ( 'NONE',  ( 0.000000000000000000, 0.000000000000000000, 1.000000000000000000 ) ) ;
#42333=ORIENTED_EDGE ( 'NONE', *, *, #30777, .F. ) ;
#42334=VECTOR ( 'NONE', #38702, 1000.000000000000000 ) ;
#42342=FACE_OUTER_BOUND ( 'NONE', #32531, .T. ) ;
#42348=CARTESIAN_POINT ( 'NONE',  ( -164.9459734468149463, 1.025126265847089657, -37.43171244307202272 ) ) ;
#42351=CARTESIAN_POINT ( 'NONE',  ( -45.67084718096785423, -1.750000000000009326, -158.1565861772249377 ) ) ;
#42353=( BOUNDED_CURVE ( )  B_SPLINE_CURVE ( 3, ( #35064, #50633, #15534, #31197 ),
 .UNSPECIFIED., .F., .F. ) 
 B_SPLINE_CURVE_WITH_KNOTS ( ( 4, 4 ),
 ( 0.000000000000000000, 1.570796326794896558 ),
 .UNSPECIFIED. ) 
 CURVE ( )  GEOMETRIC_REPRESENTATION_ITEM ( )  RATIONAL_B_SPLINE_CURVE ( ( 1.000000000000000000, 0.8047378541243649375, 0.8047378541243649375, 1.000000000000000000 ) ) 
 REPRESENTATION_ITEM ( '' )  );
#42355=ORIENTED_EDGE ( 'NONE', *, *, #8382, .T. ) ;
#42358=CARTESIAN_POINT ( 'NONE',  ( 31.55402655318503236, 1.025126265847089435, -117.4317124430720156 ) ) ;
#42360=ORIENTED_EDGE ( 'NONE', *, *, #314, .F. ) ;
#42364=EDGE_CURVE ( 'NONE', #49806, #22181, #5017, .T. ) ;
#42365=ORIENTED_EDGE ( 'NONE', *, *, #22080, .T. ) ;
#42379=EDGE_LOOP ( 'NONE', ( #42298, #12360 ) ) ;
#42383=CARTESIAN_POINT ( 'NONE',  ( 113.3040265531850537, 0.000000000000000000, 165.0000000000000000 ) ) ;
#42386=ORIENTED_EDGE ( 'NONE', *, *, #2878, .F. ) ;
#42394=ORIENTED_EDGE ( 'NONE', *, *, #38681, .T. ) ;
#42398=ORIENTED_EDGE ( 'NONE', *, *, #11534, .F. ) ;
#42399=CARTESIAN_POINT ( 'NONE',  ( 74.32915281903215998, 1.750000000000009548, -0.2068387089191121020 ) ) ;
#42401=DIRECTION ( 'NONE',  ( -1.000000000000000000, 0.000000000000000000, 0.000000000000000000 ) ) ;
#42408=CARTESIAN_POINT ( 'NONE',  ( 195.0540265531851105, -1.025126265847089435, 82.56828755692798438 ) ) ;
#42411=VERTEX_POINT ( 'NONE', #17327 ) ;
#42414=EDGE_LOOP ( 'NONE', ( #36118, #45489, #39403, #39861, #46226, #32488 ) ) ;
#42415=CARTESIAN_POINT ( 'NONE',  ( -8.445973446814962315, 1.025126265847096985, 162.5682875569279986 ) ) ;
#42417=VERTEX_POINT ( 'NONE', #16578 ) ;
#42421=VERTEX_POINT ( 'NONE', #21677 ) ;
#42422=DIRECTION ( 'NONE',  ( -1.000000000000000000, -0.000000000000000000, -0.000000000000000000 ) ) ;
#42425=ADVANCED_FACE ( 'NONE', ( #49586 ), #5779, .T. ) ;
#42426=DIRECTION ( 'NONE',  ( -0.000000000000000000, -0.000000000000000000, -1.000000000000000000 ) ) ;
#42430=( BOUNDED_CURVE ( )  B_SPLINE_CURVE ( 3, ( #12066, #31321, #16408, #7969 ),
 .UNSPECIFIED., .F., .F. ) 
 B_SPLINE_CURVE_WITH_KNOTS ( ( 4, 4 ),
 ( 0.000000000000000000, 1.570796326794896558 ),
 .UNSPECIFIED. ) 
 CURVE ( )  GEOMETRIC_REPRESENTATION_ITEM ( )  RATIONAL_B_SPLINE_CURVE ( ( 1.000000000000000000, 0.8047378541243649375, 0.8047378541243649375, 1.000000000000000000 ) ) 
 REPRESENTATION_ITEM ( '' )  );
#42438=CARTESIAN_POINT ( 'NONE',  ( -210.0000000000000568, 0.000000000000000000, -119.1817124430720440 ) ) ;
#42443=EDGE_CURVE ( 'NONE', #40582, #17018, #27223, .T. ) ;
#42444=CYLINDRICAL_SURFACE ( 'NONE', #30419, 1.750000000000001554 ) ;
#42448=EDGE_CURVE ( 'NONE', #40485, #30782, #18656, .T. ) ;
#42453=VERTEX_POINT ( 'NONE', #17581 ) ;
#42455=LINE ( 'NONE', #2456, #20995 ) ;
#42459=VERTEX_POINT ( 'NONE', #14223 ) ;
#42462=CYLINDRICAL_SURFACE ( 'NONE', #29981, 1.750000000000015543 ) ;
#42464=VERTEX_POINT ( 'NONE', #29886 ) ;
#42465=ORIENTED_EDGE ( 'NONE', *, *, #7218, .T. ) ;
#42472=ORIENTED_EDGE ( 'NONE', *, *, #25370, .F. ) ;
#42475=CARTESIAN_POINT ( 'NONE',  ( 33.30402655318503946, 1.750000000000010214, -39.18171244307202983 ) ) ;
#42478=ORIENTED_EDGE ( 'NONE', *, *, #34394, .T. ) ;
#42480=VERTEX_POINT ( 'NONE', #29382 ) ;
#42481=CARTESIAN_POINT ( 'NONE',  ( 111.5540265531850679, 0.000000000000000000, 42.56828755692795596 ) ) ;
#42482=CARTESIAN_POINT ( 'NONE',  ( 155.0540265531850537, 2.143131898507880377E-16, 2.568287556927978166 ) ) ;
#42483=( BOUNDED_CURVE ( )  B_SPLINE_CURVE ( 3, ( #10967, #8145, #24052, #23265 ),
 .UNSPECIFIED., .F., .F. ) 
 B_SPLINE_CURVE_WITH_KNOTS ( ( 4, 4 ),
 ( 3.141592653589793116, 4.712388980384689674 ),
 .UNSPECIFIED. ) 
 CURVE ( )  GEOMETRIC_REPRESENTATION_ITEM ( )  RATIONAL_B_SPLINE_CURVE ( ( 1.000000000000000000, 0.8047378541243649375, 0.8047378541243649375, 1.000000000000000000 ) ) 
 REPRESENTATION_ITEM ( '' )  );
#42484=EDGE_CURVE ( 'NONE', #49918, #23986, #32480, .T. ) ;
#42487=EDGE_CURVE ( 'NONE', #17310, #8816, #37368, .T. ) ;
#42490=VERTEX_POINT ( 'NONE', #10394 ) ;
#42494=( BOUNDED_CURVE ( )  B_SPLINE_CURVE ( 3, ( #20320, #7517, #23152, #23918 ),
 .UNSPECIFIED., .F., .F. ) 
 B_SPLINE_CURVE_WITH_KNOTS ( ( 4, 4 ),
 ( 4.712388980384689674, 6.283185307179586232 ),
 .UNSPECIFIED. ) 
 CURVE ( )  GEOMETRIC_REPRESENTATION_ITEM ( )  RATIONAL_B_SPLINE_CURVE ( ( 1.000000000000000000, 0.8047378541243649375, 0.8047378541243649375, 1.000000000000000000 ) ) 
 REPRESENTATION_ITEM ( '' )  );
#42497=CARTESIAN_POINT ( 'NONE',  ( 113.3040265531850537, 1.749999999999997113, 40.81828755692798438 ) ) ;
#42502=FACE_OUTER_BOUND ( 'NONE', #10995, .T. ) ;
#42510=CARTESIAN_POINT ( 'NONE',  ( 74.32915281903215998, -1.750000000000010436, -80.20683870891910772 ) ) ;
#42515=ORIENTED_EDGE ( 'NONE', *, *, #6658, .T. ) ;
#42519=EDGE_LOOP ( 'NONE', ( #44481, #36557, #15532, #23746, #47966, #46756 ) ) ;
#42526=AXIS2_PLACEMENT_3D ( 'NONE', #3566, #27187, #7688 ) ;
#42535=ORIENTED_EDGE ( 'NONE', *, *, #21222, .F. ) ;
#42538=ORIENTED_EDGE ( 'NONE', *, *, #26445, .F. ) ;
#42539=FACE_OUTER_BOUND ( 'NONE', #12946, .T. ) ;
#42545=CARTESIAN_POINT ( 'NONE',  ( 71.55402655318505367, 0.000000000000000000, -165.0000000000000000 ) ) ;
#42546=EDGE_CURVE ( 'NONE', #50239, #8111, #50085, .T. ) ;
#42548=CARTESIAN_POINT ( 'NONE',  ( 31.55402655318503236, -1.025126265847089657, 119.0682875569279560 ) ) ;
#42553=VERTEX_POINT ( 'NONE', #3697 ) ;
#42554=EDGE_CURVE ( 'NONE', #21151, #17197, #29174, .T. ) ;
#42556=EDGE_CURVE ( 'NONE', #48152, #45274, #34425, .T. ) ;
#42558=DIRECTION ( 'NONE',  ( -1.000000000000000000, -0.000000000000000000, -0.000000000000000000 ) ) ;
#42561=EDGE_LOOP ( 'NONE', ( #48453, #34506, #29929, #43918, #33036, #20706 ) ) ;
#42563=VECTOR ( 'NONE', #9230, 1000.000000000000000 ) ;
#42564=CARTESIAN_POINT ( 'NONE',  ( -126.6959734468149321, 1.749999999999997335, -79.18171244307201562 ) ) ;
#42575=LINE ( 'NONE', #26938, #1980 ) ;
#42578=ORIENTED_EDGE ( 'NONE', *, *, #49624, .T. ) ;
#42579=DIRECTION ( 'NONE',  ( 1.000000000000000000, 0.000000000000000000, 0.000000000000000000 ) ) ;
#42584=CARTESIAN_POINT ( 'NONE',  ( 153.3040265531850537, 0.000000000000000000, 165.0000000000000000 ) ) ;
#42591=AXIS2_PLACEMENT_3D ( 'NONE', #1010, #35917, #32823 ) ;
#42592=VECTOR ( 'NONE', #13176, 1000.000000000000000 ) ;
#42600=ORIENTED_EDGE ( 'NONE', *, *, #23556, .T. ) ;
#42601=CARTESIAN_POINT ( 'NONE',  ( 191.5540265531850537, 1.025126265847089213, -160.9317124430720014 ) ) ;
#42603=CARTESIAN_POINT ( 'NONE',  ( -210.0000000000000568, 0.000000000000000000, 122.5682875569279844 ) ) ;
#42608=EDGE_LOOP ( 'NONE', ( #33676, #16318, #38505, #19780, #3601, #38340 ) ) ;
#42620=DIRECTION ( 'NONE',  ( -1.000000000000000000, -0.000000000000000000, -0.000000000000000000 ) ) ;
#42622=ORIENTED_EDGE ( 'NONE', *, *, #12042, .F. ) ;
#42625=CARTESIAN_POINT ( 'NONE',  ( 210.0000000000000568, 0.000000000000000000, 160.8182875569279702 ) ) ;
#42626=CARTESIAN_POINT ( 'NONE',  ( -46.69597344681494633, 1.750000000000010214, -39.18171244307202983 ) ) ;
#42628=( BOUNDED_CURVE ( )  B_SPLINE_CURVE ( 3, ( #34767, #3169, #19080, #30139 ),
 .UNSPECIFIED., .F., .F. ) 
 B_SPLINE_CURVE_WITH_KNOTS ( ( 4, 4 ),
 ( 3.141592653589793116, 4.712388980384689674 ),
 .UNSPECIFIED. ) 
 CURVE ( )  GEOMETRIC_REPRESENTATION_ITEM ( )  RATIONAL_B_SPLINE_CURVE ( ( 1.000000000000000000, 0.8047378541243649375, 0.8047378541243649375, 1.000000000000000000 ) ) 
 REPRESENTATION_ITEM ( '' )  );
#42632=CARTESIAN_POINT ( 'NONE',  ( 35.05402655318504657, 2.143131898507882349E-16, 165.0000000000000000 ) ) ;
#42637=CYLINDRICAL_SURFACE ( 'NONE', #11840, 1.750000000000010214 ) ;
#42640=CARTESIAN_POINT ( 'NONE',  ( 115.0540265531850395, 2.143131898507847836E-16, -0.9317124430719969652 ) ) ;
#42641=VERTEX_POINT ( 'NONE', #21116 ) ;
#42648=( BOUNDED_CURVE ( )  B_SPLINE_CURVE ( 3, ( #40031, #39025, #23867, #35435 ),
 .UNSPECIFIED., .F., .F. ) 
 B_SPLINE_CURVE_WITH_KNOTS ( ( 4, 4 ),
 ( 4.712388980384689674, 6.283185307179586232 ),
 .UNSPECIFIED. ) 
 CURVE ( )  GEOMETRIC_REPRESENTATION_ITEM ( )  RATIONAL_B_SPLINE_CURVE ( ( 1.000000000000000000, 0.8047378541243649375, 0.8047378541243649375, 1.000000000000000000 ) ) 
 REPRESENTATION_ITEM ( '' )  );
#42656=FACE_OUTER_BOUND ( 'NONE', #33516, .T. ) ;
#42659=EDGE_LOOP ( 'NONE', ( #46329, #19009, #45300, #14647, #29298, #11942 ) ) ;
#42663=LINE ( 'NONE', #45982, #39818 ) ;
#42667=ORIENTED_EDGE ( 'NONE', *, *, #10352, .F. ) ;
#42671=DIRECTION ( 'NONE',  ( -0.000000000000000000, -0.000000000000000000, -1.000000000000000000 ) ) ;
#42672=ORIENTED_EDGE ( 'NONE', *, *, #36269, .T. ) ;
#42673=CARTESIAN_POINT ( 'NONE',  ( -88.44597344681497475, 0.000000000000000000, 39.06828755692795596 ) ) ;
#42675=ORIENTED_EDGE ( 'NONE', *, *, #28784, .T. ) ;
#42677=CARTESIAN_POINT ( 'NONE',  ( 210.0000000000000568, 0.000000000000000000, 120.8182875569279702 ) ) ;
#42679=CARTESIAN_POINT ( 'NONE',  ( 153.3040265531850537, -1.750000000000009992, 0.8182875569279768335 ) ) ;
#42683=VERTEX_POINT ( 'NONE', #35799 ) ;
#42697=DIRECTION ( 'NONE',  ( -1.000000000000000000, -0.000000000000000000, -0.000000000000000000 ) ) ;
#42700=AXIS2_PLACEMENT_3D ( 'NONE', #35095, #46325, #42254 ) ;
#42704=CYLINDRICAL_SURFACE ( 'NONE', #29165, 1.750000000000015543 ) ;
#42708=CARTESIAN_POINT ( 'NONE',  ( -126.6959734468149321, -1.749999999999997113, 40.81828755692798438 ) ) ;
#42709=LINE ( 'NONE', #7584, #24948 ) ;
#42710=LINE ( 'NONE', #42969, #20973 ) ;
#42713=VERTEX_POINT ( 'NONE', #23964 ) ;
#42716=ORIENTED_EDGE ( 'NONE', *, *, #22712, .T. ) ;
#42721=( BOUNDED_CURVE ( )  B_SPLINE_CURVE ( 3, ( #23432, #30621, #12136, #4430 ),
 .UNSPECIFIED., .F., .F. ) 
 B_SPLINE_CURVE_WITH_KNOTS ( ( 4, 4 ),
 ( 3.141592653589793116, 4.712388980384689674 ),
 .UNSPECIFIED. ) 
 CURVE ( )  GEOMETRIC_REPRESENTATION_ITEM ( )  RATIONAL_B_SPLINE_CURVE ( ( 1.000000000000000000, 0.8047378541243649375, 0.8047378541243649375, 1.000000000000000000 ) ) 
 REPRESENTATION_ITEM ( '' )  );
#42724=DIRECTION ( 'NONE',  ( -0.000000000000000000, -0.000000000000000000, -1.000000000000000000 ) ) ;
#42734=EDGE_CURVE ( 'NONE', #12712, #16019, #12908, .T. ) ;
#42738=EDGE_CURVE ( 'NONE', #10420, #13192, #7902, .T. ) ;
#42741=CARTESIAN_POINT ( 'NONE',  ( 151.5540265531850537, 0.000000000000000000, -37.43171244307205825 ) ) ;
#42742=EDGE_CURVE ( 'NONE', #5180, #23932, #13123, .T. ) ;
#42743=CARTESIAN_POINT ( 'NONE',  ( 151.5540265531850537, 0.000000000000000000, 165.0000000000000000 ) ) ;
#42747=CARTESIAN_POINT ( 'NONE',  ( -206.6959734468149463, 0.000000000000000000, 165.0000000000000000 ) ) ;
#42748=CARTESIAN_POINT ( 'NONE',  ( -166.6959734468149463, -1.750000000000009992, -159.1817124430720298 ) ) ;
#42749=ORIENTED_EDGE ( 'NONE', *, *, #13596, .F. ) ;
#42751=CARTESIAN_POINT ( 'NONE',  ( -165.6708471809677974, 1.750000000000010214, 121.8434138227750623 ) ) ;
#42752=EDGE_LOOP ( 'NONE', ( #23924, #23488, #39792, #1086, #38677, #6714 ) ) ;
#42759=CARTESIAN_POINT ( 'NONE',  ( 35.05402655318504657, 2.143131898507880377E-16, 2.568287556927978166 ) ) ;
#42763=ORIENTED_EDGE ( 'NONE', *, *, #38948, .T. ) ;
#42766=ADVANCED_FACE ( 'NONE', ( #39625 ), #32177, .T. ) ;
#42767=ADVANCED_FACE ( 'NONE', ( #32674 ), #48272, .T. ) ;
#42771=FACE_OUTER_BOUND ( 'NONE', #2905, .T. ) ;
#42773=EDGE_CURVE ( 'NONE', #12693, #14684, #39973, .T. ) ;
#42781=CARTESIAN_POINT ( 'NONE',  ( 195.0540265531851105, 2.143131898507880377E-16, -160.9317124430720014 ) ) ;
#42783=EDGE_LOOP ( 'NONE', ( #25499, #30343, #13683, #8246, #36664, #30841 ) ) ;
#42787=( BOUNDED_CURVE ( )  B_SPLINE_CURVE ( 3, ( #38116, #30404, #14494, #48646 ),
 .UNSPECIFIED., .F., .F. ) 
 B_SPLINE_CURVE_WITH_KNOTS ( ( 4, 4 ),
 ( 4.712388980384689674, 6.283185307179586232 ),
 .UNSPECIFIED. ) 
 CURVE ( )  GEOMETRIC_REPRESENTATION_ITEM ( )  RATIONAL_B_SPLINE_CURVE ( ( 1.000000000000000000, 0.8047378541243649375, 0.8047378541243649375, 1.000000000000000000 ) ) 
 REPRESENTATION_ITEM ( '' )  );
#42788=VECTOR ( 'NONE', #48810, 1000.000000000000000 ) ;
#42791=EDGE_CURVE ( 'NONE', #38537, #24864, #39667, .T. ) ;
#42797=CARTESIAN_POINT ( 'NONE',  ( -127.7210997126620242, 1.749999999999996225, -158.1565861772249377 ) ) ;
#42798=CARTESIAN_POINT ( 'NONE',  ( -128.4459734468149179, 0.000000000000000000, 119.0682875569279986 ) ) ;
#42802=CARTESIAN_POINT ( 'NONE',  ( -86.69597344681494633, -1.750000000000010214, 40.81828755692798438 ) ) ;
#42803=CARTESIAN_POINT ( 'NONE',  ( -208.4459734468149463, 0.000000000000000000, 165.0000000000000000 ) ) ;
#42804=AXIS2_PLACEMENT_3D ( 'NONE', #28306, #12644, #8814 ) ;
#42813=CYLINDRICAL_SURFACE ( 'NONE', #44484, 1.750000000000008438 ) ;
#42817=DIRECTION ( 'NONE',  ( -1.000000000000000000, 0.000000000000000000, 0.000000000000000000 ) ) ;
#42819=CARTESIAN_POINT ( 'NONE',  ( -88.44597344681497475, 0.000000000000000000, 2.568287556928006143 ) ) ;
#42822=ORIENTED_EDGE ( 'NONE', *, *, #41633, .F. ) ;
#42825=ORIENTED_EDGE ( 'NONE', *, *, #7013, .T. ) ;
#42834=ORIENTED_EDGE ( 'NONE', *, *, #18614, .F. ) ;
#42835=CARTESIAN_POINT ( 'NONE',  ( -84.94597344681494633, 2.143131898507880377E-16, 122.5682875569279702 ) ) ;
#42841=EDGE_CURVE ( 'NONE', #24864, #47066, #50086, .T. ) ;
#42843=EDGE_CURVE ( 'NONE', #2131, #33144, #4598, .T. ) ;
#42848=CARTESIAN_POINT ( 'NONE',  ( -164.9459734468149463, 2.143131898507880377E-16, -37.43171244307205825 ) ) ;
#42850=EDGE_LOOP ( 'NONE', ( #19832, #7189, #36887, #48644, #34357, #32053 ) ) ;
#42857=CYLINDRICAL_SURFACE ( 'NONE', #33961, 1.750000000000036193 ) ;
#42859=FACE_OUTER_BOUND ( 'NONE', #30008, .T. ) ;
#42861=ORIENTED_EDGE ( 'NONE', *, *, #26127, .T. ) ;
#42863=CARTESIAN_POINT ( 'NONE',  ( -126.6959734468149321, -1.749999999999996891, -159.1817124430720298 ) ) ;
#42865=ORIENTED_EDGE ( 'NONE', *, *, #8334, .T. ) ;
#42869=CARTESIAN_POINT ( 'NONE',  ( 210.0000000000000568, 0.000000000000000000, -39.18171244307202983 ) ) ;
#42872=CARTESIAN_POINT ( 'NONE',  ( 31.55402655318503236, 0.000000000000000000, -40.93171244307205825 ) ) ;
#42874=CARTESIAN_POINT ( 'NONE',  ( 195.0540265531851105, -1.025126265847089657, 119.0682875569279560 ) ) ;
#42877=DIRECTION ( 'NONE',  ( 1.000000000000000000, 0.000000000000000000, 0.000000000000000000 ) ) ;
#42878=VECTOR ( 'NONE', #19802, 1000.000000000000000 ) ;
#42879=ORIENTED_EDGE ( 'NONE', *, *, #3558, .T. ) ;
#42881=ORIENTED_EDGE ( 'NONE', *, *, #464, .F. ) ;
#42885=ORIENTED_EDGE ( 'NONE', *, *, #40386, .F. ) ;
#42893=DIRECTION ( 'NONE',  ( -1.000000000000000000, 0.000000000000000000, 0.000000000000000000 ) ) ;
#42894=EDGE_CURVE ( 'NONE', #47864, #6375, #43543, .T. ) ;
#42895=CARTESIAN_POINT ( 'NONE',  ( -126.6959734468149321, 1.749999999999996891, 160.8182875569279702 ) ) ;
#42899=DIRECTION ( 'NONE',  ( -1.000000000000000000, -0.000000000000000000, -0.000000000000000000 ) ) ;
#42908=ORIENTED_EDGE ( 'NONE', *, *, #48474, .T. ) ;
#42910=DIRECTION ( 'NONE',  ( 0.000000000000000000, 0.000000000000000000, 1.000000000000000000 ) ) ;
#42912=CARTESIAN_POINT ( 'NONE',  ( -165.6708471809677974, -1.750000000000009326, -158.1565861772249377 ) ) ;
#42916=ORIENTED_EDGE ( 'NONE', *, *, #19516, .F. ) ;
#42917=EDGE_CURVE ( 'NONE', #11294, #10604, #48750, .T. ) ;
#42924=ORIENTED_EDGE ( 'NONE', *, *, #37108, .F. ) ;
#42930=ORIENTED_EDGE ( 'NONE', *, *, #41224, .F. ) ;
#42934=( BOUNDED_CURVE ( )  B_SPLINE_CURVE ( 3, ( #3787, #19437, #35116, #50691 ),
 .UNSPECIFIED., .F., .F. ) 
 B_SPLINE_CURVE_WITH_KNOTS ( ( 4, 4 ),
 ( 3.141592653589793116, 4.712388980384689674 ),
 .UNSPECIFIED. ) 
 CURVE ( )  GEOMETRIC_REPRESENTATION_ITEM ( )  RATIONAL_B_SPLINE_CURVE ( ( 1.000000000000000000, 0.8047378541243649375, 0.8047378541243649375, 1.000000000000000000 ) ) 
 REPRESENTATION_ITEM ( '' )  );
#42942=( BOUNDED_CURVE ( )  B_SPLINE_CURVE ( 3, ( #19201, #4334, #35148, #46623 ),
 .UNSPECIFIED., .F., .F. ) 
 B_SPLINE_CURVE_WITH_KNOTS ( ( 4, 4 ),
 ( 0.000000000000000000, 1.570796326794896780 ),
 .UNSPECIFIED. ) 
 CURVE ( )  GEOMETRIC_REPRESENTATION_ITEM ( )  RATIONAL_B_SPLINE_CURVE ( ( 1.000000000000000000, 0.8047378541243649375, 0.8047378541243649375, 1.000000000000000000 ) ) 
 REPRESENTATION_ITEM ( '' )  );
#42949=ORIENTED_EDGE ( 'NONE', *, *, #41265, .T. ) ;
#42952=( BOUNDED_CURVE ( )  B_SPLINE_CURVE ( 3, ( #25026, #47569, #12705, #24515 ),
 .UNSPECIFIED., .F., .F. ) 
 B_SPLINE_CURVE_WITH_KNOTS ( ( 4, 4 ),
 ( 4.712388980384689674, 6.283185307179586232 ),
 .UNSPECIFIED. ) 
 CURVE ( )  GEOMETRIC_REPRESENTATION_ITEM ( )  RATIONAL_B_SPLINE_CURVE ( ( 1.000000000000000000, 0.8047378541243649375, 0.8047378541243649375, 1.000000000000000000 ) ) 
 REPRESENTATION_ITEM ( '' )  );
#42957=CARTESIAN_POINT ( 'NONE',  ( -128.4459734468149463, -1.025126265847081886, 119.0682875569279702 ) ) ;
#42962=CARTESIAN_POINT ( 'NONE',  ( 155.0540265531850537, 2.143131898507880377E-16, 82.56828755692798438 ) ) ;
#42965=ORIENTED_EDGE ( 'NONE', *, *, #1217, .F. ) ;
#42969=CARTESIAN_POINT ( 'NONE',  ( 210.0000000000000568, 2.143131898507881116E-16, 39.06828755692797728 ) ) ;
#42974=EDGE_CURVE ( 'NONE', #36777, #4637, #3220, .T. ) ;
#42977=CARTESIAN_POINT ( 'NONE',  ( -208.4459734468149463, 0.000000000000000000, 165.0000000000000000 ) ) ;
#42987=DIRECTION ( 'NONE',  ( -1.000000000000000000, -0.000000000000000000, -0.000000000000000000 ) ) ;
#42996=CARTESIAN_POINT ( 'NONE',  ( 210.0000000000000568, 2.143131898507881856E-16, 119.0682875569279560 ) ) ;
#42997=CARTESIAN_POINT ( 'NONE',  ( 35.05402655318504657, 2.143131898507880377E-16, -117.4317124430720156 ) ) ;
#43001=CARTESIAN_POINT ( 'NONE',  ( 31.55402655318503236, 0.000000000000000000, 42.56828755692798438 ) ) ;
#43004=EDGE_CURVE ( 'NONE', #23447, #38333, #8501, .T. ) ;
#43010=DIRECTION ( 'NONE',  ( -1.000000000000000000, 0.000000000000000000, 0.000000000000000000 ) ) ;
#43011=CARTESIAN_POINT ( 'NONE',  ( -168.4459734468149747, -1.025126265847089213, -160.9317124430720014 ) ) ;
#43012=ORIENTED_EDGE ( 'NONE', *, *, #3670, .T. ) ;
#43020=CARTESIAN_POINT ( 'NONE',  ( -87.72109971266203843, 1.750000000000009548, -40.20683870891912193 ) ) ;
#43023=ORIENTED_EDGE ( 'NONE', *, *, #35697, .T. ) ;
#43024=ORIENTED_EDGE ( 'NONE', *, *, #21202, .F. ) ;
#43028=ORIENTED_EDGE ( 'NONE', *, *, #5823, .T. ) ;
#43030=CARTESIAN_POINT ( 'NONE',  ( -8.445973446814914354, 0.000000000000000000, 162.5682875569279702 ) ) ;
#43031=( BOUNDED_CURVE ( )  B_SPLINE_CURVE ( 3, ( #6350, #36679, #21997, #9186 ),
 .UNSPECIFIED., .F., .F. ) 
 B_SPLINE_CURVE_WITH_KNOTS ( ( 4, 4 ),
 ( 1.570796326794896558, 3.141592653589793116 ),
 .UNSPECIFIED. ) 
 CURVE ( )  GEOMETRIC_REPRESENTATION_ITEM ( )  RATIONAL_B_SPLINE_CURVE ( ( 1.000000000000000000, 0.8047378541243649375, 0.8047378541243649375, 1.000000000000000000 ) ) 
 REPRESENTATION_ITEM ( '' )  );
#43034=EDGE_LOOP ( 'NONE', ( #7487, #38324, #45692, #34926, #33667, #7641 ) ) ;
#43035=CYLINDRICAL_SURFACE ( 'NONE', #19245, 1.750000000000015543 ) ;
#43042=VECTOR ( 'NONE', #9192, 1000.000000000000000 ) ;
#43043=ORIENTED_EDGE ( 'NONE', *, *, #41582, .T. ) ;
#43046=EDGE_CURVE ( 'NONE', #4462, #34536, #9009, .T. ) ;
#43062=DIRECTION ( 'NONE',  ( -0.000000000000000000, -0.000000000000000000, -1.000000000000000000 ) ) ;
#43067=AXIS2_PLACEMENT_3D ( 'NONE', #14487, #25280, #9878 ) ;
#43070=CARTESIAN_POINT ( 'NONE',  ( -7.721099712662037540, 1.750000000000023315, 81.84341382277507648 ) ) ;
#43071=DIRECTION ( 'NONE',  ( -1.000000000000000000, -0.000000000000000000, -0.000000000000000000 ) ) ;
#43073=EDGE_CURVE ( 'NONE', #49857, #50159, #20299, .T. ) ;
#43077=CYLINDRICAL_SURFACE ( 'NONE', #14699, 1.750000000000015543 ) ;
#43082=VERTEX_POINT ( 'NONE', #47703 ) ;
#43086=CARTESIAN_POINT ( 'NONE',  ( 35.05402655318504657, 2.143131898507880377E-16, 165.0000000000000000 ) ) ;
#43087=VECTOR ( 'NONE', #407, 1000.000000000000000 ) ;
#43096=( BOUNDED_CURVE ( )  B_SPLINE_CURVE ( 3, ( #33407, #48977, #9284, #25695 ),
 .UNSPECIFIED., .F., .F. ) 
 B_SPLINE_CURVE_WITH_KNOTS ( ( 4, 4 ),
 ( 4.712388980384689674, 6.283185307179586232 ),
 .UNSPECIFIED. ) 
 CURVE ( )  GEOMETRIC_REPRESENTATION_ITEM ( )  RATIONAL_B_SPLINE_CURVE ( ( 1.000000000000000000, 0.8047378541243649375, 0.8047378541243649375, 1.000000000000000000 ) ) 
 REPRESENTATION_ITEM ( '' )  );
#43099=EDGE_CURVE ( 'NONE', #38145, #29600, #16204, .T. ) ;
#43102=DIRECTION ( 'NONE',  ( -1.000000000000000000, -0.000000000000000000, -0.000000000000000000 ) ) ;
#43104=ORIENTED_EDGE ( 'NONE', *, *, #15333, .T. ) ;
#43105=CARTESIAN_POINT ( 'NONE',  ( -208.4459734468149463, 0.000000000000000000, -165.0000000000000000 ) ) ;
#43109=( BOUNDED_CURVE ( )  B_SPLINE_CURVE ( 3, ( #12913, #17283, #1392, #44209 ),
 .UNSPECIFIED., .F., .F. ) 
 B_SPLINE_CURVE_WITH_KNOTS ( ( 4, 4 ),
 ( 4.712388980384689674, 6.283185307179586232 ),
 .UNSPECIFIED. ) 
 CURVE ( )  GEOMETRIC_REPRESENTATION_ITEM ( )  RATIONAL_B_SPLINE_CURVE ( ( 1.000000000000000000, 0.8047378541243649375, 0.8047378541243649375, 1.000000000000000000 ) ) 
 REPRESENTATION_ITEM ( '' )  );
#43125=CARTESIAN_POINT ( 'NONE',  ( -6.695973446814940111, 1.750000000000023759, 40.81828755692798438 ) ) ;
#43133=CARTESIAN_POINT ( 'NONE',  ( -126.6959734468149321, 0.000000000000000000, 165.0000000000000000 ) ) ;
#43142=CARTESIAN_POINT ( 'NONE',  ( 193.3040265531851105, 1.750000000000010214, 40.81828755692798438 ) ) ;
#43143=LINE ( 'NONE', #34966, #16764 ) ;
#43149=EDGE_CURVE ( 'NONE', #46777, #41284, #20554, .T. ) ;
#43150=CARTESIAN_POINT ( 'NONE',  ( -168.4459734468149747, 1.025126265847089435, -77.43171244307200141 ) ) ;
#43152=( NAMED_UNIT ( * ) SI_UNIT ( $, .STERADIAN. ) SOLID_ANGLE_UNIT ( ) );
#43173=ORIENTED_EDGE ( 'NONE', *, *, #35291, .F. ) ;
#43175=CARTESIAN_POINT ( 'NONE',  ( 35.05402655318503946, 0.000000000000000000, 162.5682875569279702 ) ) ;
#43176=ORIENTED_EDGE ( 'NONE', *, *, #1764, .F. ) ;
#43177=CARTESIAN_POINT ( 'NONE',  ( -128.4459734468149179, 0.000000000000000000, -117.4317124430720725 ) ) ;
#43182=ORIENTED_EDGE ( 'NONE', *, *, #38426, .F. ) ;
#43183=EDGE_CURVE ( 'NONE', #47427, #2039, #40560, .T. ) ;
#43189=ORIENTED_EDGE ( 'NONE', *, *, #37492, .F. ) ;
#43202=CARTESIAN_POINT ( 'NONE',  ( 210.0000000000000568, 2.143131898507881856E-16, -80.93171244307202983 ) ) ;
#43203=ADVANCED_FACE ( 'NONE', ( #22059 ), #49470, .T. ) ;
#43209=EDGE_CURVE ( 'NONE', #24506, #44363, #24238, .T. ) ;
#43211=DIRECTION ( 'NONE',  ( 0.000000000000000000, 0.000000000000000000, 1.000000000000000000 ) ) ;
#43213=ADVANCED_FACE ( 'NONE', ( #10509 ), #45128, .T. ) ;
#43216=ORIENTED_EDGE ( 'NONE', *, *, #30694, .F. ) ;
#43220=ORIENTED_EDGE ( 'NONE', *, *, #27757, .F. ) ;
#43222=CARTESIAN_POINT ( 'NONE',  ( -128.4459734468149179, 0.000000000000000000, 42.56828755692794175 ) ) ;
#43223=DIRECTION ( 'NONE',  ( -0.000000000000000000, -0.000000000000000000, -1.000000000000000000 ) ) ;
#43225=ORIENTED_EDGE ( 'NONE', *, *, #23556, .F. ) ;
#43237=EDGE_CURVE ( 'NONE', #41284, #47386, #34734, .T. ) ;
#43238=LINE ( 'NONE', #20145, #27544 ) ;
#43239=( BOUNDED_CURVE ( )  B_SPLINE_CURVE ( 3, ( #13073, #36455, #47677, #47937 ),
 .UNSPECIFIED., .F., .F. ) 
 B_SPLINE_CURVE_WITH_KNOTS ( ( 4, 4 ),
 ( 0.000000000000000000, 1.570796326794896558 ),
 .UNSPECIFIED. ) 
 CURVE ( )  GEOMETRIC_REPRESENTATION_ITEM ( )  RATIONAL_B_SPLINE_CURVE ( ( 1.000000000000000000, 0.8047378541243649375, 0.8047378541243649375, 1.000000000000000000 ) ) 
 REPRESENTATION_ITEM ( '' )  );
#43242=LINE ( 'NONE', #8108, #24158 ) ;
#43243=CARTESIAN_POINT ( 'NONE',  ( 111.5540265531850537, 1.025126265847081664, -117.4317124430720440 ) ) ;
#43245=ORIENTED_EDGE ( 'NONE', *, *, #29806, .F. ) ;
#43246=DIRECTION ( 'NONE',  ( -0.000000000000000000, -0.000000000000000000, -1.000000000000000000 ) ) ;
#43247=( BOUNDED_CURVE ( )  B_SPLINE_CURVE ( 3, ( #13647, #48502, #23757, #13143 ),
 .UNSPECIFIED., .F., .F. ) 
 B_SPLINE_CURVE_WITH_KNOTS ( ( 4, 4 ),
 ( 3.141592653589793116, 4.712388980384689674 ),
 .UNSPECIFIED. ) 
 CURVE ( )  GEOMETRIC_REPRESENTATION_ITEM ( )  RATIONAL_B_SPLINE_CURVE ( ( 1.000000000000000000, 0.8047378541243649375, 0.8047378541243649375, 1.000000000000000000 ) ) 
 REPRESENTATION_ITEM ( '' )  );
#43253=ORIENTED_EDGE ( 'NONE', *, *, #28511, .F. ) ;
#43256=CARTESIAN_POINT ( 'NONE',  ( -164.9459734468149463, 2.143131898507880377E-16, -160.9317124430720014 ) ) ;
#43258=FACE_OUTER_BOUND ( 'NONE', #5380, .T. ) ;
#43259=ORIENTED_EDGE ( 'NONE', *, *, #10685, .T. ) ;
#43262=( BOUNDED_CURVE ( )  B_SPLINE_CURVE ( 3, ( #41925, #22176, #22421, #25516 ),
 .UNSPECIFIED., .F., .F. ) 
 B_SPLINE_CURVE_WITH_KNOTS ( ( 4, 4 ),
 ( 0.000000000000000000, 1.570796326794896780 ),
 .UNSPECIFIED. ) 
 CURVE ( )  GEOMETRIC_REPRESENTATION_ITEM ( )  RATIONAL_B_SPLINE_CURVE ( ( 1.000000000000000000, 0.8047378541243649375, 0.8047378541243649375, 1.000000000000000000 ) ) 
 REPRESENTATION_ITEM ( '' )  );
#43265=CARTESIAN_POINT ( 'NONE',  ( -8.445973446814976526, 0.000000000000000000, 2.568287556928034121 ) ) ;
#43266=ADVANCED_FACE ( 'NONE', ( #5652 ), #13348, .T. ) ;
#43268=EDGE_CURVE ( 'NONE', #21250, #50360, #20627, .T. ) ;
#43278=CARTESIAN_POINT ( 'NONE',  ( 31.55402655318503236, 0.000000000000000000, 2.568287556927978166 ) ) ;
#43279=ORIENTED_EDGE ( 'NONE', *, *, #47915, .F. ) ;
#43280=DIRECTION ( 'NONE',  ( 0.000000000000000000, 0.000000000000000000, 1.000000000000000000 ) ) ;
#43282=EDGE_LOOP ( 'NONE', ( #26430, #411, #15707, #43480, #13752, #10117 ) ) ;
#43286=VERTEX_POINT ( 'NONE', #30274 ) ;
#43290=ORIENTED_EDGE ( 'NONE', *, *, #1396, .F. ) ;
#43293=DIRECTION ( 'NONE',  ( -1.000000000000000000, -0.000000000000000000, -0.000000000000000000 ) ) ;
#43295=ORIENTED_EDGE ( 'NONE', *, *, #44396, .F. ) ;
#43297=CYLINDRICAL_SURFACE ( 'NONE', #44784, 1.750000000000001554 ) ;
#43298=CARTESIAN_POINT ( 'NONE',  ( -6.695973446814940111, 0.000000000000000000, 165.0000000000000000 ) ) ;
#43301=ORIENTED_EDGE ( 'NONE', *, *, #43769, .F. ) ;
#43307=CARTESIAN_POINT ( 'NONE',  ( -46.69597344681494633, -1.750000000000009992, 0.8182875569279768335 ) ) ;
#43309=DIRECTION ( 'NONE',  ( -0.000000000000000000, -0.000000000000000000, -1.000000000000000000 ) ) ;
#43312=CARTESIAN_POINT ( 'NONE',  ( -206.6959734468149463, 1.750000000000010214, 40.81828755692798438 ) ) ;
#43320=CARTESIAN_POINT ( 'NONE',  ( 151.5540265531850537, 1.025126265847089657, 119.0682875569279560 ) ) ;
#43321=EDGE_LOOP ( 'NONE', ( #4177, #63, #49417, #40660, #43606, #44887 ) ) ;
#43326=CARTESIAN_POINT ( 'NONE',  ( 151.5540265531850537, 0.000000000000000000, 162.5682875569279702 ) ) ;
#43327=AXIS2_PLACEMENT_3D ( 'NONE', #49392, #10688, #34059 ) ;
#43329=CARTESIAN_POINT ( 'NONE',  ( -210.0000000000000568, 0.000000000000000000, 0.8182875569279768335 ) ) ;
#43332=( BOUNDED_CURVE ( )  B_SPLINE_CURVE ( 3, ( #1860, #13390, #44669, #2351 ),
 .UNSPECIFIED., .F., .F. ) 
 B_SPLINE_CURVE_WITH_KNOTS ( ( 4, 4 ),
 ( 3.141592653589793116, 4.712388980384689674 ),
 .UNSPECIFIED. ) 
 CURVE ( )  GEOMETRIC_REPRESENTATION_ITEM ( )  RATIONAL_B_SPLINE_CURVE ( ( 1.000000000000000000, 0.8047378541243649375, 0.8047378541243649375, 1.000000000000000000 ) ) 
 REPRESENTATION_ITEM ( '' )  );
#43333=CIRCLE ( 'NONE', #21220, 1.750000000000001554 ) ;
#43336=CARTESIAN_POINT ( 'NONE',  ( 155.0540265531850537, -1.025126265847089213, -160.9317124430720014 ) ) ;
#43346=ORIENTED_EDGE ( 'NONE', *, *, #19160, .T. ) ;
#43347=CARTESIAN_POINT ( 'NONE',  ( 210.0000000000000568, 0.000000000000000000, -119.1817124430720440 ) ) ;
#43348=DIRECTION ( 'NONE',  ( -0.000000000000000000, -0.000000000000000000, -1.000000000000000000 ) ) ;
#43349=CARTESIAN_POINT ( 'NONE',  ( 210.0000000000000568, 2.143131898507881856E-16, 79.06828755692797017 ) ) ;
#43355=DIRECTION ( 'NONE',  ( -1.000000000000000000, -0.000000000000000000, -0.000000000000000000 ) ) ;
#43360=ORIENTED_EDGE ( 'NONE', *, *, #1265, .F. ) ;
#43361=CARTESIAN_POINT ( 'NONE',  ( 210.0000000000000568, 0.000000000000000000, -117.4317124430720298 ) ) ;
#43367=ORIENTED_EDGE ( 'NONE', *, *, #4502, .F. ) ;
#43374=ORIENTED_EDGE ( 'NONE', *, *, #21239, .T. ) ;
#43377=EDGE_CURVE ( 'NONE', #20584, #29162, #42062, .T. ) ;
#43387=FACE_OUTER_BOUND ( 'NONE', #35420, .T. ) ;
#43388=EDGE_CURVE ( 'NONE', #15960, #36214, #25871, .T. ) ;
#43389=( BOUNDED_CURVE ( )  B_SPLINE_CURVE ( 3, ( #21867, #2350, #47812, #33664 ),
 .UNSPECIFIED., .F., .F. ) 
 B_SPLINE_CURVE_WITH_KNOTS ( ( 4, 4 ),
 ( 4.712388980384689674, 6.283185307179586232 ),
 .UNSPECIFIED. ) 
 CURVE ( )  GEOMETRIC_REPRESENTATION_ITEM ( )  RATIONAL_B_SPLINE_CURVE ( ( 1.000000000000000000, 0.8047378541243649375, 0.8047378541243649375, 1.000000000000000000 ) ) 
 REPRESENTATION_ITEM ( '' )  );
#43392=ORIENTED_EDGE ( 'NONE', *, *, #9536, .F. ) ;
#43393=PLANE ( 'NONE',  #31077 ) ;
#43395=LINE ( 'NONE', #4162, #34453 ) ;
#43397=( BOUNDED_CURVE ( )  B_SPLINE_CURVE ( 3, ( #16698, #43150, #39566, #31622 ),
 .UNSPECIFIED., .F., .F. ) 
 B_SPLINE_CURVE_WITH_KNOTS ( ( 4, 4 ),
 ( 3.141592653589793116, 4.712388980384689674 ),
 .UNSPECIFIED. ) 
 CURVE ( )  GEOMETRIC_REPRESENTATION_ITEM ( )  RATIONAL_B_SPLINE_CURVE ( ( 1.000000000000000000, 0.8047378541243649375, 0.8047378541243649375, 1.000000000000000000 ) ) 
 REPRESENTATION_ITEM ( '' )  );
#43398=CARTESIAN_POINT ( 'NONE',  ( 74.32915281903215998, -1.750000000000009548, 41.84341382277508359 ) ) ;
#43401=ORIENTED_EDGE ( 'NONE', *, *, #47562, .F. ) ;
#43402=AXIS2_PLACEMENT_3D ( 'NONE', #7635, #35363, #23263 ) ;
#43403=CIRCLE ( 'NONE', #13909, 1.750000000000008438 ) ;
#43404=CARTESIAN_POINT ( 'NONE',  ( 210.0000000000000568, 0.000000000000000000, -77.43171244307200141 ) ) ;
#43405=CARTESIAN_POINT ( 'NONE',  ( 210.0000000000000568, 0.000000000000000000, -119.1817124430720440 ) ) ;
#43408=DIRECTION ( 'NONE',  ( -1.000000000000000000, -0.000000000000000000, -0.000000000000000000 ) ) ;
#43409=CARTESIAN_POINT ( 'NONE',  ( 193.3040265531851105, 0.000000000000000000, 165.0000000000000000 ) ) ;
#43410=AXIS2_PLACEMENT_3D ( 'NONE', #43929, #5686, #17495 ) ;
#43417=EDGE_CURVE ( 'NONE', #21466, #29055, #41396, .T. ) ;
#43422=DIRECTION ( 'NONE',  ( 1.000000000000000000, 0.000000000000000000, 0.000000000000000000 ) ) ;
#43424=DIRECTION ( 'NONE',  ( -0.000000000000000000, -0.000000000000000000, -1.000000000000000000 ) ) ;
#43425=ADVANCED_FACE ( 'NONE', ( #29182 ), #41980, .T. ) ;
#43426=ORIENTED_EDGE ( 'NONE', *, *, #6473, .T. ) ;
#43428=EDGE_LOOP ( 'NONE', ( #15978, #28880, #48595, #34521, #48835, #46298 ) ) ;
#43431=ORIENTED_EDGE ( 'NONE', *, *, #37481, .T. ) ;
#43432=VERTEX_POINT ( 'NONE', #41475 ) ;
#43433=VERTEX_POINT ( 'NONE', #1973 ) ;
#43435=CARTESIAN_POINT ( 'NONE',  ( -6.695973446814940111, -1.750000000000024203, 120.8182875569279702 ) ) ;
#43444=ORIENTED_EDGE ( 'NONE', *, *, #5253, .T. ) ;
#43447=FACE_OUTER_BOUND ( 'NONE', #9087, .T. ) ;
#43448=CARTESIAN_POINT ( 'NONE',  ( 34.32915281903212446, -1.750000000000009548, 161.8434138227750907 ) ) ;
#43449=AXIS2_PLACEMENT_3D ( 'NONE', #10348, #19800, #47470 ) ;
#43455=ORIENTED_EDGE ( 'NONE', *, *, #39634, .F. ) ;
#43469=EDGE_CURVE ( 'NONE', #5743, #6144, #18356, .T. ) ;
#43477=ADVANCED_FACE ( 'NONE', ( #14266 ), #17619, .T. ) ;
#43480=ORIENTED_EDGE ( 'NONE', *, *, #23078, .T. ) ;
#43485=CYLINDRICAL_SURFACE ( 'NONE', #28050, 1.749999999999973799 ) ;
#43492=DIRECTION ( 'NONE',  ( 0.000000000000000000, 0.000000000000000000, -1.000000000000000000 ) ) ;
#43500=CYLINDRICAL_SURFACE ( 'NONE', #42088, 1.750000000000015543 ) ;
#43502=ORIENTED_EDGE ( 'NONE', *, *, #24252, .T. ) ;
#43504=CARTESIAN_POINT ( 'NONE',  ( 33.30402655318503946, 1.750000000000009992, -159.1817124430720298 ) ) ;
#43506=CARTESIAN_POINT ( 'NONE',  ( -86.69597344681494633, -1.750000000000010658, 120.8182875569279702 ) ) ;
#43509=CARTESIAN_POINT ( 'NONE',  ( 152.2789002873379900, -1.750000000000009548, -40.20683870891912193 ) ) ;
#43511=CARTESIAN_POINT ( 'NONE',  ( -4.945973446814903696, 2.143131898507913410E-16, 165.0000000000000000 ) ) ;
#43512=CARTESIAN_POINT ( 'NONE',  ( 191.5540265531850537, 1.025126265847089657, -120.9317124430720440 ) ) ;
#43516=DIRECTION ( 'NONE',  ( -1.000000000000000000, -0.000000000000000000, -0.000000000000000000 ) ) ;
#43517=VECTOR ( 'NONE', #48484, 1000.000000000000000 ) ;
#43521=EDGE_CURVE ( 'NONE', #29044, #36853, #38115, .T. ) ;
#43522=ORIENTED_EDGE ( 'NONE', *, *, #16957, .F. ) ;
#43523=DIRECTION ( 'NONE',  ( -0.000000000000000000, -0.000000000000000000, -1.000000000000000000 ) ) ;
#43524=CARTESIAN_POINT ( 'NONE',  ( -88.44597344681497475, 0.000000000000000000, 159.0682875569279418 ) ) ;
#43529=ORIENTED_EDGE ( 'NONE', *, *, #20537, .F. ) ;
#43532=ORIENTED_EDGE ( 'NONE', *, *, #2352, .T. ) ;
#43533=ORIENTED_EDGE ( 'NONE', *, *, #26768, .F. ) ;
#43535=DIRECTION ( 'NONE',  ( 0.000000000000000000, 0.000000000000000000, -1.000000000000000000 ) ) ;
#43536=( BOUNDED_CURVE ( )  B_SPLINE_CURVE ( 3, ( #45890, #30041, #22071, #34393 ),
 .UNSPECIFIED., .F., .F. ) 
 B_SPLINE_CURVE_WITH_KNOTS ( ( 4, 4 ),
 ( 4.712388980384689674, 6.283185307179586232 ),
 .UNSPECIFIED. ) 
 CURVE ( )  GEOMETRIC_REPRESENTATION_ITEM ( )  RATIONAL_B_SPLINE_CURVE ( ( 1.000000000000000000, 0.8047378541243649375, 0.8047378541243649375, 1.000000000000000000 ) ) 
 REPRESENTATION_ITEM ( '' )  );
#43541=CARTESIAN_POINT ( 'NONE',  ( -164.9459734468149463, 2.143131898507880377E-16, 39.06828755692798438 ) ) ;
#43542=ORIENTED_EDGE ( 'NONE', *, *, #314, .T. ) ;
#43543=( BOUNDED_CURVE ( )  B_SPLINE_CURVE ( 3, ( #38559, #15689, #26985, #7500 ),
 .UNSPECIFIED., .F., .F. ) 
 B_SPLINE_CURVE_WITH_KNOTS ( ( 4, 4 ),
 ( 0.000000000000000000, 1.570796326794896558 ),
 .UNSPECIFIED. ) 
 CURVE ( )  GEOMETRIC_REPRESENTATION_ITEM ( )  RATIONAL_B_SPLINE_CURVE ( ( 1.000000000000000000, 0.8047378541243649375, 0.8047378541243649375, 1.000000000000000000 ) ) 
 REPRESENTATION_ITEM ( '' )  );
#43547=ORIENTED_EDGE ( 'NONE', *, *, #11750, .T. ) ;
#43550=CARTESIAN_POINT ( 'NONE',  ( -84.94597344681494633, 2.143131898507880377E-16, -120.9317124430720156 ) ) ;
#43554=DIRECTION ( 'NONE',  ( -1.000000000000000000, -0.000000000000000000, -0.000000000000000000 ) ) ;
#43556=EDGE_LOOP ( 'NONE', ( #36199, #30852, #44575, #41359, #30428, #27509 ) ) ;
#43557=ORIENTED_EDGE ( 'NONE', *, *, #23803, .F. ) ;
#43559=CARTESIAN_POINT ( 'NONE',  ( 193.3040265531851105, 1.750000000000010658, 80.81828755692798438 ) ) ;
#43561=( BOUNDED_CURVE ( )  B_SPLINE_CURVE ( 3, ( #49069, #21663, #25025, #25774 ),
 .UNSPECIFIED., .F., .F. ) 
 B_SPLINE_CURVE_WITH_KNOTS ( ( 4, 4 ),
 ( 4.712388980384689674, 6.283185307179586232 ),
 .UNSPECIFIED. ) 
 CURVE ( )  GEOMETRIC_REPRESENTATION_ITEM ( )  RATIONAL_B_SPLINE_CURVE ( ( 1.000000000000000000, 0.8047378541243649375, 0.8047378541243649375, 1.000000000000000000 ) ) 
 REPRESENTATION_ITEM ( '' )  );
#43564=ORIENTED_EDGE ( 'NONE', *, *, #11444, .F. ) ;
#43565=CARTESIAN_POINT ( 'NONE',  ( 31.55402655318506788, 0.000000000000000000, 162.5682875569279702 ) ) ;
#43567=CARTESIAN_POINT ( 'NONE',  ( -208.4459734468149463, 0.000000000000000000, 165.0000000000000000 ) ) ;
#43569=CARTESIAN_POINT ( 'NONE',  ( -86.69597344681494633, 1.750000000000009992, 160.8182875569279702 ) ) ;
#43571=CARTESIAN_POINT ( 'NONE',  ( 210.0000000000000568, 2.143131898507880377E-16, -0.9317124430720331585 ) ) ;
#43574=CARTESIAN_POINT ( 'NONE',  ( -46.69597344681494633, 0.000000000000000000, -165.0000000000000000 ) ) ;
#43587=ORIENTED_EDGE ( 'NONE', *, *, #15885, .F. ) ;
#43593=CARTESIAN_POINT ( 'NONE',  ( 111.5540265531850679, 0.000000000000000000, -120.9317124430720156 ) ) ;
#43594=ORIENTED_EDGE ( 'NONE', *, *, #25262, .F. ) ;
#43597=VERTEX_POINT ( 'NONE', #49811 ) ;
#43599=DIRECTION ( 'NONE',  ( -0.000000000000000000, -0.000000000000000000, -1.000000000000000000 ) ) ;
#43600=ORIENTED_EDGE ( 'NONE', *, *, #45666, .F. ) ;
#43602=CARTESIAN_POINT ( 'NONE',  ( -4.945973446814903696, 2.143131898507912917E-16, -37.43171244307200141 ) ) ;
#43606=ORIENTED_EDGE ( 'NONE', *, *, #29206, .F. ) ;
#43609=CARTESIAN_POINT ( 'NONE',  ( 113.3040265531850537, 1.749999999999996891, -159.1817124430720298 ) ) ;
#43612=ORIENTED_EDGE ( 'NONE', *, *, #28048, .F. ) ;
#43614=EDGE_CURVE ( 'NONE', #35055, #9213, #39468, .T. ) ;
#43615=VECTOR ( 'NONE', #30130, 1000.000000000000000 ) ;
#43619=CARTESIAN_POINT ( 'NONE',  ( -204.9459734468149463, 2.143131898507880377E-16, 82.56828755692798438 ) ) ;
#43622=ORIENTED_EDGE ( 'NONE', *, *, #24834, .T. ) ;
#43625=CARTESIAN_POINT ( 'NONE',  ( 75.05402655318509630, 2.143131898507880377E-16, 79.06828755692797017 ) ) ;
#43626=ORIENTED_EDGE ( 'NONE', *, *, #32564, .T. ) ;
#43630=CARTESIAN_POINT ( 'NONE',  ( 210.0000000000000568, 0.000000000000000000, 40.81828755692798438 ) ) ;
#43633=DIRECTION ( 'NONE',  ( -1.000000000000000000, -0.000000000000000000, -0.000000000000000000 ) ) ;
#43635=CARTESIAN_POINT ( 'NONE',  ( -168.4459734468149463, 0.000000000000000000, 165.0000000000000000 ) ) ;
#43638=CARTESIAN_POINT ( 'NONE',  ( 113.3040265531850537, -1.749999999999996891, 0.8182875569279768335 ) ) ;
#43642=CARTESIAN_POINT ( 'NONE',  ( 114.3291528190321173, -1.749999999999996891, -40.20683870891911482 ) ) ;
#43647=FACE_OUTER_BOUND ( 'NONE', #41702, .T. ) ;
#43658=CARTESIAN_POINT ( 'NONE',  ( -206.6959734468149463, -1.750000000000009992, 0.8182875569279768335 ) ) ;
#43661=CARTESIAN_POINT ( 'NONE',  ( 112.2789002873379758, -1.749999999999996891, -118.1565861772249661 ) ) ;
#43667=CARTESIAN_POINT ( 'NONE',  ( 194.3291528190321742, 1.750000000000010214, 79.79316129108087807 ) ) ;
#43670=CYLINDRICAL_SURFACE ( 'NONE', #30836, 1.749999999999973799 ) ;
#43676=ORIENTED_EDGE ( 'NONE', *, *, #1502, .F. ) ;
#43686=VECTOR ( 'NONE', #11037, 1000.000000000000000 ) ;
#43687=LINE ( 'NONE', #4946, #1263 ) ;
#43688=ORIENTED_EDGE ( 'NONE', *, *, #29011, .F. ) ;
#43691=( BOUNDED_CURVE ( )  B_SPLINE_CURVE ( 3, ( #2917, #34246, #41430, #7045 ),
 .UNSPECIFIED., .F., .F. ) 
 B_SPLINE_CURVE_WITH_KNOTS ( ( 4, 4 ),
 ( 3.141592653589793116, 4.712388980384689674 ),
 .UNSPECIFIED. ) 
 CURVE ( )  GEOMETRIC_REPRESENTATION_ITEM ( )  RATIONAL_B_SPLINE_CURVE ( ( 1.000000000000000000, 0.8047378541243649375, 0.8047378541243649375, 1.000000000000000000 ) ) 
 REPRESENTATION_ITEM ( '' )  );
#43693=AXIS2_PLACEMENT_3D ( 'NONE', #25412, #33376, #29510 ) ;
#43696=CARTESIAN_POINT ( 'NONE',  ( -126.6959734468149321, -1.749999999999997335, 80.81828755692798438 ) ) ;
#43698=ORIENTED_EDGE ( 'NONE', *, *, #17490, .T. ) ;
#43700=( BOUNDED_CURVE ( )  B_SPLINE_CURVE ( 3, ( #28561, #40123, #39881, #47266 ),
 .UNSPECIFIED., .F., .F. ) 
 B_SPLINE_CURVE_WITH_KNOTS ( ( 4, 4 ),
 ( 0.000000000000000000, 1.570796326794896558 ),
 .UNSPECIFIED. ) 
 CURVE ( )  GEOMETRIC_REPRESENTATION_ITEM ( )  RATIONAL_B_SPLINE_CURVE ( ( 1.000000000000000000, 0.8047378541243649375, 0.8047378541243649375, 1.000000000000000000 ) ) 
 REPRESENTATION_ITEM ( '' )  );
#43702=CARTESIAN_POINT ( 'NONE',  ( 153.3040265531850537, 0.000000000000000000, 165.0000000000000000 ) ) ;
#43703=DIRECTION ( 'NONE',  ( 0.000000000000000000, 0.000000000000000000, 1.000000000000000000 ) ) ;
#43706=EDGE_CURVE ( 'NONE', #20580, #49549, #20020, .T. ) ;
#43712=ORIENTED_EDGE ( 'NONE', *, *, #9831, .F. ) ;
#43716=CARTESIAN_POINT ( 'NONE',  ( 191.5540265531850537, 1.025126265847088991, 2.568287556927986159 ) ) ;
#43718=FACE_OUTER_BOUND ( 'NONE', #37790, .T. ) ;
#43722=ORIENTED_EDGE ( 'NONE', *, *, #28417, .T. ) ;
#43732=CARTESIAN_POINT ( 'NONE',  ( -47.72109971266203132, 1.750000000000009548, -38.15658617722494483 ) ) ;
#43733=CARTESIAN_POINT ( 'NONE',  ( 35.05402655318504657, 1.025126265847089657, 42.56828755692799149 ) ) ;
#43735=DIRECTION ( 'NONE',  ( -0.000000000000000000, -0.000000000000000000, -1.000000000000000000 ) ) ;
#43740=ADVANCED_FACE ( 'NONE', ( #48503 ), #1611, .T. ) ;
#43746=VERTEX_POINT ( 'NONE', #40846 ) ;
#43750=ORIENTED_EDGE ( 'NONE', *, *, #1859, .F. ) ;
#43754=ORIENTED_EDGE ( 'NONE', *, *, #37164, .F. ) ;
#43755=CARTESIAN_POINT ( 'NONE',  ( 210.0000000000000568, 2.143131898507881856E-16, 119.0682875569279560 ) ) ;
#43756=CARTESIAN_POINT ( 'NONE',  ( -208.4459734468148611, 1.025126265847089435, 122.5682875569280128 ) ) ;
#43758=VECTOR ( 'NONE', #47926, 1000.000000000000000 ) ;
#43761=DIRECTION ( 'NONE',  ( -1.000000000000000000, 0.000000000000000000, 0.000000000000000000 ) ) ;
#43762=VERTEX_POINT ( 'NONE', #32655 ) ;
#43765=CYLINDRICAL_SURFACE ( 'NONE', #11763, 1.750000000000001554 ) ;
#43766=DIRECTION ( 'NONE',  ( 0.000000000000000000, 0.000000000000000000, 1.000000000000000000 ) ) ;
#43767=CARTESIAN_POINT ( 'NONE',  ( -88.44597344681497475, 0.000000000000000000, 165.0000000000000000 ) ) ;
#43769=EDGE_CURVE ( 'NONE', #16395, #22572, #17994, .T. ) ;
#43770=ADVANCED_FACE ( 'NONE', ( #29551 ), #40607, .T. ) ;
#43773=EDGE_CURVE ( 'NONE', #15646, #15638, #43332, .T. ) ;
#43777=ORIENTED_EDGE ( 'NONE', *, *, #16558, .T. ) ;
#43783=VERTEX_POINT ( 'NONE', #49256 ) ;
#43784=CARTESIAN_POINT ( 'NONE',  ( 193.3040265531851105, 1.750000000000010658, -119.1817124430720440 ) ) ;
#43787=DIRECTION ( 'NONE',  ( -1.000000000000000000, -0.000000000000000000, -0.000000000000000000 ) ) ;
#43794=VERTEX_POINT ( 'NONE', #21597 ) ;
#43796=ORIENTED_EDGE ( 'NONE', *, *, #4877, .F. ) ;
#43798=CARTESIAN_POINT ( 'NONE',  ( -86.69597344681494633, -1.750000000000010214, 40.81828755692798438 ) ) ;
#43800=DIRECTION ( 'NONE',  ( 0.000000000000000000, 0.000000000000000000, 1.000000000000000000 ) ) ;
#43801=ORIENTED_EDGE ( 'NONE', *, *, #31944, .F. ) ;
#43806=ORIENTED_EDGE ( 'NONE', *, *, #33839, .F. ) ;
#43808=EDGE_CURVE ( 'NONE', #42453, #43432, #34515, .T. ) ;
#43812=CARTESIAN_POINT ( 'NONE',  ( 210.0000000000000568, 0.000000000000000000, 40.81828755692798438 ) ) ;
#43813=CARTESIAN_POINT ( 'NONE',  ( 193.3040265531851105, 1.750000000000010658, -79.18171244307201562 ) ) ;
#43815=VECTOR ( 'NONE', #23013, 1000.000000000000000 ) ;
#43820=DIRECTION ( 'NONE',  ( -1.000000000000000000, 0.000000000000000000, 0.000000000000000000 ) ) ;
#43829=CARTESIAN_POINT ( 'NONE',  ( -204.9459734468149463, 2.143131898507880377E-16, 159.0682875569279702 ) ) ;
#43833=VECTOR ( 'NONE', #14022, 1000.000000000000000 ) ;
#43837=( BOUNDED_CURVE ( )  B_SPLINE_CURVE ( 3, ( #35220, #15445, #27256, #23135 ),
 .UNSPECIFIED., .F., .F. ) 
 B_SPLINE_CURVE_WITH_KNOTS ( ( 4, 4 ),
 ( 0.000000000000000000, 1.570796326794896558 ),
 .UNSPECIFIED. ) 
 CURVE ( )  GEOMETRIC_REPRESENTATION_ITEM ( )  RATIONAL_B_SPLINE_CURVE ( ( 1.000000000000000000, 0.8047378541243649375, 0.8047378541243649375, 1.000000000000000000 ) ) 
 REPRESENTATION_ITEM ( '' )  );
#43844=CARTESIAN_POINT ( 'NONE',  ( -45.67084718096785423, 1.750000000000009548, -0.2068387089191121020 ) ) ;
#43845=( BOUNDED_CURVE ( )  B_SPLINE_CURVE ( 3, ( #36697, #40767, #1521, #13551 ),
 .UNSPECIFIED., .F., .F. ) 
 B_SPLINE_CURVE_WITH_KNOTS ( ( 4, 4 ),
 ( 1.570796326794896558, 3.141592653589793116 ),
 .UNSPECIFIED. ) 
 CURVE ( )  GEOMETRIC_REPRESENTATION_ITEM ( )  RATIONAL_B_SPLINE_CURVE ( ( 1.000000000000000000, 0.8047378541243649375, 0.8047378541243649375, 1.000000000000000000 ) ) 
 REPRESENTATION_ITEM ( '' )  );
#43846=ADVANCED_FACE ( 'NONE', ( #15425 ), #26967, .T. ) ;
#43847=VERTEX_POINT ( 'NONE', #41608 ) ;
#43851=EDGE_LOOP ( 'NONE', ( #42150, #24343 ) ) ;
#43853=CARTESIAN_POINT ( 'NONE',  ( 111.5540265531850679, 0.000000000000000000, 165.0000000000000000 ) ) ;
#43854=CIRCLE ( 'NONE', #13527, 1.750000000000015543 ) ;
#43855=ORIENTED_EDGE ( 'NONE', *, *, #17834, .F. ) ;
#43859=( BOUNDED_CURVE ( )  B_SPLINE_CURVE ( 3, ( #32984, #10115, #33982, #41670 ),
 .UNSPECIFIED., .F., .F. ) 
 B_SPLINE_CURVE_WITH_KNOTS ( ( 4, 4 ),
 ( 0.000000000000000000, 1.570796326794896558 ),
 .UNSPECIFIED. ) 
 CURVE ( )  GEOMETRIC_REPRESENTATION_ITEM ( )  RATIONAL_B_SPLINE_CURVE ( ( 1.000000000000000000, 0.8047378541243649375, 0.8047378541243649375, 1.000000000000000000 ) ) 
 REPRESENTATION_ITEM ( '' )  );
#43863=VERTEX_POINT ( 'NONE', #2593 ) ;
#43866=CARTESIAN_POINT ( 'NONE',  ( 154.3291528190321458, -1.750000000000009548, 41.84341382277508359 ) ) ;
#43868=ORIENTED_EDGE ( 'NONE', *, *, #29003, .T. ) ;
#43870=( GEOMETRIC_REPRESENTATION_CONTEXT ( 3 ) GLOBAL_UNCERTAINTY_ASSIGNED_CONTEXT ( ( #15216 ) ) GLOBAL_UNIT_ASSIGNED_CONTEXT ( ( #32165, #4949, #5458 ) ) REPRESENTATION_CONTEXT ( 'NONE', 'WORKASPACE' ) );
#43877=CARTESIAN_POINT ( 'NONE',  ( 210.0000000000000568, 0.000000000000000000, 162.5682875569279702 ) ) ;
#43880=DIRECTION ( 'NONE',  ( -1.000000000000000000, 0.000000000000000000, 0.000000000000000000 ) ) ;
#43884=VERTEX_POINT ( 'NONE', #46686 ) ;
#43893=AXIS2_PLACEMENT_3D ( 'NONE', #42438, #6794, #38620 ) ;
#43899=CARTESIAN_POINT ( 'NONE',  ( 151.5540265531850537, 1.025126265847089435, -40.93171244307204404 ) ) ;
#43904=EDGE_CURVE ( 'NONE', #29317, #45409, #30831, .T. ) ;
#43905=CARTESIAN_POINT ( 'NONE',  ( -206.6959734468149463, 1.750000000000009992, 160.8182875569279702 ) ) ;
#43908=ORIENTED_EDGE ( 'NONE', *, *, #20903, .T. ) ;
#43916=DIRECTION ( 'NONE',  ( -1.000000000000000000, -0.000000000000000000, -0.000000000000000000 ) ) ;
#43917=ORIENTED_EDGE ( 'NONE', *, *, #38385, .T. ) ;
#43918=ORIENTED_EDGE ( 'NONE', *, *, #7021, .F. ) ;
#43921=ORIENTED_EDGE ( 'NONE', *, *, #39498, .T. ) ;
#43929=CARTESIAN_POINT ( 'NONE',  ( 210.0000000000000568, 0.000000000000000000, 40.81828755692798438 ) ) ;
#43930=DIRECTION ( 'NONE',  ( -0.000000000000000000, -0.000000000000000000, -1.000000000000000000 ) ) ;
#43938=ORIENTED_EDGE ( 'NONE', *, *, #17337, .F. ) ;
#43940=CARTESIAN_POINT ( 'NONE',  ( 115.0540265531850395, -1.025126265847081664, -117.4317124430720440 ) ) ;
#43942=ORIENTED_EDGE ( 'NONE', *, *, #40094, .F. ) ;
#43943=CARTESIAN_POINT ( 'NONE',  ( 113.3040265531850537, 1.749999999999996891, 160.8182875569279702 ) ) ;
#43946=DIRECTION ( 'NONE',  ( -0.000000000000000000, -0.000000000000000000, -1.000000000000000000 ) ) ;
#43947=VERTEX_POINT ( 'NONE', #49760 ) ;
#43957=CARTESIAN_POINT ( 'NONE',  ( -84.94597344681494633, 2.143131898507880377E-16, 42.56828755692798438 ) ) ;
#43963=EDGE_CURVE ( 'NONE', #31470, #49119, #30573, .T. ) ;
#43970=EDGE_CURVE ( 'NONE', #7277, #46718, #38788, .T. ) ;
#43981=CARTESIAN_POINT ( 'NONE',  ( -124.9459734468149463, 2.143131898507847836E-16, 165.0000000000000000 ) ) ;
#43982=CYLINDRICAL_SURFACE ( 'NONE', #14937, 1.750000000000010214 ) ;
#43986=EDGE_CURVE ( 'NONE', #13983, #26888, #41693, .T. ) ;
#43987=EDGE_CURVE ( 'NONE', #38451, #50334, #30928, .T. ) ;
#43996=( BOUNDED_CURVE ( )  B_SPLINE_CURVE ( 3, ( #5463, #44196, #29073, #24222 ),
 .UNSPECIFIED., .F., .F. ) 
 B_SPLINE_CURVE_WITH_KNOTS ( ( 4, 4 ),
 ( 4.712388980384689674, 6.283185307179586232 ),
 .UNSPECIFIED. ) 
 CURVE ( )  GEOMETRIC_REPRESENTATION_ITEM ( )  RATIONAL_B_SPLINE_CURVE ( ( 1.000000000000000000, 0.8047378541243649375, 0.8047378541243649375, 1.000000000000000000 ) ) 
 REPRESENTATION_ITEM ( '' )  );
#43997=CARTESIAN_POINT ( 'NONE',  ( -86.69597344681496054, 0.000000000000000000, 165.0000000000000000 ) ) ;
#43999=ORIENTED_EDGE ( 'NONE', *, *, #28778, .F. ) ;
#44002=CARTESIAN_POINT ( 'NONE',  ( 73.30402655318508209, 0.000000000000000000, 165.0000000000000000 ) ) ;
#44004=LINE ( 'NONE', #5271, #41797 ) ;
#44005=DIRECTION ( 'NONE',  ( -0.000000000000000000, -0.000000000000000000, -1.000000000000000000 ) ) ;
#44006=ORIENTED_EDGE ( 'NONE', *, *, #30342, .F. ) ;
#44008=DIRECTION ( 'NONE',  ( 0.000000000000000000, 0.000000000000000000, 1.000000000000000000 ) ) ;
#44014=EDGE_CURVE ( 'NONE', #8314, #16057, #1401, .T. ) ;
#44022=CARTESIAN_POINT ( 'NONE',  ( 210.0000000000000568, 0.000000000000000000, 80.81828755692798438 ) ) ;
#44023=VERTEX_POINT ( 'NONE', #12087 ) ;
#44026=CARTESIAN_POINT ( 'NONE',  ( 31.55402655318503236, -1.025126265847089435, 2.568287556927986159 ) ) ;
#44027=ORIENTED_EDGE ( 'NONE', *, *, #37207, .T. ) ;
#44028=CARTESIAN_POINT ( 'NONE',  ( 210.0000000000000568, 0.000000000000000000, 120.8182875569279702 ) ) ;
#44032=LINE ( 'NONE', #12241, #27927 ) ;
#44034=CARTESIAN_POINT ( 'NONE',  ( 32.27890028733795447, 1.750000000000010436, 79.79316129108087807 ) ) ;
#44040=ADVANCED_FACE ( 'NONE', ( #42859 ), #27485, .T. ) ;
#44045=LINE ( 'NONE', #8912, #9508 ) ;
#44048=EDGE_CURVE ( 'NONE', #45429, #45821, #36164, .T. ) ;
#44051=ORIENTED_EDGE ( 'NONE', *, *, #41129, .T. ) ;
#44059=CARTESIAN_POINT ( 'NONE',  ( 33.30402655318503946, 1.750000000000010658, -79.18171244307201562 ) ) ;
#44061=CARTESIAN_POINT ( 'NONE',  ( 210.0000000000000568, 0.000000000000000000, 120.8182875569279702 ) ) ;
#44063=CARTESIAN_POINT ( 'NONE',  ( 210.0000000000000568, 0.000000000000000000, -79.18171244307201562 ) ) ;
#44065=CARTESIAN_POINT ( 'NONE',  ( 113.3040265531850537, -1.749999999999997335, -119.1817124430720440 ) ) ;
#44066=CARTESIAN_POINT ( 'NONE',  ( -204.9459734468148895, -1.025126265847089657, -80.93171244307201562 ) ) ;
#44068=CYLINDRICAL_SURFACE ( 'NONE', #6773, 1.750000000000015543 ) ;
#44069=CARTESIAN_POINT ( 'NONE',  ( -124.9459734468149463, 2.143131898507847836E-16, 119.0682875569279844 ) ) ;
#44070=LINE ( 'NONE', #6095, #25507 ) ;
#44072=EDGE_CURVE ( 'NONE', #39708, #24104, #6624, .T. ) ;
#44073=( BOUNDED_CURVE ( )  B_SPLINE_CURVE ( 3, ( #2222, #24565, #25316, #37146 ),
 .UNSPECIFIED., .F., .F. ) 
 B_SPLINE_CURVE_WITH_KNOTS ( ( 4, 4 ),
 ( 1.570796326794896558, 3.141592653589793116 ),
 .UNSPECIFIED. ) 
 CURVE ( )  GEOMETRIC_REPRESENTATION_ITEM ( )  RATIONAL_B_SPLINE_CURVE ( ( 1.000000000000000000, 0.8047378541243649375, 0.8047378541243649375, 1.000000000000000000 ) ) 
 REPRESENTATION_ITEM ( '' )  );
#44089=DIRECTION ( 'NONE',  ( -0.000000000000000000, -0.000000000000000000, -1.000000000000000000 ) ) ;
#44093=ORIENTED_EDGE ( 'NONE', *, *, #32738, .T. ) ;
#44094=CARTESIAN_POINT ( 'NONE',  ( -206.6959734468149463, 0.000000000000000000, 165.0000000000000000 ) ) ;
#44095=EDGE_CURVE ( 'NONE', #3325, #8469, #37820, .T. ) ;
#44103=ADVANCED_FACE ( 'NONE', ( #41295 ), #44119, .T. ) ;
#44104=VERTEX_POINT ( 'NONE', #24650 ) ;
#44108=ORIENTED_EDGE ( 'NONE', *, *, #28149, .T. ) ;
#44113=ORIENTED_EDGE ( 'NONE', *, *, #3765, .T. ) ;
#44117=CARTESIAN_POINT ( 'NONE',  ( 151.5540265531850537, 1.025126265847088991, -157.4317124430720582 ) ) ;
#44118=EDGE_CURVE ( 'NONE', #214, #38516, #29256, .T. ) ;
#44119=PLANE ( 'NONE',  #6699 ) ;
#44121=CARTESIAN_POINT ( 'NONE',  ( -5.670847180967843570, 1.750000000000023315, -40.20683870891912903 ) ) ;
#44126=ORIENTED_EDGE ( 'NONE', *, *, #6890, .F. ) ;
#44127=SHAPE_DEFINITION_REPRESENTATION ( #30252, #50327 ) ;
#44130=( BOUNDED_CURVE ( )  B_SPLINE_CURVE ( 3, ( #5285, #47593, #9137, #40448 ),
 .UNSPECIFIED., .F., .F. ) 
 B_SPLINE_CURVE_WITH_KNOTS ( ( 4, 4 ),
 ( 4.712388980384689674, 6.283185307179586232 ),
 .UNSPECIFIED. ) 
 CURVE ( )  GEOMETRIC_REPRESENTATION_ITEM ( )  RATIONAL_B_SPLINE_CURVE ( ( 1.000000000000000000, 0.8047378541243649375, 0.8047378541243649375, 1.000000000000000000 ) ) 
 REPRESENTATION_ITEM ( '' )  );
#44134=CARTESIAN_POINT ( 'NONE',  ( -128.4459734468149463, -1.025126265847082108, 82.56828755692798438 ) ) ;
#44140=CARTESIAN_POINT ( 'NONE',  ( -86.69597344681494633, 1.750000000000010658, 80.81828755692798438 ) ) ;
#44141=CLOSED_SHELL ( 'NONE', ( #13547, #38395, #43477, #14569, #2413, #33993, #18896, #8537, #45560, #49789, #31065, #5764, #3401, #48213, #9887, #24613, #48966, #18612, #40282, #40726, #48728, #48698, #7394, #9388, #23439, #32513, #45952, #30027, #27230, #47226, #27119, #37554, #5739, #45556, #48759, #37603, #10645, #49963, #7317, #12495, #23934, #22417, #48486, #38747, #35352, #28717, #7352, #14854, #12699, #21311, #31576, #48444, #8341, #21060, #48639, #27618, #37558, #2688, #45213, #7246, #45568, #28942, #50137, #18962, #13950, #1798, #3273, #19401, #30403, #24445, #48725, #39757, #26427, #26860, #29301, #7784, #40940, #11739, #22707, #18453, #31862, #31231, #30445, #21002, #5735, #27499, #38159, #15355, #31360, #7825, #194, #44922, #44040, #20035, #23086, #29324, #43425, #19039, #39635, #26004, #26717, #45521, #20853, #16255, #2148, #34609, #20791, #17215, #12662, #25594, #45922, #27075, #37828, #32473, #20250, #49947, #1125, #36942, #33484, #2939, #7365, #24603, #15479, #8216, #39888, #32275, #11229, #18464, #32414, #42425, #37895, #16847, #2293, #4286, #12696, #50623, #10140, #13000, #3294, #10146, #34016, #7724, #12124, #47574, #29746, #46010, #1786, #40594, #15920, #34770, #32140, #14320, #30579, #38603, #40225, #20475, #37735, #452, #2317, #49591, #22668, #43266, #13298, #25654, #39179, #30195, #604, #15573, #37959, #26568, #143, #5178, #18499, #29315, #7964, #2353, #2699, #28038, #21856, #12994, #34129, #10086, #1994, #8760, #36198, #47281, #27266, #20502, #2003, #2892, #45871, #39972, #43213, #36230, #42766, #27446, #34101, #3564, #37277, #47635, #7774, #25123, #37969, #45411, #26442, #14829, #19545, #45367, #6671, #48925, #49414, #43203, #4221, #25929, #30544, #40723, #34673, #9962, #21900, #15178, #7827, #15866, #35050, #41348, #13770, #49302, #13363, #653, #39044, #232, #34301, #45247, #36567, #33341, #18586, #23976, #39720, #30079, #7762, #19575, #5780, #38716, #35601, #22006, #815, #12751, #1996, #47175, #9591, #703, #11390, #25065, #23386, #26115, #33420, #5201, #4975, #49702, #14930, #36174, #10018, #8456, #49266, #21487, #43770, #38674, #18409, #46708, #31837, #3710, #45074, #34011, #38887, #45753, #37557, #19781, #28072, #38253, #4531, #24876, #41498, #18395, #9257, #44387, #3260, #9246, #32570, #23709, #11453, #5593, #182, #25550, #2983, #48105, #27784, #20965, #3289, #36496, #801, #22452, #22044, #10941, #3593, #25099, #32312, #6891, #49064, #9173, #47905, #27352, #12374, #34017, #16500, #40670, #47205, #9278, #13747, #31992, #3328, #45672, #38685, #33218, #48970, #526, #43740, #29363, #5592, #25656, #40556, #12628, #8328, #47, #38824, #581, #41990, #18496, #23047, #19229, #35990, #44103, #47213, #23639, #39967, #4967, #41510, #44678, #23066, #44399, #31137, #39016, #45900, #20571, #18920, #30581, #41504, #20177, #14209, #26167, #24607, #27201, #11304, #14355, #47752, #35412, #19876, #13419, #19837, #36917, #14642, #31153, #46253, #40997, #17949, #35646, #944, #45875, #37958, #12967, #30997, #29261, #12965, #32544, #15570, #42022, #38736, #2940, #9758, #46807, #28446, #48236, #20594, #26426, #47441, #46866, #29613, #18902, #48788, #43846, #10484, #30717, #22478, #8297, #15524, #27238, #7120, #34134, #24610, #11951, #23342, #22522, #29346, #15152, #36848, #19263, #3948, #41341, #40418, #22397, #5475, #16541, #29579, #45505, #31651, #16624, #48831, #23949, #8883, #24007, #2013, #2440, #46734, #6814, #23460, #15220, #10541, #22457, #42767, #39355, #41045, #41209, #30929, #25674, #50315, #24894, #34271, #49898, #45896, #44180, #10252, #39017, #19411, #38394, #28085, #49339, #45314, #45432, #21178, #13760, #21119, #23156, #8669, #48148, #6165, #29998, #37175, #10774, #29364, #15531, #13067, #8153, #40373, #13206, #44568, #39521, #40034, #28975 ) ) ;
#44149=CARTESIAN_POINT ( 'NONE',  ( -205.6708471809678827, 1.750000000000010214, -120.2068387089191219 ) ) ;
#44150=CYLINDRICAL_SURFACE ( 'NONE', #22411, 1.750000000000015543 ) ;
#44154=CARTESIAN_POINT ( 'NONE',  ( -6.695973446814940111, 1.750000000000024203, -79.18171244307201562 ) ) ;
#44155=EDGE_LOOP ( 'NONE', ( #48058, #41982, #38285, #24905, #5415 ) ) ;
#44162=EDGE_LOOP ( 'NONE', ( #5472, #27561, #11364, #4781, #46687, #13055 ) ) ;
#44163=DIRECTION ( 'NONE',  ( -1.000000000000000000, -0.000000000000000000, -0.000000000000000000 ) ) ;
#44165=EDGE_CURVE ( 'NONE', #46611, #1904, #24896, .T. ) ;
#44166=AXIS2_PLACEMENT_3D ( 'NONE', #42625, #50538, #35215 ) ;
#44167=ORIENTED_EDGE ( 'NONE', *, *, #48154, .T. ) ;
#44170=CARTESIAN_POINT ( 'NONE',  ( 193.3040265531851105, -1.750000000000010214, 40.81828755692798438 ) ) ;
#44171=CARTESIAN_POINT ( 'NONE',  ( 33.30402655318503946, -1.750000000000010658, -119.1817124430720440 ) ) ;
#44173=CARTESIAN_POINT ( 'NONE',  ( -128.4459734468149463, 1.025126265847081886, -120.9317124430720440 ) ) ;
#44177=CARTESIAN_POINT ( 'NONE',  ( 210.0000000000000568, 0.000000000000000000, -77.43171244307200141 ) ) ;
#44179=FACE_OUTER_BOUND ( 'NONE', #32152, .T. ) ;
#44180=ADVANCED_FACE ( 'NONE', ( #17695 ), #33360, .T. ) ;
#44183=VERTEX_POINT ( 'NONE', #34366 ) ;
#44184=ORIENTED_EDGE ( 'NONE', *, *, #43004, .F. ) ;
#44189=EDGE_LOOP ( 'NONE', ( #24277, #13442, #36596, #21026, #32959, #47652 ) ) ;
#44195=CARTESIAN_POINT ( 'NONE',  ( 210.0000000000000568, 2.143131898507881856E-16, -120.9317124430720582 ) ) ;
#44196=CARTESIAN_POINT ( 'NONE',  ( -45.67084718096785423, -1.750000000000010436, 119.7931612910808781 ) ) ;
#44199=CARTESIAN_POINT ( 'NONE',  ( -8.445973446814976526, 0.000000000000000000, 165.0000000000000000 ) ) ;
#44203=VECTOR ( 'NONE', #6421, 1000.000000000000000 ) ;
#44209=CARTESIAN_POINT ( 'NONE',  ( 71.55402655318505367, 0.000000000000000000, -80.93171244307204404 ) ) ;
#44210=VERTEX_POINT ( 'NONE', #23049 ) ;
#44214=EDGE_CURVE ( 'NONE', #28470, #25557, #34216, .T. ) ;
#44215=ORIENTED_EDGE ( 'NONE', *, *, #4904, .F. ) ;
#44216=CARTESIAN_POINT ( 'NONE',  ( -126.6959734468149321, 1.749999999999997113, -39.18171244307202983 ) ) ;
#44219=CARTESIAN_POINT ( 'NONE',  ( -210.0000000000000568, 0.000000000000000000, 120.8182875569279702 ) ) ;
#44220=EDGE_LOOP ( 'NONE', ( #19927, #3417, #24375, #17, #17366, #40969 ) ) ;
#44221=ORIENTED_EDGE ( 'NONE', *, *, #22115, .T. ) ;
#44222=CARTESIAN_POINT ( 'NONE',  ( -166.6959734468149463, 0.000000000000000000, 165.0000000000000000 ) ) ;
#44228=CARTESIAN_POINT ( 'NONE',  ( -204.9459734468149463, 2.143131898507880377E-16, -0.9317124430720247208 ) ) ;
#44233=VECTOR ( 'NONE', #29914, 1000.000000000000000 ) ;
#44236=CIRCLE ( 'NONE', #49906, 1.750000000000001554 ) ;
#44243=CIRCLE ( 'NONE', #5761, 1.750000000000008438 ) ;
#44245=ORIENTED_EDGE ( 'NONE', *, *, #12642, .F. ) ;
#44247=CARTESIAN_POINT ( 'NONE',  ( 35.05402655318504657, 2.143131898507880377E-16, 79.06828755692797017 ) ) ;
#44250=VECTOR ( 'NONE', #43408, 1000.000000000000000 ) ;
#44254=PLANE ( 'NONE',  #3600 ) ;
#44255=ORIENTED_EDGE ( 'NONE', *, *, #48136, .T. ) ;
#44261=CARTESIAN_POINT ( 'NONE',  ( 155.0540265531850537, 2.143131898507880377E-16, 165.0000000000000000 ) ) ;
#44262=CARTESIAN_POINT ( 'NONE',  ( -128.4459734468149179, 0.000000000000000000, 79.06828755692799859 ) ) ;
#44265=( BOUNDED_CURVE ( )  B_SPLINE_CURVE ( 3, ( #37545, #14423, #26738, #30585 ),
 .UNSPECIFIED., .F., .F. ) 
 B_SPLINE_CURVE_WITH_KNOTS ( ( 4, 4 ),
 ( 1.570796326794896558, 3.141592653589793116 ),
 .UNSPECIFIED. ) 
 CURVE ( )  GEOMETRIC_REPRESENTATION_ITEM ( )  RATIONAL_B_SPLINE_CURVE ( ( 1.000000000000000000, 0.8047378541243649375, 0.8047378541243649375, 1.000000000000000000 ) ) 
 REPRESENTATION_ITEM ( '' )  );
#44266=ORIENTED_EDGE ( 'NONE', *, *, #8020, .F. ) ;
#44269=CARTESIAN_POINT ( 'NONE',  ( -87.72109971266203843, 1.750000000000009548, 159.7931612910809065 ) ) ;
#44270=ORIENTED_EDGE ( 'NONE', *, *, #9155, .F. ) ;
#44271=CARTESIAN_POINT ( 'NONE',  ( -127.7210997126620242, 1.749999999999996225, 1.843413822775058497 ) ) ;
#44275=CARTESIAN_POINT ( 'NONE',  ( -206.6959734468149463, -1.750000000000009992, 0.8182875569279768335 ) ) ;
#44278=CARTESIAN_POINT ( 'NONE',  ( -168.4459734468149463, 0.000000000000000000, -80.93171244307201562 ) ) ;
#44284=( BOUNDED_CURVE ( )  B_SPLINE_CURVE ( 3, ( #2129, #1877, #22628, #18256 ),
 .UNSPECIFIED., .F., .F. ) 
 B_SPLINE_CURVE_WITH_KNOTS ( ( 4, 4 ),
 ( 3.141592653589793116, 4.712388980384689674 ),
 .UNSPECIFIED. ) 
 CURVE ( )  GEOMETRIC_REPRESENTATION_ITEM ( )  RATIONAL_B_SPLINE_CURVE ( ( 1.000000000000000000, 0.8047378541243649375, 0.8047378541243649375, 1.000000000000000000 ) ) 
 REPRESENTATION_ITEM ( '' )  );
#44293=CARTESIAN_POINT ( 'NONE',  ( 210.0000000000000568, 0.000000000000000000, 2.568287556927987048 ) ) ;
#44297=CARTESIAN_POINT ( 'NONE',  ( -88.44597344681497475, 0.000000000000000000, 79.06828755692795596 ) ) ;
#44302=CARTESIAN_POINT ( 'NONE',  ( 152.2789002873379900, 1.750000000000009548, 41.84341382277508359 ) ) ;
#44303=CARTESIAN_POINT ( 'NONE',  ( -84.94597344681497475, 0.000000000000000000, 162.5682875569279702 ) ) ;
#44304=CARTESIAN_POINT ( 'NONE',  ( 210.0000000000000568, 0.000000000000000000, 82.56828755692799859 ) ) ;
#44305=EDGE_CURVE ( 'NONE', #45850, #4734, #17120, .T. ) ;
#44307=LINE ( 'NONE', #33046, #34205 ) ;
#44312=CARTESIAN_POINT ( 'NONE',  ( -4.945973446814903696, 2.143131898507912917E-16, 39.06828755692792754 ) ) ;
#44313=EDGE_CURVE ( 'NONE', #28555, #10095, #10744, .T. ) ;
#44317=CARTESIAN_POINT ( 'NONE',  ( -208.4459734468149463, 0.000000000000000000, 159.0682875569279702 ) ) ;
#44318=EDGE_LOOP ( 'NONE', ( #2642, #10912, #16774, #42328, #44108, #3604 ) ) ;
#44325=EDGE_CURVE ( 'NONE', #9127, #38516, #39489, .T. ) ;
#44327=CARTESIAN_POINT ( 'NONE',  ( -206.6959734468149463, 0.000000000000000000, 165.0000000000000000 ) ) ;
#44329=CARTESIAN_POINT ( 'NONE',  ( -128.4459734468149463, -1.025126265847081886, 39.06828755692799149 ) ) ;
#44335=AXIS2_PLACEMENT_3D ( 'NONE', #14101, #33378, #25672 ) ;
#44342=CARTESIAN_POINT ( 'NONE',  ( 75.05402655318509630, 2.143131898507880377E-16, 79.06828755692797017 ) ) ;
#44347=FACE_OUTER_BOUND ( 'NONE', #46275, .T. ) ;
#44351=ORIENTED_EDGE ( 'NONE', *, *, #28379, .T. ) ;
#44356=LINE ( 'NONE', #5115, #28380 ) ;
#44357=DIRECTION ( 'NONE',  ( 1.000000000000000000, 0.000000000000000000, 0.000000000000000000 ) ) ;
#44359=EDGE_LOOP ( 'NONE', ( #19247, #43917, #45683, #5446, #28996, #25293 ) ) ;
#44363=VERTEX_POINT ( 'NONE', #19963 ) ;
#44369=( BOUNDED_CURVE ( )  B_SPLINE_CURVE ( 3, ( #15354, #42033, #46360, #50447 ),
 .UNSPECIFIED., .F., .F. ) 
 B_SPLINE_CURVE_WITH_KNOTS ( ( 4, 4 ),
 ( 1.570796326794896558, 3.141592653589793116 ),
 .UNSPECIFIED. ) 
 CURVE ( )  GEOMETRIC_REPRESENTATION_ITEM ( )  RATIONAL_B_SPLINE_CURVE ( ( 1.000000000000000000, 0.8047378541243649375, 0.8047378541243649375, 1.000000000000000000 ) ) 
 REPRESENTATION_ITEM ( '' )  );
#44370=CARTESIAN_POINT ( 'NONE',  ( -44.94597344681493922, 2.143131898507880377E-16, 119.0682875569279702 ) ) ;
#44372=VECTOR ( 'NONE', #42098, 1000.000000000000000 ) ;
#44373=ORIENTED_EDGE ( 'NONE', *, *, #48967, .T. ) ;
#44379=EDGE_CURVE ( 'NONE', #18308, #29317, #48243, .T. ) ;
#44382=ORIENTED_EDGE ( 'NONE', *, *, #43209, .T. ) ;
#44387=ADVANCED_FACE ( 'NONE', ( #4327 ), #28438, .T. ) ;
#44389=DIRECTION ( 'NONE',  ( -1.000000000000000000, -0.000000000000000000, -0.000000000000000000 ) ) ;
#44392=CARTESIAN_POINT ( 'NONE',  ( -207.7210997126620384, -1.750000000000009548, -38.15658617722494483 ) ) ;
#44394=CARTESIAN_POINT ( 'NONE',  ( 74.32915281903215998, 1.750000000000009548, -158.1565861772249377 ) ) ;
#44395=CYLINDRICAL_SURFACE ( 'NONE', #1192, 1.750000000000001554 ) ;
#44396=EDGE_CURVE ( 'NONE', #18600, #40520, #49072, .T. ) ;
#44398=ORIENTED_EDGE ( 'NONE', *, *, #20329, .F. ) ;
#44399=ADVANCED_FACE ( 'NONE', ( #22179 ), #14474, .T. ) ;
#44402=ORIENTED_EDGE ( 'NONE', *, *, #31827, .T. ) ;
#44406=CARTESIAN_POINT ( 'NONE',  ( -8.445973446814976526, 0.000000000000000000, 165.0000000000000000 ) ) ;
#44411=DIRECTION ( 'NONE',  ( 0.000000000000000000, 0.000000000000000000, 1.000000000000000000 ) ) ;
#44416=CARTESIAN_POINT ( 'NONE',  ( -125.6708471809678542, -1.749999999999997113, -80.20683870891909351 ) ) ;
#44418=ORIENTED_EDGE ( 'NONE', *, *, #22703, .F. ) ;
#44419=CARTESIAN_POINT ( 'NONE',  ( -127.7210997126620242, 1.749999999999997113, -120.2068387089191219 ) ) ;
#44420=CYLINDRICAL_SURFACE ( 'NONE', #45559, 1.750000000000015543 ) ;
#44423=CYLINDRICAL_SURFACE ( 'NONE', #38245, 1.750000000000010214 ) ;
#44424=CARTESIAN_POINT ( 'NONE',  ( 31.55402655318503236, 0.000000000000000000, -0.9317124430720247208 ) ) ;
#44425=( BOUNDED_CURVE ( )  B_SPLINE_CURVE ( 3, ( #24995, #43716, #48536, #40395 ),
 .UNSPECIFIED., .F., .F. ) 
 B_SPLINE_CURVE_WITH_KNOTS ( ( 4, 4 ),
 ( 3.141592653589793116, 4.712388980384689674 ),
 .UNSPECIFIED. ) 
 CURVE ( )  GEOMETRIC_REPRESENTATION_ITEM ( )  RATIONAL_B_SPLINE_CURVE ( ( 1.000000000000000000, 0.8047378541243649375, 0.8047378541243649375, 1.000000000000000000 ) ) 
 REPRESENTATION_ITEM ( '' )  );
#44427=VERTEX_POINT ( 'NONE', #9176 ) ;
#44428=ORIENTED_EDGE ( 'NONE', *, *, #50255, .F. ) ;
#44429=ORIENTED_EDGE ( 'NONE', *, *, #172, .T. ) ;
#44432=( BOUNDED_CURVE ( )  B_SPLINE_CURVE ( 3, ( #28457, #7949, #39249, #507 ),
 .UNSPECIFIED., .F., .F. ) 
 B_SPLINE_CURVE_WITH_KNOTS ( ( 4, 4 ),
 ( 3.141592653589793116, 4.712388980384689674 ),
 .UNSPECIFIED. ) 
 CURVE ( )  GEOMETRIC_REPRESENTATION_ITEM ( )  RATIONAL_B_SPLINE_CURVE ( ( 1.000000000000000000, 0.8047378541243649375, 0.8047378541243649375, 1.000000000000000000 ) ) 
 REPRESENTATION_ITEM ( '' )  );
#44438=CARTESIAN_POINT ( 'NONE',  ( 210.0000000000000568, 0.000000000000000000, -117.4317124430720298 ) ) ;
#44440=DIRECTION ( 'NONE',  ( -0.000000000000000000, -0.000000000000000000, -1.000000000000000000 ) ) ;
#44443=ORIENTED_EDGE ( 'NONE', *, *, #32894, .T. ) ;
#44444=DIRECTION ( 'NONE',  ( -1.000000000000000000, -0.000000000000000000, -0.000000000000000000 ) ) ;
#44451=ORIENTED_EDGE ( 'NONE', *, *, #6106, .T. ) ;
#44455=CARTESIAN_POINT ( 'NONE',  ( -124.9459734468149463, 2.143131898507847836E-16, 165.0000000000000000 ) ) ;
#44458=CARTESIAN_POINT ( 'NONE',  ( 210.0000000000000568, 0.000000000000000000, 160.8182875569279702 ) ) ;
#44462=ORIENTED_EDGE ( 'NONE', *, *, #6094, .F. ) ;
#44464=LINE ( 'NONE', #41395, #17269 ) ;
#44468=ORIENTED_EDGE ( 'NONE', *, *, #12832, .F. ) ;
#44469=FACE_OUTER_BOUND ( 'NONE', #32265, .T. ) ;
#44472=ORIENTED_EDGE ( 'NONE', *, *, #42143, .T. ) ;
#44476=AXIS2_PLACEMENT_3D ( 'NONE', #46839, #15340, #448 ) ;
#44480=AXIS2_PLACEMENT_3D ( 'NONE', #40992, #36925, #17388 ) ;
#44481=ORIENTED_EDGE ( 'NONE', *, *, #28374, .F. ) ;
#44484=AXIS2_PLACEMENT_3D ( 'NONE', #46633, #35668, #7686 ) ;
#44485=CARTESIAN_POINT ( 'NONE',  ( 193.3040265531851105, 1.750000000000010214, -39.18171244307202983 ) ) ;
#44488=CYLINDRICAL_SURFACE ( 'NONE', #8754, 1.750000000000001554 ) ;
#44489=DIRECTION ( 'NONE',  ( 0.000000000000000000, 0.000000000000000000, 1.000000000000000000 ) ) ;
#44494=CARTESIAN_POINT ( 'NONE',  ( -126.6959734468149321, 1.749999999999997335, 80.81828755692798438 ) ) ;
#44495=VERTEX_POINT ( 'NONE', #20725 ) ;
#44498=CARTESIAN_POINT ( 'NONE',  ( -85.67084718096784002, -1.750000000000009548, -160.2068387089191219 ) ) ;
#44502=DIRECTION ( 'NONE',  ( -0.000000000000000000, -0.000000000000000000, -1.000000000000000000 ) ) ;
#44503=CARTESIAN_POINT ( 'NONE',  ( -164.9459734468149463, 2.143131898507880377E-16, -117.4317124430720725 ) ) ;
#44505=CARTESIAN_POINT ( 'NONE',  ( -88.44597344681497475, 0.000000000000000000, -0.9317124430720524764 ) ) ;
#44513=CARTESIAN_POINT ( 'NONE',  ( -46.69597344681494633, 1.750000000000010658, 120.8182875569279702 ) ) ;
#44517=CARTESIAN_POINT ( 'NONE',  ( 75.05402655318509630, 1.025126265847089435, 2.568287556927986159 ) ) ;
#44519=ORIENTED_EDGE ( 'NONE', *, *, #20462, .T. ) ;
#44526=CARTESIAN_POINT ( 'NONE',  ( 31.55402655318503236, 0.000000000000000000, 79.06828755692797017 ) ) ;
#44534=CARTESIAN_POINT ( 'NONE',  ( -88.44597344681494633, -1.025126265847089879, -77.43171244307200141 ) ) ;
#44536=ORIENTED_EDGE ( 'NONE', *, *, #10815, .F. ) ;
#44537=ORIENTED_EDGE ( 'NONE', *, *, #21107, .T. ) ;
#44542=EDGE_CURVE ( 'NONE', #17971, #36229, #40233, .T. ) ;
#44544=CARTESIAN_POINT ( 'NONE',  ( -5.670847180967843570, 1.750000000000023537, -118.1565861772249519 ) ) ;
#44547=CARTESIAN_POINT ( 'NONE',  ( -206.6959734468149463, 1.750000000000010214, 40.81828755692798438 ) ) ;
#44549=FACE_OUTER_BOUND ( 'NONE', #40227, .T. ) ;
#44553=( BOUNDED_CURVE ( )  B_SPLINE_CURVE ( 3, ( #46461, #46717, #18782, #49544 ),
 .UNSPECIFIED., .F., .F. ) 
 B_SPLINE_CURVE_WITH_KNOTS ( ( 4, 4 ),
 ( 4.712388980384689674, 6.283185307179586232 ),
 .UNSPECIFIED. ) 
 CURVE ( )  GEOMETRIC_REPRESENTATION_ITEM ( )  RATIONAL_B_SPLINE_CURVE ( ( 1.000000000000000000, 0.8047378541243649375, 0.8047378541243649375, 1.000000000000000000 ) ) 
 REPRESENTATION_ITEM ( '' )  );
#44558=( BOUNDED_CURVE ( )  B_SPLINE_CURVE ( 3, ( #30923, #27993, #44134, #36474 ),
 .UNSPECIFIED., .F., .F. ) 
 B_SPLINE_CURVE_WITH_KNOTS ( ( 4, 4 ),
 ( 1.570796326794896558, 3.141592653589793116 ),
 .UNSPECIFIED. ) 
 CURVE ( )  GEOMETRIC_REPRESENTATION_ITEM ( )  RATIONAL_B_SPLINE_CURVE ( ( 1.000000000000000000, 0.8047378541243649375, 0.8047378541243649375, 1.000000000000000000 ) ) 
 REPRESENTATION_ITEM ( '' )  );
#44561=CARTESIAN_POINT ( 'NONE',  ( 193.3040265531851105, 1.750000000000009992, 0.8182875569279768335 ) ) ;
#44563=CARTESIAN_POINT ( 'NONE',  ( -168.4459734468149463, 0.000000000000000000, -117.4317124430720725 ) ) ;
#44564=CARTESIAN_POINT ( 'NONE',  ( -126.6959734468149321, -1.749999999999997113, 40.81828755692798438 ) ) ;
#44565=VECTOR ( 'NONE', #50057, 1000.000000000000000 ) ;
#44568=ADVANCED_FACE ( 'NONE', ( #13017 ), #41928, .F. ) ;
#44572=( BOUNDED_CURVE ( )  B_SPLINE_CURVE ( 3, ( #13385, #25194, #40840, #41098 ),
 .UNSPECIFIED., .F., .F. ) 
 B_SPLINE_CURVE_WITH_KNOTS ( ( 4, 4 ),
 ( 0.000000000000000000, 1.570796326794896558 ),
 .UNSPECIFIED. ) 
 CURVE ( )  GEOMETRIC_REPRESENTATION_ITEM ( )  RATIONAL_B_SPLINE_CURVE ( ( 1.000000000000000000, 0.8047378541243649375, 0.8047378541243649375, 1.000000000000000000 ) ) 
 REPRESENTATION_ITEM ( '' )  );
#44573=ORIENTED_EDGE ( 'NONE', *, *, #38380, .F. ) ;
#44574=CARTESIAN_POINT ( 'NONE',  ( 71.55402655318505367, -1.025126265847089657, -80.93171244307201562 ) ) ;
#44575=ORIENTED_EDGE ( 'NONE', *, *, #8680, .F. ) ;
#44576=ORIENTED_EDGE ( 'NONE', *, *, #15514, .F. ) ;
#44577=VECTOR ( 'NONE', #37130, 1000.000000000000000 ) ;
#44578=ORIENTED_EDGE ( 'NONE', *, *, #34343, .F. ) ;
#44580=CARTESIAN_POINT ( 'NONE',  ( -4.945973446814903696, 2.143131898507912917E-16, -80.93171244307204404 ) ) ;
#44588=ORIENTED_EDGE ( 'NONE', *, *, #27378, .T. ) ;
#44593=CARTESIAN_POINT ( 'NONE',  ( -7.721099712662037540, -1.750000000000022871, 1.843413822775074040 ) ) ;
#44594=CYLINDRICAL_SURFACE ( 'NONE', #36816, 1.750000000000015543 ) ;
#44595=EDGE_LOOP ( 'NONE', ( #45994, #27565, #26791, #5957, #22656, #26516 ) ) ;
#44596=AXIS2_PLACEMENT_3D ( 'NONE', #34973, #19793, #11603 ) ;
#44598=ORIENTED_EDGE ( 'NONE', *, *, #9208, .F. ) ;
#44600=CARTESIAN_POINT ( 'NONE',  ( 151.5540265531850537, 0.000000000000000000, 2.568287556927978166 ) ) ;
#44610=VECTOR ( 'NONE', #21455, 1000.000000000000000 ) ;
#44611=CARTESIAN_POINT ( 'NONE',  ( 210.0000000000000568, 0.000000000000000000, -157.4317124430720298 ) ) ;
#44613=EDGE_CURVE ( 'NONE', #43433, #32767, #11886, .T. ) ;
#44614=CARTESIAN_POINT ( 'NONE',  ( 75.05402655318509630, 2.143131898507880377E-16, -117.4317124430720156 ) ) ;
#44616=VECTOR ( 'NONE', #10384, 1000.000000000000000 ) ;
#44618=ORIENTED_EDGE ( 'NONE', *, *, #18638, .F. ) ;
#44619=PRODUCT_CONTEXT ( 'NONE', #21033, 'mechanical' ) ;
#44623=DIRECTION ( 'NONE',  ( -1.000000000000000000, -0.000000000000000000, -0.000000000000000000 ) ) ;
#44631=VECTOR ( 'NONE', #34794, 1000.000000000000000 ) ;
#44633=CARTESIAN_POINT ( 'NONE',  ( -168.4459734468149463, 0.000000000000000000, -40.93171244307202983 ) ) ;
#44635=EDGE_CURVE ( 'NONE', #26837, #44023, #14775, .T. ) ;
#44639=CARTESIAN_POINT ( 'NONE',  ( 153.3040265531850537, 1.750000000000010658, 120.8182875569279702 ) ) ;
#44642=ORIENTED_EDGE ( 'NONE', *, *, #40051, .F. ) ;
#44643=EDGE_CURVE ( 'NONE', #26888, #50033, #8292, .T. ) ;
#44647=LINE ( 'NONE', #9524, #24551 ) ;
#44648=VECTOR ( 'NONE', #11774, 1000.000000000000000 ) ;
#44655=CARTESIAN_POINT ( 'NONE',  ( 210.0000000000000568, 0.000000000000000000, -119.1817124430720440 ) ) ;
#44657=ORIENTED_EDGE ( 'NONE', *, *, #25612, .F. ) ;
#44660=( BOUNDED_CURVE ( )  B_SPLINE_CURVE ( 3, ( #23315, #35149, #34931, #15622 ),
 .UNSPECIFIED., .F., .F. ) 
 B_SPLINE_CURVE_WITH_KNOTS ( ( 4, 4 ),
 ( 0.000000000000000000, 1.570796326794896558 ),
 .UNSPECIFIED. ) 
 CURVE ( )  GEOMETRIC_REPRESENTATION_ITEM ( )  RATIONAL_B_SPLINE_CURVE ( ( 1.000000000000000000, 0.8047378541243649375, 0.8047378541243649375, 1.000000000000000000 ) ) 
 REPRESENTATION_ITEM ( '' )  );
#44662=ORIENTED_EDGE ( 'NONE', *, *, #22908, .T. ) ;
#44664=CYLINDRICAL_SURFACE ( 'NONE', #44723, 1.750000000000001554 ) ;
#44665=EDGE_LOOP ( 'NONE', ( #29804, #36950, #20902, #41763, #49940 ) ) ;
#44669=CARTESIAN_POINT ( 'NONE',  ( 74.32915281903215998, -1.750000000000009326, -158.1565861772249377 ) ) ;
#44670=EDGE_CURVE ( 'NONE', #33964, #11965, #3018, .T. ) ;
#44672=EDGE_CURVE ( 'NONE', #12712, #18308, #39765, .T. ) ;
#44673=ORIENTED_EDGE ( 'NONE', *, *, #24389, .F. ) ;
#44678=ADVANCED_FACE ( 'NONE', ( #1372 ), #32415, .T. ) ;
#44681=EDGE_CURVE ( 'NONE', #44427, #18915, #20096, .T. ) ;
#44684=VERTEX_POINT ( 'NONE', #8312 ) ;
#44687=CARTESIAN_POINT ( 'NONE',  ( 210.0000000000000568, 2.143131898507876926E-16, -80.93171244307202983 ) ) ;
#44690=VECTOR ( 'NONE', #217, 1000.000000000000000 ) ;
#44691=CARTESIAN_POINT ( 'NONE',  ( 210.0000000000000568, 2.143131898507881856E-16, -80.93171244307202983 ) ) ;
#44693=CARTESIAN_POINT ( 'NONE',  ( -210.0000000000000568, 0.000000000000000000, -79.18171244307201562 ) ) ;
#44711=AXIS2_PLACEMENT_3D ( 'NONE', #48171, #36443, #26326 ) ;
#44718=ORIENTED_EDGE ( 'NONE', *, *, #11533, .T. ) ;
#44722=( BOUNDED_CURVE ( )  B_SPLINE_CURVE ( 3, ( #37237, #26407, #2060, #41806 ),
 .UNSPECIFIED., .F., .F. ) 
 B_SPLINE_CURVE_WITH_KNOTS ( ( 4, 4 ),
 ( 3.141592653589793116, 4.712388980384689674 ),
 .UNSPECIFIED. ) 
 CURVE ( )  GEOMETRIC_REPRESENTATION_ITEM ( )  RATIONAL_B_SPLINE_CURVE ( ( 1.000000000000000000, 0.8047378541243649375, 0.8047378541243649375, 1.000000000000000000 ) ) 
 REPRESENTATION_ITEM ( '' )  );
#44723=AXIS2_PLACEMENT_3D ( 'NONE', #40351, #9051, #21340 ) ;
#44728=CARTESIAN_POINT ( 'NONE',  ( -168.4459734468149463, 0.000000000000000000, 159.0682875569279702 ) ) ;
#44731=ORIENTED_EDGE ( 'NONE', *, *, #33478, .T. ) ;
#44733=ORIENTED_EDGE ( 'NONE', *, *, #36328, .T. ) ;
#44734=( BOUNDED_CURVE ( )  B_SPLINE_CURVE ( 3, ( #41647, #50302, #49546, #6492 ),
 .UNSPECIFIED., .F., .F. ) 
 B_SPLINE_CURVE_WITH_KNOTS ( ( 4, 4 ),
 ( 0.000000000000000000, 1.570796326794896558 ),
 .UNSPECIFIED. ) 
 CURVE ( )  GEOMETRIC_REPRESENTATION_ITEM ( )  RATIONAL_B_SPLINE_CURVE ( ( 1.000000000000000000, 0.8047378541243649375, 0.8047378541243649375, 1.000000000000000000 ) ) 
 REPRESENTATION_ITEM ( '' )  );
#44737=CARTESIAN_POINT ( 'NONE',  ( 193.3040265531851105, 1.750000000000010658, 120.8182875569279702 ) ) ;
#44739=EDGE_CURVE ( 'NONE', #46959, #34536, #27560, .T. ) ;
#44742=CARTESIAN_POINT ( 'NONE',  ( -46.69597344681494633, -1.750000000000010214, -39.18171244307202983 ) ) ;
#44743=CARTESIAN_POINT ( 'NONE',  ( -205.6708471809678827, -1.750000000000009326, 1.843413822775066269 ) ) ;
#44745=VERTEX_POINT ( 'NONE', #9062 ) ;
#44747=EDGE_CURVE ( 'NONE', #2022, #47416, #22334, .T. ) ;
#44748=LINE ( 'NONE', #6779, #44616 ) ;
#44749=DIRECTION ( 'NONE',  ( -0.000000000000000000, -0.000000000000000000, -1.000000000000000000 ) ) ;
#44752=CARTESIAN_POINT ( 'NONE',  ( 151.5540265531850537, 0.000000000000000000, 122.5682875569279702 ) ) ;
#44753=DIRECTION ( 'NONE',  ( 0.000000000000000000, 0.000000000000000000, 1.000000000000000000 ) ) ;
#44757=CARTESIAN_POINT ( 'NONE',  ( 151.5540265531850537, -1.025126265847089435, 2.568287556927986159 ) ) ;
#44759=ORIENTED_EDGE ( 'NONE', *, *, #42108, .F. ) ;
#44762=EDGE_CURVE ( 'NONE', #16264, #40358, #32875, .T. ) ;
#44766=DIRECTION ( 'NONE',  ( -1.000000000000000000, 0.000000000000000000, 0.000000000000000000 ) ) ;
#44768=LINE ( 'NONE', #38370, #4083 ) ;
#44774=DIRECTION ( 'NONE',  ( -1.000000000000000000, 0.000000000000000000, 0.000000000000000000 ) ) ;
#44782=EDGE_CURVE ( 'NONE', #19656, #10604, #44957, .T. ) ;
#44783=CARTESIAN_POINT ( 'NONE',  ( 111.5540265531850537, -1.025126265847081886, 119.0682875569279702 ) ) ;
#44784=AXIS2_PLACEMENT_3D ( 'NONE', #31777, #12014, #4059 ) ;
#44792=CARTESIAN_POINT ( 'NONE',  ( -208.4459734468149463, 0.000000000000000000, -120.9317124430720156 ) ) ;
#44799=CARTESIAN_POINT ( 'NONE',  ( 73.30402655318508209, 0.000000000000000000, 165.0000000000000000 ) ) ;
#44800=ORIENTED_EDGE ( 'NONE', *, *, #21037, .T. ) ;
#44801=ORIENTED_EDGE ( 'NONE', *, *, #8392, .T. ) ;
#44803=DIRECTION ( 'NONE',  ( -1.000000000000000000, 0.000000000000000000, 0.000000000000000000 ) ) ;
#44806=VECTOR ( 'NONE', #3925, 1000.000000000000000 ) ;
#44808=CARTESIAN_POINT ( 'NONE',  ( -207.7210997126620384, -1.750000000000010214, -118.1565861772249519 ) ) ;
#44809=CARTESIAN_POINT ( 'NONE',  ( -207.7210997126620384, -1.750000000000009548, 39.79316129108089228 ) ) ;
#44811=DIRECTION ( 'NONE',  ( -0.000000000000000000, -0.000000000000000000, -1.000000000000000000 ) ) ;
#44812=CARTESIAN_POINT ( 'NONE',  ( 71.55402655318505367, 1.025126265847089213, 42.56828755692799149 ) ) ;
#44817=CARTESIAN_POINT ( 'NONE',  ( 210.0000000000000568, 0.000000000000000000, 120.8182875569279702 ) ) ;
#44825=ORIENTED_EDGE ( 'NONE', *, *, #29716, .F. ) ;
#44831=CARTESIAN_POINT ( 'NONE',  ( 193.3040265531851105, 1.750000000000010658, 120.8182875569279702 ) ) ;
#44832=ORIENTED_EDGE ( 'NONE', *, *, #35030, .F. ) ;
#44833=CARTESIAN_POINT ( 'NONE',  ( 33.30402655318503946, -1.750000000000010658, -119.1817124430720440 ) ) ;
#44834=ORIENTED_EDGE ( 'NONE', *, *, #43237, .T. ) ;
#44848=ORIENTED_EDGE ( 'NONE', *, *, #37611, .F. ) ;
#44855=CARTESIAN_POINT ( 'NONE',  ( -164.9459734468149463, 2.143131898507880377E-16, -157.4317124430720582 ) ) ;
#44857=ORIENTED_EDGE ( 'NONE', *, *, #21901, .F. ) ;
#44860=( BOUNDED_CURVE ( )  B_SPLINE_CURVE ( 3, ( #27590, #28333, #8836, #44216 ),
 .UNSPECIFIED., .F., .F. ) 
 B_SPLINE_CURVE_WITH_KNOTS ( ( 4, 4 ),
 ( 3.141592653589793116, 4.712388980384689674 ),
 .UNSPECIFIED. ) 
 CURVE ( )  GEOMETRIC_REPRESENTATION_ITEM ( )  RATIONAL_B_SPLINE_CURVE ( ( 1.000000000000000000, 0.8047378541243649375, 0.8047378541243649375, 1.000000000000000000 ) ) 
 REPRESENTATION_ITEM ( '' )  );
#44865=EDGE_CURVE ( 'NONE', #36589, #18600, #46598, .T. ) ;
#44866=( BOUNDED_CURVE ( )  B_SPLINE_CURVE ( 3, ( #34430, #41857, #50008, #7220 ),
 .UNSPECIFIED., .F., .F. ) 
 B_SPLINE_CURVE_WITH_KNOTS ( ( 4, 4 ),
 ( 1.570796326794896558, 3.141592653589793116 ),
 .UNSPECIFIED. ) 
 CURVE ( )  GEOMETRIC_REPRESENTATION_ITEM ( )  RATIONAL_B_SPLINE_CURVE ( ( 1.000000000000000000, 0.8047378541243649375, 0.8047378541243649375, 1.000000000000000000 ) ) 
 REPRESENTATION_ITEM ( '' )  );
#44867=VECTOR ( 'NONE', #42426, 1000.000000000000000 ) ;
#44871=DIRECTION ( 'NONE',  ( -0.000000000000000000, -0.000000000000000000, -1.000000000000000000 ) ) ;
#44874=CYLINDRICAL_SURFACE ( 'NONE', #43693, 1.750000000000008438 ) ;
#44875=VERTEX_POINT ( 'NONE', #25978 ) ;
#44878=( BOUNDED_CURVE ( )  B_SPLINE_CURVE ( 3, ( #45058, #48887, #5578, #29198 ),
 .UNSPECIFIED., .F., .F. ) 
 B_SPLINE_CURVE_WITH_KNOTS ( ( 4, 4 ),
 ( 0.000000000000000000, 1.570796326794896558 ),
 .UNSPECIFIED. ) 
 CURVE ( )  GEOMETRIC_REPRESENTATION_ITEM ( )  RATIONAL_B_SPLINE_CURVE ( ( 1.000000000000000000, 0.8047378541243649375, 0.8047378541243649375, 1.000000000000000000 ) ) 
 REPRESENTATION_ITEM ( '' )  );
#44879=CARTESIAN_POINT ( 'NONE',  ( -45.67084718096785423, 1.750000000000009548, -158.1565861772249377 ) ) ;
#44887=ORIENTED_EDGE ( 'NONE', *, *, #14838, .F. ) ;
#44888=CARTESIAN_POINT ( 'NONE',  ( -4.945973446814917018, 1.025126265847097207, 159.0682875569279418 ) ) ;
#44889=VERTEX_POINT ( 'NONE', #40617 ) ;
#44891=CARTESIAN_POINT ( 'NONE',  ( 35.05402655318504657, 2.143131898507880377E-16, 79.06828755692797017 ) ) ;
#44894=EDGE_LOOP ( 'NONE', ( #29711, #35384, #45614, #5, #28298, #28922 ) ) ;
#44895=CARTESIAN_POINT ( 'NONE',  ( 151.5540265531850537, -1.025126265847089213, -160.9317124430720014 ) ) ;
#44897=PLANE ( 'NONE',  #37729 ) ;
#44898=CARTESIAN_POINT ( 'NONE',  ( -47.72109971266203132, -1.750000000000009548, -40.20683870891912193 ) ) ;
#44902=CARTESIAN_POINT ( 'NONE',  ( 73.30402655318508209, 0.000000000000000000, -165.0000000000000000 ) ) ;
#44905=CARTESIAN_POINT ( 'NONE',  ( -128.4459734468149179, 0.000000000000000000, 122.5682875569279418 ) ) ;
#44908=CARTESIAN_POINT ( 'NONE',  ( -166.6959734468149463, 1.750000000000009992, 0.8182875569279768335 ) ) ;
#44914=ORIENTED_EDGE ( 'NONE', *, *, #27720, .F. ) ;
#44918=( BOUNDED_CURVE ( )  B_SPLINE_CURVE ( 3, ( #44370, #28750, #4646, #9240 ),
 .UNSPECIFIED., .F., .F. ) 
 B_SPLINE_CURVE_WITH_KNOTS ( ( 4, 4 ),
 ( 0.000000000000000000, 1.570796326794896558 ),
 .UNSPECIFIED. ) 
 CURVE ( )  GEOMETRIC_REPRESENTATION_ITEM ( )  RATIONAL_B_SPLINE_CURVE ( ( 1.000000000000000000, 0.8047378541243649375, 0.8047378541243649375, 1.000000000000000000 ) ) 
 REPRESENTATION_ITEM ( '' )  );
#44920=CARTESIAN_POINT ( 'NONE',  ( -87.72109971266203843, -1.750000000000010214, 81.84341382277507648 ) ) ;
#44922=ADVANCED_FACE ( 'NONE', ( #1869 ), #13660, .T. ) ;
#44923=CARTESIAN_POINT ( 'NONE',  ( -126.6959734468149321, -1.749999999999996891, 0.8182875569279768335 ) ) ;
#44930=EDGE_CURVE ( 'NONE', #3579, #37204, #30511, .T. ) ;
#44933=CARTESIAN_POINT ( 'NONE',  ( -4.945973446814916130, -1.025126265847097429, 119.0682875569279133 ) ) ;
#44934=CYLINDRICAL_SURFACE ( 'NONE', #33235, 1.750000000000008438 ) ;
#44937=ORIENTED_EDGE ( 'NONE', *, *, #24635, .T. ) ;
#44942=CARTESIAN_POINT ( 'NONE',  ( -124.9459734468149463, 2.143131898507847836E-16, 2.568287556927950632 ) ) ;
#44957=( BOUNDED_CURVE ( )  B_SPLINE_CURVE ( 3, ( #39364, #17765, #37299, #2121 ),
 .UNSPECIFIED., .F., .F. ) 
 B_SPLINE_CURVE_WITH_KNOTS ( ( 4, 4 ),
 ( 0.000000000000000000, 1.570796326794896558 ),
 .UNSPECIFIED. ) 
 CURVE ( )  GEOMETRIC_REPRESENTATION_ITEM ( )  RATIONAL_B_SPLINE_CURVE ( ( 1.000000000000000000, 0.8047378541243649375, 0.8047378541243649375, 1.000000000000000000 ) ) 
 REPRESENTATION_ITEM ( '' )  );
#44961=CARTESIAN_POINT ( 'NONE',  ( -5.670847180967843570, -1.750000000000022427, 1.843413822775074040 ) ) ;
#44969=ORIENTED_EDGE ( 'NONE', *, *, #3434, .F. ) ;
#44970=VERTEX_POINT ( 'NONE', #26730 ) ;
#44973=CARTESIAN_POINT ( 'NONE',  ( -204.9459734468148895, 1.025126265847089657, 79.06828755692797017 ) ) ;
#44979=CARTESIAN_POINT ( 'NONE',  ( -128.4459734468149463, -1.025126265847082108, -37.43171244307203693 ) ) ;
#44993=CARTESIAN_POINT ( 'NONE',  ( 35.05402655318504657, 2.143131898507882349E-16, -165.0000000000000000 ) ) ;
#45002=CARTESIAN_POINT ( 'NONE',  ( -166.6959734468149463, 0.000000000000000000, 165.0000000000000000 ) ) ;
#45012=CARTESIAN_POINT ( 'NONE',  ( 73.30402655318508209, -1.750000000000009992, -159.1817124430720298 ) ) ;
#45017=FACE_OUTER_BOUND ( 'NONE', #39714, .T. ) ;
#45027=LINE ( 'NONE', #25816, #22996 ) ;
#45028=CIRCLE ( 'NONE', #33566, 1.750000000000009992 ) ;
#45031=ORIENTED_EDGE ( 'NONE', *, *, #22507, .T. ) ;
#45033=CARTESIAN_POINT ( 'NONE',  ( 35.05402655318504657, 1.025126265847089435, 2.568287556927986159 ) ) ;
#45034=ORIENTED_EDGE ( 'NONE', *, *, #32619, .T. ) ;
#45038=EDGE_CURVE ( 'NONE', #35686, #17256, #1098, .T. ) ;
#45046=FACE_OUTER_BOUND ( 'NONE', #13708, .T. ) ;
#45049=DIRECTION ( 'NONE',  ( -1.000000000000000000, -0.000000000000000000, -0.000000000000000000 ) ) ;
#45050=FACE_OUTER_BOUND ( 'NONE', #47853, .T. ) ;
#45058=CARTESIAN_POINT ( 'NONE',  ( -48.44597344681492501, 0.000000000000000000, 162.5682875569279702 ) ) ;
#45059=CARTESIAN_POINT ( 'NONE',  ( -86.69597344681494633, 1.750000000000010214, 40.81828755692798438 ) ) ;
#45061=DIRECTION ( 'NONE',  ( -1.000000000000000000, -0.000000000000000000, -0.000000000000000000 ) ) ;
#45068=FACE_OUTER_BOUND ( 'NONE', #34024, .T. ) ;
#45070=LINE ( 'NONE', #41503, #7837 ) ;
#45071=( GEOMETRIC_REPRESENTATION_CONTEXT ( 3 ) GLOBAL_UNCERTAINTY_ASSIGNED_CONTEXT ( ( #40005 ) ) GLOBAL_UNIT_ASSIGNED_CONTEXT ( ( #7757, #31364, #43152 ) ) REPRESENTATION_CONTEXT ( 'NONE', 'WORKASPACE' ) );
#45074=ADVANCED_FACE ( 'NONE', ( #16685 ), #27490, .T. ) ;
#45075=EDGE_CURVE ( 'NONE', #50239, #38442, #39296, .T. ) ;
#45077=ORIENTED_EDGE ( 'NONE', *, *, #1217, .T. ) ;
#45079=CARTESIAN_POINT ( 'NONE',  ( -166.6959734468149463, 1.750000000000010658, 80.81828755692798438 ) ) ;
#45088=CYLINDRICAL_SURFACE ( 'NONE', #4155, 1.750000000000015543 ) ;
#45090=ORIENTED_EDGE ( 'NONE', *, *, #595, .F. ) ;
#45095=EDGE_CURVE ( 'NONE', #2812, #4778, #24026, .T. ) ;
#45096=CARTESIAN_POINT ( 'NONE',  ( -6.695973446814940111, -1.750000000000024203, -79.18171244307201562 ) ) ;
#45105=ORIENTED_EDGE ( 'NONE', *, *, #35565, .T. ) ;
#45107=ORIENTED_EDGE ( 'NONE', *, *, #2008, .F. ) ;
#45109=FACE_OUTER_BOUND ( 'NONE', #18982, .T. ) ;
#45111=ORIENTED_EDGE ( 'NONE', *, *, #40246, .T. ) ;
#45112=DIRECTION ( 'NONE',  ( -0.000000000000000000, -0.000000000000000000, -1.000000000000000000 ) ) ;
#45115=CARTESIAN_POINT ( 'NONE',  ( 111.5540265531850537, 1.025126265847081886, 39.06828755692799149 ) ) ;
#45127=ORIENTED_EDGE ( 'NONE', *, *, #26779, .F. ) ;
#45128=CYLINDRICAL_SURFACE ( 'NONE', #44335, 1.750000000000015543 ) ;
#45130=CARTESIAN_POINT ( 'NONE',  ( -46.69597344681494633, 1.750000000000009992, -159.1817124430720298 ) ) ;
#45133=VECTOR ( 'NONE', #13395, 1000.000000000000000 ) ;
#45134=ORIENTED_EDGE ( 'NONE', *, *, #12176, .F. ) ;
#45137=CARTESIAN_POINT ( 'NONE',  ( -5.670847180967843570, 1.750000000000022871, 159.7931612910808781 ) ) ;
#45139=CARTESIAN_POINT ( 'NONE',  ( -85.67084718096784002, 1.750000000000010214, 119.7931612910808781 ) ) ;
#45140=VECTOR ( 'NONE', #16582, 1000.000000000000000 ) ;
#45142=CARTESIAN_POINT ( 'NONE',  ( 74.32915281903215998, 1.750000000000010214, 119.7931612910808781 ) ) ;
#45146=CARTESIAN_POINT ( 'NONE',  ( 75.05402655318509630, 2.143131898507880377E-16, -77.43171244307198720 ) ) ;
#45147=DIRECTION ( 'NONE',  ( -0.000000000000000000, -0.000000000000000000, -1.000000000000000000 ) ) ;
#45148=CARTESIAN_POINT ( 'NONE',  ( 114.3291528190321173, 1.749999999999996669, -158.1565861772249377 ) ) ;
#45149=CARTESIAN_POINT ( 'NONE',  ( -127.7210997126620242, 1.749999999999996669, -118.1565861772249661 ) ) ;
#45153=ORIENTED_EDGE ( 'NONE', *, *, #5891, .T. ) ;
#45154=FACE_OUTER_BOUND ( 'NONE', #49423, .T. ) ;
#45155=( BOUNDED_CURVE ( )  B_SPLINE_CURVE ( 3, ( #36397, #47368, #12264, #27924 ),
 .UNSPECIFIED., .F., .F. ) 
 B_SPLINE_CURVE_WITH_KNOTS ( ( 4, 4 ),
 ( 4.712388980384689674, 6.283185307179586232 ),
 .UNSPECIFIED. ) 
 CURVE ( )  GEOMETRIC_REPRESENTATION_ITEM ( )  RATIONAL_B_SPLINE_CURVE ( ( 1.000000000000000000, 0.8047378541243649375, 0.8047378541243649375, 1.000000000000000000 ) ) 
 REPRESENTATION_ITEM ( '' )  );
#45158=CARTESIAN_POINT ( 'NONE',  ( 33.30402655318503946, 1.750000000000009992, -159.1817124430720298 ) ) ;
#45159=EDGE_LOOP ( 'NONE', ( #18965, #5633, #25876, #33514, #2556, #11445 ) ) ;
#45161=( BOUNDED_CURVE ( )  B_SPLINE_CURVE ( 3, ( #8119, #34825, #3225, #27108 ),
 .UNSPECIFIED., .F., .F. ) 
 B_SPLINE_CURVE_WITH_KNOTS ( ( 4, 4 ),
 ( 4.712388980384689674, 6.283185307179586232 ),
 .UNSPECIFIED. ) 
 CURVE ( )  GEOMETRIC_REPRESENTATION_ITEM ( )  RATIONAL_B_SPLINE_CURVE ( ( 1.000000000000000000, 0.8047378541243649375, 0.8047378541243649375, 1.000000000000000000 ) ) 
 REPRESENTATION_ITEM ( '' )  );
#45162=AXIS2_PLACEMENT_3D ( 'NONE', #15560, #31223, #11706 ) ;
#45165=CARTESIAN_POINT ( 'NONE',  ( 195.0540265531851105, 1.025126265847089879, -77.43171244307200141 ) ) ;
#45167=CARTESIAN_POINT ( 'NONE',  ( -48.44597344681496054, -1.025126265847089435, -157.4317124430720582 ) ) ;
#45174=CARTESIAN_POINT ( 'NONE',  ( 31.55402655318503236, 0.000000000000000000, 119.0682875569279702 ) ) ;
#45175=( BOUNDED_CURVE ( )  B_SPLINE_CURVE ( 3, ( #46735, #34487, #50065, #11636 ),
 .UNSPECIFIED., .F., .F. ) 
 B_SPLINE_CURVE_WITH_KNOTS ( ( 4, 4 ),
 ( 0.000000000000000000, 1.570796326794896558 ),
 .UNSPECIFIED. ) 
 CURVE ( )  GEOMETRIC_REPRESENTATION_ITEM ( )  RATIONAL_B_SPLINE_CURVE ( ( 1.000000000000000000, 0.8047378541243649375, 0.8047378541243649375, 1.000000000000000000 ) ) 
 REPRESENTATION_ITEM ( '' )  );
#45184=CARTESIAN_POINT ( 'NONE',  ( 210.0000000000000568, 0.000000000000000000, 80.81828755692798438 ) ) ;
#45189=EDGE_LOOP ( 'NONE', ( #17146, #32859, #34110, #5566, #29797 ) ) ;
#45193=EDGE_LOOP ( 'NONE', ( #18226, #19652, #42394, #1825, #28862, #12095 ) ) ;
#45197=VECTOR ( 'NONE', #485, 1000.000000000000000 ) ;
#45201=AXIS2_PLACEMENT_3D ( 'NONE', #32704, #9352, #31957 ) ;
#45211=EDGE_CURVE ( 'NONE', #26902, #39755, #35800, .T. ) ;
#45213=ADVANCED_FACE ( 'NONE', ( #48696 ), #33619, .T. ) ;
#45219=CARTESIAN_POINT ( 'NONE',  ( 31.55402655318503236, 1.025126265847089213, 159.0682875569279418 ) ) ;
#45222=ORIENTED_EDGE ( 'NONE', *, *, #1396, .T. ) ;
#45228=ORIENTED_EDGE ( 'NONE', *, *, #11770, .F. ) ;
#45233=CARTESIAN_POINT ( 'NONE',  ( 191.5540265531851105, 0.000000000000000000, -0.9317124430720247208 ) ) ;
#45234=ORIENTED_EDGE ( 'NONE', *, *, #13659, .T. ) ;
#45246=CARTESIAN_POINT ( 'NONE',  ( -204.9459734468149463, 2.143131898507880377E-16, -40.93171244307202983 ) ) ;
#45247=ADVANCED_FACE ( 'NONE', ( #11529 ), #27178, .T. ) ;
#45249=LINE ( 'NONE', #42181, #42161 ) ;
#45250=ORIENTED_EDGE ( 'NONE', *, *, #17778, .F. ) ;
#45255=CARTESIAN_POINT ( 'NONE',  ( 71.55402655318505367, 1.025126265847089435, -117.4317124430720156 ) ) ;
#45258=CYLINDRICAL_SURFACE ( 'NONE', #13846, 1.750000000000001554 ) ;
#45259=CARTESIAN_POINT ( 'NONE',  ( 32.27890028733795447, -1.750000000000010214, 121.8434138227750623 ) ) ;
#45260=DIRECTION ( 'NONE',  ( -0.000000000000000000, -0.000000000000000000, -1.000000000000000000 ) ) ;
#45261=VECTOR ( 'NONE', #19821, 1000.000000000000000 ) ;
#45263=DIRECTION ( 'NONE',  ( -0.000000000000000000, -0.000000000000000000, -1.000000000000000000 ) ) ;
#45266=EDGE_CURVE ( 'NONE', #36841, #40138, #3552, .T. ) ;
#45272=EDGE_CURVE ( 'NONE', #11294, #20141, #34130, .T. ) ;
#45274=VERTEX_POINT ( 'NONE', #49711 ) ;
#45275=ORIENTED_EDGE ( 'NONE', *, *, #45534, .T. ) ;
#45276=CARTESIAN_POINT ( 'NONE',  ( 75.05402655318509630, 2.143131898507880377E-16, 42.56828755692799859 ) ) ;
#45279=CARTESIAN_POINT ( 'NONE',  ( 74.32915281903215998, 1.750000000000009548, 39.79316129108089228 ) ) ;
#45280=EDGE_LOOP ( 'NONE', ( #1224, #21841, #25663, #29038, #6611, #25041 ) ) ;
#45282=CARTESIAN_POINT ( 'NONE',  ( 151.5540265531850537, 0.000000000000000000, 39.06828755692798438 ) ) ;
#45294=ORIENTED_EDGE ( 'NONE', *, *, #44313, .F. ) ;
#45297=LINE ( 'NONE', #30179, #2465 ) ;
#45299=CARTESIAN_POINT ( 'NONE',  ( -206.6959734468149463, 1.750000000000009992, -159.1817124430720298 ) ) ;
#45300=ORIENTED_EDGE ( 'NONE', *, *, #10891, .T. ) ;
#45302=CARTESIAN_POINT ( 'NONE',  ( 75.05402655318509630, 1.025126265847088991, 162.5682875569279133 ) ) ;
#45314=ADVANCED_FACE ( 'NONE', ( #992 ), #734, .F. ) ;
#45315=CARTESIAN_POINT ( 'NONE',  ( 192.2789002873380184, 1.750000000000010436, 79.79316129108087807 ) ) ;
#45318=ORIENTED_EDGE ( 'NONE', *, *, #30288, .T. ) ;
#45319=FACE_OUTER_BOUND ( 'NONE', #18100, .T. ) ;
#45320=( BOUNDED_CURVE ( )  B_SPLINE_CURVE ( 3, ( #49391, #14793, #34557, #42997 ),
 .UNSPECIFIED., .F., .F. ) 
 B_SPLINE_CURVE_WITH_KNOTS ( ( 4, 4 ),
 ( 1.570796326794896558, 3.141592653589793116 ),
 .UNSPECIFIED. ) 
 CURVE ( )  GEOMETRIC_REPRESENTATION_ITEM ( )  RATIONAL_B_SPLINE_CURVE ( ( 1.000000000000000000, 0.8047378541243649375, 0.8047378541243649375, 1.000000000000000000 ) ) 
 REPRESENTATION_ITEM ( '' )  );
#45321=DIRECTION ( 'NONE',  ( -1.000000000000000000, -0.000000000000000000, -0.000000000000000000 ) ) ;
#45324=CARTESIAN_POINT ( 'NONE',  ( 31.55402655318503236, 1.025126265847089657, -80.93171244307201562 ) ) ;
#45328=DIRECTION ( 'NONE',  ( -1.000000000000000000, 0.000000000000000000, 0.000000000000000000 ) ) ;
#45329=CARTESIAN_POINT ( 'NONE',  ( -128.4459734468149179, 0.000000000000000000, -77.43171244307204404 ) ) ;
#45332=CARTESIAN_POINT ( 'NONE',  ( 31.55402655318503236, 0.000000000000000000, -117.4317124430720156 ) ) ;
#45333=ORIENTED_EDGE ( 'NONE', *, *, #16790, .F. ) ;
#45334=VERTEX_POINT ( 'NONE', #4817 ) ;
#45336=ORIENTED_EDGE ( 'NONE', *, *, #34465, .T. ) ;
#45339=VECTOR ( 'NONE', #21847, 1000.000000000000000 ) ;
#45344=DIRECTION ( 'NONE',  ( -1.000000000000000000, 0.000000000000000000, 0.000000000000000000 ) ) ;
#45345=FACE_OUTER_BOUND ( 'NONE', #38316, .T. ) ;
#45350=CARTESIAN_POINT ( 'NONE',  ( -8.445973446814976526, 0.000000000000000000, 119.0682875569279418 ) ) ;
#45352=CARTESIAN_POINT ( 'NONE',  ( 75.05402655318509630, 2.143131898507880377E-16, -37.43171244307200141 ) ) ;
#45355=VERTEX_POINT ( 'NONE', #38989 ) ;
#45366=CARTESIAN_POINT ( 'NONE',  ( -6.695973446814940111, 1.750000000000024203, 80.81828755692798438 ) ) ;
#45367=ADVANCED_FACE ( 'NONE', ( #47637 ), #39242, .T. ) ;
#45375=EDGE_CURVE ( 'NONE', #50159, #43433, #28952, .T. ) ;
#45376=CARTESIAN_POINT ( 'NONE',  ( 191.5540265531851105, 0.000000000000000000, -40.93171244307202983 ) ) ;
#45380=CARTESIAN_POINT ( 'NONE',  ( -126.6959734468149321, 1.749999999999997335, -119.1817124430720440 ) ) ;
#45385=EDGE_CURVE ( 'NONE', #38997, #23844, #44660, .T. ) ;
#45388=VECTOR ( 'NONE', #28987, 1000.000000000000000 ) ;
#45392=EDGE_LOOP ( 'NONE', ( #9023, #6141, #47087, #33236, #48572, #45720 ) ) ;
#45394=EDGE_LOOP ( 'NONE', ( #22205, #160, #10946, #23428, #19077, #22232 ) ) ;
#45396=FACE_OUTER_BOUND ( 'NONE', #46528, .T. ) ;
#45401=ORIENTED_EDGE ( 'NONE', *, *, #13089, .T. ) ;
#45404=CIRCLE ( 'NONE', #32453, 1.750000000000001554 ) ;
#45408=VERTEX_POINT ( 'NONE', #46881 ) ;
#45409=VERTEX_POINT ( 'NONE', #27429 ) ;
#45411=ADVANCED_FACE ( 'NONE', ( #19726 ), #35402, .T. ) ;
#45412=ORIENTED_EDGE ( 'NONE', *, *, #2896, .F. ) ;
#45416=CARTESIAN_POINT ( 'NONE',  ( -4.945973446814916130, -1.025126265847097207, 82.56828755692798438 ) ) ;
#45417=ORIENTED_EDGE ( 'NONE', *, *, #47562, .T. ) ;
#45420=DIRECTION ( 'NONE',  ( -0.000000000000000000, -0.000000000000000000, -1.000000000000000000 ) ) ;
#45427=DIRECTION ( 'NONE',  ( -0.000000000000000000, -0.000000000000000000, -1.000000000000000000 ) ) ;
#45429=VERTEX_POINT ( 'NONE', #44312 ) ;
#45430=CARTESIAN_POINT ( 'NONE',  ( 112.2789002873379758, 1.749999999999996669, 41.84341382277508359 ) ) ;
#45432=ADVANCED_FACE ( 'NONE', ( #5335 ), #40496, .T. ) ;
#45434=EDGE_CURVE ( 'NONE', #47604, #7572, #16828, .T. ) ;
#45435=DIRECTION ( 'NONE',  ( -0.000000000000000000, -0.000000000000000000, -1.000000000000000000 ) ) ;
#45436=CYLINDRICAL_SURFACE ( 'NONE', #12930, 1.750000000000008438 ) ;
#45438=VECTOR ( 'NONE', #40457, 1000.000000000000000 ) ;
#45439=DIRECTION ( 'NONE',  ( 0.000000000000000000, 0.000000000000000000, 1.000000000000000000 ) ) ;
#45449=ORIENTED_EDGE ( 'NONE', *, *, #16272, .F. ) ;
#45451=LINE ( 'NONE', #49285, #12243 ) ;
#45453=CYLINDRICAL_SURFACE ( 'NONE', #43449, 1.750000000000001554 ) ;
#45454=CARTESIAN_POINT ( 'NONE',  ( 114.3291528190321173, 1.749999999999996891, 121.8434138227750481 ) ) ;
#45456=FACE_OUTER_BOUND ( 'NONE', #47597, .T. ) ;
#45461=DIRECTION ( 'NONE',  ( -0.000000000000000000, -0.000000000000000000, -1.000000000000000000 ) ) ;
#45463=CARTESIAN_POINT ( 'NONE',  ( -4.945973446814903696, 2.143131898507912917E-16, 2.568287556928034121 ) ) ;
#45464=( BOUNDED_CURVE ( )  B_SPLINE_CURVE ( 3, ( #44275, #5804, #48857, #9146 ),
 .UNSPECIFIED., .F., .F. ) 
 B_SPLINE_CURVE_WITH_KNOTS ( ( 4, 4 ),
 ( 1.570796326794896558, 3.141592653589793116 ),
 .UNSPECIFIED. ) 
 CURVE ( )  GEOMETRIC_REPRESENTATION_ITEM ( )  RATIONAL_B_SPLINE_CURVE ( ( 1.000000000000000000, 0.8047378541243649375, 0.8047378541243649375, 1.000000000000000000 ) ) 
 REPRESENTATION_ITEM ( '' )  );
#45465=ORIENTED_EDGE ( 'NONE', *, *, #41016, .F. ) ;
#45469=EDGE_CURVE ( 'NONE', #13512, #37466, #28686, .T. ) ;
#45470=CIRCLE ( 'NONE', #30794, 1.750000000000015543 ) ;
#45471=ORIENTED_EDGE ( 'NONE', *, *, #19909, .T. ) ;
#45474=CARTESIAN_POINT ( 'NONE',  ( -4.945973446814903696, 2.143131898507912917E-16, 165.0000000000000000 ) ) ;
#45480=CIRCLE ( 'NONE', #20938, 1.750000000000001554 ) ;
#45484=VECTOR ( 'NONE', #19142, 1000.000000000000000 ) ;
#45486=AXIS2_PLACEMENT_3D ( 'NONE', #31923, #7813, #35026 ) ;
#45487=ORIENTED_EDGE ( 'NONE', *, *, #2907, .T. ) ;
#45489=ORIENTED_EDGE ( 'NONE', *, *, #50257, .F. ) ;
#45493=CARTESIAN_POINT ( 'NONE',  ( 210.0000000000000568, 0.000000000000000000, 2.568287556927987048 ) ) ;
#45494=ORIENTED_EDGE ( 'NONE', *, *, #28017, .F. ) ;
#45497=FACE_OUTER_BOUND ( 'NONE', #48533, .T. ) ;
#45498=ORIENTED_EDGE ( 'NONE', *, *, #2907, .F. ) ;
#45499=CARTESIAN_POINT ( 'NONE',  ( -208.4459734468148611, 1.025126265847088991, 2.568287556927986159 ) ) ;
#45502=CARTESIAN_POINT ( 'NONE',  ( -87.72109971266203843, 1.750000000000009548, -160.2068387089191219 ) ) ;
#45503=CARTESIAN_POINT ( 'NONE',  ( -164.9459734468149463, -1.025126265847089657, -120.9317124430720440 ) ) ;
#45504=EDGE_LOOP ( 'NONE', ( #20953, #22419 ) ) ;
#45505=ADVANCED_FACE ( 'NONE', ( #9689 ), #13273, .T. ) ;
#45506=DIRECTION ( 'NONE',  ( -0.000000000000000000, -0.000000000000000000, -1.000000000000000000 ) ) ;
#45507=CARTESIAN_POINT ( 'NONE',  ( 113.3040265531850537, 0.000000000000000000, 165.0000000000000000 ) ) ;
#45508=CARTESIAN_POINT ( 'NONE',  ( 73.30402655318508209, 0.000000000000000000, 165.0000000000000000 ) ) ;
#45513=DIRECTION ( 'NONE',  ( -1.000000000000000000, -0.000000000000000000, -0.000000000000000000 ) ) ;
#45521=ADVANCED_FACE ( 'NONE', ( #9181 ), #44068, .T. ) ;
#45523=VECTOR ( 'NONE', #43293, 1000.000000000000000 ) ;
#45525=CARTESIAN_POINT ( 'NONE',  ( 151.5540265531850537, -1.025126265847089657, 42.56828755692799149 ) ) ;
#45528=EDGE_CURVE ( 'NONE', #9801, #12079, #33312, .T. ) ;
#45534=EDGE_CURVE ( 'NONE', #30766, #12663, #4294, .T. ) ;
#45539=ORIENTED_EDGE ( 'NONE', *, *, #10236, .T. ) ;
#45540=ORIENTED_EDGE ( 'NONE', *, *, #30901, .F. ) ;
#45541=CARTESIAN_POINT ( 'NONE',  ( -206.6959734468149463, 1.750000000000010214, -39.18171244307202983 ) ) ;
#45550=AXIS2_PLACEMENT_3D ( 'NONE', #8113, #42724, #35079 ) ;
#45556=ADVANCED_FACE ( 'NONE', ( #40748 ), #1745, .T. ) ;
#45557=LINE ( 'NONE', #1984, #19214 ) ;
#45559=AXIS2_PLACEMENT_3D ( 'NONE', #32650, #48498, #5689 ) ;
#45560=ADVANCED_FACE ( 'NONE', ( #16897 ), #33052, .T. ) ;
#45565=CARTESIAN_POINT ( 'NONE',  ( -206.6959734468149463, 1.750000000000010658, -79.18171244307201562 ) ) ;
#45566=ORIENTED_EDGE ( 'NONE', *, *, #32054, .F. ) ;
#45568=ADVANCED_FACE ( 'NONE', ( #1993 ), #3488, .T. ) ;
#45569=DIRECTION ( 'NONE',  ( 1.000000000000000000, 0.000000000000000000, 0.000000000000000000 ) ) ;
#45571=CARTESIAN_POINT ( 'NONE',  ( -164.9459734468149463, -1.025126265847089213, -160.9317124430720014 ) ) ;
#45573=AXIS2_PLACEMENT_3D ( 'NONE', #44902, #25444, #17744 ) ;
#45576=ORIENTED_EDGE ( 'NONE', *, *, #6529, .T. ) ;
#45589=ORIENTED_EDGE ( 'NONE', *, *, #7832, .F. ) ;
#45590=LINE ( 'NONE', #41764, #16700 ) ;
#45594=VERTEX_POINT ( 'NONE', #46322 ) ;
#45596=EDGE_CURVE ( 'NONE', #40426, #31866, #50174, .T. ) ;
#45608=CARTESIAN_POINT ( 'NONE',  ( -86.69597344681494633, 1.750000000000010658, 80.81828755692798438 ) ) ;
#45612=CARTESIAN_POINT ( 'NONE',  ( -48.44597344681495343, 0.000000000000000000, 165.0000000000000000 ) ) ;
#45614=ORIENTED_EDGE ( 'NONE', *, *, #30059, .T. ) ;
#45620=DIRECTION ( 'NONE',  ( -1.000000000000000000, -0.000000000000000000, -0.000000000000000000 ) ) ;
#45623=CARTESIAN_POINT ( 'NONE',  ( 193.3040265531851105, -1.750000000000009992, 0.8182875569279768335 ) ) ;
#45624=AXIS2_PLACEMENT_3D ( 'NONE', #9996, #34123, #49202 ) ;
#45628=( BOUNDED_CURVE ( )  B_SPLINE_CURVE ( 3, ( #22658, #3406, #3665, #27018 ),
 .UNSPECIFIED., .F., .F. ) 
 B_SPLINE_CURVE_WITH_KNOTS ( ( 4, 4 ),
 ( 0.000000000000000000, 1.570796326794896558 ),
 .UNSPECIFIED. ) 
 CURVE ( )  GEOMETRIC_REPRESENTATION_ITEM ( )  RATIONAL_B_SPLINE_CURVE ( ( 1.000000000000000000, 0.8047378541243649375, 0.8047378541243649375, 1.000000000000000000 ) ) 
 REPRESENTATION_ITEM ( '' )  );
#45630=ORIENTED_EDGE ( 'NONE', *, *, #48967, .F. ) ;
#45631=CARTESIAN_POINT ( 'NONE',  ( -205.6708471809678827, -1.750000000000009548, -40.20683870891912193 ) ) ;
#45633=CARTESIAN_POINT ( 'NONE',  ( -124.9459734468149321, -1.025126265847081664, 122.5682875569279702 ) ) ;
#45640=CARTESIAN_POINT ( 'NONE',  ( -88.44597344681497475, 0.000000000000000000, 165.0000000000000000 ) ) ;
#45642=EDGE_LOOP ( 'NONE', ( #42622, #30069, #20867, #50177, #36699, #15555 ) ) ;
#45645=EDGE_CURVE ( 'NONE', #41652, #8390, #4693, .T. ) ;
#45652=LINE ( 'NONE', #29528, #48218 ) ;
#45654=VERTEX_POINT ( 'NONE', #22498 ) ;
#45659=CARTESIAN_POINT ( 'NONE',  ( -44.94597344681493922, 1.025126265847089435, 2.568287556927986159 ) ) ;
#45661=VERTEX_POINT ( 'NONE', #38175 ) ;
#45662=EDGE_CURVE ( 'NONE', #38893, #24608, #2991, .T. ) ;
#45663=VERTEX_POINT ( 'NONE', #31990 ) ;
#45664=CYLINDRICAL_SURFACE ( 'NONE', #538, 1.750000000000015543 ) ;
#45666=EDGE_CURVE ( 'NONE', #30495, #39140, #4017, .T. ) ;
#45671=DIRECTION ( 'NONE',  ( -0.000000000000000000, -0.000000000000000000, -1.000000000000000000 ) ) ;
#45672=ADVANCED_FACE ( 'NONE', ( #38934 ), #43765, .T. ) ;
#45673=LINE ( 'NONE', #26210, #36618 ) ;
#45676=DIRECTION ( 'NONE',  ( -1.000000000000000000, -0.000000000000000000, -0.000000000000000000 ) ) ;
#45679=CARTESIAN_POINT ( 'NONE',  ( -204.9459734468149463, 2.143131898507880377E-16, 165.0000000000000000 ) ) ;
#45683=ORIENTED_EDGE ( 'NONE', *, *, #50042, .T. ) ;
#45685=CARTESIAN_POINT ( 'NONE',  ( 194.3291528190321742, -1.750000000000009548, -118.1565861772249519 ) ) ;
#45686=CARTESIAN_POINT ( 'NONE',  ( -88.44597344681497475, 0.000000000000000000, 165.0000000000000000 ) ) ;
#45687=CARTESIAN_POINT ( 'NONE',  ( 115.0540265531850395, 1.025126265847081886, 79.06828755692797017 ) ) ;
#45688=AXIS2_PLACEMENT_3D ( 'NONE', #13899, #13666, #5962 ) ;
#45690=CYLINDRICAL_SURFACE ( 'NONE', #14291, 1.750000000000015543 ) ;
#45691=DIRECTION ( 'NONE',  ( -0.000000000000000000, -0.000000000000000000, -1.000000000000000000 ) ) ;
#45692=ORIENTED_EDGE ( 'NONE', *, *, #42443, .T. ) ;
#45705=ORIENTED_EDGE ( 'NONE', *, *, #48476, .F. ) ;
#45710=DIRECTION ( 'NONE',  ( -1.000000000000000000, -0.000000000000000000, -0.000000000000000000 ) ) ;
#45711=FACE_OUTER_BOUND ( 'NONE', #7615, .T. ) ;
#45714=VERTEX_POINT ( 'NONE', #47330 ) ;
#45716=CARTESIAN_POINT ( 'NONE',  ( -125.6708471809678542, 1.749999999999996669, -38.15658617722495194 ) ) ;
#45717=EDGE_CURVE ( 'NONE', #13126, #16395, #7995, .T. ) ;
#45720=ORIENTED_EDGE ( 'NONE', *, *, #4498, .T. ) ;
#45722=CARTESIAN_POINT ( 'NONE',  ( -84.94597344681494633, 2.143131898507880377E-16, -77.43171244307204404 ) ) ;
#45727=EDGE_CURVE ( 'NONE', #10604, #45654, #22355, .T. ) ;
#45733=ORIENTED_EDGE ( 'NONE', *, *, #18732, .F. ) ;
#45734=ORIENTED_EDGE ( 'NONE', *, *, #44325, .T. ) ;
#45742=CARTESIAN_POINT ( 'NONE',  ( 31.55402655318503236, 0.000000000000000000, 159.0682875569279702 ) ) ;
#45745=CARTESIAN_POINT ( 'NONE',  ( -88.44597344681491791, 2.143131898507880377E-16, -160.9317124430720298 ) ) ;
#45750=CYLINDRICAL_SURFACE ( 'NONE', #6808, 1.750000000000015543 ) ;
#45751=DIRECTION ( 'NONE',  ( -1.000000000000000000, -0.000000000000000000, -0.000000000000000000 ) ) ;
#45753=ADVANCED_FACE ( 'NONE', ( #24291 ), #11463, .T. ) ;
#45755=( BOUNDED_CURVE ( )  B_SPLINE_CURVE ( 3, ( #49723, #30276, #45886, #39001 ),
 .UNSPECIFIED., .F., .F. ) 
 B_SPLINE_CURVE_WITH_KNOTS ( ( 4, 4 ),
 ( 1.570796326794896558, 3.141592653589793116 ),
 .UNSPECIFIED. ) 
 CURVE ( )  GEOMETRIC_REPRESENTATION_ITEM ( )  RATIONAL_B_SPLINE_CURVE ( ( 1.000000000000000000, 0.8047378541243649375, 0.8047378541243649375, 1.000000000000000000 ) ) 
 REPRESENTATION_ITEM ( '' )  );
#45757=FACE_OUTER_BOUND ( 'NONE', #49574, .T. ) ;
#45759=CARTESIAN_POINT ( 'NONE',  ( 151.5540265531850537, -1.025126265847089213, -0.9317124430720324924 ) ) ;
#45760=CIRCLE ( 'NONE', #9750, 1.750000000000008438 ) ;
#45763=( BOUNDED_CURVE ( )  B_SPLINE_CURVE ( 3, ( #32884, #37253, #17220, #5911 ),
 .UNSPECIFIED., .F., .F. ) 
 B_SPLINE_CURVE_WITH_KNOTS ( ( 4, 4 ),
 ( 3.141592653589793116, 4.712388980384689674 ),
 .UNSPECIFIED. ) 
 CURVE ( )  GEOMETRIC_REPRESENTATION_ITEM ( )  RATIONAL_B_SPLINE_CURVE ( ( 1.000000000000000000, 0.8047378541243649375, 0.8047378541243649375, 1.000000000000000000 ) ) 
 REPRESENTATION_ITEM ( '' )  );
#45766=ORIENTED_EDGE ( 'NONE', *, *, #32264, .F. ) ;
#45771=CARTESIAN_POINT ( 'NONE',  ( -206.6959734468149463, -1.750000000000009992, -159.1817124430720298 ) ) ;
#45779=CARTESIAN_POINT ( 'NONE',  ( -45.67084718096785423, 1.750000000000009326, 161.8434138227750907 ) ) ;
#45780=CARTESIAN_POINT ( 'NONE',  ( -207.7210997126620384, 1.750000000000009548, -118.1565861772249519 ) ) ;
#45783=ORIENTED_EDGE ( 'NONE', *, *, #23161, .T. ) ;
#45787=CARTESIAN_POINT ( 'NONE',  ( 191.5540265531851105, 0.000000000000000000, -37.43171244307205825 ) ) ;
#45789=CARTESIAN_POINT ( 'NONE',  ( 210.0000000000000568, 0.000000000000000000, 122.5682875569279844 ) ) ;
#45790=ORIENTED_EDGE ( 'NONE', *, *, #5525, .T. ) ;
#45791=DIRECTION ( 'NONE',  ( 0.000000000000000000, 0.000000000000000000, 1.000000000000000000 ) ) ;
#45792=CARTESIAN_POINT ( 'NONE',  ( 74.32915281903215998, -1.750000000000009548, 81.84341382277507648 ) ) ;
#45794=ORIENTED_EDGE ( 'NONE', *, *, #42894, .T. ) ;
#45798=VECTOR ( 'NONE', #13280, 1000.000000000000000 ) ;
#45799=CYLINDRICAL_SURFACE ( 'NONE', #21816, 1.750000000000001554 ) ;
#45800=CARTESIAN_POINT ( 'NONE',  ( -205.6708471809678827, 1.750000000000009548, -160.2068387089191219 ) ) ;
#45807=LINE ( 'NONE', #38420, #25064 ) ;
#45819=VECTOR ( 'NONE', #32186, 1000.000000000000000 ) ;
#45820=CARTESIAN_POINT ( 'NONE',  ( -46.69597344681494633, 1.750000000000009992, 160.8182875569279702 ) ) ;
#45821=VERTEX_POINT ( 'NONE', #23250 ) ;
#45826=ORIENTED_EDGE ( 'NONE', *, *, #41633, .T. ) ;
#45828=ORIENTED_EDGE ( 'NONE', *, *, #7966, .T. ) ;
#45829=VERTEX_POINT ( 'NONE', #50665 ) ;
#45835=CARTESIAN_POINT ( 'NONE',  ( 210.0000000000000568, 0.000000000000000000, -159.1817124430720298 ) ) ;
#45836=EDGE_CURVE ( 'NONE', #34748, #3643, #23526, .T. ) ;
#45840=EDGE_CURVE ( 'NONE', #40426, #38146, #47832, .T. ) ;
#45841=DIRECTION ( 'NONE',  ( -0.000000000000000000, -0.000000000000000000, -1.000000000000000000 ) ) ;
#45842=CARTESIAN_POINT ( 'NONE',  ( -208.4459734468149463, 0.000000000000000000, -80.93171244307201562 ) ) ;
#45846=CARTESIAN_POINT ( 'NONE',  ( -7.721099712662037540, -1.750000000000023537, 79.79316129108087807 ) ) ;
#45847=DIRECTION ( 'NONE',  ( 0.000000000000000000, 0.000000000000000000, 1.000000000000000000 ) ) ;
#45849=ORIENTED_EDGE ( 'NONE', *, *, #28625, .T. ) ;
#45850=VERTEX_POINT ( 'NONE', #25043 ) ;
#45851=CARTESIAN_POINT ( 'NONE',  ( 210.0000000000000568, 0.000000000000000000, 82.56828755692799859 ) ) ;
#45857=DIRECTION ( 'NONE',  ( -0.000000000000000000, -0.000000000000000000, -1.000000000000000000 ) ) ;
#45859=EDGE_CURVE ( 'NONE', #22212, #47361, #1112, .T. ) ;
#45861=VECTOR ( 'NONE', #33393, 1000.000000000000000 ) ;
#45867=AXIS2_PLACEMENT_3D ( 'NONE', #21720, #17867, #44803 ) ;
#45870=EDGE_CURVE ( 'NONE', #17731, #34855, #23619, .T. ) ;
#45871=ADVANCED_FACE ( 'NONE', ( #17079 ), #36615, .T. ) ;
#45875=ADVANCED_FACE ( 'NONE', ( #1687 ), #13477, .T. ) ;
#45877=CARTESIAN_POINT ( 'NONE',  ( 111.5540265531850679, 0.000000000000000000, 165.0000000000000000 ) ) ;
#45879=ORIENTED_EDGE ( 'NONE', *, *, #42841, .T. ) ;
#45886=CARTESIAN_POINT ( 'NONE',  ( -44.94597344681493922, 1.025126265847089879, -77.43171244307200141 ) ) ;
#45888=CARTESIAN_POINT ( 'NONE',  ( -4.945973446814916130, 1.025126265847097429, 119.0682875569279133 ) ) ;
#45890=CARTESIAN_POINT ( 'NONE',  ( 73.30402655318508209, -1.750000000000010214, -39.18171244307202983 ) ) ;
#45894=ORIENTED_EDGE ( 'NONE', *, *, #48338, .T. ) ;
#45895=DIRECTION ( 'NONE',  ( -0.000000000000000000, -0.000000000000000000, -1.000000000000000000 ) ) ;
#45896=ADVANCED_FACE ( 'NONE', ( #32499 ), #21175, .T. ) ;
#45900=ADVANCED_FACE ( 'NONE', ( #48333 ), #29138, .T. ) ;
#45901=EDGE_CURVE ( 'NONE', #47066, #26504, #26044, .T. ) ;
#45904=CARTESIAN_POINT ( 'NONE',  ( -8.445973446814964092, 1.025126265847096985, 42.56828755692800570 ) ) ;
#45906=CARTESIAN_POINT ( 'NONE',  ( -44.94597344681493922, -1.025126265847088991, 2.568287556927986159 ) ) ;
#45911=ORIENTED_EDGE ( 'NONE', *, *, #6658, .F. ) ;
#45912=EDGE_LOOP ( 'NONE', ( #44351, #16728, #1459, #22336, #29774, #12163 ) ) ;
#45914=EDGE_CURVE ( 'NONE', #5639, #8857, #28865, .T. ) ;
#45917=CARTESIAN_POINT ( 'NONE',  ( -8.445973446814964092, 1.025126265847097429, -80.93171244307204404 ) ) ;
#45918=ORIENTED_EDGE ( 'NONE', *, *, #16831, .F. ) ;
#45920=( BOUNDED_CURVE ( )  B_SPLINE_CURVE ( 3, ( #47990, #8290, #23930, #39594 ),
 .UNSPECIFIED., .F., .F. ) 
 B_SPLINE_CURVE_WITH_KNOTS ( ( 4, 4 ),
 ( 3.141592653589793116, 4.712388980384689674 ),
 .UNSPECIFIED. ) 
 CURVE ( )  GEOMETRIC_REPRESENTATION_ITEM ( )  RATIONAL_B_SPLINE_CURVE ( ( 1.000000000000000000, 0.8047378541243649375, 0.8047378541243649375, 1.000000000000000000 ) ) 
 REPRESENTATION_ITEM ( '' )  );
#45921=ORIENTED_EDGE ( 'NONE', *, *, #28778, .T. ) ;
#45922=ADVANCED_FACE ( 'NONE', ( #26802 ), #37863, .T. ) ;
#45923=CARTESIAN_POINT ( 'NONE',  ( 35.05402655318504657, 2.143131898507880377E-16, -157.4317124430720014 ) ) ;
#45927=VERTEX_POINT ( 'NONE', #18079 ) ;
#45930=CARTESIAN_POINT ( 'NONE',  ( 114.3291528190321173, 1.749999999999996669, 1.843413822775057609 ) ) ;
#45938=CARTESIAN_POINT ( 'NONE',  ( -84.94597344681494633, 2.143131898507873721E-16, -165.0000000000000000 ) ) ;
#45941=CARTESIAN_POINT ( 'NONE',  ( -124.9459734468149463, 2.143131898507847836E-16, -157.4317124430720582 ) ) ;
#45945=ORIENTED_EDGE ( 'NONE', *, *, #29695, .T. ) ;
#45948=EDGE_CURVE ( 'NONE', #37949, #27161, #34128, .T. ) ;
#45952=ADVANCED_FACE ( 'NONE', ( #18577 ), #45750, .T. ) ;
#45954=ORIENTED_EDGE ( 'NONE', *, *, #21433, .T. ) ;
#45956=ORIENTED_EDGE ( 'NONE', *, *, #459, .F. ) ;
#45957=DIRECTION ( 'NONE',  ( -1.000000000000000000, 0.000000000000000000, 0.000000000000000000 ) ) ;
#45964=CARTESIAN_POINT ( 'NONE',  ( -165.6708471809677974, -1.750000000000009326, 1.843413822775066269 ) ) ;
#45966=CARTESIAN_POINT ( 'NONE',  ( -87.72109971266203843, -1.750000000000010214, 121.8434138227750623 ) ) ;
#45969=EDGE_LOOP ( 'NONE', ( #38063, #39886, #45790, #4562, #7714 ) ) ;
#45970=CARTESIAN_POINT ( 'NONE',  ( -206.6959734468149463, -1.750000000000009992, 160.8182875569279702 ) ) ;
#45982=CARTESIAN_POINT ( 'NONE',  ( 35.05402655318504657, 2.143131898507880377E-16, 165.0000000000000000 ) ) ;
#45988=CARTESIAN_POINT ( 'NONE',  ( -46.69597344681494633, 1.750000000000009992, 160.8182875569279702 ) ) ;
#45992=CARTESIAN_POINT ( 'NONE',  ( 210.0000000000000568, 0.000000000000000000, 120.8182875569279702 ) ) ;
#45994=ORIENTED_EDGE ( 'NONE', *, *, #33928, .F. ) ;
#46001=( BOUNDED_CURVE ( )  B_SPLINE_CURVE ( 3, ( #24328, #32274, #46855, #4052 ),
 .UNSPECIFIED., .F., .F. ) 
 B_SPLINE_CURVE_WITH_KNOTS ( ( 4, 4 ),
 ( 3.141592653589793116, 4.712388980384689674 ),
 .UNSPECIFIED. ) 
 CURVE ( )  GEOMETRIC_REPRESENTATION_ITEM ( )  RATIONAL_B_SPLINE_CURVE ( ( 1.000000000000000000, 0.8047378541243649375, 0.8047378541243649375, 1.000000000000000000 ) ) 
 REPRESENTATION_ITEM ( '' )  );
#46002=CARTESIAN_POINT ( 'NONE',  ( 71.55402655318505367, 1.025126265847089213, -0.9317124430720324924 ) ) ;
#46005=AXIS2_PLACEMENT_3D ( 'NONE', #48938, #13824, #29497 ) ;
#46006=DIRECTION ( 'NONE',  ( -0.000000000000000000, -0.000000000000000000, -1.000000000000000000 ) ) ;
#46008=FACE_OUTER_BOUND ( 'NONE', #36025, .T. ) ;
#46010=ADVANCED_FACE ( 'NONE', ( #38363 ), #49335, .T. ) ;
#46011=EDGE_CURVE ( 'NONE', #16170, #20298, #27630, .T. ) ;
#46020=CARTESIAN_POINT ( 'NONE',  ( 210.0000000000000568, 2.143131898507881856E-16, 79.06828755692797017 ) ) ;
#46028=DIRECTION ( 'NONE',  ( -0.000000000000000000, -0.000000000000000000, -1.000000000000000000 ) ) ;
#46032=AXIS2_PLACEMENT_3D ( 'NONE', #44061, #29875, #16625 ) ;
#46034=EDGE_CURVE ( 'NONE', #17107, #41447, #9921, .T. ) ;
#46035=CARTESIAN_POINT ( 'NONE',  ( 73.30402655318508209, -1.750000000000010658, 120.8182875569279702 ) ) ;
#46036=CARTESIAN_POINT ( 'NONE',  ( 210.0000000000000568, 2.143131898507881856E-16, -120.9317124430720582 ) ) ;
#46038=VERTEX_POINT ( 'NONE', #20793 ) ;
#46043=ORIENTED_EDGE ( 'NONE', *, *, #16863, .T. ) ;
#46045=CARTESIAN_POINT ( 'NONE',  ( -208.4459734468149463, 0.000000000000000000, 162.5682875569279702 ) ) ;
#46046=LINE ( 'NONE', #37655, #1291 ) ;
#46048=EDGE_LOOP ( 'NONE', ( #29357, #29128, #27982, #18955, #1821, #19587 ) ) ;
#46056=CARTESIAN_POINT ( 'NONE',  ( -164.9459734468149463, 2.143131898507880377E-16, -37.43171244307205825 ) ) ;
#46057=( BOUNDED_CURVE ( )  B_SPLINE_CURVE ( 3, ( #10593, #34467, #45964, #49792 ),
 .UNSPECIFIED., .F., .F. ) 
 B_SPLINE_CURVE_WITH_KNOTS ( ( 4, 4 ),
 ( 3.141592653589793116, 4.712388980384689674 ),
 .UNSPECIFIED. ) 
 CURVE ( )  GEOMETRIC_REPRESENTATION_ITEM ( )  RATIONAL_B_SPLINE_CURVE ( ( 1.000000000000000000, 0.8047378541243649375, 0.8047378541243649375, 1.000000000000000000 ) ) 
 REPRESENTATION_ITEM ( '' )  );
#46058=AXIS2_PLACEMENT_3D ( 'NONE', #3347, #49749, #30562 ) ;
#46062=DIRECTION ( 'NONE',  ( 0.000000000000000000, 0.000000000000000000, 1.000000000000000000 ) ) ;
#46063=AXIS2_PLACEMENT_3D ( 'NONE', #47462, #28002, #31624 ) ;
#46064=ORIENTED_EDGE ( 'NONE', *, *, #18888, .T. ) ;
#46067=AXIS2_PLACEMENT_3D ( 'NONE', #34834, #29691, #30455 ) ;
#46072=DIRECTION ( 'NONE',  ( -0.000000000000000000, -0.000000000000000000, -1.000000000000000000 ) ) ;
#46073=VECTOR ( 'NONE', #24224, 1000.000000000000000 ) ;
#46075=ORIENTED_EDGE ( 'NONE', *, *, #17961, .T. ) ;
#46077=CARTESIAN_POINT ( 'NONE',  ( -8.445973446814962315, 1.025126265847096985, 159.0682875569279418 ) ) ;
#46086=AXIS2_PLACEMENT_3D ( 'NONE', #39433, #11971, #27627 ) ;
#46088=DIRECTION ( 'NONE',  ( -1.000000000000000000, -0.000000000000000000, -0.000000000000000000 ) ) ;
#46093=EDGE_CURVE ( 'NONE', #46904, #17107, #39383, .T. ) ;
#46097=ORIENTED_EDGE ( 'NONE', *, *, #36689, .F. ) ;
#46098=CARTESIAN_POINT ( 'NONE',  ( 74.32915281903215998, 1.750000000000009548, -38.15658617722494483 ) ) ;
#46101=ORIENTED_EDGE ( 'NONE', *, *, #50578, .F. ) ;
#46104=DIRECTION ( 'NONE',  ( -1.000000000000000000, -0.000000000000000000, -0.000000000000000000 ) ) ;
#46106=CARTESIAN_POINT ( 'NONE',  ( 210.0000000000000568, 0.000000000000000000, -119.1817124430720440 ) ) ;
#46107=ORIENTED_EDGE ( 'NONE', *, *, #25852, .T. ) ;
#46108=AXIS2_PLACEMENT_3D ( 'NONE', #10962, #46072, #18147 ) ;
#46114=CARTESIAN_POINT ( 'NONE',  ( 151.5540265531850537, 0.000000000000000000, 82.56828755692798438 ) ) ;
#46116=DIRECTION ( 'NONE',  ( -1.000000000000000000, 0.000000000000000000, 0.000000000000000000 ) ) ;
#46118=CARTESIAN_POINT ( 'NONE',  ( -204.9459734468149463, 2.143131898507880377E-16, -117.4317124430720725 ) ) ;
#46119=CARTESIAN_POINT ( 'NONE',  ( -6.695973446814940111, -1.750000000000023759, -39.18171244307202983 ) ) ;
#46120=CARTESIAN_POINT ( 'NONE',  ( -127.7210997126620242, -1.749999999999996891, -120.2068387089191219 ) ) ;
#46121=CARTESIAN_POINT ( 'NONE',  ( -46.69597344681494633, -1.750000000000010214, 40.81828755692798438 ) ) ;
#46126=DIRECTION ( 'NONE',  ( 1.000000000000000000, 0.000000000000000000, 0.000000000000000000 ) ) ;
#46128=CARTESIAN_POINT ( 'NONE',  ( 73.30402655318508209, 1.750000000000009992, 0.8182875569279768335 ) ) ;
#46130=CYLINDRICAL_SURFACE ( 'NONE', #20699, 1.750000000000015543 ) ;
#46131=ORIENTED_EDGE ( 'NONE', *, *, #5525, .F. ) ;
#46133=ORIENTED_EDGE ( 'NONE', *, *, #25848, .F. ) ;
#46135=DIRECTION ( 'NONE',  ( -1.000000000000000000, -0.000000000000000000, -0.000000000000000000 ) ) ;
#46143=EDGE_CURVE ( 'NONE', #35861, #20525, #15263, .T. ) ;
#46145=CYLINDRICAL_SURFACE ( 'NONE', #20478, 1.750000000000015543 ) ;
#46147=ORIENTED_EDGE ( 'NONE', *, *, #49113, .F. ) ;
#46148=CARTESIAN_POINT ( 'NONE',  ( -85.67084718096784002, 1.750000000000010214, 121.8434138227750623 ) ) ;
#46149=CARTESIAN_POINT ( 'NONE',  ( 195.0540265531851105, 1.025126265847089435, -40.93171244307204404 ) ) ;
#46155=EDGE_CURVE ( 'NONE', #829, #20412, #44558, .T. ) ;
#46156=CARTESIAN_POINT ( 'NONE',  ( 151.5540265531850537, 0.000000000000000000, 2.568287556927978166 ) ) ;
#46158=EDGE_CURVE ( 'NONE', #47386, #36841, #49785, .T. ) ;
#46160=VERTEX_POINT ( 'NONE', #15499 ) ;
#46166=CARTESIAN_POINT ( 'NONE',  ( -4.945973446814903696, 2.143131898507912917E-16, 82.56828755692801280 ) ) ;
#46174=DIRECTION ( 'NONE',  ( -1.000000000000000000, 0.000000000000000000, 0.000000000000000000 ) ) ;
#46183=CARTESIAN_POINT ( 'NONE',  ( 31.55402655318503236, -1.025126265847089435, 39.06828755692797728 ) ) ;
#46189=CARTESIAN_POINT ( 'NONE',  ( 210.0000000000000568, 0.000000000000000000, -37.43171244307202272 ) ) ;
#46198=( BOUNDED_CURVE ( )  B_SPLINE_CURVE ( 3, ( #36307, #36052, #1145, #35543 ),
 .UNSPECIFIED., .F., .F. ) 
 B_SPLINE_CURVE_WITH_KNOTS ( ( 4, 4 ),
 ( 1.570796326794896558, 3.141592653589793116 ),
 .UNSPECIFIED. ) 
 CURVE ( )  GEOMETRIC_REPRESENTATION_ITEM ( )  RATIONAL_B_SPLINE_CURVE ( ( 1.000000000000000000, 0.8047378541243649375, 0.8047378541243649375, 1.000000000000000000 ) ) 
 REPRESENTATION_ITEM ( '' )  );
#46202=EDGE_LOOP ( 'NONE', ( #7480, #48752, #5355, #40538, #35731 ) ) ;
#46203=DIRECTION ( 'NONE',  ( -0.000000000000000000, -0.000000000000000000, -1.000000000000000000 ) ) ;
#46204=CARTESIAN_POINT ( 'NONE',  ( -164.9459734468149463, 2.143131898507880377E-16, -40.93171244307202983 ) ) ;
#46205=CARTESIAN_POINT ( 'NONE',  ( -44.94597344681493922, 2.143131898507880377E-16, 159.0682875569279702 ) ) ;
#46207=CYLINDRICAL_SURFACE ( 'NONE', #37625, 1.750000000000001554 ) ;
#46208=CARTESIAN_POINT ( 'NONE',  ( -124.9459734468149321, 1.025126265847081219, 162.5682875569279133 ) ) ;
#46213=DIRECTION ( 'NONE',  ( -1.000000000000000000, -0.000000000000000000, -0.000000000000000000 ) ) ;
#46221=AXIS2_PLACEMENT_3D ( 'NONE', #33663, #6450, #49757 ) ;
#46225=ORIENTED_EDGE ( 'NONE', *, *, #27807, .F. ) ;
#46226=ORIENTED_EDGE ( 'NONE', *, *, #50404, .F. ) ;
#46227=CARTESIAN_POINT ( 'NONE',  ( -127.7210997126620242, -1.749999999999996891, -118.1565861772249661 ) ) ;
#46228=CARTESIAN_POINT ( 'NONE',  ( 191.5540265531850537, -1.025126265847089435, 39.06828755692797728 ) ) ;
#46231=DIRECTION ( 'NONE',  ( -1.000000000000000000, 0.000000000000000000, 0.000000000000000000 ) ) ;
#46235=CYLINDRICAL_SURFACE ( 'NONE', #23043, 1.750000000000015543 ) ;
#46238=VECTOR ( 'NONE', #44005, 1000.000000000000000 ) ;
#46239=ORIENTED_EDGE ( 'NONE', *, *, #31152, .T. ) ;
#46240=ORIENTED_EDGE ( 'NONE', *, *, #26331, .F. ) ;
#46245=ORIENTED_EDGE ( 'NONE', *, *, #12659, .T. ) ;
#46246=ORIENTED_EDGE ( 'NONE', *, *, #37452, .F. ) ;
#46247=DIRECTION ( 'NONE',  ( -1.000000000000000000, 0.000000000000000000, 0.000000000000000000 ) ) ;
#46250=CARTESIAN_POINT ( 'NONE',  ( -168.4459734468149463, 0.000000000000000000, -40.93171244307202983 ) ) ;
#46253=ADVANCED_FACE ( 'NONE', ( #26164 ), #14608, .T. ) ;
#46255=CARTESIAN_POINT ( 'NONE',  ( -206.6959734468149463, 1.750000000000010658, -79.18171244307201562 ) ) ;
#46267=VECTOR ( 'NONE', #29217, 1000.000000000000000 ) ;
#46274=ORIENTED_EDGE ( 'NONE', *, *, #9661, .F. ) ;
#46275=EDGE_LOOP ( 'NONE', ( #48505, #32068, #10338, #33343, #27697, #46225 ) ) ;
#46276=FACE_OUTER_BOUND ( 'NONE', #34234, .T. ) ;
#46278=AXIS2_PLACEMENT_3D ( 'NONE', #29569, #37797, #21361 ) ;
#46279=EDGE_CURVE ( 'NONE', #36017, #27788, #15173, .T. ) ;
#46285=DIRECTION ( 'NONE',  ( -1.000000000000000000, -0.000000000000000000, -0.000000000000000000 ) ) ;
#46290=EDGE_CURVE ( 'NONE', #31511, #29900, #11279, .T. ) ;
#46293=LINE ( 'NONE', #18112, #4504 ) ;
#46296=EDGE_CURVE ( 'NONE', #10383, #48103, #20409, .T. ) ;
#46298=ORIENTED_EDGE ( 'NONE', *, *, #30901, .T. ) ;
#46301=CARTESIAN_POINT ( 'NONE',  ( -46.69597344681494633, -1.750000000000010658, -119.1817124430720440 ) ) ;
#46303=( BOUNDED_CURVE ( )  B_SPLINE_CURVE ( 3, ( #20897, #28096, #24257, #21393 ),
 .UNSPECIFIED., .F., .F. ) 
 B_SPLINE_CURVE_WITH_KNOTS ( ( 4, 4 ),
 ( 4.712388980384689674, 6.283185307179586232 ),
 .UNSPECIFIED. ) 
 CURVE ( )  GEOMETRIC_REPRESENTATION_ITEM ( )  RATIONAL_B_SPLINE_CURVE ( ( 1.000000000000000000, 0.8047378541243649375, 0.8047378541243649375, 1.000000000000000000 ) ) 
 REPRESENTATION_ITEM ( '' )  );
#46306=CARTESIAN_POINT ( 'NONE',  ( -46.69597344681494633, 1.750000000000009992, 160.8182875569279702 ) ) ;
#46308=FACE_OUTER_BOUND ( 'NONE', #33130, .T. ) ;
#46312=PLANE ( 'NONE',  #1228 ) ;
#46316=CARTESIAN_POINT ( 'NONE',  ( -208.4459734468148611, 1.025126265847089657, 79.06828755692797017 ) ) ;
#46322=CARTESIAN_POINT ( 'NONE',  ( 35.05402655318504657, 2.143131898507880377E-16, -120.9317124430720725 ) ) ;
#46325=DIRECTION ( 'NONE',  ( -0.000000000000000000, -0.000000000000000000, -1.000000000000000000 ) ) ;
#46326=AXIS2_PLACEMENT_3D ( 'NONE', #26131, #10483, #18173 ) ;
#46329=ORIENTED_EDGE ( 'NONE', *, *, #18952, .F. ) ;
#46331=CARTESIAN_POINT ( 'NONE',  ( 31.55402655318503236, 0.000000000000000000, 79.06828755692797017 ) ) ;
#46333=CIRCLE ( 'NONE', #7039, 1.750000000000015543 ) ;
#46336=AXIS2_PLACEMENT_3D ( 'NONE', #38638, #42211, #22710 ) ;
#46337=VERTEX_POINT ( 'NONE', #34378 ) ;
#46347=ORIENTED_EDGE ( 'NONE', *, *, #17207, .T. ) ;
#46348=ORIENTED_EDGE ( 'NONE', *, *, #28784, .F. ) ;
#46351=EDGE_CURVE ( 'NONE', #42713, #14002, #6333, .T. ) ;
#46356=DIRECTION ( 'NONE',  ( -1.000000000000000000, -0.000000000000000000, -0.000000000000000000 ) ) ;
#46360=CARTESIAN_POINT ( 'NONE',  ( -128.4459734468149463, -1.025126265847081664, -157.4317124430720582 ) ) ;
#46364=( BOUNDED_CURVE ( )  B_SPLINE_CURVE ( 3, ( #5831, #44544, #33044, #20724 ),
 .UNSPECIFIED., .F., .F. ) 
 B_SPLINE_CURVE_WITH_KNOTS ( ( 4, 4 ),
 ( 1.570796326794896558, 3.141592653589793116 ),
 .UNSPECIFIED. ) 
 CURVE ( )  GEOMETRIC_REPRESENTATION_ITEM ( )  RATIONAL_B_SPLINE_CURVE ( ( 1.000000000000000000, 0.8047378541243649375, 0.8047378541243649375, 1.000000000000000000 ) ) 
 REPRESENTATION_ITEM ( '' )  );
#46373=EDGE_CURVE ( 'NONE', #29572, #13781, #6033, .T. ) ;
#46374=( BOUNDED_CURVE ( )  B_SPLINE_CURVE ( 3, ( #50214, #26925, #26173, #38999 ),
 .UNSPECIFIED., .F., .F. ) 
 B_SPLINE_CURVE_WITH_KNOTS ( ( 4, 4 ),
 ( 0.000000000000000000, 1.570796326794896558 ),
 .UNSPECIFIED. ) 
 CURVE ( )  GEOMETRIC_REPRESENTATION_ITEM ( )  RATIONAL_B_SPLINE_CURVE ( ( 1.000000000000000000, 0.8047378541243649375, 0.8047378541243649375, 1.000000000000000000 ) ) 
 REPRESENTATION_ITEM ( '' )  );
#46376=ORIENTED_EDGE ( 'NONE', *, *, #37207, .F. ) ;
#46377=AXIS2_PLACEMENT_3D ( 'NONE', #30885, #22906, #39592 ) ;
#46379=CARTESIAN_POINT ( 'NONE',  ( -7.721099712662037540, 1.750000000000023981, -120.2068387089191219 ) ) ;
#46382=DIRECTION ( 'NONE',  ( 0.000000000000000000, 0.000000000000000000, 1.000000000000000000 ) ) ;
#46383=CYLINDRICAL_SURFACE ( 'NONE', #29027, 1.750000000000036193 ) ;
#46384=LINE ( 'NONE', #15114, #31700 ) ;
#46385=CARTESIAN_POINT ( 'NONE',  ( 193.3040265531851105, 1.750000000000010214, -39.18171244307202983 ) ) ;
#46387=VERTEX_POINT ( 'NONE', #31804 ) ;
#46395=FACE_OUTER_BOUND ( 'NONE', #26880, .T. ) ;
#46401=ORIENTED_EDGE ( 'NONE', *, *, #5298, .F. ) ;
#46403=ORIENTED_EDGE ( 'NONE', *, *, #14200, .F. ) ;
#46410=AXIS2_PLACEMENT_3D ( 'NONE', #25766, #14970, #46231 ) ;
#46412=CARTESIAN_POINT ( 'NONE',  ( -86.69597344681494633, 1.750000000000010214, -39.18171244307202983 ) ) ;
#46416=CARTESIAN_POINT ( 'NONE',  ( 33.30402655318503946, -1.750000000000009992, 0.8182875569279768335 ) ) ;
#46417=CARTESIAN_POINT ( 'NONE',  ( -48.44597344681495343, 0.000000000000000000, -80.93171244307204404 ) ) ;
#46418=ORIENTED_EDGE ( 'NONE', *, *, #26488, .F. ) ;
#46423=VECTOR ( 'NONE', #41550, 1000.000000000000000 ) ;
#46429=ORIENTED_EDGE ( 'NONE', *, *, #19317, .T. ) ;
#46430=CARTESIAN_POINT ( 'NONE',  ( 33.30402655318503946, -1.750000000000009992, -159.1817124430720298 ) ) ;
#46431=CARTESIAN_POINT ( 'NONE',  ( -8.445973446814976526, 0.000000000000000000, -77.43171244307198720 ) ) ;
#46441=CARTESIAN_POINT ( 'NONE',  ( 32.27890028733795447, -1.750000000000009548, 39.79316129108089228 ) ) ;
#46448=CYLINDRICAL_SURFACE ( 'NONE', #44166, 1.750000000000001554 ) ;
#46449=CARTESIAN_POINT ( 'NONE',  ( -164.9459734468149463, 2.143131898507890731E-16, -165.0000000000000000 ) ) ;
#46450=CARTESIAN_POINT ( 'NONE',  ( -166.6959734468149463, 1.750000000000010658, 80.81828755692798438 ) ) ;
#46455=ORIENTED_EDGE ( 'NONE', *, *, #47222, .T. ) ;
#46459=ORIENTED_EDGE ( 'NONE', *, *, #458, .T. ) ;
#46461=CARTESIAN_POINT ( 'NONE',  ( 153.3040265531850537, 1.750000000000009992, 0.8182875569279768335 ) ) ;
#46462=ORIENTED_EDGE ( 'NONE', *, *, #22248, .T. ) ;
#46465=DIRECTION ( 'NONE',  ( 0.000000000000000000, 0.000000000000000000, 1.000000000000000000 ) ) ;
#46466=ORIENTED_EDGE ( 'NONE', *, *, #37276, .T. ) ;
#46473=CARTESIAN_POINT ( 'NONE',  ( -44.94597344681493922, -1.025126265847089435, -77.43171244307200141 ) ) ;
#46479=ORIENTED_EDGE ( 'NONE', *, *, #31186, .T. ) ;
#46485=ORIENTED_EDGE ( 'NONE', *, *, #33145, .F. ) ;
#46489=CARTESIAN_POINT ( 'NONE',  ( -206.6959734468149463, 1.750000000000010658, 120.8182875569279702 ) ) ;
#46495=DIRECTION ( 'NONE',  ( -0.000000000000000000, -0.000000000000000000, -1.000000000000000000 ) ) ;
#46497=( BOUNDED_CURVE ( )  B_SPLINE_CURVE ( 3, ( #36542, #872, #37048, #17013 ),
 .UNSPECIFIED., .F., .F. ) 
 B_SPLINE_CURVE_WITH_KNOTS ( ( 4, 4 ),
 ( 3.141592653589793116, 4.712388980384689674 ),
 .UNSPECIFIED. ) 
 CURVE ( )  GEOMETRIC_REPRESENTATION_ITEM ( )  RATIONAL_B_SPLINE_CURVE ( ( 1.000000000000000000, 0.8047378541243649375, 0.8047378541243649375, 1.000000000000000000 ) ) 
 REPRESENTATION_ITEM ( '' )  );
#46502=ORIENTED_EDGE ( 'NONE', *, *, #49974, .T. ) ;
#46505=( BOUNDED_CURVE ( )  B_SPLINE_CURVE ( 3, ( #22730, #19390, #6833, #30435 ),
 .UNSPECIFIED., .F., .F. ) 
 B_SPLINE_CURVE_WITH_KNOTS ( ( 4, 4 ),
 ( 1.570796326794896558, 3.141592653589793116 ),
 .UNSPECIFIED. ) 
 CURVE ( )  GEOMETRIC_REPRESENTATION_ITEM ( )  RATIONAL_B_SPLINE_CURVE ( ( 1.000000000000000000, 0.8047378541243649375, 0.8047378541243649375, 1.000000000000000000 ) ) 
 REPRESENTATION_ITEM ( '' )  );
#46508=CARTESIAN_POINT ( 'NONE',  ( -168.4459734468149747, -1.025126265847089213, 162.5682875569279133 ) ) ;
#46511=EDGE_CURVE ( 'NONE', #16197, #3985, #11583, .T. ) ;
#46518=DIRECTION ( 'NONE',  ( -0.000000000000000000, -0.000000000000000000, -1.000000000000000000 ) ) ;
#46520=( BOUNDED_CURVE ( )  B_SPLINE_CURVE ( 3, ( #3618, #11324, #39051, #34692 ),
 .UNSPECIFIED., .F., .F. ) 
 B_SPLINE_CURVE_WITH_KNOTS ( ( 4, 4 ),
 ( 1.570796326794896558, 3.141592653589793116 ),
 .UNSPECIFIED. ) 
 CURVE ( )  GEOMETRIC_REPRESENTATION_ITEM ( )  RATIONAL_B_SPLINE_CURVE ( ( 1.000000000000000000, 0.8047378541243649375, 0.8047378541243649375, 1.000000000000000000 ) ) 
 REPRESENTATION_ITEM ( '' )  );
#46522=ORIENTED_EDGE ( 'NONE', *, *, #49008, .T. ) ;
#46527=EDGE_LOOP ( 'NONE', ( #23085, #32285, #10914, #1286, #17760, #34281 ) ) ;
#46528=EDGE_LOOP ( 'NONE', ( #48011, #2382, #31762, #19475, #36333, #31130 ) ) ;
#46533=ORIENTED_EDGE ( 'NONE', *, *, #29761, .F. ) ;
#46535=ORIENTED_EDGE ( 'NONE', *, *, #2659, .T. ) ;
#46541=VERTEX_POINT ( 'NONE', #41243 ) ;
#46543=CARTESIAN_POINT ( 'NONE',  ( -48.44597344681496054, -1.025126265847089213, -160.9317124430720014 ) ) ;
#46547=ORIENTED_EDGE ( 'NONE', *, *, #11238, .F. ) ;
#46549=CARTESIAN_POINT ( 'NONE',  ( 35.05402655318504657, 2.143131898507880377E-16, -37.43171244307200141 ) ) ;
#46552=LINE ( 'NONE', #31730, #32263 ) ;
#46556=CARTESIAN_POINT ( 'NONE',  ( -208.4459734468149463, 0.000000000000000000, -77.43171244307204404 ) ) ;
#46560=CARTESIAN_POINT ( 'NONE',  ( 210.0000000000000568, 0.000000000000000000, 120.8182875569279702 ) ) ;
#46561=CARTESIAN_POINT ( 'NONE',  ( -206.6959734468149463, 1.750000000000010658, 80.81828755692798438 ) ) ;
#46562=AXIS2_PLACEMENT_3D ( 'NONE', #939, #36098, #43766 ) ;
#46563=EDGE_CURVE ( 'NONE', #34063, #16264, #43031, .T. ) ;
#46570=CARTESIAN_POINT ( 'NONE',  ( -87.72109971266203843, 1.750000000000009548, -78.15658617722490931 ) ) ;
#46583=CARTESIAN_POINT ( 'NONE',  ( 71.55402655318505367, 0.000000000000000000, 39.06828755692795596 ) ) ;
#46586=EDGE_CURVE ( 'NONE', #33796, #12365, #29697, .T. ) ;
#46587=ORIENTED_EDGE ( 'NONE', *, *, #28702, .F. ) ;
#46588=CARTESIAN_POINT ( 'NONE',  ( 210.0000000000000568, 2.143131898507881856E-16, -120.9317124430720582 ) ) ;
#46589=ORIENTED_EDGE ( 'NONE', *, *, #50436, .F. ) ;
#46595=EDGE_CURVE ( 'NONE', #42421, #50239, #9528, .T. ) ;
#46598=( BOUNDED_CURVE ( )  B_SPLINE_CURVE ( 3, ( #29818, #13153, #29062, #49005 ),
 .UNSPECIFIED., .F., .F. ) 
 B_SPLINE_CURVE_WITH_KNOTS ( ( 4, 4 ),
 ( 1.570796326794896558, 3.141592653589793116 ),
 .UNSPECIFIED. ) 
 CURVE ( )  GEOMETRIC_REPRESENTATION_ITEM ( )  RATIONAL_B_SPLINE_CURVE ( ( 1.000000000000000000, 0.8047378541243649375, 0.8047378541243649375, 1.000000000000000000 ) ) 
 REPRESENTATION_ITEM ( '' )  );
#46602=CARTESIAN_POINT ( 'NONE',  ( 31.55402655318503236, 0.000000000000000000, 165.0000000000000000 ) ) ;
#46604=CARTESIAN_POINT ( 'NONE',  ( 31.55402655318503236, 1.025126265847089213, 162.5682875569279133 ) ) ;
#46611=VERTEX_POINT ( 'NONE', #44317 ) ;
#46612=ORIENTED_EDGE ( 'NONE', *, *, #29011, .T. ) ;
#46623=CARTESIAN_POINT ( 'NONE',  ( -6.695973446814940111, 1.750000000000023315, 0.8182875569279768335 ) ) ;
#46626=VECTOR ( 'NONE', #27197, 1000.000000000000000 ) ;
#46627=CARTESIAN_POINT ( 'NONE',  ( -206.6959734468149463, -1.750000000000010658, -119.1817124430720440 ) ) ;
#46632=DIRECTION ( 'NONE',  ( 0.000000000000000000, 0.000000000000000000, -1.000000000000000000 ) ) ;
#46633=CARTESIAN_POINT ( 'NONE',  ( 33.30402655318503946, 0.000000000000000000, 165.0000000000000000 ) ) ;
#46636=VECTOR ( 'NONE', #50512, 1000.000000000000000 ) ;
#46640=CARTESIAN_POINT ( 'NONE',  ( -87.72109971266203843, 1.750000000000009326, 1.843413822775066269 ) ) ;
#46644=AXIS2_PLACEMENT_3D ( 'NONE', #32752, #25552, #8888 ) ;
#46645=EDGE_LOOP ( 'NONE', ( #8860, #1485, #36165, #44573, #12008, #10096 ) ) ;
#46647=VERTEX_POINT ( 'NONE', #10956 ) ;
#46649=ORIENTED_EDGE ( 'NONE', *, *, #3966, .F. ) ;
#46652=CARTESIAN_POINT ( 'NONE',  ( -126.6959734468149321, 1.749999999999997335, -79.18171244307201562 ) ) ;
#46653=EDGE_CURVE ( 'NONE', #9039, #48199, #13218, .T. ) ;
#46655=CARTESIAN_POINT ( 'NONE',  ( 154.3291528190321458, 1.750000000000009548, 159.7931612910809065 ) ) ;
#46657=( BOUNDED_CURVE ( )  B_SPLINE_CURVE ( 3, ( #5821, #21215, #44534, #12764 ),
 .UNSPECIFIED., .F., .F. ) 
 B_SPLINE_CURVE_WITH_KNOTS ( ( 4, 4 ),
 ( 1.570796326794896558, 3.141592653589793116 ),
 .UNSPECIFIED. ) 
 CURVE ( )  GEOMETRIC_REPRESENTATION_ITEM ( )  RATIONAL_B_SPLINE_CURVE ( ( 1.000000000000000000, 0.8047378541243649375, 0.8047378541243649375, 1.000000000000000000 ) ) 
 REPRESENTATION_ITEM ( '' )  );
#46659=CARTESIAN_POINT ( 'NONE',  ( 191.5540265531851105, 0.000000000000000000, 82.56828755692798438 ) ) ;
#46665=( BOUNDED_CURVE ( )  B_SPLINE_CURVE ( 3, ( #1383, #8576, #24229, #20361 ),
 .UNSPECIFIED., .F., .F. ) 
 B_SPLINE_CURVE_WITH_KNOTS ( ( 4, 4 ),
 ( 0.000000000000000000, 1.570796326794896558 ),
 .UNSPECIFIED. ) 
 CURVE ( )  GEOMETRIC_REPRESENTATION_ITEM ( )  RATIONAL_B_SPLINE_CURVE ( ( 1.000000000000000000, 0.8047378541243649375, 0.8047378541243649375, 1.000000000000000000 ) ) 
 REPRESENTATION_ITEM ( '' )  );
#46670=VECTOR ( 'NONE', #15709, 1000.000000000000000 ) ;
#46676=DIRECTION ( 'NONE',  ( 0.000000000000000000, 0.000000000000000000, 1.000000000000000000 ) ) ;
#46679=CARTESIAN_POINT ( 'NONE',  ( -87.72109971266203843, 1.750000000000010436, 119.7931612910808781 ) ) ;
#46686=CARTESIAN_POINT ( 'NONE',  ( -128.4459734468149179, 0.000000000000000000, -0.9317124430719969652 ) ) ;
#46687=ORIENTED_EDGE ( 'NONE', *, *, #47287, .T. ) ;
#46691=ORIENTED_EDGE ( 'NONE', *, *, #24340, .T. ) ;
#46692=ORIENTED_EDGE ( 'NONE', *, *, #25798, .T. ) ;
#46694=CARTESIAN_POINT ( 'NONE',  ( -206.6959734468149463, -1.750000000000009992, -159.1817124430720298 ) ) ;
#46695=CARTESIAN_POINT ( 'NONE',  ( -48.44597344681495343, 0.000000000000000000, 165.0000000000000000 ) ) ;
#46698=FACE_OUTER_BOUND ( 'NONE', #27654, .T. ) ;
#46707=EDGE_LOOP ( 'NONE', ( #39429, #4367, #12697, #15091, #19450, #27853 ) ) ;
#46708=ADVANCED_FACE ( 'NONE', ( #18391 ), #22500, .T. ) ;
#46709=VECTOR ( 'NONE', #28112, 1000.000000000000000 ) ;
#46712=VECTOR ( 'NONE', #30317, 1000.000000000000000 ) ;
#46717=CARTESIAN_POINT ( 'NONE',  ( 152.2789002873379900, 1.750000000000009548, -0.2068387089191121020 ) ) ;
#46718=VERTEX_POINT ( 'NONE', #18140 ) ;
#46722=FACE_OUTER_BOUND ( 'NONE', #34162, .T. ) ;
#46727=ORIENTED_EDGE ( 'NONE', *, *, #24747, .T. ) ;
#46728=CARTESIAN_POINT ( 'NONE',  ( -204.9459734468149463, 2.143131898507880377E-16, 165.0000000000000000 ) ) ;
#46730=ORIENTED_EDGE ( 'NONE', *, *, #1764, .T. ) ;
#46734=ADVANCED_FACE ( 'NONE', ( #29960 ), #33814, .T. ) ;
#46735=CARTESIAN_POINT ( 'NONE',  ( -128.4459734468149179, 0.000000000000000000, -40.93171244307202983 ) ) ;
#46743=CARTESIAN_POINT ( 'NONE',  ( 33.30402655318503946, -1.750000000000010658, -79.18171244307201562 ) ) ;
#46745=DIRECTION ( 'NONE',  ( 1.000000000000000000, 0.000000000000000000, -0.000000000000000000 ) ) ;
#46746=AXIS2_PLACEMENT_3D ( 'NONE', #31178, #16030, #11927 ) ;
#46747=ORIENTED_EDGE ( 'NONE', *, *, #25519, .F. ) ;
#46749=ORIENTED_EDGE ( 'NONE', *, *, #22860, .F. ) ;
#46755=ORIENTED_EDGE ( 'NONE', *, *, #30470, .T. ) ;
#46756=ORIENTED_EDGE ( 'NONE', *, *, #48675, .F. ) ;
#46758=CARTESIAN_POINT ( 'NONE',  ( 191.5540265531850537, -1.025126265847089657, 42.56828755692799149 ) ) ;
#46764=CARTESIAN_POINT ( 'NONE',  ( -164.9459734468149463, 2.143131898507880377E-16, -0.9317124430720247208 ) ) ;
#46769=CYLINDRICAL_SURFACE ( 'NONE', #17227, 1.750000000000001554 ) ;
#46770=CARTESIAN_POINT ( 'NONE',  ( 154.3291528190321458, -1.750000000000009548, 121.8434138227750623 ) ) ;
#46772=AXIS2_PLACEMENT_3D ( 'NONE', #11717, #50149, #34836 ) ;
#46775=ORIENTED_EDGE ( 'NONE', *, *, #44313, .T. ) ;
#46777=VERTEX_POINT ( 'NONE', #25512 ) ;
#46778=FACE_OUTER_BOUND ( 'NONE', #49099, .T. ) ;
#46787=EDGE_LOOP ( 'NONE', ( #27502, #4701, #20066, #15786, #22299 ) ) ;
#46788=ORIENTED_EDGE ( 'NONE', *, *, #7072, .T. ) ;
#46792=CARTESIAN_POINT ( 'NONE',  ( 192.2789002873380184, -1.750000000000009548, -38.15658617722494483 ) ) ;
#46794=( BOUNDED_CURVE ( )  B_SPLINE_CURVE ( 3, ( #19816, #4428, #35495, #50307 ),
 .UNSPECIFIED., .F., .F. ) 
 B_SPLINE_CURVE_WITH_KNOTS ( ( 4, 4 ),
 ( 0.000000000000000000, 1.570796326794896558 ),
 .UNSPECIFIED. ) 
 CURVE ( )  GEOMETRIC_REPRESENTATION_ITEM ( )  RATIONAL_B_SPLINE_CURVE ( ( 1.000000000000000000, 0.8047378541243649375, 0.8047378541243649375, 1.000000000000000000 ) ) 
 REPRESENTATION_ITEM ( '' )  );
#46799=DIRECTION ( 'NONE',  ( 1.000000000000000000, 0.000000000000000000, 0.000000000000000000 ) ) ;
#46804=( BOUNDED_CURVE ( )  B_SPLINE_CURVE ( 3, ( #21227, #36915, #4576, #47628 ),
 .UNSPECIFIED., .F., .F. ) 
 B_SPLINE_CURVE_WITH_KNOTS ( ( 4, 4 ),
 ( 3.141592653589793116, 4.712388980384689674 ),
 .UNSPECIFIED. ) 
 CURVE ( )  GEOMETRIC_REPRESENTATION_ITEM ( )  RATIONAL_B_SPLINE_CURVE ( ( 1.000000000000000000, 0.8047378541243649375, 0.8047378541243649375, 1.000000000000000000 ) ) 
 REPRESENTATION_ITEM ( '' )  );
#46806=VECTOR ( 'NONE', #36995, 1000.000000000000000 ) ;
#46807=ADVANCED_FACE ( 'NONE', ( #49066 ), #2657, .T. ) ;
#46811=CARTESIAN_POINT ( 'NONE',  ( 73.30402655318508209, 1.750000000000009992, -159.1817124430720298 ) ) ;
#46812=EDGE_LOOP ( 'NONE', ( #26224, #16364, #49731, #27407, #38584, #20423 ) ) ;
#46816=CARTESIAN_POINT ( 'NONE',  ( -86.69597344681494633, -1.750000000000010658, 120.8182875569279702 ) ) ;
#46819=DIRECTION ( 'NONE',  ( -1.000000000000000000, -0.000000000000000000, -0.000000000000000000 ) ) ;
#46820=( BOUNDED_CURVE ( )  B_SPLINE_CURVE ( 3, ( #3539, #24082, #35647, #27166 ),
 .UNSPECIFIED., .F., .F. ) 
 B_SPLINE_CURVE_WITH_KNOTS ( ( 4, 4 ),
 ( 3.141592653589793116, 4.712388980384689674 ),
 .UNSPECIFIED. ) 
 CURVE ( )  GEOMETRIC_REPRESENTATION_ITEM ( )  RATIONAL_B_SPLINE_CURVE ( ( 1.000000000000000000, 0.8047378541243649375, 0.8047378541243649375, 1.000000000000000000 ) ) 
 REPRESENTATION_ITEM ( '' )  );
#46821=CARTESIAN_POINT ( 'NONE',  ( 111.5540265531850679, 0.000000000000000000, 119.0682875569279844 ) ) ;
#46824=EDGE_CURVE ( 'NONE', #13712, #11195, #21658, .T. ) ;
#46835=CARTESIAN_POINT ( 'NONE',  ( 71.55402655318505367, 0.000000000000000000, -0.9317124430720524764 ) ) ;
#46839=CARTESIAN_POINT ( 'NONE',  ( 210.0000000000000568, 0.000000000000000000, 80.81828755692798438 ) ) ;
#46841=AXIS2_PLACEMENT_3D ( 'NONE', #29054, #41358, #16999 ) ;
#46843=CARTESIAN_POINT ( 'NONE',  ( -166.6959734468149463, -1.750000000000010658, -119.1817124430720440 ) ) ;
#46847=EDGE_CURVE ( 'NONE', #4637, #40403, #22054, .T. ) ;
#46848=ORIENTED_EDGE ( 'NONE', *, *, #13316, .F. ) ;
#46851=CARTESIAN_POINT ( 'NONE',  ( -126.6959734468149321, 0.000000000000000000, 165.0000000000000000 ) ) ;
#46854=ORIENTED_EDGE ( 'NONE', *, *, #38876, .T. ) ;
#46855=CARTESIAN_POINT ( 'NONE',  ( 72.27890028733797578, 1.750000000000009548, 121.8434138227750623 ) ) ;
#46864=ORIENTED_EDGE ( 'NONE', *, *, #6052, .F. ) ;
#46866=ADVANCED_FACE ( 'NONE', ( #50549 ), #42637, .T. ) ;
#46875=CARTESIAN_POINT ( 'NONE',  ( 152.2789002873379900, -1.750000000000010214, 81.84341382277507648 ) ) ;
#46877=DIRECTION ( 'NONE',  ( -1.000000000000000000, -0.000000000000000000, -0.000000000000000000 ) ) ;
#46881=CARTESIAN_POINT ( 'NONE',  ( 31.55402655318503236, 0.000000000000000000, -120.9317124430720725 ) ) ;
#46890=ORIENTED_EDGE ( 'NONE', *, *, #40902, .F. ) ;
#46893=CARTESIAN_POINT ( 'NONE',  ( -86.69597344681494633, 1.750000000000009992, 0.8182875569279768335 ) ) ;
#46895=VERTEX_POINT ( 'NONE', #50295 ) ;
#46901=CARTESIAN_POINT ( 'NONE',  ( 210.0000000000000568, 2.143131898507881116E-16, 39.06828755692797728 ) ) ;
#46902=CARTESIAN_POINT ( 'NONE',  ( 194.3291528190321742, 1.750000000000010214, 121.8434138227750623 ) ) ;
#46904=VERTEX_POINT ( 'NONE', #49786 ) ;
#46905=LINE ( 'NONE', #38002, #43686 ) ;
#46906=ORIENTED_EDGE ( 'NONE', *, *, #41357, .F. ) ;
#46908=CARTESIAN_POINT ( 'NONE',  ( 71.55402655318505367, -1.025126265847089213, 162.5682875569279133 ) ) ;
#46911=CARTESIAN_POINT ( 'NONE',  ( -86.69597344681494633, 1.750000000000010658, 120.8182875569279702 ) ) ;
#46914=CARTESIAN_POINT ( 'NONE',  ( 192.2789002873380184, 1.750000000000009548, 161.8434138227750907 ) ) ;
#46917=AXIS2_PLACEMENT_3D ( 'NONE', #17593, #33268, #21190 ) ;
#46924=CARTESIAN_POINT ( 'NONE',  ( 191.5540265531851105, 0.000000000000000000, -0.9317124430720247208 ) ) ;
#46926=EDGE_CURVE ( 'NONE', #37586, #38893, #14440, .T. ) ;
#46944=CARTESIAN_POINT ( 'NONE',  ( 111.5540265531850679, 0.000000000000000000, -80.93171244307201562 ) ) ;
#46945=CARTESIAN_POINT ( 'NONE',  ( 35.05402655318504657, 2.143131898507880377E-16, -117.4317124430720156 ) ) ;
#46947=CIRCLE ( 'NONE', #21600, 1.749999999999987566 ) ;
#46950=EDGE_LOOP ( 'NONE', ( #18624, #32159, #20593, #38346, #26463, #34037 ) ) ;
#46952=VECTOR ( 'NONE', #46819, 1000.000000000000000 ) ;
#46953=DIRECTION ( 'NONE',  ( -1.000000000000000000, 0.000000000000000000, 0.000000000000000000 ) ) ;
#46956=( BOUNDED_CURVE ( )  B_SPLINE_CURVE ( 3, ( #33437, #49011, #21879, #37543 ),
 .UNSPECIFIED., .F., .F. ) 
 B_SPLINE_CURVE_WITH_KNOTS ( ( 4, 4 ),
 ( 4.712388980384689674, 6.283185307179586232 ),
 .UNSPECIFIED. ) 
 CURVE ( )  GEOMETRIC_REPRESENTATION_ITEM ( )  RATIONAL_B_SPLINE_CURVE ( ( 1.000000000000000000, 0.8047378541243649375, 0.8047378541243649375, 1.000000000000000000 ) ) 
 REPRESENTATION_ITEM ( '' )  );
#46958=CARTESIAN_POINT ( 'NONE',  ( 152.2789002873379900, 1.750000000000009548, -40.20683870891912193 ) ) ;
#46959=VERTEX_POINT ( 'NONE', #46204 ) ;
#46962=ORIENTED_EDGE ( 'NONE', *, *, #23529, .T. ) ;
#46965=( BOUNDED_CURVE ( )  B_SPLINE_CURVE ( 3, ( #48680, #44593, #5878, #25141 ),
 .UNSPECIFIED., .F., .F. ) 
 B_SPLINE_CURVE_WITH_KNOTS ( ( 4, 4 ),
 ( 1.570796326794896558, 3.141592653589793116 ),
 .UNSPECIFIED. ) 
 CURVE ( )  GEOMETRIC_REPRESENTATION_ITEM ( )  RATIONAL_B_SPLINE_CURVE ( ( 1.000000000000000000, 0.8047378541243649375, 0.8047378541243649375, 1.000000000000000000 ) ) 
 REPRESENTATION_ITEM ( '' )  );
#46967=CARTESIAN_POINT ( 'NONE',  ( -4.945973446814903696, 2.143131898507912917E-16, 122.5682875569279986 ) ) ;
#46969=EDGE_CURVE ( 'NONE', #35861, #47433, #33948, .T. ) ;
#46970=VECTOR ( 'NONE', #17313, 1000.000000000000000 ) ;
#46973=EDGE_LOOP ( 'NONE', ( #13256, #4945, #2722, #45031, #26753, #28815 ) ) ;
#46976=CARTESIAN_POINT ( 'NONE',  ( 33.30402655318503946, 1.750000000000010658, 80.81828755692798438 ) ) ;
#46978=ORIENTED_EDGE ( 'NONE', *, *, #46595, .F. ) ;
#46979=VERTEX_POINT ( 'NONE', #41890 ) ;
#46980=DIRECTION ( 'NONE',  ( 0.000000000000000000, 0.000000000000000000, -1.000000000000000000 ) ) ;
#46981=ORIENTED_EDGE ( 'NONE', *, *, #4220, .F. ) ;
#46982=EDGE_CURVE ( 'NONE', #37466, #18505, #3382, .T. ) ;
#46992=LINE ( 'NONE', #44177, #49633 ) ;
#46999=ORIENTED_EDGE ( 'NONE', *, *, #3769, .T. ) ;
#47001=EDGE_CURVE ( 'NONE', #46611, #10420, #18454, .T. ) ;
#47003=CARTESIAN_POINT ( 'NONE',  ( -165.6708471809677974, 1.750000000000009548, -40.20683870891912193 ) ) ;
#47011=CIRCLE ( 'NONE', #19156, 1.750000000000015543 ) ;
#47014=ORIENTED_EDGE ( 'NONE', *, *, #1159, .F. ) ;
#47018=CARTESIAN_POINT ( 'NONE',  ( 115.0540265531850395, -1.025126265847081664, 42.56828755692797017 ) ) ;
#47019=CARTESIAN_POINT ( 'NONE',  ( -8.445973446814976526, 0.000000000000000000, -165.0000000000000000 ) ) ;
#47021=VECTOR ( 'NONE', #25252, 1000.000000000000000 ) ;
#47022=CARTESIAN_POINT ( 'NONE',  ( 195.0540265531851105, -1.025126265847089657, 79.06828755692797017 ) ) ;
#47026=CARTESIAN_POINT ( 'NONE',  ( -164.9459734468149463, 2.143131898507880377E-16, -157.4317124430720582 ) ) ;
#47030=CARTESIAN_POINT ( 'NONE',  ( 210.0000000000000568, 2.143131898507876926E-16, 119.0682875569279560 ) ) ;
#47036=CARTESIAN_POINT ( 'NONE',  ( 194.3291528190321742, -1.750000000000009548, -78.15658617722490931 ) ) ;
#47037=DIRECTION ( 'NONE',  ( -0.000000000000000000, -0.000000000000000000, -1.000000000000000000 ) ) ;
#47041=CARTESIAN_POINT ( 'NONE',  ( -124.9459734468149321, -1.025126265847081886, 39.06828755692799149 ) ) ;
#47044=DIRECTION ( 'NONE',  ( -0.000000000000000000, -0.000000000000000000, -1.000000000000000000 ) ) ;
#47048=ORIENTED_EDGE ( 'NONE', *, *, #28141, .T. ) ;
#47057=VERTEX_POINT ( 'NONE', #20310 ) ;
#47060=CARTESIAN_POINT ( 'NONE',  ( -45.67084718096785423, 1.750000000000009548, -40.20683870891912193 ) ) ;
#47061=CYLINDRICAL_SURFACE ( 'NONE', #26541, 1.750000000000001554 ) ;
#47066=VERTEX_POINT ( 'NONE', #24179 ) ;
#47067=CARTESIAN_POINT ( 'NONE',  ( 73.30402655318508209, 0.000000000000000000, 165.0000000000000000 ) ) ;
#47069=CARTESIAN_POINT ( 'NONE',  ( 151.5540265531850537, -1.025126265847089435, -40.93171244307204404 ) ) ;
#47070=ORIENTED_EDGE ( 'NONE', *, *, #17445, .T. ) ;
#47071=CARTESIAN_POINT ( 'NONE',  ( 75.05402655318509630, 2.143131898507880377E-16, 165.0000000000000000 ) ) ;
#47087=ORIENTED_EDGE ( 'NONE', *, *, #1093, .T. ) ;
#47088=CARTESIAN_POINT ( 'NONE',  ( 35.05402655318504657, -1.025126265847089213, 42.56828755692799149 ) ) ;
#47093=VERTEX_POINT ( 'NONE', #578 ) ;
#47096=FACE_OUTER_BOUND ( 'NONE', #17919, .T. ) ;
#47097=( BOUNDED_CURVE ( )  B_SPLINE_CURVE ( 3, ( #21325, #2821, #18479, #29280 ),
 .UNSPECIFIED., .F., .F. ) 
 B_SPLINE_CURVE_WITH_KNOTS ( ( 4, 4 ),
 ( 4.712388980384689674, 6.283185307179586232 ),
 .UNSPECIFIED. ) 
 CURVE ( )  GEOMETRIC_REPRESENTATION_ITEM ( )  RATIONAL_B_SPLINE_CURVE ( ( 1.000000000000000000, 0.8047378541243649375, 0.8047378541243649375, 1.000000000000000000 ) ) 
 REPRESENTATION_ITEM ( '' )  );
#47098=EDGE_LOOP ( 'NONE', ( #3390, #2757, #9922, #23118, #29830 ) ) ;
#47101=( BOUNDED_CURVE ( )  B_SPLINE_CURVE ( 3, ( #36231, #20805, #39316, #35473 ),
 .UNSPECIFIED., .F., .F. ) 
 B_SPLINE_CURVE_WITH_KNOTS ( ( 4, 4 ),
 ( 0.000000000000000000, 1.570796326794896558 ),
 .UNSPECIFIED. ) 
 CURVE ( )  GEOMETRIC_REPRESENTATION_ITEM ( )  RATIONAL_B_SPLINE_CURVE ( ( 1.000000000000000000, 0.8047378541243649375, 0.8047378541243649375, 1.000000000000000000 ) ) 
 REPRESENTATION_ITEM ( '' )  );
#47107=AXIS2_PLACEMENT_3D ( 'NONE', #13185, #41398, #1650 ) ;
#47109=ORIENTED_EDGE ( 'NONE', *, *, #7377, .T. ) ;
#47111=PLANE ( 'NONE',  #37432 ) ;
#47112=DIRECTION ( 'NONE',  ( -0.000000000000000000, -0.000000000000000000, -1.000000000000000000 ) ) ;
#47114=VECTOR ( 'NONE', #8452, 1000.000000000000000 ) ;
#47115=ORIENTED_EDGE ( 'NONE', *, *, #7621, .T. ) ;
#47120=( BOUNDED_CURVE ( )  B_SPLINE_CURVE ( 3, ( #33135, #48215, #28763, #44140 ),
 .UNSPECIFIED., .F., .F. ) 
 B_SPLINE_CURVE_WITH_KNOTS ( ( 4, 4 ),
 ( 0.000000000000000000, 1.570796326794896558 ),
 .UNSPECIFIED. ) 
 CURVE ( )  GEOMETRIC_REPRESENTATION_ITEM ( )  RATIONAL_B_SPLINE_CURVE ( ( 1.000000000000000000, 0.8047378541243649375, 0.8047378541243649375, 1.000000000000000000 ) ) 
 REPRESENTATION_ITEM ( '' )  );
#47122=EDGE_LOOP ( 'NONE', ( #25835, #48603, #6287, #39911, #35292, #21767 ) ) ;
#47131=DIRECTION ( 'NONE',  ( -1.000000000000000000, 0.000000000000000000, 0.000000000000000000 ) ) ;
#47133=DIRECTION ( 'NONE',  ( -0.000000000000000000, -0.000000000000000000, -1.000000000000000000 ) ) ;
#47135=AXIS2_PLACEMENT_3D ( 'NONE', #16631, #9434, #25100 ) ;
#47141=ORIENTED_EDGE ( 'NONE', *, *, #1188, .T. ) ;
#47142=CARTESIAN_POINT ( 'NONE',  ( -128.4459734468149463, 1.025126265847081886, -80.93171244307201562 ) ) ;
#47144=DIRECTION ( 'NONE',  ( 0.000000000000000000, 0.000000000000000000, 1.000000000000000000 ) ) ;
#47145=EDGE_CURVE ( 'NONE', #29162, #9194, #23720, .T. ) ;
#47147=DIRECTION ( 'NONE',  ( -0.000000000000000000, -0.000000000000000000, -1.000000000000000000 ) ) ;
#47153=ORIENTED_EDGE ( 'NONE', *, *, #27757, .T. ) ;
#47166=CARTESIAN_POINT ( 'NONE',  ( 191.5540265531850537, 1.025126265847089435, 82.56828755692798438 ) ) ;
#47175=ADVANCED_FACE ( 'NONE', ( #37504 ), #32630, .T. ) ;
#47176=CARTESIAN_POINT ( 'NONE',  ( -84.94597344681493212, -1.025126265847089435, -117.4317124430720156 ) ) ;
#47179=EDGE_CURVE ( 'NONE', #7572, #214, #49284, .T. ) ;
#47180=CARTESIAN_POINT ( 'NONE',  ( 153.3040265531850537, 1.750000000000010658, 80.81828755692798438 ) ) ;
#47183=CARTESIAN_POINT ( 'NONE',  ( -86.69597344681494633, 1.750000000000009992, 0.8182875569279768335 ) ) ;
#47187=CARTESIAN_POINT ( 'NONE',  ( -6.695973446814940111, 0.000000000000000000, 165.0000000000000000 ) ) ;
#47200=DIRECTION ( 'NONE',  ( 1.000000000000000000, 0.000000000000000000, 0.000000000000000000 ) ) ;
#47205=ADVANCED_FACE ( 'NONE', ( #5160 ), #44395, .T. ) ;
#47206=CARTESIAN_POINT ( 'NONE',  ( -210.0000000000000568, 2.143131898507884075E-16, -40.93171244307203693 ) ) ;
#47213=ADVANCED_FACE ( 'NONE', ( #5412 ), #1827, .T. ) ;
#47220=CYLINDRICAL_SURFACE ( 'NONE', #5756, 1.750000000000008438 ) ;
#47221=CARTESIAN_POINT ( 'NONE',  ( -206.6959734468149463, -1.750000000000009992, 160.8182875569279702 ) ) ;
#47222=EDGE_CURVE ( 'NONE', #47848, #12229, #9766, .T. ) ;
#47224=FACE_OUTER_BOUND ( 'NONE', #42312, .T. ) ;
#47226=ADVANCED_FACE ( 'NONE', ( #22324 ), #22076, .T. ) ;
#47227=EDGE_CURVE ( 'NONE', #10600, #6064, #3777, .T. ) ;
#47233=CARTESIAN_POINT ( 'NONE',  ( 33.30402655318503946, -1.750000000000010214, 40.81828755692798438 ) ) ;
#47235=CARTESIAN_POINT ( 'NONE',  ( 75.05402655318509630, 2.143131898507880377E-16, 165.0000000000000000 ) ) ;
#47236=EDGE_CURVE ( 'NONE', #1434, #49119, #42575, .T. ) ;
#47243=CYLINDRICAL_SURFACE ( 'NONE', #5955, 1.750000000000001554 ) ;
#47251=VERTEX_POINT ( 'NONE', #41827 ) ;
#47256=FACE_OUTER_BOUND ( 'NONE', #37591, .T. ) ;
#47260=ORIENTED_EDGE ( 'NONE', *, *, #37313, .F. ) ;
#47266=CARTESIAN_POINT ( 'NONE',  ( -86.69597344681494633, -1.750000000000009992, -159.1817124430720298 ) ) ;
#47275=( BOUNDED_CURVE ( )  B_SPLINE_CURVE ( 3, ( #33867, #22298, #18441, #49455 ),
 .UNSPECIFIED., .F., .F. ) 
 B_SPLINE_CURVE_WITH_KNOTS ( ( 4, 4 ),
 ( 1.570796326794896558, 3.141592653589793116 ),
 .UNSPECIFIED. ) 
 CURVE ( )  GEOMETRIC_REPRESENTATION_ITEM ( )  RATIONAL_B_SPLINE_CURVE ( ( 1.000000000000000000, 0.8047378541243649375, 0.8047378541243649375, 1.000000000000000000 ) ) 
 REPRESENTATION_ITEM ( '' )  );
#47276=CARTESIAN_POINT ( 'NONE',  ( 152.2789002873379900, -1.750000000000009548, 159.7931612910809065 ) ) ;
#47279=EDGE_CURVE ( 'NONE', #50433, #32098, #49980, .T. ) ;
#47281=ADVANCED_FACE ( 'NONE', ( #45396 ), #38263, .T. ) ;
#47287=EDGE_CURVE ( 'NONE', #12365, #8857, #9032, .T. ) ;
#47288=EDGE_CURVE ( 'NONE', #45663, #19177, #47946, .T. ) ;
#47295=LINE ( 'NONE', #35552, #22600 ) ;
#47298=VERTEX_POINT ( 'NONE', #26425 ) ;
#47304=DIRECTION ( 'NONE',  ( -1.000000000000000000, 0.000000000000000000, 0.000000000000000000 ) ) ;
#47306=ORIENTED_EDGE ( 'NONE', *, *, #39974, .T. ) ;
#47309=EDGE_LOOP ( 'NONE', ( #5226, #20984, #33415, #41261, #37823, #2947 ) ) ;
#47312=ORIENTED_EDGE ( 'NONE', *, *, #16654, .F. ) ;
#47316=AXIS2_PLACEMENT_3D ( 'NONE', #6017, #33493, #10627 ) ;
#47321=CARTESIAN_POINT ( 'NONE',  ( 31.55402655318503236, 0.000000000000000000, -0.9317124430720247208 ) ) ;
#47327=DIRECTION ( 'NONE',  ( -0.000000000000000000, -0.000000000000000000, -1.000000000000000000 ) ) ;
#47328=EDGE_LOOP ( 'NONE', ( #10618, #10585, #25996, #560, #36061, #30583 ) ) ;
#47330=CARTESIAN_POINT ( 'NONE',  ( -8.445973446814976526, 0.000000000000000000, 42.56828755692802702 ) ) ;
#47334=CARTESIAN_POINT ( 'NONE',  ( 195.0540265531851105, -1.025126265847089213, -0.9317124430720324924 ) ) ;
#47336=CARTESIAN_POINT ( 'NONE',  ( 195.0540265531851105, 1.025126265847089213, -160.9317124430720014 ) ) ;
#47345=ORIENTED_EDGE ( 'NONE', *, *, #30059, .F. ) ;
#47348=ORIENTED_EDGE ( 'NONE', *, *, #18325, .T. ) ;
#47349=ORIENTED_EDGE ( 'NONE', *, *, #4981, .T. ) ;
#47352=ORIENTED_EDGE ( 'NONE', *, *, #21188, .F. ) ;
#47359=CARTESIAN_POINT ( 'NONE',  ( -85.67084718096784002, -1.750000000000010436, -120.2068387089191219 ) ) ;
#47361=VERTEX_POINT ( 'NONE', #25943 ) ;
#47363=CARTESIAN_POINT ( 'NONE',  ( -4.945973446814903696, 2.143131898507912917E-16, -0.9317124430720524764 ) ) ;
#47364=DIRECTION ( 'NONE',  ( -1.000000000000000000, 0.000000000000000000, 0.000000000000000000 ) ) ;
#47365=ORIENTED_EDGE ( 'NONE', *, *, #9293, .F. ) ;
#47368=CARTESIAN_POINT ( 'NONE',  ( -7.721099712662037540, -1.750000000000023315, 159.7931612910808781 ) ) ;
#47370=ORIENTED_EDGE ( 'NONE', *, *, #28748, .F. ) ;
#47384=CARTESIAN_POINT ( 'NONE',  ( -206.6959734468149463, -1.750000000000010214, 40.81828755692798438 ) ) ;
#47386=VERTEX_POINT ( 'NONE', #41578 ) ;
#47389=PLANE ( 'NONE',  #42202 ) ;
#47392=( BOUNDED_CURVE ( )  B_SPLINE_CURVE ( 3, ( #24681, #4416, #6108, #8272 ),
 .UNSPECIFIED., .F., .F. ) 
 B_SPLINE_CURVE_WITH_KNOTS ( ( 4, 4 ),
 ( 3.141592653589793116, 4.712388980384689674 ),
 .UNSPECIFIED. ) 
 CURVE ( )  GEOMETRIC_REPRESENTATION_ITEM ( )  RATIONAL_B_SPLINE_CURVE ( ( 1.000000000000000000, 0.8047378541243649375, 0.8047378541243649375, 1.000000000000000000 ) ) 
 REPRESENTATION_ITEM ( '' )  );
#47393=ORIENTED_EDGE ( 'NONE', *, *, #4272, .F. ) ;
#47399=VERTEX_POINT ( 'NONE', #12544 ) ;
#47401=CARTESIAN_POINT ( 'NONE',  ( 210.0000000000000568, 0.000000000000000000, 120.8182875569279702 ) ) ;
#47405=( BOUNDED_CURVE ( )  B_SPLINE_CURVE ( 3, ( #3631, #11336, #31094, #42872 ),
 .UNSPECIFIED., .F., .F. ) 
 B_SPLINE_CURVE_WITH_KNOTS ( ( 4, 4 ),
 ( 4.712388980384689674, 6.283185307179586232 ),
 .UNSPECIFIED. ) 
 CURVE ( )  GEOMETRIC_REPRESENTATION_ITEM ( )  RATIONAL_B_SPLINE_CURVE ( ( 1.000000000000000000, 0.8047378541243649375, 0.8047378541243649375, 1.000000000000000000 ) ) 
 REPRESENTATION_ITEM ( '' )  );
#47410=EDGE_CURVE ( 'NONE', #21250, #26375, #19481, .T. ) ;
#47411=EDGE_CURVE ( 'NONE', #41652, #23545, #24369, .T. ) ;
#47414=CARTESIAN_POINT ( 'NONE',  ( 73.30402655318508209, 1.750000000000010658, 80.81828755692798438 ) ) ;
#47416=VERTEX_POINT ( 'NONE', #4102 ) ;
#47417=CARTESIAN_POINT ( 'NONE',  ( -127.7210997126620242, 1.749999999999996669, -160.2068387089191219 ) ) ;
#47418=CARTESIAN_POINT ( 'NONE',  ( 114.3291528190321173, 1.749999999999996891, -78.15658617722492352 ) ) ;
#47420=DIRECTION ( 'NONE',  ( 1.000000000000000000, 0.000000000000000000, 0.000000000000000000 ) ) ;
#47422=( BOUNDED_CURVE ( )  B_SPLINE_CURVE ( 3, ( #9925, #25583, #41223, #37410 ),
 .UNSPECIFIED., .F., .F. ) 
 B_SPLINE_CURVE_WITH_KNOTS ( ( 4, 4 ),
 ( 1.570796326794896558, 3.141592653589793116 ),
 .UNSPECIFIED. ) 
 CURVE ( )  GEOMETRIC_REPRESENTATION_ITEM ( )  RATIONAL_B_SPLINE_CURVE ( ( 1.000000000000000000, 0.8047378541243649375, 0.8047378541243649375, 1.000000000000000000 ) ) 
 REPRESENTATION_ITEM ( '' )  );
#47423=CARTESIAN_POINT ( 'NONE',  ( -168.4459734468149463, 0.000000000000000000, 159.0682875569279702 ) ) ;
#47427=VERTEX_POINT ( 'NONE', #519 ) ;
#47428=DIRECTION ( 'NONE',  ( -1.000000000000000000, -0.000000000000000000, -0.000000000000000000 ) ) ;
#47429=CARTESIAN_POINT ( 'NONE',  ( -204.9459734468149463, 2.143131898507880377E-16, 122.5682875569279702 ) ) ;
#47430=ORIENTED_EDGE ( 'NONE', *, *, #27156, .F. ) ;
#47432=EDGE_CURVE ( 'NONE', #38061, #11639, #19500, .T. ) ;
#47433=VERTEX_POINT ( 'NONE', #4358 ) ;
#47434=EDGE_CURVE ( 'NONE', #40403, #32098, #5722, .T. ) ;
#47441=ADVANCED_FACE ( 'NONE', ( #35169 ), #47654, .T. ) ;
#47442=AXIS2_PLACEMENT_3D ( 'NONE', #33204, #29583, #2620 ) ;
#47451=ORIENTED_EDGE ( 'NONE', *, *, #25511, .T. ) ;
#47453=CARTESIAN_POINT ( 'NONE',  ( 210.0000000000000568, 2.143131898507880377E-16, -160.9317124430720298 ) ) ;
#47456=CARTESIAN_POINT ( 'NONE',  ( -84.94597344681493212, 1.025126265847089879, -117.4317124430720156 ) ) ;
#47457=VERTEX_POINT ( 'NONE', #8211 ) ;
#47462=CARTESIAN_POINT ( 'NONE',  ( 210.0000000000000568, 0.000000000000000000, -119.1817124430720440 ) ) ;
#47466=ORIENTED_EDGE ( 'NONE', *, *, #45870, .F. ) ;
#47468=CARTESIAN_POINT ( 'NONE',  ( -46.69597344681494633, 0.000000000000000000, 165.0000000000000000 ) ) ;
#47470=DIRECTION ( 'NONE',  ( -1.000000000000000000, 0.000000000000000000, 0.000000000000000000 ) ) ;
#47482=VERTEX_POINT ( 'NONE', #40515 ) ;
#47484=CARTESIAN_POINT ( 'NONE',  ( 210.0000000000000568, 0.000000000000000000, -117.4317124430720298 ) ) ;
#47489=VERTEX_POINT ( 'NONE', #5858 ) ;
#47498=ORIENTED_EDGE ( 'NONE', *, *, #33201, .T. ) ;
#47505=VERTEX_POINT ( 'NONE', #28955 ) ;
#47514=DIRECTION ( 'NONE',  ( -0.000000000000000000, -0.000000000000000000, -1.000000000000000000 ) ) ;
#47525=LINE ( 'NONE', #17015, #17643 ) ;
#47526=FACE_OUTER_BOUND ( 'NONE', #30648, .T. ) ;
#47528=ORIENTED_EDGE ( 'NONE', *, *, #46279, .T. ) ;
#47529=ORIENTED_EDGE ( 'NONE', *, *, #40359, .T. ) ;
#47534=EDGE_CURVE ( 'NONE', #9513, #4058, #25070, .T. ) ;
#47538=CARTESIAN_POINT ( 'NONE',  ( 194.3291528190321742, -1.750000000000009548, -160.2068387089191219 ) ) ;
#47539=ORIENTED_EDGE ( 'NONE', *, *, #46653, .F. ) ;
#47545=CARTESIAN_POINT ( 'NONE',  ( 155.0540265531850537, 1.025126265847089879, 82.56828755692798438 ) ) ;
#47546=CARTESIAN_POINT ( 'NONE',  ( 154.3291528190321458, 1.750000000000010214, 79.79316129108087807 ) ) ;
#47548=ORIENTED_EDGE ( 'NONE', *, *, #40051, .T. ) ;
#47551=CARTESIAN_POINT ( 'NONE',  ( -124.9459734468149463, 2.143131898507847836E-16, -157.4317124430720582 ) ) ;
#47552=CARTESIAN_POINT ( 'NONE',  ( 151.5540265531850537, 1.025126265847089657, 79.06828755692797017 ) ) ;
#47555=ORIENTED_EDGE ( 'NONE', *, *, #5552, .T. ) ;
#47562=EDGE_CURVE ( 'NONE', #24104, #47298, #7684, .T. ) ;
#47564=VERTEX_POINT ( 'NONE', #48158 ) ;
#47568=( BOUNDED_CURVE ( )  B_SPLINE_CURVE ( 3, ( #49557, #25011, #2166, #10367 ),
 .UNSPECIFIED., .F., .F. ) 
 B_SPLINE_CURVE_WITH_KNOTS ( ( 4, 4 ),
 ( 3.141592653589793116, 4.712388980384689674 ),
 .UNSPECIFIED. ) 
 CURVE ( )  GEOMETRIC_REPRESENTATION_ITEM ( )  RATIONAL_B_SPLINE_CURVE ( ( 1.000000000000000000, 0.8047378541243649375, 0.8047378541243649375, 1.000000000000000000 ) ) 
 REPRESENTATION_ITEM ( '' )  );
#47569=CARTESIAN_POINT ( 'NONE',  ( 112.2789002873379758, 1.749999999999996891, -40.20683870891911482 ) ) ;
#47574=ADVANCED_FACE ( 'NONE', ( #9453 ), #5597, .T. ) ;
#47575=CARTESIAN_POINT ( 'NONE',  ( 33.30402655318503946, -1.750000000000010658, 80.81828755692798438 ) ) ;
#47576=CARTESIAN_POINT ( 'NONE',  ( 210.0000000000000568, 0.000000000000000000, 2.568287556927987048 ) ) ;
#47579=DIRECTION ( 'NONE',  ( -1.000000000000000000, -0.000000000000000000, -0.000000000000000000 ) ) ;
#47582=LINE ( 'NONE', #11974, #27384 ) ;
#47585=CARTESIAN_POINT ( 'NONE',  ( 193.3040265531851105, 1.750000000000010658, -119.1817124430720440 ) ) ;
#47586=EDGE_CURVE ( 'NONE', #4462, #38061, #9332, .T. ) ;
#47591=VECTOR ( 'NONE', #942, 1000.000000000000000 ) ;
#47592=DIRECTION ( 'NONE',  ( 1.000000000000000000, 0.000000000000000000, 0.000000000000000000 ) ) ;
#47593=CARTESIAN_POINT ( 'NONE',  ( -45.67084718096785423, -1.750000000000010436, 79.79316129108087807 ) ) ;
#47597=EDGE_LOOP ( 'NONE', ( #26511, #48682, #20967, #161, #29617, #35817 ) ) ;
#47598=CARTESIAN_POINT ( 'NONE',  ( -6.695973446814940111, -1.750000000000024203, -119.1817124430720440 ) ) ;
#47600=CARTESIAN_POINT ( 'NONE',  ( 33.30402655318503946, -1.750000000000010658, -79.18171244307201562 ) ) ;
#47602=CYLINDRICAL_SURFACE ( 'NONE', #27369, 1.750000000000008438 ) ;
#47603=ORIENTED_EDGE ( 'NONE', *, *, #2916, .F. ) ;
#47604=VERTEX_POINT ( 'NONE', #6110 ) ;
#47606=EDGE_CURVE ( 'NONE', #4486, #40841, #32268, .T. ) ;
#47607=CARTESIAN_POINT ( 'NONE',  ( -167.7210997126620384, -1.750000000000010214, -80.20683870891910772 ) ) ;
#47614=CARTESIAN_POINT ( 'NONE',  ( -204.9459734468148895, 1.025126265847089657, 119.0682875569279560 ) ) ;
#47615=DIRECTION ( 'NONE',  ( -1.000000000000000000, 0.000000000000000000, 0.000000000000000000 ) ) ;
#47617=ORIENTED_EDGE ( 'NONE', *, *, #26257, .T. ) ;
#47618=DIRECTION ( 'NONE',  ( -1.000000000000000000, -0.000000000000000000, -0.000000000000000000 ) ) ;
#47623=ORIENTED_EDGE ( 'NONE', *, *, #27370, .F. ) ;
#47625=CARTESIAN_POINT ( 'NONE',  ( 73.30402655318508209, -1.750000000000010658, -119.1817124430720440 ) ) ;
#47628=CARTESIAN_POINT ( 'NONE',  ( -46.69597344681494633, -1.750000000000010658, 120.8182875569279702 ) ) ;
#47631=CARTESIAN_POINT ( 'NONE',  ( -48.44597344681496054, -1.025126265847089213, 159.0682875569279418 ) ) ;
#47633=CARTESIAN_POINT ( 'NONE',  ( -166.6959734468149463, -1.750000000000009992, -159.1817124430720298 ) ) ;
#47635=ADVANCED_FACE ( 'NONE', ( #41761 ), #18153, .T. ) ;
#47637=FACE_OUTER_BOUND ( 'NONE', #45280, .T. ) ;
#47639=CARTESIAN_POINT ( 'NONE',  ( -6.695973446814940111, 0.000000000000000000, 165.0000000000000000 ) ) ;
#47640=( BOUNDED_CURVE ( )  B_SPLINE_CURVE ( 3, ( #4618, #20263, #32072, #27461 ),
 .UNSPECIFIED., .F., .F. ) 
 B_SPLINE_CURVE_WITH_KNOTS ( ( 4, 4 ),
 ( 1.570796326794896558, 3.141592653589793116 ),
 .UNSPECIFIED. ) 
 CURVE ( )  GEOMETRIC_REPRESENTATION_ITEM ( )  RATIONAL_B_SPLINE_CURVE ( ( 1.000000000000000000, 0.8047378541243649375, 0.8047378541243649375, 1.000000000000000000 ) ) 
 REPRESENTATION_ITEM ( '' )  );
#47644=DIRECTION ( 'NONE',  ( 0.000000000000000000, 0.000000000000000000, 1.000000000000000000 ) ) ;
#47646=LINE ( 'NONE', #5344, #32408 ) ;
#47652=ORIENTED_EDGE ( 'NONE', *, *, #35010, .F. ) ;
#47654=CYLINDRICAL_SURFACE ( 'NONE', #1909, 1.750000000000010214 ) ;
#47656=ORIENTED_EDGE ( 'NONE', *, *, #6542, .F. ) ;
#47657=DIRECTION ( 'NONE',  ( -0.000000000000000000, -0.000000000000000000, -1.000000000000000000 ) ) ;
#47659=VERTEX_POINT ( 'NONE', #33831 ) ;
#47660=EDGE_CURVE ( 'NONE', #28177, #19656, #15075, .T. ) ;
#47664=ORIENTED_EDGE ( 'NONE', *, *, #5838, .T. ) ;
#47666=CYLINDRICAL_SURFACE ( 'NONE', #10317, 1.750000000000001554 ) ;
#47668=AXIS2_PLACEMENT_3D ( 'NONE', #39860, #24198, #1350 ) ;
#47674=CYLINDRICAL_SURFACE ( 'NONE', #8955, 1.750000000000015543 ) ;
#47677=CARTESIAN_POINT ( 'NONE',  ( -5.670847180967843570, 1.750000000000023537, 79.79316129108087807 ) ) ;
#47685=CARTESIAN_POINT ( 'NONE',  ( 75.05402655318509630, -1.025126265847089435, -77.43171244307200141 ) ) ;
#47686=CIRCLE ( 'NONE', #15796, 1.750000000000001554 ) ;
#47696=CARTESIAN_POINT ( 'NONE',  ( -7.721099712662037540, 1.750000000000023315, -38.15658617722493062 ) ) ;
#47697=( BOUNDED_CURVE ( )  B_SPLINE_CURVE ( 3, ( #43326, #31811, #23333, #748 ),
 .UNSPECIFIED., .F., .F. ) 
 B_SPLINE_CURVE_WITH_KNOTS ( ( 4, 4 ),
 ( 0.000000000000000000, 1.570796326794896558 ),
 .UNSPECIFIED. ) 
 CURVE ( )  GEOMETRIC_REPRESENTATION_ITEM ( )  RATIONAL_B_SPLINE_CURVE ( ( 1.000000000000000000, 0.8047378541243649375, 0.8047378541243649375, 1.000000000000000000 ) ) 
 REPRESENTATION_ITEM ( '' )  );
#47701=DIRECTION ( 'NONE',  ( 0.000000000000000000, 0.000000000000000000, -1.000000000000000000 ) ) ;
#47703=CARTESIAN_POINT ( 'NONE',  ( 71.55402655318505367, 0.000000000000000000, -80.93171244307204404 ) ) ;
#47705=( BOUNDED_CURVE ( )  B_SPLINE_CURVE ( 3, ( #24687, #44895, #40332, #36757 ),
 .UNSPECIFIED., .F., .F. ) 
 B_SPLINE_CURVE_WITH_KNOTS ( ( 4, 4 ),
 ( 0.000000000000000000, 1.570796326794896558 ),
 .UNSPECIFIED. ) 
 CURVE ( )  GEOMETRIC_REPRESENTATION_ITEM ( )  RATIONAL_B_SPLINE_CURVE ( ( 1.000000000000000000, 0.8047378541243649375, 0.8047378541243649375, 1.000000000000000000 ) ) 
 REPRESENTATION_ITEM ( '' )  );
#47708=CARTESIAN_POINT ( 'NONE',  ( 210.0000000000000568, 0.000000000000000000, 0.8182875569279768335 ) ) ;
#47709=CARTESIAN_POINT ( 'NONE',  ( 154.3291528190321458, -1.750000000000010436, -80.20683870891910772 ) ) ;
#47710=EDGE_CURVE ( 'NONE', #4446, #46038, #6021, .T. ) ;
#47717=CARTESIAN_POINT ( 'NONE',  ( 73.30402655318508209, 1.750000000000009992, -159.1817124430720298 ) ) ;
#47721=CARTESIAN_POINT ( 'NONE',  ( 210.0000000000000568, 0.000000000000000000, -159.1817124430720298 ) ) ;
#47740=ORIENTED_EDGE ( 'NONE', *, *, #15062, .T. ) ;
#47746=ORIENTED_EDGE ( 'NONE', *, *, #13920, .F. ) ;
#47751=CARTESIAN_POINT ( 'NONE',  ( 210.0000000000000568, 2.143131898507880377E-16, -0.9317124430720331585 ) ) ;
#47752=ADVANCED_FACE ( 'NONE', ( #35366 ), #199, .T. ) ;
#47755=CARTESIAN_POINT ( 'NONE',  ( 192.2789002873380184, 1.750000000000009548, -0.2068387089191121020 ) ) ;
#47760=ORIENTED_EDGE ( 'NONE', *, *, #18145, .F. ) ;
#47762=FACE_OUTER_BOUND ( 'NONE', #30109, .T. ) ;
#47766=DIRECTION ( 'NONE',  ( -1.000000000000000000, -0.000000000000000000, -0.000000000000000000 ) ) ;
#47772=CARTESIAN_POINT ( 'NONE',  ( 151.5540265531850537, -1.025126265847089213, 159.0682875569279418 ) ) ;
#47773=CARTESIAN_POINT ( 'NONE',  ( 113.3040265531850537, 0.000000000000000000, 165.0000000000000000 ) ) ;
#47776=EDGE_LOOP ( 'NONE', ( #35496, #32082, #7379, #45734, #37257, #15945 ) ) ;
#47783=ORIENTED_EDGE ( 'NONE', *, *, #16785, .T. ) ;
#47787=CARTESIAN_POINT ( 'NONE',  ( -6.695973446814940111, 1.750000000000023315, 160.8182875569279702 ) ) ;
#47788=VECTOR ( 'NONE', #33586, 1000.000000000000000 ) ;
#47793=EDGE_CURVE ( 'NONE', #13192, #3794, #27388, .T. ) ;
#47795=EDGE_LOOP ( 'NONE', ( #8922, #9245, #44825, #27724, #14020, #32374 ) ) ;
#47800=ORIENTED_EDGE ( 'NONE', *, *, #778, .T. ) ;
#47803=CARTESIAN_POINT ( 'NONE',  ( 71.55402655318505367, 1.025126265847089435, 82.56828755692798438 ) ) ;
#47805=CARTESIAN_POINT ( 'NONE',  ( 112.2789002873379758, -1.749999999999996891, -120.2068387089191219 ) ) ;
#47806=VERTEX_POINT ( 'NONE', #8146 ) ;
#47809=PLANE ( 'NONE',  #13559 ) ;
#47812=CARTESIAN_POINT ( 'NONE',  ( -128.4459734468149463, -1.025126265847081442, 159.0682875569279418 ) ) ;
#47815=CARTESIAN_POINT ( 'NONE',  ( -6.695973446814940111, -1.750000000000024203, 80.81828755692798438 ) ) ;
#47816=ORIENTED_EDGE ( 'NONE', *, *, #34594, .T. ) ;
#47823=CARTESIAN_POINT ( 'NONE',  ( 153.3040265531850537, 1.750000000000010658, 120.8182875569279702 ) ) ;
#47825=CIRCLE ( 'NONE', #50262, 1.750000000000009992 ) ;
#47827=DIRECTION ( 'NONE',  ( -1.000000000000000000, -0.000000000000000000, -0.000000000000000000 ) ) ;
#47832=LINE ( 'NONE', #33001, #38806 ) ;
#47834=AXIS2_PLACEMENT_3D ( 'NONE', #28546, #36266, #21092 ) ;
#47840=( BOUNDED_CURVE ( )  B_SPLINE_CURVE ( 3, ( #19875, #24758, #28092, #24251 ),
 .UNSPECIFIED., .F., .F. ) 
 B_SPLINE_CURVE_WITH_KNOTS ( ( 4, 4 ),
 ( 4.712388980384689674, 6.283185307179586232 ),
 .UNSPECIFIED. ) 
 CURVE ( )  GEOMETRIC_REPRESENTATION_ITEM ( )  RATIONAL_B_SPLINE_CURVE ( ( 1.000000000000000000, 0.8047378541243649375, 0.8047378541243649375, 1.000000000000000000 ) ) 
 REPRESENTATION_ITEM ( '' )  );
#47843=EDGE_CURVE ( 'NONE', #16057, #29337, #12912, .T. ) ;
#47848=VERTEX_POINT ( 'NONE', #8655 ) ;
#47849=CARTESIAN_POINT ( 'NONE',  ( 33.30402655318503946, 0.000000000000000000, 165.0000000000000000 ) ) ;
#47850=CARTESIAN_POINT ( 'NONE',  ( 74.32915281903215998, 1.750000000000009548, 1.843413822775065825 ) ) ;
#47853=EDGE_LOOP ( 'NONE', ( #2454, #17068, #34080, #19434, #42280, #31913 ) ) ;
#47855=ORIENTED_EDGE ( 'NONE', *, *, #6057, .F. ) ;
#47860=ORIENTED_EDGE ( 'NONE', *, *, #40758, .F. ) ;
#47861=CARTESIAN_POINT ( 'NONE',  ( 31.55402655318503236, 1.025126265847089657, 79.06828755692797017 ) ) ;
#47864=VERTEX_POINT ( 'NONE', #40197 ) ;
#47866=( BOUNDED_CURVE ( )  B_SPLINE_CURVE ( 3, ( #38142, #34535, #50116, #26831 ),
 .UNSPECIFIED., .F., .F. ) 
 B_SPLINE_CURVE_WITH_KNOTS ( ( 4, 4 ),
 ( 3.141592653589793116, 4.712388980384689674 ),
 .UNSPECIFIED. ) 
 CURVE ( )  GEOMETRIC_REPRESENTATION_ITEM ( )  RATIONAL_B_SPLINE_CURVE ( ( 1.000000000000000000, 0.8047378541243649375, 0.8047378541243649375, 1.000000000000000000 ) ) 
 REPRESENTATION_ITEM ( '' )  );
#47868=AXIS2_PLACEMENT_3D ( 'NONE', #8432, #13015, #5323 ) ;
#47871=CARTESIAN_POINT ( 'NONE',  ( 153.3040265531850537, 0.000000000000000000, 165.0000000000000000 ) ) ;
#47878=CYLINDRICAL_SURFACE ( 'NONE', #15586, 1.750000000000015543 ) ;
#47884=AXIS2_PLACEMENT_3D ( 'NONE', #28899, #36884, #37629 ) ;
#47885=CARTESIAN_POINT ( 'NONE',  ( 112.2789002873379758, 1.749999999999996669, -38.15658617722495194 ) ) ;
#47887=CARTESIAN_POINT ( 'NONE',  ( -88.44597344681494633, -1.025126265847089657, 79.06828755692797017 ) ) ;
#47888=CARTESIAN_POINT ( 'NONE',  ( 195.0540265531851105, 1.025126265847089435, 2.568287556927986159 ) ) ;
#47898=CARTESIAN_POINT ( 'NONE',  ( 35.05402655318504657, 2.143131898507880377E-16, 122.5682875569279702 ) ) ;
#47899=DIRECTION ( 'NONE',  ( -0.000000000000000000, -0.000000000000000000, -1.000000000000000000 ) ) ;
#47902=ORIENTED_EDGE ( 'NONE', *, *, #12727, .F. ) ;
#47904=EDGE_CURVE ( 'NONE', #42641, #26504, #2140, .T. ) ;
#47905=ADVANCED_FACE ( 'NONE', ( #32253 ), #17095, .T. ) ;
#47906=CARTESIAN_POINT ( 'NONE',  ( -48.44597344681496054, 1.025126265847089213, -160.9317124430720014 ) ) ;
#47908=CARTESIAN_POINT ( 'NONE',  ( -44.94597344681493922, -1.025126265847089435, -117.4317124430720156 ) ) ;
#47913=EDGE_LOOP ( 'NONE', ( #5164, #30642, #29214, #15275, #25264, #10099 ) ) ;
#47915=EDGE_CURVE ( 'NONE', #14561, #49775, #28363, .T. ) ;
#47920=LINE ( 'NONE', #20005, #33922 ) ;
#47921=AXIS2_PLACEMENT_3D ( 'NONE', #36388, #28664, #47615 ) ;
#47922=ORIENTED_EDGE ( 'NONE', *, *, #49464, .T. ) ;
#47924=DIRECTION ( 'NONE',  ( -1.000000000000000000, 0.000000000000000000, 0.000000000000000000 ) ) ;
#47926=DIRECTION ( 'NONE',  ( -0.000000000000000000, -0.000000000000000000, -1.000000000000000000 ) ) ;
#47930=CYLINDRICAL_SURFACE ( 'NONE', #26450, 1.750000000000015543 ) ;
#47931=AXIS2_PLACEMENT_3D ( 'NONE', #37549, #17270, #45439 ) ;
#47933=CARTESIAN_POINT ( 'NONE',  ( 210.0000000000000568, 0.000000000000000000, 0.8182875569279768335 ) ) ;
#47935=AXIS2_PLACEMENT_3D ( 'NONE', #2539, #33861, #49448 ) ;
#47937=CARTESIAN_POINT ( 'NONE',  ( -6.695973446814940111, 1.750000000000024203, 80.81828755692798438 ) ) ;
#47943=CARTESIAN_POINT ( 'NONE',  ( -45.67084718096785423, -1.750000000000010436, -80.20683870891910772 ) ) ;
#47944=CARTESIAN_POINT ( 'NONE',  ( 194.3291528190321742, 1.750000000000009548, 159.7931612910809065 ) ) ;
#47946=( BOUNDED_CURVE ( )  B_SPLINE_CURVE ( 3, ( #30287, #29781, #37748, #15134 ),
 .UNSPECIFIED., .F., .F. ) 
 B_SPLINE_CURVE_WITH_KNOTS ( ( 4, 4 ),
 ( 1.570796326794896558, 3.141592653589793116 ),
 .UNSPECIFIED. ) 
 CURVE ( )  GEOMETRIC_REPRESENTATION_ITEM ( )  RATIONAL_B_SPLINE_CURVE ( ( 1.000000000000000000, 0.8047378541243649375, 0.8047378541243649375, 1.000000000000000000 ) ) 
 REPRESENTATION_ITEM ( '' )  );
#47947=DIRECTION ( 'NONE',  ( -0.000000000000000000, -0.000000000000000000, -1.000000000000000000 ) ) ;
#47952=EDGE_LOOP ( 'NONE', ( #29909, #34053 ) ) ;
#47954=CARTESIAN_POINT ( 'NONE',  ( 115.0540265531850395, 2.143131898507847836E-16, -77.43171244307204404 ) ) ;
#47955=VECTOR ( 'NONE', #14122, 1000.000000000000000 ) ;
#47958=VECTOR ( 'NONE', #19637, 1000.000000000000000 ) ;
#47962=AXIS2_PLACEMENT_3D ( 'NONE', #23967, #39627, #23468 ) ;
#47963=CYLINDRICAL_SURFACE ( 'NONE', #32373, 1.750000000000010214 ) ;
#47964=CARTESIAN_POINT ( 'NONE',  ( -48.44597344681495343, 0.000000000000000000, 79.06828755692797017 ) ) ;
#47965=AXIS2_PLACEMENT_3D ( 'NONE', #35126, #12010, #34599 ) ;
#47966=ORIENTED_EDGE ( 'NONE', *, *, #47236, .F. ) ;
#47967=DIRECTION ( 'NONE',  ( -1.000000000000000000, 0.000000000000000000, 0.000000000000000000 ) ) ;
#47974=CARTESIAN_POINT ( 'NONE',  ( -204.9459734468148895, -1.025126265847089213, -37.43171244307202272 ) ) ;
#47979=DIRECTION ( 'NONE',  ( -1.000000000000000000, -0.000000000000000000, -0.000000000000000000 ) ) ;
#47984=ORIENTED_EDGE ( 'NONE', *, *, #24747, .F. ) ;
#47986=LINE ( 'NONE', #24193, #39069 ) ;
#47988=AXIS2_PLACEMENT_3D ( 'NONE', #49243, #37025, #33165 ) ;
#47990=CARTESIAN_POINT ( 'NONE',  ( 155.0540265531850537, 2.143131898507880377E-16, 82.56828755692798438 ) ) ;
#47995=FACE_OUTER_BOUND ( 'NONE', #36802, .T. ) ;
#48004=CIRCLE ( 'NONE', #1365, 1.750000000000015543 ) ;
#48006=DIRECTION ( 'NONE',  ( -1.000000000000000000, -0.000000000000000000, -0.000000000000000000 ) ) ;
#48008=( BOUNDED_CURVE ( )  B_SPLINE_CURVE ( 3, ( #10642, #26553, #17148, #41949 ),
 .UNSPECIFIED., .F., .F. ) 
 B_SPLINE_CURVE_WITH_KNOTS ( ( 4, 4 ),
 ( 4.712388980384689674, 6.283185307179586232 ),
 .UNSPECIFIED. ) 
 CURVE ( )  GEOMETRIC_REPRESENTATION_ITEM ( )  RATIONAL_B_SPLINE_CURVE ( ( 1.000000000000000000, 0.8047378541243649375, 0.8047378541243649375, 1.000000000000000000 ) ) 
 REPRESENTATION_ITEM ( '' )  );
#48011=ORIENTED_EDGE ( 'NONE', *, *, #22650, .F. ) ;
#48013=CARTESIAN_POINT ( 'NONE',  ( -167.7210997126620384, 1.750000000000009548, -40.20683870891912193 ) ) ;
#48017=CARTESIAN_POINT ( 'NONE',  ( -44.94597344681493922, 1.025126265847089879, -117.4317124430720156 ) ) ;
#48022=DIRECTION ( 'NONE',  ( -1.000000000000000000, 0.000000000000000000, 0.000000000000000000 ) ) ;
#48023=CARTESIAN_POINT ( 'NONE',  ( 151.5540265531850537, 0.000000000000000000, 159.0682875569279702 ) ) ;
#48027=ORIENTED_EDGE ( 'NONE', *, *, #42734, .T. ) ;
#48037=CARTESIAN_POINT ( 'NONE',  ( -167.7210997126620384, 1.750000000000009548, -160.2068387089191219 ) ) ;
#48038=DIRECTION ( 'NONE',  ( -1.000000000000000000, -0.000000000000000000, -0.000000000000000000 ) ) ;
#48039=EDGE_CURVE ( 'NONE', #214, #27650, #4387, .T. ) ;
#48041=ORIENTED_EDGE ( 'NONE', *, *, #25203, .T. ) ;
#48043=VECTOR ( 'NONE', #24325, 1000.000000000000000 ) ;
#48044=CARTESIAN_POINT ( 'NONE',  ( 153.3040265531850537, 1.750000000000010658, 80.81828755692798438 ) ) ;
#48048=CARTESIAN_POINT ( 'NONE',  ( -46.69597344681494633, 1.750000000000010214, -39.18171244307202983 ) ) ;
#48050=CARTESIAN_POINT ( 'NONE',  ( 191.5540265531850537, -1.025126265847089879, -77.43171244307200141 ) ) ;
#48051=DIRECTION ( 'NONE',  ( -1.000000000000000000, -0.000000000000000000, -0.000000000000000000 ) ) ;
#48058=ORIENTED_EDGE ( 'NONE', *, *, #42272, .F. ) ;
#48059=ORIENTED_EDGE ( 'NONE', *, *, #38410, .F. ) ;
#48061=DIRECTION ( 'NONE',  ( -0.000000000000000000, -0.000000000000000000, -1.000000000000000000 ) ) ;
#48065=ORIENTED_EDGE ( 'NONE', *, *, #33211, .T. ) ;
#48071=CARTESIAN_POINT ( 'NONE',  ( 151.5540265531850537, 0.000000000000000000, 122.5682875569279702 ) ) ;
#48072=DIRECTION ( 'NONE',  ( 1.000000000000000000, 0.000000000000000000, 0.000000000000000000 ) ) ;
#48073=EDGE_CURVE ( 'NONE', #9715, #45355, #14256, .T. ) ;
#48079=DIRECTION ( 'NONE',  ( -0.000000000000000000, -0.000000000000000000, -1.000000000000000000 ) ) ;
#48084=CARTESIAN_POINT ( 'NONE',  ( 210.0000000000000568, 0.000000000000000000, 160.8182875569279702 ) ) ;
#48085=CARTESIAN_POINT ( 'NONE',  ( -6.695973446814940111, -1.750000000000024203, -119.1817124430720440 ) ) ;
#48090=CARTESIAN_POINT ( 'NONE',  ( 113.3040265531850537, 1.749999999999997335, 120.8182875569279702 ) ) ;
#48091=EDGE_CURVE ( 'NONE', #13146, #36974, #35996, .T. ) ;
#48092=AXIS2_PLACEMENT_3D ( 'NONE', #28377, #8866, #24524 ) ;
#48100=CARTESIAN_POINT ( 'NONE',  ( -84.94597344681494633, 2.143131898507880377E-16, -160.9317124430720014 ) ) ;
#48103=VERTEX_POINT ( 'NONE', #16227 ) ;
#48105=ADVANCED_FACE ( 'NONE', ( #27531 ), #16723, .T. ) ;
#48106=DIRECTION ( 'NONE',  ( -1.000000000000000000, -0.000000000000000000, -0.000000000000000000 ) ) ;
#48109=CARTESIAN_POINT ( 'NONE',  ( 33.30402655318503946, 1.750000000000009992, 0.8182875569279768335 ) ) ;
#48110=VERTEX_POINT ( 'NONE', #47484 ) ;
#48112=CARTESIAN_POINT ( 'NONE',  ( 71.55402655318505367, 0.000000000000000000, 79.06828755692797017 ) ) ;
#48115=CARTESIAN_POINT ( 'NONE',  ( 155.0540265531850537, 0.000000000000000000, 162.5682875569279702 ) ) ;
#48120=VERTEX_POINT ( 'NONE', #20069 ) ;
#48123=ORIENTED_EDGE ( 'NONE', *, *, #35978, .F. ) ;
#48127=FACE_OUTER_BOUND ( 'NONE', #30620, .T. ) ;
#48129=EDGE_CURVE ( 'NONE', #33010, #42224, #33613, .T. ) ;
#48134=CARTESIAN_POINT ( 'NONE',  ( 193.3040265531851105, 1.750000000000009992, 0.8182875569279768335 ) ) ;
#48136=EDGE_CURVE ( 'NONE', #34969, #21408, #14554, .T. ) ;
#48137=DIRECTION ( 'NONE',  ( -1.000000000000000000, -0.000000000000000000, -0.000000000000000000 ) ) ;
#48142=( BOUNDED_CURVE ( )  B_SPLINE_CURVE ( 3, ( #49109, #13998, #45279, #10159 ),
 .UNSPECIFIED., .F., .F. ) 
 B_SPLINE_CURVE_WITH_KNOTS ( ( 4, 4 ),
 ( 0.000000000000000000, 1.570796326794896558 ),
 .UNSPECIFIED. ) 
 CURVE ( )  GEOMETRIC_REPRESENTATION_ITEM ( )  RATIONAL_B_SPLINE_CURVE ( ( 1.000000000000000000, 0.8047378541243649375, 0.8047378541243649375, 1.000000000000000000 ) ) 
 REPRESENTATION_ITEM ( '' )  );
#48145=ORIENTED_EDGE ( 'NONE', *, *, #41771, .F. ) ;
#48147=( BOUNDED_CURVE ( )  B_SPLINE_CURVE ( 3, ( #44059, #5572, #5063, #20723 ),
 .UNSPECIFIED., .F., .F. ) 
 B_SPLINE_CURVE_WITH_KNOTS ( ( 4, 4 ),
 ( 1.570796326794896558, 3.141592653589793116 ),
 .UNSPECIFIED. ) 
 CURVE ( )  GEOMETRIC_REPRESENTATION_ITEM ( )  RATIONAL_B_SPLINE_CURVE ( ( 1.000000000000000000, 0.8047378541243649375, 0.8047378541243649375, 1.000000000000000000 ) ) 
 REPRESENTATION_ITEM ( '' )  );
#48148=ADVANCED_FACE ( 'NONE', ( #4681 ), #20321, .T. ) ;
#48149=DIRECTION ( 'NONE',  ( 0.000000000000000000, 0.000000000000000000, -1.000000000000000000 ) ) ;
#48152=VERTEX_POINT ( 'NONE', #23919 ) ;
#48154=EDGE_CURVE ( 'NONE', #5511, #29610, #16529, .T. ) ;
#48158=CARTESIAN_POINT ( 'NONE',  ( 31.55402655318506788, 0.000000000000000000, 162.5682875569279702 ) ) ;
#48159=CARTESIAN_POINT ( 'NONE',  ( -44.94597344681493922, 1.025126265847089213, -0.9317124430720324924 ) ) ;
#48160=( BOUNDED_CURVE ( )  B_SPLINE_CURVE ( 3, ( #42802, #39998, #4584, #19722 ),
 .UNSPECIFIED., .F., .F. ) 
 B_SPLINE_CURVE_WITH_KNOTS ( ( 4, 4 ),
 ( 4.712388980384689674, 6.283185307179586232 ),
 .UNSPECIFIED. ) 
 CURVE ( )  GEOMETRIC_REPRESENTATION_ITEM ( )  RATIONAL_B_SPLINE_CURVE ( ( 1.000000000000000000, 0.8047378541243649375, 0.8047378541243649375, 1.000000000000000000 ) ) 
 REPRESENTATION_ITEM ( '' )  );
#48162=CARTESIAN_POINT ( 'NONE',  ( 210.0000000000000568, 0.000000000000000000, 40.81828755692798438 ) ) ;
#48165=AXIS2_PLACEMENT_3D ( 'NONE', #31170, #10894, #3701 ) ;
#48167=CARTESIAN_POINT ( 'NONE',  ( -168.4459734468149747, -1.025126265847089435, 39.06828755692797728 ) ) ;
#48171=CARTESIAN_POINT ( 'NONE',  ( -126.6959734468149321, 0.000000000000000000, 165.0000000000000000 ) ) ;
#48175=ORIENTED_EDGE ( 'NONE', *, *, #1241, .F. ) ;
#48186=LINE ( 'NONE', #5383, #45388 ) ;
#48187=CARTESIAN_POINT ( 'NONE',  ( 210.0000000000000568, 2.143131898507881116E-16, -40.93171244307203693 ) ) ;
#48189=EDGE_CURVE ( 'NONE', #41782, #34169, #35874, .T. ) ;
#48199=VERTEX_POINT ( 'NONE', #40827 ) ;
#48208=DIRECTION ( 'NONE',  ( -1.000000000000000000, -0.000000000000000000, -0.000000000000000000 ) ) ;
#48213=ADVANCED_FACE ( 'NONE', ( #1835 ), #5923, .T. ) ;
#48215=CARTESIAN_POINT ( 'NONE',  ( -84.94597344681493212, 1.025126265847089657, 79.06828755692797017 ) ) ;
#48218=VECTOR ( 'NONE', #14116, 1000.000000000000000 ) ;
#48225=CARTESIAN_POINT ( 'NONE',  ( -204.9459734468148895, 1.025126265847089435, -157.4317124430720582 ) ) ;
#48232=FACE_OUTER_BOUND ( 'NONE', #49535, .T. ) ;
#48234=VERTEX_POINT ( 'NONE', #9281 ) ;
#48235=CARTESIAN_POINT ( 'NONE',  ( 195.0540265531851105, 1.025126265847089435, -157.4317124430720582 ) ) ;
#48236=ADVANCED_FACE ( 'NONE', ( #13627 ), #32637, .T. ) ;
#48239=ORIENTED_EDGE ( 'NONE', *, *, #47001, .F. ) ;
#48241=CARTESIAN_POINT ( 'NONE',  ( -124.9459734468149463, 2.143131898507847836E-16, -80.93171244307201562 ) ) ;
#48243=( BOUNDED_CURVE ( )  B_SPLINE_CURVE ( 3, ( #16888, #20986, #49572, #36406 ),
 .UNSPECIFIED., .F., .F. ) 
 B_SPLINE_CURVE_WITH_KNOTS ( ( 4, 4 ),
 ( 4.712388980384689674, 6.283185307179586232 ),
 .UNSPECIFIED. ) 
 CURVE ( )  GEOMETRIC_REPRESENTATION_ITEM ( )  RATIONAL_B_SPLINE_CURVE ( ( 1.000000000000000000, 0.8047378541243649375, 0.8047378541243649375, 1.000000000000000000 ) ) 
 REPRESENTATION_ITEM ( '' )  );
#48253=ORIENTED_EDGE ( 'NONE', *, *, #31190, .F. ) ;
#48254=ORIENTED_EDGE ( 'NONE', *, *, #39811, .F. ) ;
#48261=CARTESIAN_POINT ( 'NONE',  ( -46.69597344681494633, -1.750000000000010658, 80.81828755692798438 ) ) ;
#48269=CARTESIAN_POINT ( 'NONE',  ( -128.4459734468149463, 1.025126265847081442, -0.9317124430720195027 ) ) ;
#48272=CYLINDRICAL_SURFACE ( 'NONE', #11628, 1.750000000000015543 ) ;
#48278=CARTESIAN_POINT ( 'NONE',  ( -168.4459734468149463, 0.000000000000000000, -0.9317124430720247208 ) ) ;
#48280=DIRECTION ( 'NONE',  ( -0.000000000000000000, -0.000000000000000000, -1.000000000000000000 ) ) ;
#48283=LINE ( 'NONE', #21629, #42592 ) ;
#48291=FACE_OUTER_BOUND ( 'NONE', #43428, .T. ) ;
#48292=ORIENTED_EDGE ( 'NONE', *, *, #47660, .F. ) ;
#48293=ORIENTED_EDGE ( 'NONE', *, *, #34192, .F. ) ;
#48295=CARTESIAN_POINT ( 'NONE',  ( -48.44597344681495343, 0.000000000000000000, -157.4317124430720014 ) ) ;
#48297=( BOUNDED_CURVE ( )  B_SPLINE_CURVE ( 3, ( #35936, #46914, #23869, #21 ),
 .UNSPECIFIED., .F., .F. ) 
 B_SPLINE_CURVE_WITH_KNOTS ( ( 4, 4 ),
 ( 4.712388980384689674, 6.283185307179586232 ),
 .UNSPECIFIED. ) 
 CURVE ( )  GEOMETRIC_REPRESENTATION_ITEM ( )  RATIONAL_B_SPLINE_CURVE ( ( 1.000000000000000000, 0.8047378541243649375, 0.8047378541243649375, 1.000000000000000000 ) ) 
 REPRESENTATION_ITEM ( '' )  );
#48300=FACE_OUTER_BOUND ( 'NONE', #27035, .T. ) ;
#48301=CYLINDRICAL_SURFACE ( 'NONE', #26588, 1.750000000000001554 ) ;
#48303=DIRECTION ( 'NONE',  ( -1.000000000000000000, 0.000000000000000000, 0.000000000000000000 ) ) ;
#48304=ORIENTED_EDGE ( 'NONE', *, *, #3111, .T. ) ;
#48306=ORIENTED_EDGE ( 'NONE', *, *, #23972, .T. ) ;
#48307=( BOUNDED_CURVE ( )  B_SPLINE_CURVE ( 3, ( #38006, #37757, #10033, #50237 ),
 .UNSPECIFIED., .F., .F. ) 
 B_SPLINE_CURVE_WITH_KNOTS ( ( 4, 4 ),
 ( 0.000000000000000000, 1.570796326794896558 ),
 .UNSPECIFIED. ) 
 CURVE ( )  GEOMETRIC_REPRESENTATION_ITEM ( )  RATIONAL_B_SPLINE_CURVE ( ( 1.000000000000000000, 0.8047378541243649375, 0.8047378541243649375, 1.000000000000000000 ) ) 
 REPRESENTATION_ITEM ( '' )  );
#48308=VECTOR ( 'NONE', #3726, 1000.000000000000000 ) ;
#48311=CARTESIAN_POINT ( 'NONE',  ( 210.0000000000000568, 2.143131898507881856E-16, -80.93171244307202983 ) ) ;
#48315=EDGE_LOOP ( 'NONE', ( #48747, #46691, #6338, #17548, #22889, #3935 ) ) ;
#48317=DIRECTION ( 'NONE',  ( -1.000000000000000000, -0.000000000000000000, -0.000000000000000000 ) ) ;
#48326=LINE ( 'NONE', #9123, #26247 ) ;
#48329=CARTESIAN_POINT ( 'NONE',  ( -207.7210997126620384, 1.750000000000009548, -40.20683870891912193 ) ) ;
#48333=FACE_OUTER_BOUND ( 'NONE', #45193, .T. ) ;
#48337=EDGE_CURVE ( 'NONE', #23318, #46337, #17233, .T. ) ;
#48338=EDGE_CURVE ( 'NONE', #48435, #27161, #41333, .T. ) ;
#48340=CYLINDRICAL_SURFACE ( 'NONE', #48392, 1.750000000000001554 ) ;
#48341=AXIS2_PLACEMENT_3D ( 'NONE', #698, #27909, #43535 ) ;
#48347=DIRECTION ( 'NONE',  ( -1.000000000000000000, 0.000000000000000000, 0.000000000000000000 ) ) ;
#48351=ORIENTED_EDGE ( 'NONE', *, *, #18172, .F. ) ;
#48358=EDGE_CURVE ( 'NONE', #45714, #45821, #49868, .T. ) ;
#48362=CARTESIAN_POINT ( 'NONE',  ( -167.7210997126620384, -1.750000000000009548, -0.2068387089191121020 ) ) ;
#48363=ORIENTED_EDGE ( 'NONE', *, *, #28156, .F. ) ;
#48364=ORIENTED_EDGE ( 'NONE', *, *, #33151, .T. ) ;
#48368=CARTESIAN_POINT ( 'NONE',  ( -6.695973446814940111, -1.750000000000023315, -159.1817124430720298 ) ) ;
#48375=ORIENTED_EDGE ( 'NONE', *, *, #39961, .T. ) ;
#48380=DIRECTION ( 'NONE',  ( 0.000000000000000000, 0.000000000000000000, -1.000000000000000000 ) ) ;
#48383=CARTESIAN_POINT ( 'NONE',  ( 112.2789002873379758, -1.749999999999996669, -158.1565861772249377 ) ) ;
#48384=CARTESIAN_POINT ( 'NONE',  ( -88.44597344681497475, 0.000000000000000000, -157.4317124430720014 ) ) ;
#48389=VECTOR ( 'NONE', #28131, 1000.000000000000000 ) ;
#48391=CARTESIAN_POINT ( 'NONE',  ( -88.44597344681494633, -1.025126265847089435, -157.4317124430720582 ) ) ;
#48392=AXIS2_PLACEMENT_3D ( 'NONE', #20422, #24540, #1947 ) ;
#48393=DIRECTION ( 'NONE',  ( 0.000000000000000000, 0.000000000000000000, 1.000000000000000000 ) ) ;
#48394=EDGE_CURVE ( 'NONE', #23844, #15960, #21759, .T. ) ;
#48395=CYLINDRICAL_SURFACE ( 'NONE', #15057, 1.750000000000010214 ) ;
#48397=ORIENTED_EDGE ( 'NONE', *, *, #482, .F. ) ;
#48400=LINE ( 'NONE', #24362, #43042 ) ;
#48401=DIRECTION ( 'NONE',  ( 0.000000000000000000, 0.000000000000000000, 1.000000000000000000 ) ) ;
#48402=EDGE_LOOP ( 'NONE', ( #37533, #42834 ) ) ;
#48403=CYLINDRICAL_SURFACE ( 'NONE', #22377, 1.750000000000015543 ) ;
#48404=CARTESIAN_POINT ( 'NONE',  ( -208.4459734468149463, 0.000000000000000000, 165.0000000000000000 ) ) ;
#48405=EDGE_CURVE ( 'NONE', #48120, #30382, #46947, .T. ) ;
#48406=EDGE_LOOP ( 'NONE', ( #3411, #7767, #37318, #50454, #47348 ) ) ;
#48412=ORIENTED_EDGE ( 'NONE', *, *, #23522, .T. ) ;
#48419=CYLINDRICAL_SURFACE ( 'NONE', #37203, 1.750000000000008438 ) ;
#48423=DIRECTION ( 'NONE',  ( 0.000000000000000000, 0.000000000000000000, 1.000000000000000000 ) ) ;
#48431=CARTESIAN_POINT ( 'NONE',  ( 151.5540265531850537, 0.000000000000000000, 165.0000000000000000 ) ) ;
#48435=VERTEX_POINT ( 'NONE', #11300 ) ;
#48436=DIRECTION ( 'NONE',  ( -0.000000000000000000, -0.000000000000000000, -1.000000000000000000 ) ) ;
#48441=( BOUNDED_CURVE ( )  B_SPLINE_CURVE ( 3, ( #16415, #40778, #32079, #47423 ),
 .UNSPECIFIED., .F., .F. ) 
 B_SPLINE_CURVE_WITH_KNOTS ( ( 4, 4 ),
 ( 4.712388980384689674, 6.283185307179586232 ),
 .UNSPECIFIED. ) 
 CURVE ( )  GEOMETRIC_REPRESENTATION_ITEM ( )  RATIONAL_B_SPLINE_CURVE ( ( 1.000000000000000000, 0.8047378541243649375, 0.8047378541243649375, 1.000000000000000000 ) ) 
 REPRESENTATION_ITEM ( '' )  );
#48442=CARTESIAN_POINT ( 'NONE',  ( -208.4459734468149463, 0.000000000000000000, 165.0000000000000000 ) ) ;
#48444=ADVANCED_FACE ( 'NONE', ( #38763 ), #3589, .T. ) ;
#48445=ORIENTED_EDGE ( 'NONE', *, *, #45717, .F. ) ;
#48448=( BOUNDED_CURVE ( )  B_SPLINE_CURVE ( 3, ( #3214, #18863, #34545, #50128 ),
 .UNSPECIFIED., .F., .F. ) 
 B_SPLINE_CURVE_WITH_KNOTS ( ( 4, 4 ),
 ( 0.000000000000000000, 1.570796326794896558 ),
 .UNSPECIFIED. ) 
 CURVE ( )  GEOMETRIC_REPRESENTATION_ITEM ( )  RATIONAL_B_SPLINE_CURVE ( ( 1.000000000000000000, 0.8047378541243649375, 0.8047378541243649375, 1.000000000000000000 ) ) 
 REPRESENTATION_ITEM ( '' )  );
#48450=CARTESIAN_POINT ( 'NONE',  ( 74.32915281903215998, 1.750000000000010214, -118.1565861772249519 ) ) ;
#48452=ORIENTED_EDGE ( 'NONE', *, *, #2614, .T. ) ;
#48453=ORIENTED_EDGE ( 'NONE', *, *, #44635, .F. ) ;
#48455=DIRECTION ( 'NONE',  ( 1.000000000000000000, 0.000000000000000000, 0.000000000000000000 ) ) ;
#48463=( BOUNDED_CURVE ( )  B_SPLINE_CURVE ( 3, ( #1113, #8560, #39872, #4706 ),
 .UNSPECIFIED., .F., .F. ) 
 B_SPLINE_CURVE_WITH_KNOTS ( ( 4, 4 ),
 ( 1.570796326794896558, 3.141592653589793116 ),
 .UNSPECIFIED. ) 
 CURVE ( )  GEOMETRIC_REPRESENTATION_ITEM ( )  RATIONAL_B_SPLINE_CURVE ( ( 1.000000000000000000, 0.8047378541243649375, 0.8047378541243649375, 1.000000000000000000 ) ) 
 REPRESENTATION_ITEM ( '' )  );
#48464=CARTESIAN_POINT ( 'NONE',  ( 210.0000000000000568, 0.000000000000000000, 40.81828755692798438 ) ) ;
#48470=VERTEX_POINT ( 'NONE', #4366 ) ;
#48471=LINE ( 'NONE', #13360, #32002 ) ;
#48473=VERTEX_POINT ( 'NONE', #8218 ) ;
#48474=EDGE_CURVE ( 'NONE', #28356, #3794, #47640, .T. ) ;
#48476=EDGE_CURVE ( 'NONE', #3985, #30782, #42430, .T. ) ;
#48484=DIRECTION ( 'NONE',  ( -1.000000000000000000, -0.000000000000000000, -0.000000000000000000 ) ) ;
#48485=VERTEX_POINT ( 'NONE', #23864 ) ;
#48486=ADVANCED_FACE ( 'NONE', ( #24378 ), #31579, .T. ) ;
#48487=ORIENTED_EDGE ( 'NONE', *, *, #38399, .T. ) ;
#48489=EDGE_CURVE ( 'NONE', #38537, #18600, #47920, .T. ) ;
#48494=CARTESIAN_POINT ( 'NONE',  ( 31.55402655318503236, 0.000000000000000000, -157.4317124430720014 ) ) ;
#48498=DIRECTION ( 'NONE',  ( -1.000000000000000000, -0.000000000000000000, -0.000000000000000000 ) ) ;
#48500=CYLINDRICAL_SURFACE ( 'NONE', #10414, 1.750000000000015543 ) ;
#48501=CARTESIAN_POINT ( 'NONE',  ( -206.6959734468149463, -1.750000000000010658, 120.8182875569279702 ) ) ;
#48502=CARTESIAN_POINT ( 'NONE',  ( 35.05402655318504657, -1.025126265847088991, 159.0682875569279418 ) ) ;
#48503=FACE_OUTER_BOUND ( 'NONE', #22681, .T. ) ;
#48504=ORIENTED_EDGE ( 'NONE', *, *, #28650, .F. ) ;
#48505=ORIENTED_EDGE ( 'NONE', *, *, #7214, .F. ) ;
#48507=CARTESIAN_POINT ( 'NONE',  ( -127.7210997126620242, 1.749999999999997113, 119.7931612910809065 ) ) ;
#48514=ORIENTED_EDGE ( 'NONE', *, *, #41008, .T. ) ;
#48515=CARTESIAN_POINT ( 'NONE',  ( -86.69597344681494633, 1.750000000000010658, -79.18171244307201562 ) ) ;
#48521=CARTESIAN_POINT ( 'NONE',  ( 210.0000000000000568, 2.143131898507880377E-16, -0.9317124430720331585 ) ) ;
#48524=AXIS2_PLACEMENT_3D ( 'NONE', #32554, #48137, #21737 ) ;
#48530=ORIENTED_EDGE ( 'NONE', *, *, #27439, .T. ) ;
#48533=EDGE_LOOP ( 'NONE', ( #12772, #38412, #1537, #26954, #18342, #33991 ) ) ;
#48536=CARTESIAN_POINT ( 'NONE',  ( 192.2789002873380184, 1.750000000000009326, 1.843413822775066269 ) ) ;
#48552=ORIENTED_EDGE ( 'NONE', *, *, #16445, .F. ) ;
#48562=EDGE_CURVE ( 'NONE', #40406, #27344, #7382, .T. ) ;
#48567=VECTOR ( 'NONE', #27942, 1000.000000000000000 ) ;
#48572=ORIENTED_EDGE ( 'NONE', *, *, #21247, .F. ) ;
#48574=DIRECTION ( 'NONE',  ( 0.000000000000000000, 0.000000000000000000, 1.000000000000000000 ) ) ;
#48579=DIRECTION ( 'NONE',  ( 1.000000000000000000, 0.000000000000000000, 0.000000000000000000 ) ) ;
#48583=DIRECTION ( 'NONE',  ( -1.000000000000000000, -0.000000000000000000, -0.000000000000000000 ) ) ;
#48584=CARTESIAN_POINT ( 'NONE',  ( 115.0540265531850395, 2.143131898507847836E-16, 165.0000000000000000 ) ) ;
#48586=EDGE_CURVE ( 'NONE', #44363, #4914, #39775, .T. ) ;
#48587=CARTESIAN_POINT ( 'NONE',  ( -6.695973446814940111, 0.000000000000000000, 165.0000000000000000 ) ) ;
#48588=VECTOR ( 'NONE', #4108, 1000.000000000000000 ) ;
#48591=DIRECTION ( 'NONE',  ( 0.000000000000000000, 0.000000000000000000, -1.000000000000000000 ) ) ;
#48593=CIRCLE ( 'NONE', #1948, 1.750000000000008438 ) ;
#48595=ORIENTED_EDGE ( 'NONE', *, *, #37164, .T. ) ;
#48596=CARTESIAN_POINT ( 'NONE',  ( -84.94597344681494633, 2.143131898507880377E-16, -0.9317124430720247208 ) ) ;
#48601=CARTESIAN_POINT ( 'NONE',  ( 31.55402655318503236, 0.000000000000000000, 39.06828755692798438 ) ) ;
#48602=( BOUNDED_CURVE ( )  B_SPLINE_CURVE ( 3, ( #31286, #12030, #3295, #35397 ),
 .UNSPECIFIED., .F., .F. ) 
 B_SPLINE_CURVE_WITH_KNOTS ( ( 4, 4 ),
 ( 0.000000000000000000, 1.570796326794896558 ),
 .UNSPECIFIED. ) 
 CURVE ( )  GEOMETRIC_REPRESENTATION_ITEM ( )  RATIONAL_B_SPLINE_CURVE ( ( 1.000000000000000000, 0.8047378541243649375, 0.8047378541243649375, 1.000000000000000000 ) ) 
 REPRESENTATION_ITEM ( '' )  );
#48603=ORIENTED_EDGE ( 'NONE', *, *, #27453, .T. ) ;
#48604=LINE ( 'NONE', #9402, #44577 ) ;
#48611=FACE_OUTER_BOUND ( 'NONE', #4688, .T. ) ;
#48612=VERTEX_POINT ( 'NONE', #40028 ) ;
#48615=DIRECTION ( 'NONE',  ( -1.000000000000000000, -0.000000000000000000, -0.000000000000000000 ) ) ;
#48617=DIRECTION ( 'NONE',  ( -1.000000000000000000, -0.000000000000000000, -0.000000000000000000 ) ) ;
#48618=EDGE_LOOP ( 'NONE', ( #658, #14844, #20451, #36427, #42222, #31103 ) ) ;
#48619=CARTESIAN_POINT ( 'NONE',  ( 113.3040265531850537, 0.000000000000000000, -165.0000000000000000 ) ) ;
#48620=AXIS2_PLACEMENT_3D ( 'NONE', #42584, #14640, #26704 ) ;
#48621=CARTESIAN_POINT ( 'NONE',  ( 75.05402655318509630, -1.025126265847089435, 82.56828755692798438 ) ) ;
#48627=CARTESIAN_POINT ( 'NONE',  ( 155.0540265531850537, 2.143131898507880377E-16, 159.0682875569279702 ) ) ;
#48629=ORIENTED_EDGE ( 'NONE', *, *, #12687, .T. ) ;
#48630=EDGE_CURVE ( 'NONE', #29600, #20835, #32835, .T. ) ;
#48632=CARTESIAN_POINT ( 'NONE',  ( -86.69597344681494633, -1.750000000000009992, 160.8182875569279702 ) ) ;
#48637=DIRECTION ( 'NONE',  ( -1.000000000000000000, 0.000000000000000000, 0.000000000000000000 ) ) ;
#48639=ADVANCED_FACE ( 'NONE', ( #21772 ), #48419, .T. ) ;
#48644=ORIENTED_EDGE ( 'NONE', *, *, #15287, .F. ) ;
#48646=CARTESIAN_POINT ( 'NONE',  ( 115.0540265531850395, 2.143131898507847836E-16, -0.9317124430719969652 ) ) ;
#48647=CARTESIAN_POINT ( 'NONE',  ( -166.6959734468149463, -1.750000000000009992, 0.8182875569279768335 ) ) ;
#48648=CARTESIAN_POINT ( 'NONE',  ( 195.0540265531851105, 2.143131898507880377E-16, -0.9317124430720247208 ) ) ;
#48650=CARTESIAN_POINT ( 'NONE',  ( 73.30402655318508209, 0.000000000000000000, 165.0000000000000000 ) ) ;
#48665=EDGE_CURVE ( 'NONE', #39055, #19705, #33912, .T. ) ;
#48669=ORIENTED_EDGE ( 'NONE', *, *, #43149, .F. ) ;
#48671=LINE ( 'NONE', #24872, #32447 ) ;
#48672=EDGE_CURVE ( 'NONE', #387, #11195, #12614, .T. ) ;
#48674=ORIENTED_EDGE ( 'NONE', *, *, #10325, .T. ) ;
#48675=EDGE_CURVE ( 'NONE', #22379, #1434, #30309, .T. ) ;
#48677=EDGE_CURVE ( 'NONE', #29337, #44889, #19810, .T. ) ;
#48678=AXIS2_PLACEMENT_3D ( 'NONE', #10631, #41682, #33749 ) ;
#48680=CARTESIAN_POINT ( 'NONE',  ( -6.695973446814940111, -1.750000000000023315, 0.8182875569279768335 ) ) ;
#48682=ORIENTED_EDGE ( 'NONE', *, *, #18472, .T. ) ;
#48687=DIRECTION ( 'NONE',  ( -1.000000000000000000, -0.000000000000000000, -0.000000000000000000 ) ) ;
#48690=DIRECTION ( 'NONE',  ( 0.000000000000000000, 0.000000000000000000, -1.000000000000000000 ) ) ;
#48696=FACE_OUTER_BOUND ( 'NONE', #50394, .T. ) ;
#48698=ADVANCED_FACE ( 'NONE', ( #5101 ), #2267, .T. ) ;
#48703=EDGE_CURVE ( 'NONE', #39370, #15868, #25628, .T. ) ;
#48712=DIRECTION ( 'NONE',  ( -1.000000000000000000, -0.000000000000000000, -0.000000000000000000 ) ) ;
#48713=FACE_OUTER_BOUND ( 'NONE', #22948, .T. ) ;
#48714=DIRECTION ( 'NONE',  ( -1.000000000000000000, -0.000000000000000000, -0.000000000000000000 ) ) ;
#48715=ORIENTED_EDGE ( 'NONE', *, *, #10479, .F. ) ;
#48721=ORIENTED_EDGE ( 'NONE', *, *, #49536, .F. ) ;
#48723=DIRECTION ( 'NONE',  ( 1.000000000000000000, 0.000000000000000000, 0.000000000000000000 ) ) ;
#48724=CARTESIAN_POINT ( 'NONE',  ( -166.6959734468149463, -1.750000000000009992, 160.8182875569279702 ) ) ;
#48725=ADVANCED_FACE ( 'NONE', ( #49175 ), #49430, .T. ) ;
#48726=ORIENTED_EDGE ( 'NONE', *, *, #2352, .F. ) ;
#48727=AXIS2_PLACEMENT_3D ( 'NONE', #41118, #21882, #2609 ) ;
#48728=ADVANCED_FACE ( 'NONE', ( #14827 ), #30482, .T. ) ;
#48729=CARTESIAN_POINT ( 'NONE',  ( 35.05402655318504657, -1.025126265847089435, 39.06828755692797728 ) ) ;
#48737=DIRECTION ( 'NONE',  ( 0.000000000000000000, 0.000000000000000000, 1.000000000000000000 ) ) ;
#48741=VERTEX_POINT ( 'NONE', #11248 ) ;
#48743=AXIS2_PLACEMENT_3D ( 'NONE', #26534, #46495, #46247 ) ;
#48744=( BOUNDED_CURVE ( )  B_SPLINE_CURVE ( 3, ( #18970, #34648, #15131, #19478 ),
 .UNSPECIFIED., .F., .F. ) 
 B_SPLINE_CURVE_WITH_KNOTS ( ( 4, 4 ),
 ( 4.712388980384689674, 6.283185307179586232 ),
 .UNSPECIFIED. ) 
 CURVE ( )  GEOMETRIC_REPRESENTATION_ITEM ( )  RATIONAL_B_SPLINE_CURVE ( ( 1.000000000000000000, 0.8047378541243649375, 0.8047378541243649375, 1.000000000000000000 ) ) 
 REPRESENTATION_ITEM ( '' )  );
#48747=ORIENTED_EDGE ( 'NONE', *, *, #34837, .T. ) ;
#48750=( BOUNDED_CURVE ( )  B_SPLINE_CURVE ( 3, ( #8010, #23646, #7752, #3371 ),
 .UNSPECIFIED., .F., .F. ) 
 B_SPLINE_CURVE_WITH_KNOTS ( ( 4, 4 ),
 ( 3.141592653589793116, 4.712388980384689674 ),
 .UNSPECIFIED. ) 
 CURVE ( )  GEOMETRIC_REPRESENTATION_ITEM ( )  RATIONAL_B_SPLINE_CURVE ( ( 1.000000000000000000, 0.8047378541243649375, 0.8047378541243649375, 1.000000000000000000 ) ) 
 REPRESENTATION_ITEM ( '' )  );
#48752=ORIENTED_EDGE ( 'NONE', *, *, #47001, .T. ) ;
#48753=CARTESIAN_POINT ( 'NONE',  ( -4.945973446814903696, 2.143131898507912917E-16, -160.9317124430720582 ) ) ;
#48757=ORIENTED_EDGE ( 'NONE', *, *, #5194, .T. ) ;
#48758=ORIENTED_EDGE ( 'NONE', *, *, #13944, .F. ) ;
#48759=ADVANCED_FACE ( 'NONE', ( #2523 ), #7399, .T. ) ;
#48760=CARTESIAN_POINT ( 'NONE',  ( 33.30402655318503946, 0.000000000000000000, 165.0000000000000000 ) ) ;
#48766=( BOUNDED_CURVE ( )  B_SPLINE_CURVE ( 3, ( #39133, #47018, #8078, #19354 ),
 .UNSPECIFIED., .F., .F. ) 
 B_SPLINE_CURVE_WITH_KNOTS ( ( 4, 4 ),
 ( 3.141592653589793116, 4.712388980384689674 ),
 .UNSPECIFIED. ) 
 CURVE ( )  GEOMETRIC_REPRESENTATION_ITEM ( )  RATIONAL_B_SPLINE_CURVE ( ( 1.000000000000000000, 0.8047378541243649375, 0.8047378541243649375, 1.000000000000000000 ) ) 
 REPRESENTATION_ITEM ( '' )  );
#48768=EDGE_LOOP ( 'NONE', ( #31211, #31165, #35955, #19116, #50263, #18718 ) ) ;
#48772=LINE ( 'NONE', #26226, #1565 ) ;
#48773=CIRCLE ( 'NONE', #46326, 1.750000000000008438 ) ;
#48774=FACE_OUTER_BOUND ( 'NONE', #19640, .T. ) ;
#48779=CARTESIAN_POINT ( 'NONE',  ( -168.4459734468149463, 0.000000000000000000, 165.0000000000000000 ) ) ;
#48781=CARTESIAN_POINT ( 'NONE',  ( 35.05402655318504657, 2.143131898507880377E-16, 79.06828755692797017 ) ) ;
#48782=ORIENTED_EDGE ( 'NONE', *, *, #29922, .F. ) ;
#48783=CARTESIAN_POINT ( 'NONE',  ( -8.445973446814964092, -1.025126265847097207, 39.06828755692796307 ) ) ;
#48788=ADVANCED_FACE ( 'NONE', ( #3518 ), #30227, .T. ) ;
#48794=PLANE ( 'NONE',  #2052 ) ;
#48803=ORIENTED_EDGE ( 'NONE', *, *, #23078, .F. ) ;
#48808=ORIENTED_EDGE ( 'NONE', *, *, #18331, .F. ) ;
#48809=LINE ( 'NONE', #10101, #32997 ) ;
#48810=DIRECTION ( 'NONE',  ( -1.000000000000000000, -0.000000000000000000, -0.000000000000000000 ) ) ;
#48812=ORIENTED_EDGE ( 'NONE', *, *, #39367, .F. ) ;
#48813=EDGE_CURVE ( 'NONE', #34969, #11740, #30611, .T. ) ;
#48817=VERTEX_POINT ( 'NONE', #12004 ) ;
#48819=FACE_OUTER_BOUND ( 'NONE', #50602, .T. ) ;
#48823=DIRECTION ( 'NONE',  ( 1.000000000000000000, 0.000000000000000000, 0.000000000000000000 ) ) ;
#48825=ORIENTED_EDGE ( 'NONE', *, *, #37313, .T. ) ;
#48826=LINE ( 'NONE', #21670, #14386 ) ;
#48828=CARTESIAN_POINT ( 'NONE',  ( 113.3040265531850537, -1.749999999999997335, -79.18171244307201562 ) ) ;
#48831=ADVANCED_FACE ( 'NONE', ( #42771 ), #35623, .T. ) ;
#48835=ORIENTED_EDGE ( 'NONE', *, *, #26843, .F. ) ;
#48838=EDGE_CURVE ( 'NONE', #7277, #40406, #37521, .T. ) ;
#48843=CYLINDRICAL_SURFACE ( 'NONE', #10112, 1.750000000000008438 ) ;
#48844=CARTESIAN_POINT ( 'NONE',  ( 151.5540265531850537, 0.000000000000000000, -0.9317124430720247208 ) ) ;
#48851=CARTESIAN_POINT ( 'NONE',  ( -47.72109971266203132, 1.750000000000009548, 121.8434138227750623 ) ) ;
#48852=DIRECTION ( 'NONE',  ( -0.000000000000000000, -0.000000000000000000, -1.000000000000000000 ) ) ;
#48853=DIRECTION ( 'NONE',  ( -0.000000000000000000, -0.000000000000000000, -1.000000000000000000 ) ) ;
#48857=CARTESIAN_POINT ( 'NONE',  ( -208.4459734468148611, -1.025126265847089435, 2.568287556927986159 ) ) ;
#48860=CARTESIAN_POINT ( 'NONE',  ( -48.44597344681492501, 2.143131898507880377E-16, -160.9317124430720298 ) ) ;
#48861=AXIS2_PLACEMENT_3D ( 'NONE', #33854, #22536, #18928 ) ;
#48863=CYLINDRICAL_SURFACE ( 'NONE', #8224, 1.749999999999987566 ) ;
#48865=VERTEX_POINT ( 'NONE', #43541 ) ;
#48866=ORIENTED_EDGE ( 'NONE', *, *, #49404, .F. ) ;
#48872=ORIENTED_EDGE ( 'NONE', *, *, #24859, .F. ) ;
#48875=CYLINDRICAL_SURFACE ( 'NONE', #32732, 1.750000000000015543 ) ;
#48876=ORIENTED_EDGE ( 'NONE', *, *, #735, .F. ) ;
#48877=VERTEX_POINT ( 'NONE', #23806 ) ;
#48878=CARTESIAN_POINT ( 'NONE',  ( 154.3291528190321458, -1.750000000000009326, 159.7931612910809065 ) ) ;
#48881=ORIENTED_EDGE ( 'NONE', *, *, #32894, .F. ) ;
#48882=CARTESIAN_POINT ( 'NONE',  ( -84.94597344681494633, 2.143131898507880377E-16, 165.0000000000000000 ) ) ;
#48883=CARTESIAN_POINT ( 'NONE',  ( -206.6959734468149463, -1.750000000000010214, 40.81828755692798438 ) ) ;
#48887=CARTESIAN_POINT ( 'NONE',  ( -48.44597344681496054, -1.025126265847089213, 162.5682875569279133 ) ) ;
#48889=CARTESIAN_POINT ( 'NONE',  ( -208.4459734468149179, 2.143131898507880377E-16, -160.9317124430720298 ) ) ;
#48892=( BOUNDED_CURVE ( )  B_SPLINE_CURVE ( 3, ( #46250, #22429, #49329, #2430 ),
 .UNSPECIFIED., .F., .F. ) 
 B_SPLINE_CURVE_WITH_KNOTS ( ( 4, 4 ),
 ( 0.000000000000000000, 1.570796326794896558 ),
 .UNSPECIFIED. ) 
 CURVE ( )  GEOMETRIC_REPRESENTATION_ITEM ( )  RATIONAL_B_SPLINE_CURVE ( ( 1.000000000000000000, 0.8047378541243649375, 0.8047378541243649375, 1.000000000000000000 ) ) 
 REPRESENTATION_ITEM ( '' )  );
#48898=( BOUNDED_CURVE ( )  B_SPLINE_CURVE ( 3, ( #14344, #37976, #10500, #26399 ),
 .UNSPECIFIED., .F., .F. ) 
 B_SPLINE_CURVE_WITH_KNOTS ( ( 4, 4 ),
 ( 0.000000000000000000, 1.570796326794896558 ),
 .UNSPECIFIED. ) 
 CURVE ( )  GEOMETRIC_REPRESENTATION_ITEM ( )  RATIONAL_B_SPLINE_CURVE ( ( 1.000000000000000000, 0.8047378541243649375, 0.8047378541243649375, 1.000000000000000000 ) ) 
 REPRESENTATION_ITEM ( '' )  );
#48901=CARTESIAN_POINT ( 'NONE',  ( 195.0540265531851105, 1.025126265847089213, -0.9317124430720324924 ) ) ;
#48902=ORIENTED_EDGE ( 'NONE', *, *, #37344, .F. ) ;
#48906=CYLINDRICAL_SURFACE ( 'NONE', #13229, 1.750000000000015543 ) ;
#48908=CARTESIAN_POINT ( 'NONE',  ( 153.3040265531850537, 1.750000000000010658, -119.1817124430720440 ) ) ;
#48909=DIRECTION ( 'NONE',  ( -1.000000000000000000, 0.000000000000000000, 0.000000000000000000 ) ) ;
#48911=CARTESIAN_POINT ( 'NONE',  ( 72.27890028733797578, -1.750000000000010214, -80.20683870891910772 ) ) ;
#48913=EDGE_LOOP ( 'NONE', ( #14943, #15743, #9619, #35361, #46649, #1258 ) ) ;
#48914=VERTEX_POINT ( 'NONE', #35121 ) ;
#48915=DIRECTION ( 'NONE',  ( 0.000000000000000000, 0.000000000000000000, 1.000000000000000000 ) ) ;
#48923=ORIENTED_EDGE ( 'NONE', *, *, #42554, .F. ) ;
#48925=ADVANCED_FACE ( 'NONE', ( #39212 ), #15598, .T. ) ;
#48931=ORIENTED_EDGE ( 'NONE', *, *, #48703, .F. ) ;
#48935=ORIENTED_EDGE ( 'NONE', *, *, #25262, .T. ) ;
#48938=CARTESIAN_POINT ( 'NONE',  ( 210.0000000000000568, 0.000000000000000000, -159.1817124430720298 ) ) ;
#48942=CARTESIAN_POINT ( 'NONE',  ( 151.5540265531850537, -1.025126265847089657, -80.93171244307201562 ) ) ;
#48956=CARTESIAN_POINT ( 'NONE',  ( -46.69597344681494633, 1.750000000000010658, 80.81828755692798438 ) ) ;
#48957=EDGE_CURVE ( 'NONE', #38145, #10859, #9630, .T. ) ;
#48958=VERTEX_POINT ( 'NONE', #40719 ) ;
#48966=ADVANCED_FACE ( 'NONE', ( #17608 ), #965, .T. ) ;
#48967=EDGE_CURVE ( 'NONE', #2042, #40520, #14869, .T. ) ;
#48969=ORIENTED_EDGE ( 'NONE', *, *, #15540, .F. ) ;
#48970=ADVANCED_FACE ( 'NONE', ( #48611 ), #41204, .T. ) ;
#48971=CARTESIAN_POINT ( 'NONE',  ( 210.0000000000000568, 2.143131898507880377E-16, -0.9317124430720331585 ) ) ;
#48974=( BOUNDED_CURVE ( )  B_SPLINE_CURVE ( 3, ( #7165, #27424, #35145, #31029 ),
 .UNSPECIFIED., .F., .F. ) 
 B_SPLINE_CURVE_WITH_KNOTS ( ( 4, 4 ),
 ( 1.570796326794896558, 3.141592653589793116 ),
 .UNSPECIFIED. ) 
 CURVE ( )  GEOMETRIC_REPRESENTATION_ITEM ( )  RATIONAL_B_SPLINE_CURVE ( ( 1.000000000000000000, 0.8047378541243649375, 0.8047378541243649375, 1.000000000000000000 ) ) 
 REPRESENTATION_ITEM ( '' )  );
#48977=CARTESIAN_POINT ( 'NONE',  ( 72.27890028733797578, 1.750000000000009548, -40.20683870891912193 ) ) ;
#48982=EDGE_CURVE ( 'NONE', #18302, #43286, #17106, .T. ) ;
#48985=EDGE_LOOP ( 'NONE', ( #3748, #15910, #24376, #28662, #43182, #46376 ) ) ;
#48986=CARTESIAN_POINT ( 'NONE',  ( 193.3040265531851105, 1.750000000000009992, -159.1817124430720298 ) ) ;
#48989=CARTESIAN_POINT ( 'NONE',  ( -168.4459734468149747, -1.025126265847089657, -37.43171244307202272 ) ) ;
#48994=FACE_OUTER_BOUND ( 'NONE', #38817, .T. ) ;
#49001=EDGE_LOOP ( 'NONE', ( #49106, #50316, #26862, #37430, #13584 ) ) ;
#49002=CARTESIAN_POINT ( 'NONE',  ( 151.5540265531850537, 0.000000000000000000, -37.43171244307205825 ) ) ;
#49003=CARTESIAN_POINT ( 'NONE',  ( -44.94597344681493922, -1.025126265847089213, 42.56828755692799149 ) ) ;
#49005=CARTESIAN_POINT ( 'NONE',  ( 71.55402655318505367, 0.000000000000000000, 2.568287556928006143 ) ) ;
#49007=ORIENTED_EDGE ( 'NONE', *, *, #24252, .F. ) ;
#49008=EDGE_CURVE ( 'NONE', #43597, #28550, #40209, .T. ) ;
#49011=CARTESIAN_POINT ( 'NONE',  ( 74.32915281903215998, -1.750000000000009548, -160.2068387089191219 ) ) ;
#49012=PLANE ( 'NONE',  #41623 ) ;
#49016=CARTESIAN_POINT ( 'NONE',  ( 151.5540265531850537, 1.025126265847089213, -160.9317124430720014 ) ) ;
#49017=DIRECTION ( 'NONE',  ( -1.000000000000000000, -0.000000000000000000, -0.000000000000000000 ) ) ;
#49019=ORIENTED_EDGE ( 'NONE', *, *, #20459, .F. ) ;
#49023=CARTESIAN_POINT ( 'NONE',  ( 71.55402655318505367, 1.025126265847088991, -157.4317124430720582 ) ) ;
#49024=CARTESIAN_POINT ( 'NONE',  ( 71.55402655318505367, 0.000000000000000000, 2.568287556928006143 ) ) ;
#49026=CARTESIAN_POINT ( 'NONE',  ( -124.9459734468149321, -1.025126265847081219, 2.568287556927973281 ) ) ;
#49030=DIRECTION ( 'NONE',  ( -0.000000000000000000, -0.000000000000000000, -1.000000000000000000 ) ) ;
#49034=( BOUNDED_CURVE ( )  B_SPLINE_CURVE ( 3, ( #10538, #2098, #6439, #6198 ),
 .UNSPECIFIED., .F., .F. ) 
 B_SPLINE_CURVE_WITH_KNOTS ( ( 4, 4 ),
 ( 0.000000000000000000, 1.570796326794896558 ),
 .UNSPECIFIED. ) 
 CURVE ( )  GEOMETRIC_REPRESENTATION_ITEM ( )  RATIONAL_B_SPLINE_CURVE ( ( 1.000000000000000000, 0.8047378541243649375, 0.8047378541243649375, 1.000000000000000000 ) ) 
 REPRESENTATION_ITEM ( '' )  );
#49043=CARTESIAN_POINT ( 'NONE',  ( 210.0000000000000568, 0.000000000000000000, 80.81828755692798438 ) ) ;
#49045=( BOUNDED_CURVE ( )  B_SPLINE_CURVE ( 3, ( #29466, #44574, #48911, #9456 ),
 .UNSPECIFIED., .F., .F. ) 
 B_SPLINE_CURVE_WITH_KNOTS ( ( 4, 4 ),
 ( 0.000000000000000000, 1.570796326794896558 ),
 .UNSPECIFIED. ) 
 CURVE ( )  GEOMETRIC_REPRESENTATION_ITEM ( )  RATIONAL_B_SPLINE_CURVE ( ( 1.000000000000000000, 0.8047378541243649375, 0.8047378541243649375, 1.000000000000000000 ) ) 
 REPRESENTATION_ITEM ( '' )  );
#49048=DIRECTION ( 'NONE',  ( 1.000000000000000000, 0.000000000000000000, -0.000000000000000000 ) ) ;
#49055=CARTESIAN_POINT ( 'NONE',  ( -85.67084718096784002, -1.750000000000009548, -40.20683870891912193 ) ) ;
#49057=CARTESIAN_POINT ( 'NONE',  ( -47.72109971266203132, 1.750000000000010436, -120.2068387089191219 ) ) ;
#49059=EDGE_LOOP ( 'NONE', ( #34179, #13804, #25935, #18565, #30688, #40026 ) ) ;
#49061=ORIENTED_EDGE ( 'NONE', *, *, #19343, .F. ) ;
#49064=ADVANCED_FACE ( 'NONE', ( #41465 ), #6322, .T. ) ;
#49066=FACE_OUTER_BOUND ( 'NONE', #32120, .T. ) ;
#49067=ORIENTED_EDGE ( 'NONE', *, *, #40264, .T. ) ;
#49069=CARTESIAN_POINT ( 'NONE',  ( -166.6959734468149463, -1.750000000000009992, 0.8182875569279768335 ) ) ;
#49072=LINE ( 'NONE', #45493, #43615 ) ;
#49073=VECTOR ( 'NONE', #19232, 1000.000000000000000 ) ;
#49077=AXIS2_PLACEMENT_3D ( 'NONE', #12469, #43516, #36355 ) ;
#49079=CARTESIAN_POINT ( 'NONE',  ( 32.27890028733795447, -1.750000000000009548, 159.7931612910809065 ) ) ;
#49080=CARTESIAN_POINT ( 'NONE',  ( -88.44597344681497475, 0.000000000000000000, 165.0000000000000000 ) ) ;
#49083=AXIS2_PLACEMENT_3D ( 'NONE', #13421, #16273, #8329 ) ;
#49087=CARTESIAN_POINT ( 'NONE',  ( -207.7210997126620384, 1.750000000000009548, 41.84341382277508359 ) ) ;
#49092=AXIS2_PLACEMENT_3D ( 'NONE', #36882, #33272, #44774 ) ;
#49099=EDGE_LOOP ( 'NONE', ( #38037, #11018, #48881, #29272, #11549, #3864 ) ) ;
#49106=ORIENTED_EDGE ( 'NONE', *, *, #48154, .F. ) ;
#49108=DIRECTION ( 'NONE',  ( 0.000000000000000000, 0.000000000000000000, 1.000000000000000000 ) ) ;
#49109=CARTESIAN_POINT ( 'NONE',  ( 75.05402655318509630, 2.143131898507880377E-16, 39.06828755692795596 ) ) ;
#49111=EDGE_CURVE ( 'NONE', #4629, #37476, #502, .T. ) ;
#49113=EDGE_CURVE ( 'NONE', #7079, #9194, #17855, .T. ) ;
#49114=EDGE_LOOP ( 'NONE', ( #42360, #39348, #38005, #1574, #36661, #45494 ) ) ;
#49115=DIRECTION ( 'NONE',  ( -0.000000000000000000, -0.000000000000000000, -1.000000000000000000 ) ) ;
#49119=VERTEX_POINT ( 'NONE', #18602 ) ;
#49121=EDGE_CURVE ( 'NONE', #34539, #3215, #39167, .T. ) ;
#49124=CARTESIAN_POINT ( 'NONE',  ( -88.44597344681494633, -1.025126265847089435, 2.568287556927986159 ) ) ;
#49126=LINE ( 'NONE', #29669, #25093 ) ;
#49127=VECTOR ( 'NONE', #20070, 1000.000000000000000 ) ;
#49130=DIRECTION ( 'NONE',  ( 0.000000000000000000, 0.000000000000000000, 1.000000000000000000 ) ) ;
#49136=EDGE_CURVE ( 'NONE', #24507, #50669, #41309, .T. ) ;
#49138=ORIENTED_EDGE ( 'NONE', *, *, #36112, .F. ) ;
#49142=CARTESIAN_POINT ( 'NONE',  ( 72.27890028733797578, 1.750000000000009548, 41.84341382277508359 ) ) ;
#49146=DIRECTION ( 'NONE',  ( 0.000000000000000000, 0.000000000000000000, 1.000000000000000000 ) ) ;
#49147=CARTESIAN_POINT ( 'NONE',  ( -166.6959734468149463, 1.750000000000009992, 0.8182875569279768335 ) ) ;
#49151=CARTESIAN_POINT ( 'NONE',  ( 75.05402655318509630, 2.143131898507880377E-16, 165.0000000000000000 ) ) ;
#49154=LINE ( 'NONE', #2744, #45798 ) ;
#49157=LINE ( 'NONE', #18645, #32048 ) ;
#49166=CYLINDRICAL_SURFACE ( 'NONE', #23344, 1.750000000000010214 ) ;
#49168=LINE ( 'NONE', #37686, #15092 ) ;
#49175=FACE_OUTER_BOUND ( 'NONE', #19770, .T. ) ;
#49176=ORIENTED_EDGE ( 'NONE', *, *, #14690, .F. ) ;
#49178=CARTESIAN_POINT ( 'NONE',  ( -46.69597344681494633, 0.000000000000000000, 165.0000000000000000 ) ) ;
#49182=CIRCLE ( 'NONE', #48341, 1.750000000000015543 ) ;
#49187=ORIENTED_EDGE ( 'NONE', *, *, #18952, .T. ) ;
#49194=EDGE_CURVE ( 'NONE', #29500, #37204, #23424, .T. ) ;
#49199=FACE_OUTER_BOUND ( 'NONE', #19747, .T. ) ;
#49202=DIRECTION ( 'NONE',  ( 1.000000000000000000, 0.000000000000000000, -0.000000000000000000 ) ) ;
#49206=( BOUNDED_CURVE ( )  B_SPLINE_CURVE ( 3, ( #10128, #25787, #46002, #3170 ),
 .UNSPECIFIED., .F., .F. ) 
 B_SPLINE_CURVE_WITH_KNOTS ( ( 4, 4 ),
 ( 4.712388980384689674, 6.283185307179586232 ),
 .UNSPECIFIED. ) 
 CURVE ( )  GEOMETRIC_REPRESENTATION_ITEM ( )  RATIONAL_B_SPLINE_CURVE ( ( 1.000000000000000000, 0.8047378541243649375, 0.8047378541243649375, 1.000000000000000000 ) ) 
 REPRESENTATION_ITEM ( '' )  );
#49208=ORIENTED_EDGE ( 'NONE', *, *, #25508, .F. ) ;
#49210=CARTESIAN_POINT ( 'NONE',  ( 115.0540265531850395, 2.143131898507847836E-16, -117.4317124430720725 ) ) ;
#49215=CARTESIAN_POINT ( 'NONE',  ( 111.5540265531850537, 1.025126265847081886, -80.93171244307201562 ) ) ;
#49219=CARTESIAN_POINT ( 'NONE',  ( -87.72109971266203843, 1.750000000000009548, 161.8434138227750907 ) ) ;
#49227=VECTOR ( 'NONE', #11465, 1000.000000000000000 ) ;
#49230=CARTESIAN_POINT ( 'NONE',  ( -165.6708471809677974, -1.750000000000009548, 161.8434138227750907 ) ) ;
#49231=ORIENTED_EDGE ( 'NONE', *, *, #32170, .F. ) ;
#49233=ORIENTED_EDGE ( 'NONE', *, *, #9846, .F. ) ;
#49235=CARTESIAN_POINT ( 'NONE',  ( -124.9459734468149321, -1.025126265847081442, -0.9317124430720195027 ) ) ;
#49243=CARTESIAN_POINT ( 'NONE',  ( -210.0000000000000568, 0.000000000000000000, -79.18171244307201562 ) ) ;
#49250=CARTESIAN_POINT ( 'NONE',  ( -167.7210997126620384, 1.750000000000010436, 79.79316129108087807 ) ) ;
#49256=CARTESIAN_POINT ( 'NONE',  ( -4.945973446814903696, 2.143131898507912917E-16, 82.56828755692801280 ) ) ;
#49257=ORIENTED_EDGE ( 'NONE', *, *, #14454, .T. ) ;
#49264=DIRECTION ( 'NONE',  ( 0.000000000000000000, 0.000000000000000000, 1.000000000000000000 ) ) ;
#49265=ORIENTED_EDGE ( 'NONE', *, *, #43773, .F. ) ;
#49266=ADVANCED_FACE ( 'NONE', ( #8097 ), #23742, .T. ) ;
#49268=ORIENTED_EDGE ( 'NONE', *, *, #34192, .T. ) ;
#49270=CARTESIAN_POINT ( 'NONE',  ( 75.05402655318509630, 2.143131898507880377E-16, -120.9317124430720725 ) ) ;
#49273=CARTESIAN_POINT ( 'NONE',  ( 153.3040265531850537, 1.750000000000009992, -159.1817124430720298 ) ) ;
#49275=ORIENTED_EDGE ( 'NONE', *, *, #7121, .T. ) ;
#49278=CARTESIAN_POINT ( 'NONE',  ( 33.30402655318503946, -1.750000000000009992, -159.1817124430720298 ) ) ;
#49279=EDGE_CURVE ( 'NONE', #5910, #30190, #42709, .T. ) ;
#49281=EDGE_CURVE ( 'NONE', #46895, #28486, #27006, .T. ) ;
#49284=( BOUNDED_CURVE ( )  B_SPLINE_CURVE ( 3, ( #40821, #13109, #5666, #24931 ),
 .UNSPECIFIED., .F., .F. ) 
 B_SPLINE_CURVE_WITH_KNOTS ( ( 4, 4 ),
 ( 0.000000000000000000, 1.570796326794896558 ),
 .UNSPECIFIED. ) 
 CURVE ( )  GEOMETRIC_REPRESENTATION_ITEM ( )  RATIONAL_B_SPLINE_CURVE ( ( 1.000000000000000000, 0.8047378541243649375, 0.8047378541243649375, 1.000000000000000000 ) ) 
 REPRESENTATION_ITEM ( '' )  );
#49285=CARTESIAN_POINT ( 'NONE',  ( -204.9459734468149463, 2.143131898507880377E-16, 165.0000000000000000 ) ) ;
#49287=FACE_OUTER_BOUND ( 'NONE', #5267, .T. ) ;
#49294=CYLINDRICAL_SURFACE ( 'NONE', #7458, 1.750000000000008438 ) ;
#49299=EDGE_CURVE ( 'NONE', #40803, #49373, #46303, .T. ) ;
#49302=ADVANCED_FACE ( 'NONE', ( #16801 ), #32205, .T. ) ;
#49309=CARTESIAN_POINT ( 'NONE',  ( 115.0540265531850395, -1.025126265847081219, -157.4317124430720582 ) ) ;
#49310=EDGE_CURVE ( 'NONE', #7014, #17256, #41094, .T. ) ;
#49315=DIRECTION ( 'NONE',  ( 0.000000000000000000, 0.000000000000000000, 1.000000000000000000 ) ) ;
#49318=ORIENTED_EDGE ( 'NONE', *, *, #16445, .T. ) ;
#49325=VECTOR ( 'NONE', #31366, 1000.000000000000000 ) ;
#49326=CYLINDRICAL_SURFACE ( 'NONE', #34006, 1.750000000000036193 ) ;
#49328=DIRECTION ( 'NONE',  ( -0.000000000000000000, -0.000000000000000000, -1.000000000000000000 ) ) ;
#49329=CARTESIAN_POINT ( 'NONE',  ( -167.7210997126620384, -1.750000000000009548, -40.20683870891912193 ) ) ;
#49332=LINE ( 'NONE', #37366, #32337 ) ;
#49335=CYLINDRICAL_SURFACE ( 'NONE', #34709, 1.750000000000008438 ) ;
#49337=CARTESIAN_POINT ( 'NONE',  ( -168.4459734468149463, 0.000000000000000000, -157.4317124430720582 ) ) ;
#49339=ADVANCED_FACE ( 'NONE', ( #5497 ), #48301, .T. ) ;
#49340=EDGE_CURVE ( 'NONE', #18024, #20654, #32465, .T. ) ;
#49341=( BOUNDED_CURVE ( )  B_SPLINE_CURVE ( 3, ( #31702, #42957, #136, #38890 ),
 .UNSPECIFIED., .F., .F. ) 
 B_SPLINE_CURVE_WITH_KNOTS ( ( 4, 4 ),
 ( 0.000000000000000000, 1.570796326794896558 ),
 .UNSPECIFIED. ) 
 CURVE ( )  GEOMETRIC_REPRESENTATION_ITEM ( )  RATIONAL_B_SPLINE_CURVE ( ( 1.000000000000000000, 0.8047378541243649375, 0.8047378541243649375, 1.000000000000000000 ) ) 
 REPRESENTATION_ITEM ( '' )  );
#49344=DIRECTION ( 'NONE',  ( -0.000000000000000000, -0.000000000000000000, -1.000000000000000000 ) ) ;
#49345=CARTESIAN_POINT ( 'NONE',  ( 191.5540265531851105, 0.000000000000000000, 79.06828755692797017 ) ) ;
#49349=( BOUNDED_CURVE ( )  B_SPLINE_CURVE ( 3, ( #12599, #46958, #43899, #27510 ),
 .UNSPECIFIED., .F., .F. ) 
 B_SPLINE_CURVE_WITH_KNOTS ( ( 4, 4 ),
 ( 4.712388980384689674, 6.283185307179586232 ),
 .UNSPECIFIED. ) 
 CURVE ( )  GEOMETRIC_REPRESENTATION_ITEM ( )  RATIONAL_B_SPLINE_CURVE ( ( 1.000000000000000000, 0.8047378541243649375, 0.8047378541243649375, 1.000000000000000000 ) ) 
 REPRESENTATION_ITEM ( '' )  );
#49356=CARTESIAN_POINT ( 'NONE',  ( 152.2789002873379900, -1.750000000000009548, 41.84341382277508359 ) ) ;
#49359=VECTOR ( 'NONE', #32800, 1000.000000000000000 ) ;
#49361=VERTEX_POINT ( 'NONE', #17301 ) ;
#49365=EDGE_CURVE ( 'NONE', #19154, #48435, #32972, .T. ) ;
#49368=AXIS2_PLACEMENT_3D ( 'NONE', #6303, #49344, #40942 ) ;
#49373=VERTEX_POINT ( 'NONE', #2885 ) ;
#49377=LINE ( 'NONE', #45789, #20987 ) ;
#49378=ORIENTED_EDGE ( 'NONE', *, *, #3670, .F. ) ;
#49380=CARTESIAN_POINT ( 'NONE',  ( 73.30402655318508209, -1.750000000000010658, 80.81828755692798438 ) ) ;
#49384=CYLINDRICAL_SURFACE ( 'NONE', #45867, 1.750000000000001554 ) ;
#49391=CARTESIAN_POINT ( 'NONE',  ( 33.30402655318503946, 1.750000000000010658, -119.1817124430720440 ) ) ;
#49392=CARTESIAN_POINT ( 'NONE',  ( 153.3040265531850537, 0.000000000000000000, 165.0000000000000000 ) ) ;
#49398=VECTOR ( 'NONE', #28508, 1000.000000000000000 ) ;
#49399=CARTESIAN_POINT ( 'NONE',  ( 115.0540265531850395, -1.025126265847081219, 2.568287556927973281 ) ) ;
#49400=CARTESIAN_POINT ( 'NONE',  ( -44.94597344681493922, 1.025126265847089213, -160.9317124430720014 ) ) ;
#49404=EDGE_CURVE ( 'NONE', #45594, #27492, #38868, .T. ) ;
#49407=CARTESIAN_POINT ( 'NONE',  ( -6.695973446814940111, 0.000000000000000000, 165.0000000000000000 ) ) ;
#49414=ADVANCED_FACE ( 'NONE', ( #34479 ), #29359, .T. ) ;
#49415=ORIENTED_EDGE ( 'NONE', *, *, #16489, .T. ) ;
#49417=ORIENTED_EDGE ( 'NONE', *, *, #50496, .F. ) ;
#49423=EDGE_LOOP ( 'NONE', ( #43502, #34823, #48412, #18179, #9321, #42578 ) ) ;
#49426=EDGE_LOOP ( 'NONE', ( #7651, #45826, #21929, #7586, #19690, #36067 ) ) ;
#49427=CARTESIAN_POINT ( 'NONE',  ( -87.72109971266203843, -1.750000000000009548, -38.15658617722494483 ) ) ;
#49429=CARTESIAN_POINT ( 'NONE',  ( 210.0000000000000568, 0.000000000000000000, -77.43171244307200141 ) ) ;
#49430=CYLINDRICAL_SURFACE ( 'NONE', #26552, 1.750000000000010214 ) ;
#49431=VECTOR ( 'NONE', #25374, 1000.000000000000000 ) ;
#49433=AXIS2_PLACEMENT_3D ( 'NONE', #49407, #2499, #6600 ) ;
#49434=CARTESIAN_POINT ( 'NONE',  ( 75.05402655318509630, -1.025126265847089213, -0.9317124430720324924 ) ) ;
#49437=AXIS2_PLACEMENT_3D ( 'NONE', #10713, #38693, #6874 ) ;
#49441=EDGE_LOOP ( 'NONE', ( #39275, #6427, #30247, #5742, #19815 ) ) ;
#49444=ORIENTED_EDGE ( 'NONE', *, *, #35287, .T. ) ;
#49445=ORIENTED_EDGE ( 'NONE', *, *, #45095, .T. ) ;
#49447=LINE ( 'NONE', #2538, #12284 ) ;
#49448=DIRECTION ( 'NONE',  ( -1.000000000000000000, 0.000000000000000000, 0.000000000000000000 ) ) ;
#49452=DIRECTION ( 'NONE',  ( -1.000000000000000000, -0.000000000000000000, -0.000000000000000000 ) ) ;
#49455=CARTESIAN_POINT ( 'NONE',  ( -128.4459734468149179, 0.000000000000000000, 42.56828755692794175 ) ) ;
#49464=EDGE_CURVE ( 'NONE', #1049, #20141, #26714, .T. ) ;
#49468=CARTESIAN_POINT ( 'NONE',  ( 31.55402655318503236, 0.000000000000000000, 79.06828755692797017 ) ) ;
#49470=CYLINDRICAL_SURFACE ( 'NONE', #19778, 1.750000000000008438 ) ;
#49473=CARTESIAN_POINT ( 'NONE',  ( 210.0000000000000568, 0.000000000000000000, 120.8182875569279702 ) ) ;
#49474=CARTESIAN_POINT ( 'NONE',  ( -126.6959734468149321, 1.749999999999997335, 120.8182875569279702 ) ) ;
#49476=EDGE_CURVE ( 'NONE', #45927, #43947, #35575, .T. ) ;
#49479=CARTESIAN_POINT ( 'NONE',  ( -166.6959734468149463, 0.000000000000000000, 165.0000000000000000 ) ) ;
#49485=CARTESIAN_POINT ( 'NONE',  ( 75.05402655318509630, -1.025126265847089213, -37.43171244307202272 ) ) ;
#49490=LINE ( 'NONE', #48971, #13587 ) ;
#49493=CARTESIAN_POINT ( 'NONE',  ( -164.9459734468149463, -1.025126265847089657, 119.0682875569279560 ) ) ;
#49495=CARTESIAN_POINT ( 'NONE',  ( -46.69597344681494633, -1.750000000000009992, 0.8182875569279768335 ) ) ;
#49497=ORIENTED_EDGE ( 'NONE', *, *, #26959, .F. ) ;
#49500=VERTEX_POINT ( 'NONE', #7015 ) ;
#49505=( BOUNDED_CURVE ( )  B_SPLINE_CURVE ( 3, ( #21675, #41172, #2678, #49584 ),
 .UNSPECIFIED., .F., .F. ) 
 B_SPLINE_CURVE_WITH_KNOTS ( ( 4, 4 ),
 ( 4.712388980384689674, 6.283185307179586232 ),
 .UNSPECIFIED. ) 
 CURVE ( )  GEOMETRIC_REPRESENTATION_ITEM ( )  RATIONAL_B_SPLINE_CURVE ( ( 1.000000000000000000, 0.8047378541243649375, 0.8047378541243649375, 1.000000000000000000 ) ) 
 REPRESENTATION_ITEM ( '' )  );
#49507=ORIENTED_EDGE ( 'NONE', *, *, #40910, .T. ) ;
#49509=EDGE_CURVE ( 'NONE', #49806, #13126, #793, .T. ) ;
#49512=CARTESIAN_POINT ( 'NONE',  ( -86.69597344681494633, 1.750000000000010214, 40.81828755692798438 ) ) ;
#49518=ORIENTED_EDGE ( 'NONE', *, *, #49663, .F. ) ;
#49519=CARTESIAN_POINT ( 'NONE',  ( 195.0540265531851105, -1.025126265847089435, -117.4317124430720156 ) ) ;
#49520=DIRECTION ( 'NONE',  ( 0.000000000000000000, 0.000000000000000000, 1.000000000000000000 ) ) ;
#49525=AXIS2_PLACEMENT_3D ( 'NONE', #31363, #27252, #42877 ) ;
#49527=ORIENTED_EDGE ( 'NONE', *, *, #36260, .T. ) ;
#49534=CARTESIAN_POINT ( 'NONE',  ( 113.3040265531850537, 1.749999999999997335, 80.81828755692798438 ) ) ;
#49535=EDGE_LOOP ( 'NONE', ( #44662, #8917, #11466, #34208, #37927, #17182 ) ) ;
#49536=EDGE_CURVE ( 'NONE', #19269, #920, #27280, .T. ) ;
#49537=CARTESIAN_POINT ( 'NONE',  ( 210.0000000000000568, 0.000000000000000000, 160.8182875569279702 ) ) ;
#49544=CARTESIAN_POINT ( 'NONE',  ( 151.5540265531850537, 0.000000000000000000, -0.9317124430720247208 ) ) ;
#49545=ORIENTED_EDGE ( 'NONE', *, *, #38424, .T. ) ;
#49546=CARTESIAN_POINT ( 'NONE',  ( -45.67084718096785423, 1.750000000000009548, 39.79316129108089228 ) ) ;
#49548=CARTESIAN_POINT ( 'NONE',  ( -4.945973446814917018, 1.025126265847096763, 162.5682875569279986 ) ) ;
#49549=VERTEX_POINT ( 'NONE', #19055 ) ;
#49552=CARTESIAN_POINT ( 'NONE',  ( -124.9459734468149321, 1.025126265847082108, -37.43171244307203693 ) ) ;
#49555=ORIENTED_EDGE ( 'NONE', *, *, #39324, .T. ) ;
#49557=CARTESIAN_POINT ( 'NONE',  ( 35.05402655318504657, 2.143131898507880377E-16, -77.43171244307198720 ) ) ;
#49559=ORIENTED_EDGE ( 'NONE', *, *, #14179, .T. ) ;
#49560=CARTESIAN_POINT ( 'NONE',  ( 33.30402655318503946, 0.000000000000000000, 165.0000000000000000 ) ) ;
#49564=CARTESIAN_POINT ( 'NONE',  ( -47.72109971266203132, -1.750000000000010214, -120.2068387089191219 ) ) ;
#49567=VECTOR ( 'NONE', #48687, 1000.000000000000000 ) ;
#49569=LINE ( 'NONE', #14471, #37434 ) ;
#49572=CARTESIAN_POINT ( 'NONE',  ( -4.945973446814917018, -1.025126265847096985, -0.9317124430720461481 ) ) ;
#49574=EDGE_LOOP ( 'NONE', ( #23568, #13999, #28945, #26323, #11281, #20182 ) ) ;
#49576=CARTESIAN_POINT ( 'NONE',  ( 33.30402655318503946, 0.000000000000000000, 165.0000000000000000 ) ) ;
#49578=VERTEX_POINT ( 'NONE', #7530 ) ;
#49579=CARTESIAN_POINT ( 'NONE',  ( -48.44597344681495343, 0.000000000000000000, -77.43171244307198720 ) ) ;
#49583=( BOUNDED_CURVE ( )  B_SPLINE_CURVE ( 3, ( #11365, #46473, #27782, #8289 ),
 .UNSPECIFIED., .F., .F. ) 
 B_SPLINE_CURVE_WITH_KNOTS ( ( 4, 4 ),
 ( 3.141592653589793116, 4.712388980384689674 ),
 .UNSPECIFIED. ) 
 CURVE ( )  GEOMETRIC_REPRESENTATION_ITEM ( )  RATIONAL_B_SPLINE_CURVE ( ( 1.000000000000000000, 0.8047378541243649375, 0.8047378541243649375, 1.000000000000000000 ) ) 
 REPRESENTATION_ITEM ( '' )  );
#49584=CARTESIAN_POINT ( 'NONE',  ( -164.9459734468149463, 2.143131898507880377E-16, 79.06828755692797017 ) ) ;
#49586=FACE_OUTER_BOUND ( 'NONE', #22955, .T. ) ;
#49591=ADVANCED_FACE ( 'NONE', ( #42656 ), #15468, .T. ) ;
#49593=CARTESIAN_POINT ( 'NONE',  ( 191.5540265531851105, 0.000000000000000000, -117.4317124430720725 ) ) ;
#49594=CARTESIAN_POINT ( 'NONE',  ( 152.2789002873379900, -1.750000000000009548, -0.2068387089191121020 ) ) ;
#49595=EDGE_CURVE ( 'NONE', #13512, #20319, #14967, .T. ) ;
#49604=CARTESIAN_POINT ( 'NONE',  ( 75.05402655318509630, 2.143131898507873721E-16, 165.0000000000000000 ) ) ;
#49608=EDGE_LOOP ( 'NONE', ( #13499, #37809, #40551, #25144, #14796, #41672 ) ) ;
#49611=AXIS2_PLACEMENT_3D ( 'NONE', #23871, #35438, #7469 ) ;
#49616=FACE_OUTER_BOUND ( 'NONE', #9420, .T. ) ;
#49620=EDGE_CURVE ( 'NONE', #35947, #11473, #38841, .T. ) ;
#49624=EDGE_CURVE ( 'NONE', #47427, #17436, #42721, .T. ) ;
#49625=VECTOR ( 'NONE', #29605, 1000.000000000000000 ) ;
#49626=ORIENTED_EDGE ( 'NONE', *, *, #42556, .F. ) ;
#49627=EDGE_CURVE ( 'NONE', #36951, #13485, #49583, .T. ) ;
#49628=DIRECTION ( 'NONE',  ( -1.000000000000000000, -0.000000000000000000, -0.000000000000000000 ) ) ;
#49632=ORIENTED_EDGE ( 'NONE', *, *, #6753, .T. ) ;
#49633=VECTOR ( 'NONE', #35252, 1000.000000000000000 ) ;
#49634=ORIENTED_EDGE ( 'NONE', *, *, #45840, .T. ) ;
#49636=EDGE_CURVE ( 'NONE', #14002, #18060, #2434, .T. ) ;
#49638=EDGE_CURVE ( 'NONE', #33796, #42641, #28656, .T. ) ;
#49639=CARTESIAN_POINT ( 'NONE',  ( 114.3291528190321173, 1.749999999999996669, -38.15658617722495194 ) ) ;
#49640=EDGE_LOOP ( 'NONE', ( #17892, #16937, #27463, #49991, #44006, #4195 ) ) ;
#49641=CARTESIAN_POINT ( 'NONE',  ( 193.3040265531851105, 1.750000000000010214, 40.81828755692798438 ) ) ;
#49642=( BOUNDED_CURVE ( )  B_SPLINE_CURVE ( 3, ( #22332, #45906, #41839, #49495 ),
 .UNSPECIFIED., .F., .F. ) 
 B_SPLINE_CURVE_WITH_KNOTS ( ( 4, 4 ),
 ( 3.141592653589793116, 4.712388980384689674 ),
 .UNSPECIFIED. ) 
 CURVE ( )  GEOMETRIC_REPRESENTATION_ITEM ( )  RATIONAL_B_SPLINE_CURVE ( ( 1.000000000000000000, 0.8047378541243649375, 0.8047378541243649375, 1.000000000000000000 ) ) 
 REPRESENTATION_ITEM ( '' )  );
#49643=CARTESIAN_POINT ( 'NONE',  ( -6.695973446814940111, 1.750000000000024203, 120.8182875569279702 ) ) ;
#49646=ORIENTED_EDGE ( 'NONE', *, *, #431, .F. ) ;
#49648=LINE ( 'NONE', #22750, #1298 ) ;
#49650=CARTESIAN_POINT ( 'NONE',  ( -44.94597344681493922, 2.143131898507880377E-16, -160.9317124430720582 ) ) ;
#49659=CARTESIAN_POINT ( 'NONE',  ( -6.695973446814940111, 1.750000000000024203, 80.81828755692798438 ) ) ;
#49663=EDGE_CURVE ( 'NONE', #21262, #7318, #4690, .T. ) ;
#49673=CARTESIAN_POINT ( 'NONE',  ( 35.05402655318504657, -1.025126265847088991, 2.568287556927986159 ) ) ;
#49675=ORIENTED_EDGE ( 'NONE', *, *, #28495, .T. ) ;
#49679=CARTESIAN_POINT ( 'NONE',  ( -168.4459734468149747, 1.025126265847089213, 42.56828755692799149 ) ) ;
#49687=CARTESIAN_POINT ( 'NONE',  ( 210.0000000000000568, 0.000000000000000000, 80.81828755692798438 ) ) ;
#49688=CARTESIAN_POINT ( 'NONE',  ( 73.30402655318508209, 1.750000000000009992, 160.8182875569279702 ) ) ;
#49691=ORIENTED_EDGE ( 'NONE', *, *, #46093, .F. ) ;
#49693=DIRECTION ( 'NONE',  ( -0.000000000000000000, -0.000000000000000000, -1.000000000000000000 ) ) ;
#49697=ORIENTED_EDGE ( 'NONE', *, *, #27580, .T. ) ;
#49702=ADVANCED_FACE ( 'NONE', ( #41533 ), #12376, .T. ) ;
#49703=CARTESIAN_POINT ( 'NONE',  ( -208.4459734468148611, 1.025126265847089435, 82.56828755692798438 ) ) ;
#49705=CARTESIAN_POINT ( 'NONE',  ( -86.69597344681494633, -1.750000000000010658, 120.8182875569279702 ) ) ;
#49706=DIRECTION ( 'NONE',  ( -1.000000000000000000, -0.000000000000000000, -0.000000000000000000 ) ) ;
#49711=CARTESIAN_POINT ( 'NONE',  ( 155.0540265531850537, 2.143131898507880377E-16, 119.0682875569279702 ) ) ;
#49720=CARTESIAN_POINT ( 'NONE',  ( 210.0000000000000568, 0.000000000000000000, 40.81828755692798438 ) ) ;
#49723=CARTESIAN_POINT ( 'NONE',  ( -46.69597344681494633, 1.750000000000010658, -79.18171244307201562 ) ) ;
#49724=ORIENTED_EDGE ( 'NONE', *, *, #14715, .T. ) ;
#49727=CARTESIAN_POINT ( 'NONE',  ( 75.05402655318509630, 2.143131898507880377E-16, 165.0000000000000000 ) ) ;
#49728=ORIENTED_EDGE ( 'NONE', *, *, #15563, .T. ) ;
#49730=CARTESIAN_POINT ( 'NONE',  ( 210.0000000000000568, 0.000000000000000000, 122.5682875569279844 ) ) ;
#49731=ORIENTED_EDGE ( 'NONE', *, *, #44643, .F. ) ;
#49737=FACE_OUTER_BOUND ( 'NONE', #37783, .T. ) ;
#49749=DIRECTION ( 'NONE',  ( -0.000000000000000000, -0.000000000000000000, -1.000000000000000000 ) ) ;
#49754=CARTESIAN_POINT ( 'NONE',  ( 210.0000000000000568, 0.000000000000000000, 160.8182875569279702 ) ) ;
#49757=DIRECTION ( 'NONE',  ( 0.000000000000000000, 0.000000000000000000, 1.000000000000000000 ) ) ;
#49760=CARTESIAN_POINT ( 'NONE',  ( 75.05402655318508209, 0.000000000000000000, 162.5682875569279702 ) ) ;
#49762=CARTESIAN_POINT ( 'NONE',  ( -84.94597344681493212, 1.025126265847089879, 82.56828755692798438 ) ) ;
#49768=CARTESIAN_POINT ( 'NONE',  ( 73.30402655318508209, 1.750000000000010658, -119.1817124430720440 ) ) ;
#49769=CARTESIAN_POINT ( 'NONE',  ( -44.94597344681497475, 0.000000000000000000, 162.5682875569279702 ) ) ;
#49772=CARTESIAN_POINT ( 'NONE',  ( -125.6708471809678542, 1.749999999999996669, -158.1565861772249377 ) ) ;
#49773=DIRECTION ( 'NONE',  ( 0.000000000000000000, 0.000000000000000000, 1.000000000000000000 ) ) ;
#49775=VERTEX_POINT ( 'NONE', #34105 ) ;
#49776=CARTESIAN_POINT ( 'NONE',  ( -164.9459734468149463, 1.025126265847089435, 2.568287556927986159 ) ) ;
#49777=CARTESIAN_POINT ( 'NONE',  ( -88.44597344681497475, 0.000000000000000000, 165.0000000000000000 ) ) ;
#49778=CARTESIAN_POINT ( 'NONE',  ( -204.9459734468149463, 2.143131898507880377E-16, 165.0000000000000000 ) ) ;
#49779=( BOUNDED_CURVE ( )  B_SPLINE_CURVE ( 3, ( #7261, #38838, #50309, #15462 ),
 .UNSPECIFIED., .F., .F. ) 
 B_SPLINE_CURVE_WITH_KNOTS ( ( 4, 4 ),
 ( 1.570796326794896558, 3.141592653589793116 ),
 .UNSPECIFIED. ) 
 CURVE ( )  GEOMETRIC_REPRESENTATION_ITEM ( )  RATIONAL_B_SPLINE_CURVE ( ( 1.000000000000000000, 0.8047378541243649375, 0.8047378541243649375, 1.000000000000000000 ) ) 
 REPRESENTATION_ITEM ( '' )  );
#49780=CARTESIAN_POINT ( 'NONE',  ( -164.9459734468149463, 2.143131898507880377E-16, 2.568287556927978166 ) ) ;
#49785=( BOUNDED_CURVE ( )  B_SPLINE_CURVE ( 3, ( #19351, #35037, #46758, #12587 ),
 .UNSPECIFIED., .F., .F. ) 
 B_SPLINE_CURVE_WITH_KNOTS ( ( 4, 4 ),
 ( 1.570796326794896558, 3.141592653589793116 ),
 .UNSPECIFIED. ) 
 CURVE ( )  GEOMETRIC_REPRESENTATION_ITEM ( )  RATIONAL_B_SPLINE_CURVE ( ( 1.000000000000000000, 0.8047378541243649375, 0.8047378541243649375, 1.000000000000000000 ) ) 
 REPRESENTATION_ITEM ( '' )  );
#49786=CARTESIAN_POINT ( 'NONE',  ( -88.44597344681497475, 0.000000000000000000, -80.93171244307204404 ) ) ;
#49789=ADVANCED_FACE ( 'NONE', ( #10482 ), #10729, .T. ) ;
#49792=CARTESIAN_POINT ( 'NONE',  ( -166.6959734468149463, -1.750000000000009992, 0.8182875569279768335 ) ) ;
#49794=CARTESIAN_POINT ( 'NONE',  ( -127.7210997126620242, -1.749999999999996669, 1.843413822775057609 ) ) ;
#49795=( BOUNDED_CURVE ( )  B_SPLINE_CURVE ( 3, ( #25718, #17764, #33431, #44923 ),
 .UNSPECIFIED., .F., .F. ) 
 B_SPLINE_CURVE_WITH_KNOTS ( ( 4, 4 ),
 ( 0.000000000000000000, 1.570796326794896780 ),
 .UNSPECIFIED. ) 
 CURVE ( )  GEOMETRIC_REPRESENTATION_ITEM ( )  RATIONAL_B_SPLINE_CURVE ( ( 1.000000000000000000, 0.8047378541243649375, 0.8047378541243649375, 1.000000000000000000 ) ) 
 REPRESENTATION_ITEM ( '' )  );
#49797=VERTEX_POINT ( 'NONE', #3524 ) ;
#49801=ORIENTED_EDGE ( 'NONE', *, *, #45375, .T. ) ;
#49806=VERTEX_POINT ( 'NONE', #22026 ) ;
#49811=CARTESIAN_POINT ( 'NONE',  ( 71.55402655318505367, 0.000000000000000000, -157.4317124430720014 ) ) ;
#49812=ORIENTED_EDGE ( 'NONE', *, *, #32434, .T. ) ;
#49822=CARTESIAN_POINT ( 'NONE',  ( -7.721099712662037540, 1.750000000000023315, -160.2068387089191219 ) ) ;
#49839=CARTESIAN_POINT ( 'NONE',  ( -167.7210997126620384, 1.750000000000009548, 121.8434138227750623 ) ) ;
#49841=ORIENTED_EDGE ( 'NONE', *, *, #48129, .T. ) ;
#49849=EDGE_LOOP ( 'NONE', ( #45766, #44215, #21647, #30141, #50067, #4652 ) ) ;
#49852=ORIENTED_EDGE ( 'NONE', *, *, #40735, .F. ) ;
#49857=VERTEX_POINT ( 'NONE', #41777 ) ;
#49862=DIRECTION ( 'NONE',  ( -1.000000000000000000, -0.000000000000000000, -0.000000000000000000 ) ) ;
#49863=ORIENTED_EDGE ( 'NONE', *, *, #44014, .F. ) ;
#49867=ORIENTED_EDGE ( 'NONE', *, *, #36978, .F. ) ;
#49868=( BOUNDED_CURVE ( )  B_SPLINE_CURVE ( 3, ( #41587, #45904, #6434, #15405 ),
 .UNSPECIFIED., .F., .F. ) 
 B_SPLINE_CURVE_WITH_KNOTS ( ( 4, 4 ),
 ( 3.141592653589793116, 4.712388980384689674 ),
 .UNSPECIFIED. ) 
 CURVE ( )  GEOMETRIC_REPRESENTATION_ITEM ( )  RATIONAL_B_SPLINE_CURVE ( ( 1.000000000000000000, 0.8047378541243649375, 0.8047378541243649375, 1.000000000000000000 ) ) 
 REPRESENTATION_ITEM ( '' )  );
#49872=EDGE_CURVE ( 'NONE', #37204, #16089, #44369, .T. ) ;
#49885=CARTESIAN_POINT ( 'NONE',  ( 210.0000000000000568, 0.000000000000000000, -117.4317124430720298 ) ) ;
#49887=DIRECTION ( 'NONE',  ( -0.000000000000000000, -0.000000000000000000, -1.000000000000000000 ) ) ;
#49890=CARTESIAN_POINT ( 'NONE',  ( -165.6708471809677974, -1.750000000000009548, -160.2068387089191219 ) ) ;
#49891=EDGE_CURVE ( 'NONE', #17971, #49361, #4084, .T. ) ;
#49892=CARTESIAN_POINT ( 'NONE',  ( -88.44597344681494633, 1.025126265847089435, -77.43171244307200141 ) ) ;
#49896=DIRECTION ( 'NONE',  ( 0.000000000000000000, 0.000000000000000000, 1.000000000000000000 ) ) ;
#49898=ADVANCED_FACE ( 'NONE', ( #14326 ), #34866, .F. ) ;
#49905=EDGE_CURVE ( 'NONE', #44210, #14142, #23104, .T. ) ;
#49906=AXIS2_PLACEMENT_3D ( 'NONE', #16839, #13735, #28629 ) ;
#49907=CARTESIAN_POINT ( 'NONE',  ( -164.9459734468149463, 1.025126265847089879, 122.5682875569280128 ) ) ;
#49911=CARTESIAN_POINT ( 'NONE',  ( -126.6959734468149321, 1.749999999999997335, -79.18171244307201562 ) ) ;
#49913=DIRECTION ( 'NONE',  ( -1.000000000000000000, 0.000000000000000000, 0.000000000000000000 ) ) ;
#49918=VERTEX_POINT ( 'NONE', #45842 ) ;
#49921=CARTESIAN_POINT ( 'NONE',  ( -126.6959734468149321, 1.749999999999997113, 40.81828755692798438 ) ) ;
#49922=CARTESIAN_POINT ( 'NONE',  ( 210.0000000000000568, 0.000000000000000000, 0.8182875569279768335 ) ) ;
#49932=( BOUNDED_CURVE ( )  B_SPLINE_CURVE ( 3, ( #20545, #13094, #47696, #5393 ),
 .UNSPECIFIED., .F., .F. ) 
 B_SPLINE_CURVE_WITH_KNOTS ( ( 4, 4 ),
 ( 3.141592653589793116, 4.712388980384689674 ),
 .UNSPECIFIED. ) 
 CURVE ( )  GEOMETRIC_REPRESENTATION_ITEM ( )  RATIONAL_B_SPLINE_CURVE ( ( 1.000000000000000000, 0.8047378541243649375, 0.8047378541243649375, 1.000000000000000000 ) ) 
 REPRESENTATION_ITEM ( '' )  );
#49936=CARTESIAN_POINT ( 'NONE',  ( -166.6959734468149463, -1.750000000000010214, 40.81828755692798438 ) ) ;
#49940=ORIENTED_EDGE ( 'NONE', *, *, #45859, .T. ) ;
#49943=( BOUNDED_CURVE ( )  B_SPLINE_CURVE ( 3, ( #28334, #46077, #38439, #47787 ),
 .UNSPECIFIED., .F., .F. ) 
 B_SPLINE_CURVE_WITH_KNOTS ( ( 4, 4 ),
 ( 0.000000000000000000, 1.570796326794896558 ),
 .UNSPECIFIED. ) 
 CURVE ( )  GEOMETRIC_REPRESENTATION_ITEM ( )  RATIONAL_B_SPLINE_CURVE ( ( 1.000000000000000000, 0.8047378541243649375, 0.8047378541243649375, 1.000000000000000000 ) ) 
 REPRESENTATION_ITEM ( '' )  );
#49946=AXIS2_PLACEMENT_3D ( 'NONE', #24558, #32017, #700 ) ;
#49947=ADVANCED_FACE ( 'NONE', ( #36128 ), #43035, .T. ) ;
#49949=DIRECTION ( 'NONE',  ( -1.000000000000000000, 0.000000000000000000, 0.000000000000000000 ) ) ;
#49957=AXIS2_PLACEMENT_3D ( 'NONE', #34819, #50395, #3217 ) ;
#49961=LINE ( 'NONE', #14864, #3584 ) ;
#49962=CARTESIAN_POINT ( 'NONE',  ( -125.6708471809678542, 1.749999999999996891, 119.7931612910809065 ) ) ;
#49963=ADVANCED_FACE ( 'NONE', ( #39473 ), #4558, .T. ) ;
#49964=CARTESIAN_POINT ( 'NONE',  ( -128.4459734468149463, -1.025126265847081886, -120.9317124430720440 ) ) ;
#49965=DIRECTION ( 'NONE',  ( -1.000000000000000000, 0.000000000000000000, 0.000000000000000000 ) ) ;
#49967=CARTESIAN_POINT ( 'NONE',  ( -166.6959734468149463, 1.750000000000010658, 120.8182875569279702 ) ) ;
#49972=EDGE_CURVE ( 'NONE', #49549, #28356, #40797, .T. ) ;
#49974=EDGE_CURVE ( 'NONE', #920, #2364, #46001, .T. ) ;
#49979=DIRECTION ( 'NONE',  ( -0.000000000000000000, -0.000000000000000000, -1.000000000000000000 ) ) ;
#49980=LINE ( 'NONE', #49730, #6074 ) ;
#49991=ORIENTED_EDGE ( 'NONE', *, *, #46296, .F. ) ;
#49993=CARTESIAN_POINT ( 'NONE',  ( 111.5540265531850679, 0.000000000000000000, 165.0000000000000000 ) ) ;
#49994=CYLINDRICAL_SURFACE ( 'NONE', #35589, 1.750000000000001554 ) ;
#49999=ORIENTED_EDGE ( 'NONE', *, *, #25600, .T. ) ;
#50006=ORIENTED_EDGE ( 'NONE', *, *, #43904, .T. ) ;
#50007=FACE_OUTER_BOUND ( 'NONE', #39019, .T. ) ;
#50008=CARTESIAN_POINT ( 'NONE',  ( -128.4459734468149463, -1.025126265847082108, -77.43171244307201562 ) ) ;
#50017=ORIENTED_EDGE ( 'NONE', *, *, #24678, .T. ) ;
#50020=CARTESIAN_POINT ( 'NONE',  ( -168.4459734468149463, 0.000000000000000000, -157.4317124430720582 ) ) ;
#50021=CARTESIAN_POINT ( 'NONE',  ( 155.0540265531850537, 2.143131898507880377E-16, -120.9317124430720156 ) ) ;
#50033=VERTEX_POINT ( 'NONE', #43798 ) ;
#50038=EDGE_CURVE ( 'NONE', #38466, #17310, #9159, .T. ) ;
#50042=EDGE_CURVE ( 'NONE', #36777, #8111, #44073, .T. ) ;
#50043=DIRECTION ( 'NONE',  ( -1.000000000000000000, -0.000000000000000000, -0.000000000000000000 ) ) ;
#50044=CARTESIAN_POINT ( 'NONE',  ( -124.9459734468149605, 0.000000000000000000, 162.5682875569279702 ) ) ;
#50045=ORIENTED_EDGE ( 'NONE', *, *, #32504, .T. ) ;
#50051=EDGE_LOOP ( 'NONE', ( #47984, #28977, #2366, #34817, #580, #35858 ) ) ;
#50052=ORIENTED_EDGE ( 'NONE', *, *, #49404, .T. ) ;
#50055=ORIENTED_EDGE ( 'NONE', *, *, #29937, .T. ) ;
#50057=DIRECTION ( 'NONE',  ( -0.000000000000000000, -0.000000000000000000, -1.000000000000000000 ) ) ;
#50064=CIRCLE ( 'NONE', #2570, 1.750000000000001554 ) ;
#50065=CARTESIAN_POINT ( 'NONE',  ( -127.7210997126620242, -1.749999999999996669, -40.20683870891911482 ) ) ;
#50067=ORIENTED_EDGE ( 'NONE', *, *, #4360, .F. ) ;
#50071=CARTESIAN_POINT ( 'NONE',  ( -210.0000000000000568, 2.143131898507876926E-16, 119.0682875569279560 ) ) ;
#50074=ORIENTED_EDGE ( 'NONE', *, *, #11821, .F. ) ;
#50076=CARTESIAN_POINT ( 'NONE',  ( -164.9459734468149463, 1.025126265847089657, 42.56828755692799149 ) ) ;
#50077=ORIENTED_EDGE ( 'NONE', *, *, #38467, .T. ) ;
#50081=CARTESIAN_POINT ( 'NONE',  ( 75.05402655318509630, 2.143131898507880377E-16, -117.4317124430720156 ) ) ;
#50083=DIRECTION ( 'NONE',  ( -1.000000000000000000, -0.000000000000000000, -0.000000000000000000 ) ) ;
#50084=ORIENTED_EDGE ( 'NONE', *, *, #28681, .T. ) ;
#50085=LINE ( 'NONE', #16021, #33758 ) ;
#50086=( BOUNDED_CURVE ( )  B_SPLINE_CURVE ( 3, ( #41878, #13905, #22372, #41379 ),
 .UNSPECIFIED., .F., .F. ) 
 B_SPLINE_CURVE_WITH_KNOTS ( ( 4, 4 ),
 ( 4.712388980384689674, 6.283185307179586232 ),
 .UNSPECIFIED. ) 
 CURVE ( )  GEOMETRIC_REPRESENTATION_ITEM ( )  RATIONAL_B_SPLINE_CURVE ( ( 1.000000000000000000, 0.8047378541243649375, 0.8047378541243649375, 1.000000000000000000 ) ) 
 REPRESENTATION_ITEM ( '' )  );
#50088=CARTESIAN_POINT ( 'NONE',  ( 33.30402655318503946, 1.750000000000009992, -159.1817124430720298 ) ) ;
#50097=( BOUNDED_CURVE ( )  B_SPLINE_CURVE ( 3, ( #2232, #17869, #45800, #45299 ),
 .UNSPECIFIED., .F., .F. ) 
 B_SPLINE_CURVE_WITH_KNOTS ( ( 4, 4 ),
 ( 0.000000000000000000, 1.570796326794896558 ),
 .UNSPECIFIED. ) 
 CURVE ( )  GEOMETRIC_REPRESENTATION_ITEM ( )  RATIONAL_B_SPLINE_CURVE ( ( 1.000000000000000000, 0.8047378541243649375, 0.8047378541243649375, 1.000000000000000000 ) ) 
 REPRESENTATION_ITEM ( '' )  );
#50106=AXIS2_PLACEMENT_3D ( 'NONE', #49178, #14830, #45344 ) ;
#50107=VERTEX_POINT ( 'NONE', #17112 ) ;
#50111=CARTESIAN_POINT ( 'NONE',  ( 73.30402655318508209, 0.000000000000000000, 165.0000000000000000 ) ) ;
#50115=DIRECTION ( 'NONE',  ( 1.000000000000000000, 0.000000000000000000, 0.000000000000000000 ) ) ;
#50116=CARTESIAN_POINT ( 'NONE',  ( 194.3291528190321742, -1.750000000000009548, -38.15658617722494483 ) ) ;
#50120=VECTOR ( 'NONE', #47514, 1000.000000000000000 ) ;
#50122=DIRECTION ( 'NONE',  ( -1.000000000000000000, -0.000000000000000000, -0.000000000000000000 ) ) ;
#50123=DIRECTION ( 'NONE',  ( -1.000000000000000000, -0.000000000000000000, -0.000000000000000000 ) ) ;
#50124=LINE ( 'NONE', #26836, #30847 ) ;
#50125=ORIENTED_EDGE ( 'NONE', *, *, #5488, .F. ) ;
#50128=CARTESIAN_POINT ( 'NONE',  ( 73.30402655318508209, 1.750000000000010214, -39.18171244307202983 ) ) ;
#50130=VERTEX_POINT ( 'NONE', #32775 ) ;
#50132=CARTESIAN_POINT ( 'NONE',  ( 113.3040265531850537, 1.749999999999996891, 160.8182875569279702 ) ) ;
#50133=DIRECTION ( 'NONE',  ( 0.000000000000000000, 0.000000000000000000, 1.000000000000000000 ) ) ;
#50137=ADVANCED_FACE ( 'NONE', ( #40724 ), #5560, .T. ) ;
#50138=DIRECTION ( 'NONE',  ( 1.000000000000000000, 0.000000000000000000, 0.000000000000000000 ) ) ;
#50139=CARTESIAN_POINT ( 'NONE',  ( 210.0000000000000568, 0.000000000000000000, -79.18171244307201562 ) ) ;
#50140=FACE_OUTER_BOUND ( 'NONE', #14667, .T. ) ;
#50141=CARTESIAN_POINT ( 'NONE',  ( 35.05402655318504657, -1.025126265847089213, -37.43171244307202272 ) ) ;
#50149=DIRECTION ( 'NONE',  ( -0.000000000000000000, -0.000000000000000000, -1.000000000000000000 ) ) ;
#50159=VERTEX_POINT ( 'NONE', #29176 ) ;
#50169=ORIENTED_EDGE ( 'NONE', *, *, #3410, .F. ) ;
#50170=DIRECTION ( 'NONE',  ( 0.000000000000000000, 0.000000000000000000, 1.000000000000000000 ) ) ;
#50174=( BOUNDED_CURVE ( )  B_SPLINE_CURVE ( 3, ( #7363, #42001, #10444, #10692 ),
 .UNSPECIFIED., .F., .F. ) 
 B_SPLINE_CURVE_WITH_KNOTS ( ( 4, 4 ),
 ( 3.141592653589793116, 4.712388980384689674 ),
 .UNSPECIFIED. ) 
 CURVE ( )  GEOMETRIC_REPRESENTATION_ITEM ( )  RATIONAL_B_SPLINE_CURVE ( ( 1.000000000000000000, 0.8047378541243649375, 0.8047378541243649375, 1.000000000000000000 ) ) 
 REPRESENTATION_ITEM ( '' )  );
#50176=CARTESIAN_POINT ( 'NONE',  ( 75.05402655318509630, 2.143131898507880377E-16, 79.06828755692797017 ) ) ;
#50177=ORIENTED_EDGE ( 'NONE', *, *, #11534, .T. ) ;
#50181=CARTESIAN_POINT ( 'NONE',  ( 113.3040265531850537, 1.749999999999996891, 160.8182875569279702 ) ) ;
#50182=EDGE_LOOP ( 'NONE', ( #9458, #34103, #47153, #50188, #36632, #10817 ) ) ;
#50188=ORIENTED_EDGE ( 'NONE', *, *, #20827, .T. ) ;
#50198=CYLINDRICAL_SURFACE ( 'NONE', #13226, 1.750000000000015543 ) ;
#50201=FACE_OUTER_BOUND ( 'NONE', #10225, .T. ) ;
#50214=CARTESIAN_POINT ( 'NONE',  ( 111.5540265531850537, 2.143131898507880377E-16, -160.9317124430720298 ) ) ;
#50215=CARTESIAN_POINT ( 'NONE',  ( 153.3040265531850537, 0.000000000000000000, 165.0000000000000000 ) ) ;
#50227=DIRECTION ( 'NONE',  ( 0.000000000000000000, 0.000000000000000000, 1.000000000000000000 ) ) ;
#50228=ORIENTED_EDGE ( 'NONE', *, *, #49113, .T. ) ;
#50235=( BOUNDED_CURVE ( )  B_SPLINE_CURVE ( 3, ( #19881, #12193, #12437, #40411 ),
 .UNSPECIFIED., .F., .F. ) 
 B_SPLINE_CURVE_WITH_KNOTS ( ( 4, 4 ),
 ( 4.712388980384689674, 6.283185307179586232 ),
 .UNSPECIFIED. ) 
 CURVE ( )  GEOMETRIC_REPRESENTATION_ITEM ( )  RATIONAL_B_SPLINE_CURVE ( ( 1.000000000000000000, 0.8047378541243649375, 0.8047378541243649375, 1.000000000000000000 ) ) 
 REPRESENTATION_ITEM ( '' )  );
#50237=CARTESIAN_POINT ( 'NONE',  ( 193.3040265531851105, -1.750000000000010658, -79.18171244307201562 ) ) ;
#50239=VERTEX_POINT ( 'NONE', #30690 ) ;
#50240=CARTESIAN_POINT ( 'NONE',  ( -166.6959734468149463, 0.000000000000000000, 165.0000000000000000 ) ) ;
#50243=( BOUNDED_CURVE ( )  B_SPLINE_CURVE ( 3, ( #22030, #38221, #45846, #10993 ),
 .UNSPECIFIED., .F., .F. ) 
 B_SPLINE_CURVE_WITH_KNOTS ( ( 4, 4 ),
 ( 0.000000000000000000, 1.570796326794896558 ),
 .UNSPECIFIED. ) 
 CURVE ( )  GEOMETRIC_REPRESENTATION_ITEM ( )  RATIONAL_B_SPLINE_CURVE ( ( 1.000000000000000000, 0.8047378541243649375, 0.8047378541243649375, 1.000000000000000000 ) ) 
 REPRESENTATION_ITEM ( '' )  );
#50247=CARTESIAN_POINT ( 'NONE',  ( -86.69597344681494633, -1.750000000000010214, -39.18171244307202983 ) ) ;
#50250=CARTESIAN_POINT ( 'NONE',  ( -88.44597344681491791, 0.000000000000000000, 162.5682875569279702 ) ) ;
#50255=EDGE_CURVE ( 'NONE', #46979, #29314, #46293, .T. ) ;
#50257=EDGE_CURVE ( 'NONE', #44495, #29622, #10965, .T. ) ;
#50262=AXIS2_PLACEMENT_3D ( 'NONE', #31835, #47420, #12307 ) ;
#50263=ORIENTED_EDGE ( 'NONE', *, *, #28630, .F. ) ;
#50264=AXIS2_PLACEMENT_3D ( 'NONE', #1221, #29170, #9152 ) ;
#50266=EDGE_CURVE ( 'NONE', #46387, #20835, #16228, .T. ) ;
#50275=CARTESIAN_POINT ( 'NONE',  ( -124.9459734468149463, 2.143131898507847836E-16, 82.56828755692797017 ) ) ;
#50286=AXIS2_PLACEMENT_3D ( 'NONE', #12161, #39377, #19595 ) ;
#50295=CARTESIAN_POINT ( 'NONE',  ( 33.30402655318503946, 1.750000000000010214, 40.81828755692798438 ) ) ;
#50299=CARTESIAN_POINT ( 'NONE',  ( -164.9459734468149463, 2.143131898507880377E-16, -80.93171244307201562 ) ) ;
#50300=DIRECTION ( 'NONE',  ( -0.000000000000000000, -0.000000000000000000, -1.000000000000000000 ) ) ;
#50301=ORIENTED_EDGE ( 'NONE', *, *, #7691, .F. ) ;
#50302=CARTESIAN_POINT ( 'NONE',  ( -44.94597344681493922, 1.025126265847089435, 39.06828755692797728 ) ) ;
#50307=CARTESIAN_POINT ( 'NONE',  ( 153.3040265531850537, 1.750000000000010214, -39.18171244307202983 ) ) ;
#50308=VECTOR ( 'NONE', #6587, 1000.000000000000000 ) ;
#50309=CARTESIAN_POINT ( 'NONE',  ( 111.5540265531850537, -1.025126265847082108, -77.43171244307201562 ) ) ;
#50311=EDGE_LOOP ( 'NONE', ( #3477, #25907, #36639, #11673, #42916, #383 ) ) ;
#50313=CARTESIAN_POINT ( 'NONE',  ( 210.0000000000000568, 0.000000000000000000, 0.8182875569279768335 ) ) ;
#50315=ADVANCED_FACE ( 'NONE', ( #10088 ), #48794, .F. ) ;
#50316=ORIENTED_EDGE ( 'NONE', *, *, #12725, .T. ) ;
#50322=EDGE_CURVE ( 'NONE', #26096, #19789, #21449, .T. ) ;
#50327=SHAPE_REPRESENTATION ( 'wire', ( #45486 ), #43870 ) ;
#50328=ORIENTED_EDGE ( 'NONE', *, *, #44930, .F. ) ;
#50332=CYLINDRICAL_SURFACE ( 'NONE', #19123, 1.750000000000008438 ) ;
#50334=VERTEX_POINT ( 'NONE', #20877 ) ;
#50337=EDGE_CURVE ( 'NONE', #26504, #36589, #31971, .T. ) ;
#50342=DIRECTION ( 'NONE',  ( -1.000000000000000000, -0.000000000000000000, -0.000000000000000000 ) ) ;
#50352=DIRECTION ( 'NONE',  ( -0.000000000000000000, -0.000000000000000000, -1.000000000000000000 ) ) ;
#50353=AXIS2_PLACEMENT_3D ( 'NONE', #2290, #45857, #33358 ) ;
#50360=VERTEX_POINT ( 'NONE', #32956 ) ;
#50369=CARTESIAN_POINT ( 'NONE',  ( 74.32915281903215998, 1.750000000000009548, 41.84341382277508359 ) ) ;
#50379=ORIENTED_EDGE ( 'NONE', *, *, #48489, .F. ) ;
#50384=CARTESIAN_POINT ( 'NONE',  ( -6.695973446814940111, -1.750000000000024203, 120.8182875569279702 ) ) ;
#50386=( BOUNDED_CURVE ( )  B_SPLINE_CURVE ( 3, ( #2480, #9674, #29426, #14272 ),
 .UNSPECIFIED., .F., .F. ) 
 B_SPLINE_CURVE_WITH_KNOTS ( ( 4, 4 ),
 ( 0.000000000000000000, 1.570796326794896558 ),
 .UNSPECIFIED. ) 
 CURVE ( )  GEOMETRIC_REPRESENTATION_ITEM ( )  RATIONAL_B_SPLINE_CURVE ( ( 1.000000000000000000, 0.8047378541243649375, 0.8047378541243649375, 1.000000000000000000 ) ) 
 REPRESENTATION_ITEM ( '' )  );
#50388=EDGE_CURVE ( 'NONE', #9299, #21262, #36559, .T. ) ;
#50389=DIRECTION ( 'NONE',  ( 1.000000000000000000, 0.000000000000000000, 0.000000000000000000 ) ) ;
#50391=LINE ( 'NONE', #11441, #26598 ) ;
#50392=CARTESIAN_POINT ( 'NONE',  ( 112.2789002873379758, 1.749999999999996669, -118.1565861772249661 ) ) ;
#50394=EDGE_LOOP ( 'NONE', ( #45153, #14380, #48674, #36270, #17794, #531 ) ) ;
#50395=DIRECTION ( 'NONE',  ( 1.000000000000000000, 0.000000000000000000, 0.000000000000000000 ) ) ;
#50396=( BOUNDED_CURVE ( )  B_SPLINE_CURVE ( 3, ( #40740, #28928, #44302, #28436 ),
 .UNSPECIFIED., .F., .F. ) 
 B_SPLINE_CURVE_WITH_KNOTS ( ( 4, 4 ),
 ( 3.141592653589793116, 4.712388980384689674 ),
 .UNSPECIFIED. ) 
 CURVE ( )  GEOMETRIC_REPRESENTATION_ITEM ( )  RATIONAL_B_SPLINE_CURVE ( ( 1.000000000000000000, 0.8047378541243649375, 0.8047378541243649375, 1.000000000000000000 ) ) 
 REPRESENTATION_ITEM ( '' )  );
#50398=DIRECTION ( 'NONE',  ( -1.000000000000000000, -0.000000000000000000, -0.000000000000000000 ) ) ;
#50404=EDGE_CURVE ( 'NONE', #6144, #7014, #30016, .T. ) ;
#50405=AXIS2_PLACEMENT_3D ( 'NONE', #28281, #43916, #13629 ) ;
#50416=( BOUNDED_CURVE ( )  B_SPLINE_CURVE ( 3, ( #9788, #24957, #25198, #5945 ),
 .UNSPECIFIED., .F., .F. ) 
 B_SPLINE_CURVE_WITH_KNOTS ( ( 4, 4 ),
 ( 0.000000000000000000, 1.570796326794896558 ),
 .UNSPECIFIED. ) 
 CURVE ( )  GEOMETRIC_REPRESENTATION_ITEM ( )  RATIONAL_B_SPLINE_CURVE ( ( 1.000000000000000000, 0.8047378541243649375, 0.8047378541243649375, 1.000000000000000000 ) ) 
 REPRESENTATION_ITEM ( '' )  );
#50418=CARTESIAN_POINT ( 'NONE',  ( -44.94597344681493922, 2.143131898507882349E-16, 165.0000000000000000 ) ) ;
#50422=DIRECTION ( 'NONE',  ( -1.000000000000000000, -0.000000000000000000, -0.000000000000000000 ) ) ;
#50431=CARTESIAN_POINT ( 'NONE',  ( -86.69597344681494633, 1.750000000000010214, -39.18171244307202983 ) ) ;
#50433=VERTEX_POINT ( 'NONE', #23055 ) ;
#50436=EDGE_CURVE ( 'NONE', #25384, #4446, #48974, .T. ) ;
#50439=VECTOR ( 'NONE', #43355, 1000.000000000000000 ) ;
#50442=CARTESIAN_POINT ( 'NONE',  ( -127.7210997126620242, 1.749999999999996669, 161.8434138227750907 ) ) ;
#50447=CARTESIAN_POINT ( 'NONE',  ( -128.4459734468149179, 0.000000000000000000, -157.4317124430720582 ) ) ;
#50451=ORIENTED_EDGE ( 'NONE', *, *, #22677, .T. ) ;
#50452=CARTESIAN_POINT ( 'NONE',  ( -168.4459734468149747, -1.025126265847089657, 42.56828755692799149 ) ) ;
#50454=ORIENTED_EDGE ( 'NONE', *, *, #7011, .T. ) ;
#50456=ORIENTED_EDGE ( 'NONE', *, *, #22132, .T. ) ;
#50464=CARTESIAN_POINT ( 'NONE',  ( -126.6959734468149321, 1.749999999999996891, -159.1817124430720298 ) ) ;
#50468=EDGE_CURVE ( 'NONE', #40222, #7778, #42051, .T. ) ;
#50474=CARTESIAN_POINT ( 'NONE',  ( 210.0000000000000568, 0.000000000000000000, 122.5682875569279844 ) ) ;
#50475=VECTOR ( 'NONE', #32850, 1000.000000000000000 ) ;
#50478=CYLINDRICAL_SURFACE ( 'NONE', #15832, 1.750000000000008438 ) ;
#50479=VERTEX_POINT ( 'NONE', #7427 ) ;
#50486=DIRECTION ( 'NONE',  ( -0.000000000000000000, -0.000000000000000000, -1.000000000000000000 ) ) ;
#50488=CARTESIAN_POINT ( 'NONE',  ( 75.05402655318509630, 2.143131898507880377E-16, 159.0682875569279702 ) ) ;
#50494=ORIENTED_EDGE ( 'NONE', *, *, #49365, .F. ) ;
#50496=EDGE_CURVE ( 'NONE', #18024, #25772, #40500, .T. ) ;
#50497=ORIENTED_EDGE ( 'NONE', *, *, #38535, .T. ) ;
#50508=CIRCLE ( 'NONE', #2215, 1.750000000000008438 ) ;
#50509=CARTESIAN_POINT ( 'NONE',  ( -166.6959734468149463, 1.750000000000010214, -39.18171244307202983 ) ) ;
#50511=ORIENTED_EDGE ( 'NONE', *, *, #5097, .T. ) ;
#50512=DIRECTION ( 'NONE',  ( -1.000000000000000000, -0.000000000000000000, -0.000000000000000000 ) ) ;
#50513=DIRECTION ( 'NONE',  ( 0.000000000000000000, 0.000000000000000000, 1.000000000000000000 ) ) ;
#50515=CARTESIAN_POINT ( 'NONE',  ( 210.0000000000000568, 2.143131898507880377E-16, -0.9317124430720331585 ) ) ;
#50520=CARTESIAN_POINT ( 'NONE',  ( 73.30402655318508209, 0.000000000000000000, 165.0000000000000000 ) ) ;
#50521=CARTESIAN_POINT ( 'NONE',  ( 195.0540265531851105, 2.143131898507880377E-16, 162.5682875569279702 ) ) ;
#50525=EDGE_CURVE ( 'NONE', #11488, #13632, #50634, .T. ) ;
#50529=CARTESIAN_POINT ( 'NONE',  ( 31.55402655318503236, 0.000000000000000000, 39.06828755692798438 ) ) ;
#50531=FACE_OUTER_BOUND ( 'NONE', #2899, .T. ) ;
#50533=LINE ( 'NONE', #46695, #19890 ) ;
#50537=EDGE_CURVE ( 'NONE', #39708, #45594, #7675, .T. ) ;
#50538=DIRECTION ( 'NONE',  ( -1.000000000000000000, -0.000000000000000000, -0.000000000000000000 ) ) ;
#50539=CARTESIAN_POINT ( 'NONE',  ( -165.6708471809677974, 1.750000000000009548, 159.7931612910809065 ) ) ;
#50549=FACE_OUTER_BOUND ( 'NONE', #3085, .T. ) ;
#50550=( BOUNDED_CURVE ( )  B_SPLINE_CURVE ( 3, ( #12211, #423, #36345, #24284 ),
 .UNSPECIFIED., .F., .F. ) 
 B_SPLINE_CURVE_WITH_KNOTS ( ( 4, 4 ),
 ( 4.712388980384689674, 6.283185307179586232 ),
 .UNSPECIFIED. ) 
 CURVE ( )  GEOMETRIC_REPRESENTATION_ITEM ( )  RATIONAL_B_SPLINE_CURVE ( ( 1.000000000000000000, 0.8047378541243649375, 0.8047378541243649375, 1.000000000000000000 ) ) 
 REPRESENTATION_ITEM ( '' )  );
#50552=CARTESIAN_POINT ( 'NONE',  ( 210.0000000000000568, 0.000000000000000000, -79.18171244307201562 ) ) ;
#50563=CARTESIAN_POINT ( 'NONE',  ( -166.6959734468149463, 0.000000000000000000, 165.0000000000000000 ) ) ;
#50573=FACE_OUTER_BOUND ( 'NONE', #42659, .T. ) ;
#50574=ORIENTED_EDGE ( 'NONE', *, *, #8334, .F. ) ;
#50578=EDGE_CURVE ( 'NONE', #34748, #2812, #29395, .T. ) ;
#50584=EDGE_CURVE ( 'NONE', #23383, #23653, #48826, .T. ) ;
#50588=CARTESIAN_POINT ( 'NONE',  ( -124.9459734468149463, 2.143131898507847836E-16, 159.0682875569279702 ) ) ;
#50593=ORIENTED_EDGE ( 'NONE', *, *, #41613, .T. ) ;
#50596=ORIENTED_EDGE ( 'NONE', *, *, #21596, .F. ) ;
#50600=CARTESIAN_POINT ( 'NONE',  ( 35.05402655318504657, -1.025126265847089435, 162.5682875569279133 ) ) ;
#50601=CARTESIAN_POINT ( 'NONE',  ( -206.6959734468149463, -1.750000000000010214, -39.18171244307202983 ) ) ;
#50602=EDGE_LOOP ( 'NONE', ( #27781, #42005, #228, #42675, #40012, #1219 ) ) ;
#50605=CARTESIAN_POINT ( 'NONE',  ( -84.94597344681494633, 2.143131898507880377E-16, -80.93171244307201562 ) ) ;
#50611=EDGE_CURVE ( 'NONE', #48152, #39727, #19197, .T. ) ;
#50615=CARTESIAN_POINT ( 'NONE',  ( -164.9459734468149463, 1.025126265847089435, -157.4317124430720582 ) ) ;
#50621=EDGE_CURVE ( 'NONE', #40762, #9299, #5422, .T. ) ;
#50623=ADVANCED_FACE ( 'NONE', ( #13965 ), #25782, .T. ) ;
#50627=EDGE_CURVE ( 'NONE', #31049, #40007, #20863, .T. ) ;
#50629=EDGE_LOOP ( 'NONE', ( #17610, #31451, #48726, #20915, #32135, #25249 ) ) ;
#50633=CARTESIAN_POINT ( 'NONE',  ( 111.5540265531850537, -1.025126265847081886, 39.06828755692799149 ) ) ;
#50634=( BOUNDED_CURVE ( )  B_SPLINE_CURVE ( 3, ( #35399, #46875, #34885, #46114 ),
 .UNSPECIFIED., .F., .F. ) 
 B_SPLINE_CURVE_WITH_KNOTS ( ( 4, 4 ),
 ( 1.570796326794896558, 3.141592653589793116 ),
 .UNSPECIFIED. ) 
 CURVE ( )  GEOMETRIC_REPRESENTATION_ITEM ( )  RATIONAL_B_SPLINE_CURVE ( ( 1.000000000000000000, 0.8047378541243649375, 0.8047378541243649375, 1.000000000000000000 ) ) 
 REPRESENTATION_ITEM ( '' )  );
#50647=CYLINDRICAL_SURFACE ( 'NONE', #37723, 1.750000000000008438 ) ;
#50649=CARTESIAN_POINT ( 'NONE',  ( 111.5540265531850537, -1.025126265847081442, -0.9317124430720195027 ) ) ;
#50657=CARTESIAN_POINT ( 'NONE',  ( 114.3291528190321173, 1.749999999999996669, 39.79316129108089228 ) ) ;
#50665=CARTESIAN_POINT ( 'NONE',  ( -128.4459734468149179, 0.000000000000000000, 79.06828755692799859 ) ) ;
#50669=VERTEX_POINT ( 'NONE', #10882 ) ;
#50682=CARTESIAN_POINT ( 'NONE',  ( -86.69597344681494633, 1.750000000000010214, 40.81828755692798438 ) ) ;
#50683=EDGE_CURVE ( 'NONE', #13485, #11294, #29696, .T. ) ;
#50684=ORIENTED_EDGE ( 'NONE', *, *, #4698, .T. ) ;
#50685=CYLINDRICAL_SURFACE ( 'NONE', #29820, 1.750000000000015543 ) ;
#50687=ORIENTED_EDGE ( 'NONE', *, *, #39108, .T. ) ;
#50691=CARTESIAN_POINT ( 'NONE',  ( 193.3040265531851105, -1.750000000000010658, 120.8182875569279702 ) ) ;
#50693=( BOUNDED_CURVE ( )  B_SPLINE_CURVE ( 3, ( #32379, #24936, #40082, #32634 ),
 .UNSPECIFIED., .F., .F. ) 
 B_SPLINE_CURVE_WITH_KNOTS ( ( 4, 4 ),
 ( 4.712388980384689674, 6.283185307179586232 ),
 .UNSPECIFIED. ) 
 CURVE ( )  GEOMETRIC_REPRESENTATION_ITEM ( )  RATIONAL_B_SPLINE_CURVE ( ( 1.000000000000000000, 0.8047378541243649375, 0.8047378541243649375, 1.000000000000000000 ) ) 
 REPRESENTATION_ITEM ( '' )  );
#50695=ORIENTED_EDGE ( 'NONE', *, *, #40930, .F. ) ;
#50699=VECTOR ( 'NONE', #13032, 1000.000000000000000 ) ;
#50704=CARTESIAN_POINT ( 'NONE',  ( -204.9459734468149463, 2.143131898507880377E-16, 119.0682875569279702 ) ) ;
#50711=ORIENTED_EDGE ( 'NONE', *, *, #34369, .T. ) ;
#50714=DIRECTION ( 'NONE',  ( -1.000000000000000000, -0.000000000000000000, -0.000000000000000000 ) ) ;
#50715=( BOUNDED_CURVE ( )  B_SPLINE_CURVE ( 3, ( #26047, #22438, #2927, #18082 ),
 .UNSPECIFIED., .F., .F. ) 
 B_SPLINE_CURVE_WITH_KNOTS ( ( 4, 4 ),
 ( 3.141592653589793116, 4.712388980384689674 ),
 .UNSPECIFIED. ) 
 CURVE ( )  GEOMETRIC_REPRESENTATION_ITEM ( )  RATIONAL_B_SPLINE_CURVE ( ( 1.000000000000000000, 0.8047378541243649375, 0.8047378541243649375, 1.000000000000000000 ) ) 
 REPRESENTATION_ITEM ( '' )  );
#50721=DIRECTION ( 'NONE',  ( -1.000000000000000000, 0.000000000000000000, 0.000000000000000000 ) ) ;
#50748=COLOUR_RGB('Light Blue',0.38,0.62,0.78);
#50749=FILL_AREA_STYLE_COLOUR('',#50748);
#50750=FILL_AREA_STYLE('',(#50749));
#50751=SURFACE_STYLE_FILL_AREA(#50750);
#50752=SURFACE_SIDE_STYLE('',(#50751));
#50753=SURFACE_STYLE_USAGE(.BOTH.,#50752);
#50754=PRESENTATION_STYLE_ASSIGNMENT((#50753));
ENDSEC;
END-ISO-10303-21;
